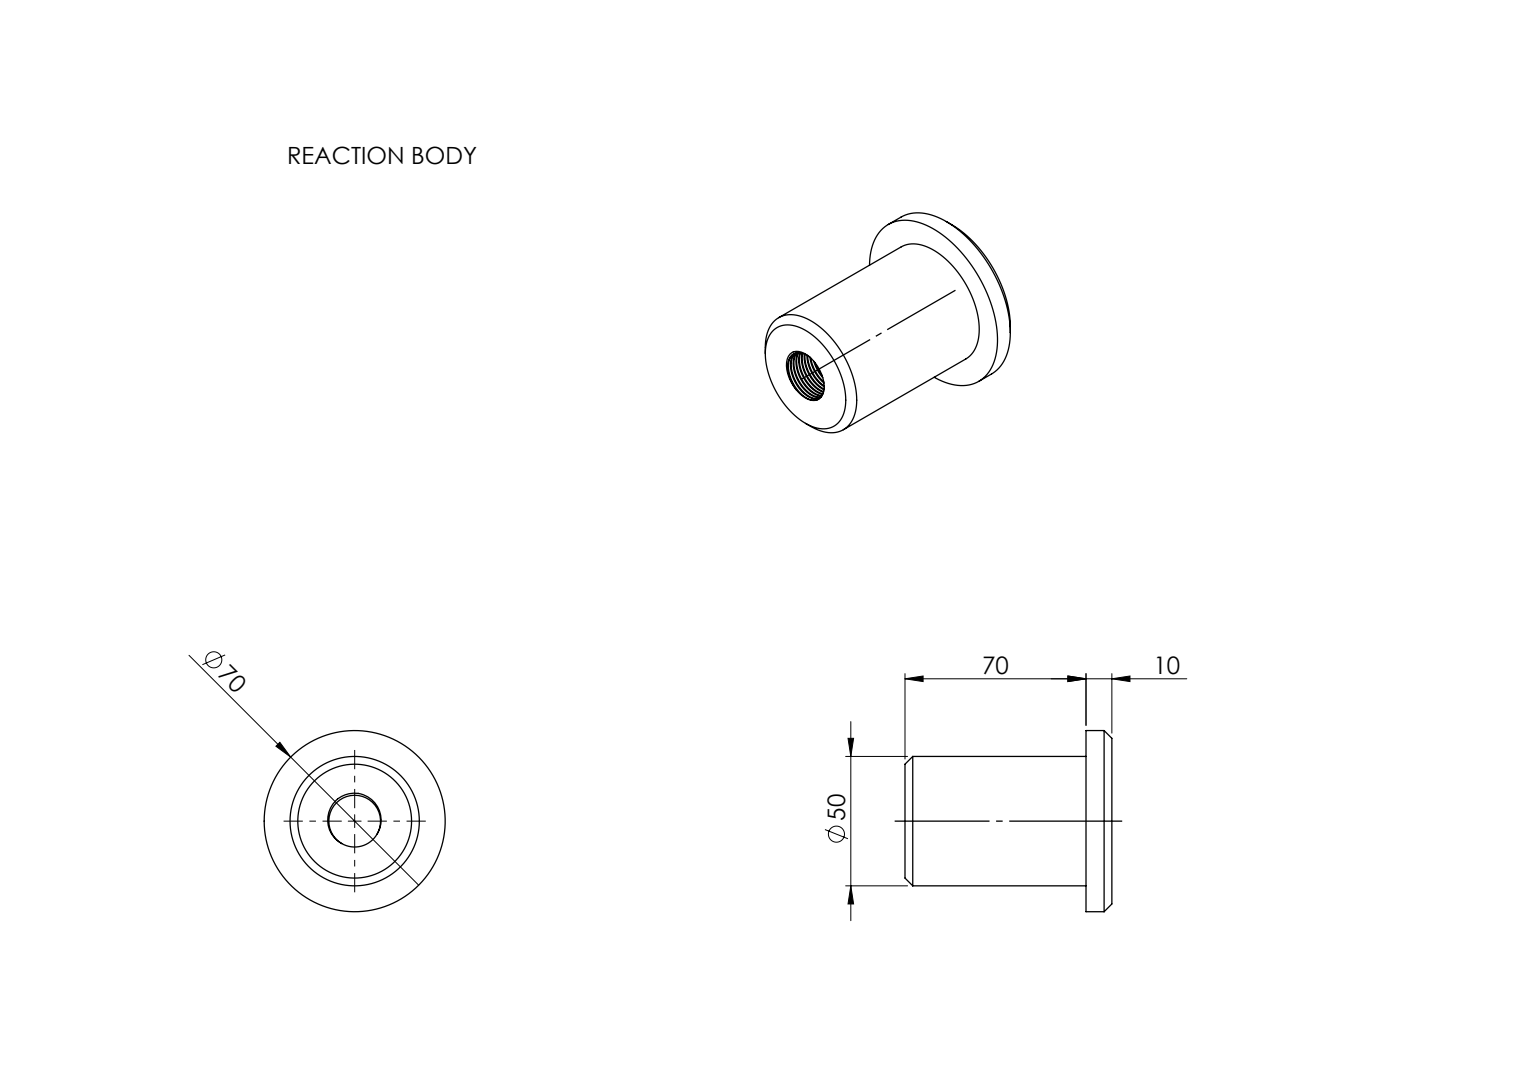
ISO-10303-21;
HEADER;
FILE_DESCRIPTION (('STEP AP203'),
    '1' );
FILE_NAME ('reaction body.step',
    '2026-09-28T05:57:06',
    ( '' ),
    ( '' ),
    'SwSTEP 2.0',
    'SolidWorks 2026',
    '' );
FILE_SCHEMA (( 'AUTOMOTIVE_DESIGN' ));
ENDSEC;

DATA;
#7=DIRECTION ( 'NONE',  ( -0.000000000000000000, -0.000000000000000000, -1.000000000000000000 ) ) ;
#8=CARTESIAN_POINT ( 'NONE',  ( -5.405949406249996869, 9.363379034771805109, -182.5312500020484094 ) ) ;
#10=DIRECTION ( 'NONE',  ( 0.000000000000000000, 0.000000000000000000, -1.000000000000000000 ) ) ;
#13=CARTESIAN_POINT ( 'NONE',  ( 10.81189881249999729, 0.000000000000000000, -100.3437500020483810 ) ) ;
#15=CARTESIAN_POINT ( 'NONE',  ( 10.81189881249999551, -6.242252689847874514, -106.6562500020483952 ) ) ;
#17=CARTESIAN_POINT ( 'NONE',  ( -10.81189881249999729, 6.242252689847871849, -113.2187500020483810 ) ) ;
#21=CARTESIAN_POINT ( 'NONE',  ( 5.000000000000000000, 8.660254037844385522, -142.7500000000000000 ) ) ;
#22=CARTESIAN_POINT ( 'NONE',  ( 4.999999999999992006, -8.660254037844389075, -2.249999999999974243 ) ) ;
#25=CARTESIAN_POINT ( 'NONE',  ( -9.999999999999998224, 5.773502691896259087, -178.7500000040967905 ) ) ;
#27=CARTESIAN_POINT ( 'NONE',  ( 10.81189881249999551, -6.242252689847874514, -29.96875000204834905 ) ) ;
#28=CARTESIAN_POINT ( 'NONE',  ( 5.000000000000000000, 8.660254037844385522, -117.2500000000000000 ) ) ;
#29=CARTESIAN_POINT ( 'NONE',  ( 5.405949406249992428, -9.363379034771808662, -141.0937500020483810 ) ) ;
#31=CARTESIAN_POINT ( 'NONE',  ( -2.293366432827344421E-15, -12.48450537969573659, -37.90625000204836681 ) ) ;
#32=( BOUNDED_CURVE ( )  B_SPLINE_CURVE ( 2, ( #493, #39950, #13606, #30683, #37364, #10382, #33502 ),
 .UNSPECIFIED., .F., .F. ) 
 B_SPLINE_CURVE_WITH_KNOTS ( ( 3, 2, 2, 3 ),
 ( 0.2462686567164180107, 0.2475124378109453960, 0.2487562189054727535, 0.2500000000000001110 ),
 .UNSPECIFIED. ) 
 CURVE ( )  GEOMETRIC_REPRESENTATION_ITEM ( )  RATIONAL_B_SPLINE_CURVE ( ( 0.9999999999999880096, 0.8660254037844506980, 1.000000000000000000, 0.8660254037844387076, 1.000000000000000000, 0.8660254037844267172, 1.000000000000011990 ) ) 
 REPRESENTATION_ITEM ( '' )  );
#34=CARTESIAN_POINT ( 'NONE',  ( 10.00000000000000000, 5.773502691896255534, -67.87500000000000000 ) ) ;
#35=CARTESIAN_POINT ( 'NONE',  ( 10.81189881249999729, 0.000000000000000000, -133.5312500020484094 ) ) ;
#37=ORIENTED_EDGE ( 'NONE', *, *, #14781, .T. ) ;
#38=CARTESIAN_POINT ( 'NONE',  ( -5.000000000000003553, -8.660254037844383745, -128.5000000000000000 ) ) ;
#39=CARTESIAN_POINT ( 'NONE',  ( 10.00000000000000000, 5.773502691896255534, -105.7500000040967905 ) ) ;
#41=CARTESIAN_POINT ( 'NONE',  ( -5.405949406250003975, -9.363379034771801557, -67.84375000204836681 ) ) ;
#47=CARTESIAN_POINT ( 'NONE',  ( 4.999999999999992006, -8.660254037844389075, -37.12500000409676915 ) ) ;
#55=EDGE_LOOP ( 'NONE', ( #10881, #42328, #28621, #40784 ) ) ;
#56=EDGE_CURVE ( 'NONE', #16041, #19819, #26737, .T. ) ;
#64=CARTESIAN_POINT ( 'NONE',  ( -2.293366432827344421E-15, -12.48450537969573659, -127.7187500020483668 ) ) ;
#65=CARTESIAN_POINT ( 'NONE',  ( -5.405949406249996869, 9.363379034771805109, -136.0312500020484094 ) ) ;
#67=CARTESIAN_POINT ( 'NONE',  ( -10.81189881249999729, -6.242252689847864744, -138.4687500020483810 ) ) ;
#68=CARTESIAN_POINT ( 'NONE',  ( 9.877642915644548438, -4.410630136379726451, -179.9999999999999716 ) ) ;
#69=( BOUNDED_CURVE ( )  B_SPLINE_CURVE ( 2, ( #4574, #21398, #14476, #34370, #4786, #36947, #20536 ),
 .UNSPECIFIED., .F., .F. ) 
 B_SPLINE_CURVE_WITH_KNOTS ( ( 3, 2, 2, 3 ),
 ( 0.1455223880597014963, 0.1467661691542288538, 0.1480099502487562391, 0.1492537313432835966 ),
 .UNSPECIFIED. ) 
 CURVE ( )  GEOMETRIC_REPRESENTATION_ITEM ( )  RATIONAL_B_SPLINE_CURVE ( ( 1.000000000000000000, 0.8660254037844387076, 1.000000000000000000, 0.8660254037844387076, 1.000000000000000000, 0.8660254037844357100, 1.000000000000003109 ) ) 
 REPRESENTATION_ITEM ( '' )  );
#70=CARTESIAN_POINT ( 'NONE',  ( 10.00000000000051159, -5.773502691895965988, -102.6249999999999858 ) ) ;
#71=CARTESIAN_POINT ( 'NONE',  ( 7.070501591499377789E-16, 11.54700538379251284, -165.1249999999999716 ) ) ;
#75=CARTESIAN_POINT ( 'NONE',  ( 10.81189881249999551, -6.242252689847874514, -53.96875000204837391 ) ) ;
#77=CARTESIAN_POINT ( 'NONE',  ( -2.293366432827344421E-15, -12.48450537969573659, -159.2187500020483810 ) ) ;
#81=CARTESIAN_POINT ( 'NONE',  ( 0.000000000000000000, 0.000000000000000000, -99.99999999999998579 ) ) ;
#83=CARTESIAN_POINT ( 'NONE',  ( 7.070501591499377789E-16, 11.54700538379251284, -90.12499999999997158 ) ) ;
#84=ORIENTED_EDGE ( 'NONE', *, *, #34120, .T. ) ;
#86=CARTESIAN_POINT ( 'NONE',  ( 5.405949406249992428, -9.363379034771808662, -112.7812500020483952 ) ) ;
#87=CARTESIAN_POINT ( 'NONE',  ( 9.999999999999998224, 0.000000000000000000, -129.8750000040967905 ) ) ;
#88=DIRECTION ( 'NONE',  ( -0.000000000000000000, -0.000000000000000000, -1.000000000000000000 ) ) ;
#92=CARTESIAN_POINT ( 'NONE',  ( -10.81189881249999729, 6.242252689847871849, -62.40625000204838813 ) ) ;
#99=DIRECTION ( 'NONE',  ( -0.000000000000000000, -0.000000000000000000, -1.000000000000000000 ) ) ;
#108=ORIENTED_EDGE ( 'NONE', *, *, #20529, .T. ) ;
#115=FACE_OUTER_BOUND ( 'NONE', #1522, .T. ) ;
#116=CARTESIAN_POINT ( 'NONE',  ( -9.999999999999998224, 1.224646799147353059E-15, -26.74999999999996803 ) ) ;
#120=CARTESIAN_POINT ( 'NONE',  ( -10.81189881249999907, -6.242252689847864744, -147.4687500020484094 ) ) ;
#121=CARTESIAN_POINT ( 'NONE',  ( -5.405949406249996869, 9.363379034771805109, -162.8437500020484094 ) ) ;
#124=CARTESIAN_POINT ( 'NONE',  ( -9.999999999999998224, 1.224646799147353059E-15, -188.7500000000000000 ) ) ;
#128=CARTESIAN_POINT ( 'NONE',  ( 10.81189881249999907, 6.242252689847868297, -184.2187500020483810 ) ) ;
#130=CARTESIAN_POINT ( 'NONE',  ( 5.405949406249992428, -9.363379034771808662, -51.28125000204835970 ) ) ;
#132=CARTESIAN_POINT ( 'NONE',  ( -9.999999999999998224, 1.224646799147353059E-15, -118.2500000000000000 ) ) ;
#135=CARTESIAN_POINT ( 'NONE',  ( -5.405949406249996869, 9.363379034771805109, -142.0312500020483810 ) ) ;
#136=CARTESIAN_POINT ( 'NONE',  ( -10.81189881249999729, 6.242252689847871849, -152.4062500020483810 ) ) ;
#141=CARTESIAN_POINT ( 'NONE',  ( -5.405949406249996869, 9.363379034771805109, -90.84375000204838102 ) ) ;
#142=ORIENTED_EDGE ( 'NONE', *, *, #37948, .T. ) ;
#144=CARTESIAN_POINT ( 'NONE',  ( -10.81189881249999729, 1.324075727343319199E-15, -186.5937500020483810 ) ) ;
#148=CARTESIAN_POINT ( 'NONE',  ( 10.81189881249999551, -6.242252689847874514, -81.15625000204839523 ) ) ;
#150=CARTESIAN_POINT ( 'NONE',  ( 5.000000000000000000, 8.660254037844385522, -57.62500000409676204 ) ) ;
#151=CARTESIAN_POINT ( 'NONE',  ( -10.81189881249999729, 6.242252689847871849, -17.21875000204836681 ) ) ;
#154=CARTESIAN_POINT ( 'NONE',  ( -10.81189881249999729, 6.242252689847871849, -11.40625000204836859 ) ) ;
#156=DIRECTION ( 'NONE',  ( -0.000000000000000000, -0.000000000000000000, -1.000000000000000000 ) ) ;
#158=CARTESIAN_POINT ( 'NONE',  ( 9.999999999999998224, 1.224646799147353059E-15, -99.99999999999998579 ) ) ;
#161=CARTESIAN_POINT ( 'NONE',  ( 0.000000000000000000, 0.000000000000000000, -99.99999999999998579 ) ) ;
#165=CARTESIAN_POINT ( 'NONE',  ( 10.81189881249999729, 6.242252689847867408, -101.7187500020483810 ) ) ;
#168=AXIS2_PLACEMENT_3D ( 'NONE', #1708, #40738, #1276 ) ;
#178=CARTESIAN_POINT ( 'NONE',  ( 5.405949406249999534, 9.363379034771803333, -149.7812500020483810 ) ) ;
#187=CARTESIAN_POINT ( 'NONE',  ( 5.405949406249999534, 9.363379034771803333, -74.59375000204838102 ) ) ;
#188=CARTESIAN_POINT ( 'NONE',  ( -10.81189881249999729, 1.324075727343319199E-15, -83.28125000204838102 ) ) ;
#190=CARTESIAN_POINT ( 'NONE',  ( -10.81189881249999729, -6.242252689847864744, -162.6562500020483810 ) ) ;
#191=CARTESIAN_POINT ( 'NONE',  ( -5.405949406249996869, 9.363379034771805109, -181.0312500020483810 ) ) ;
#192=CARTESIAN_POINT ( 'NONE',  ( -4.999999999999996447, 8.660254037844387298, -159.3750000040967905 ) ) ;
#194=CARTESIAN_POINT ( 'NONE',  ( -5.405949406250003975, -9.363379034771801557, -9.343750002048345493 ) ) ;
#196=CARTESIAN_POINT ( 'NONE',  ( -10.81189881249999729, 1.324075727343319199E-15, -113.0937500020483810 ) ) ;
#198=CARTESIAN_POINT ( 'NONE',  ( 10.81189881249999729, 0.000000000000000000, -13.53125000204835615 ) ) ;
#201=CARTESIAN_POINT ( 'NONE',  ( 5.405949406249999534, 9.363379034771803333, -112.2812500020483952 ) ) ;
#205=CARTESIAN_POINT ( 'NONE',  ( 9.999999999999996447, -5.773502691896262640, -83.50000000409676204 ) ) ;
#206=CARTESIAN_POINT ( 'NONE',  ( 9.999999999999742428, 5.773502691896404748, -134.2500000040967905 ) ) ;
#207=CARTESIAN_POINT ( 'NONE',  ( -10.81189881249999729, 1.324075727343319199E-15, -44.09375000204837391 ) ) ;
#208=ORIENTED_EDGE ( 'NONE', *, *, #27661, .F. ) ;
#212=CARTESIAN_POINT ( 'NONE',  ( 9.999999999999996447, -5.773502691896262640, -10.00000000409676026 ) ) ;
#215=CARTESIAN_POINT ( 'NONE',  ( 9.999999999999998224, 0.000000000000000000, -123.5000000000000000 ) ) ;
#218=ORIENTED_EDGE ( 'NONE', *, *, #5122, .T. ) ;
#223=VERTEX_POINT ( 'NONE', #23443 ) ;
#226=CARTESIAN_POINT ( 'NONE',  ( 10.81189881249999907, 6.242252689847868297, -182.9062500020484094 ) ) ;
#229=CARTESIAN_POINT ( 'NONE',  ( -5.405949406250003975, -9.363379034771801557, -102.3437500020483810 ) ) ;
#231=CARTESIAN_POINT ( 'NONE',  ( 10.81189881249999729, 0.000000000000000000, -105.0312500020483810 ) ) ;
#233=CARTESIAN_POINT ( 'NONE',  ( -5.405949406250003975, -9.363379034771801557, -115.8437500020483810 ) ) ;
#237=CARTESIAN_POINT ( 'NONE',  ( -9.999999999999998224, 1.224646799147353059E-15, -134.7499999999999716 ) ) ;
#238=CARTESIAN_POINT ( 'NONE',  ( -4.999999999999996447, 8.660254037844387298, -7.499999999999978684 ) ) ;
#241=CARTESIAN_POINT ( 'NONE',  ( -10.00000000000000000, -5.773502691896251982, -181.5000000040967905 ) ) ;
#243=CARTESIAN_POINT ( 'NONE',  ( 5.405949406249999534, 9.363379034771803333, -31.09375000204836326 ) ) ;
#245=CARTESIAN_POINT ( 'NONE',  ( 10.81189881249999907, 6.242252689847868297, -134.7187500020484094 ) ) ;
#247=CARTESIAN_POINT ( 'NONE',  ( 10.81189881249999729, 0.000000000000000000, -40.53125000204838102 ) ) ;
#249=CARTESIAN_POINT ( 'NONE',  ( 9.999999999999996447, -5.773502691896262640, -63.62499999999999289 ) ) ;
#250=CARTESIAN_POINT ( 'NONE',  ( 5.405949406249999534, 9.363379034771803333, -136.2812500020483810 ) ) ;
#253=ORIENTED_EDGE ( 'NONE', *, *, #28926, .T. ) ;
#254=CARTESIAN_POINT ( 'NONE',  ( -10.00000000000051337, 5.773502691895962435, -142.3750000000000000 ) ) ;
#255=CARTESIAN_POINT ( 'NONE',  ( -9.999999999999998224, 5.773502691896259087, -105.2500000040967763 ) ) ;
#256=CARTESIAN_POINT ( 'NONE',  ( -2.121150477449813534E-15, -11.54700538379251284, -146.3749999999999716 ) ) ;
#257=CARTESIAN_POINT ( 'NONE',  ( 10.81189881249999551, -6.242252689847874514, -67.46875000204838102 ) ) ;
#263=CARTESIAN_POINT ( 'NONE',  ( -10.00000000000000000, -5.773502691896251982, -39.00000000409676204 ) ) ;
#269=EDGE_CURVE ( 'NONE', #8961, #22977, #32528, .T. ) ;
#270=VERTEX_POINT ( 'NONE', #36591 ) ;
#274=CARTESIAN_POINT ( 'NONE',  ( 9.999999999999227285, 5.773502691896701400, -111.7500000040967478 ) ) ;
#279=CARTESIAN_POINT ( 'NONE',  ( -10.81189881249999729, 6.242252689847871849, -125.2187500020483810 ) ) ;
#280=CARTESIAN_POINT ( 'NONE',  ( 7.644554776091147741E-16, 12.48450537969573659, -128.6562500020483810 ) ) ;
#282=CARTESIAN_POINT ( 'NONE',  ( 10.81189881249999551, -6.242252689847874514, -139.4687500020483810 ) ) ;
#283=CARTESIAN_POINT ( 'NONE',  ( 10.64016988090102700, -2.046480638857292256, -180.0000000000000000 ) ) ;
#285=CARTESIAN_POINT ( 'NONE',  ( 7.070501591499377789E-16, 11.54700538379251284, -159.1250000000000000 ) ) ;
#286=CARTESIAN_POINT ( 'NONE',  ( -10.81189881249999729, 1.324075727343319199E-15, -0.7812500020483725827 ) ) ;
#289=CARTESIAN_POINT ( 'NONE',  ( -5.405949406249996869, 9.363379034771805109, -51.84375000204835260 ) ) ;
#291=CARTESIAN_POINT ( 'NONE',  ( 10.81189881249999551, -6.242252689847874514, -158.9687500020484094 ) ) ;
#296=CARTESIAN_POINT ( 'NONE',  ( -9.999999999999998224, 5.773502691896259087, -92.87500000000000000 ) ) ;
#297=ORIENTED_EDGE ( 'NONE', *, *, #13005, .T. ) ;
#298=CARTESIAN_POINT ( 'NONE',  ( -2.293366432827344421E-15, -12.48450537969573659, -112.9062500020483952 ) ) ;
#299=CARTESIAN_POINT ( 'NONE',  ( 10.00000000000000000, 5.773502691896255534, -128.2500000040967620 ) ) ;
#303=EDGE_CURVE ( 'NONE', #6776, #24567, #9100, .T. ) ;
#305=CARTESIAN_POINT ( 'NONE',  ( 5.405949406249999534, 9.363379034771803333, -50.78125000204835970 ) ) ;
#312=CARTESIAN_POINT ( 'NONE',  ( -4.999999999999996447, 8.660254037844387298, -130.8750000040967905 ) ) ;
#320=( BOUNDED_CURVE ( )  B_SPLINE_CURVE ( 2, ( #6511, #29389, #19660, #35453, #2432, #8903, #15567 ),
 .UNSPECIFIED., .F., .F. ) 
 B_SPLINE_CURVE_WITH_KNOTS ( ( 3, 2, 2, 3 ),
 ( 0.3955223880597015795, 0.3967661691542289648, 0.3980099502487563501, 0.3992537313432836799 ),
 .UNSPECIFIED. ) 
 CURVE ( )  GEOMETRIC_REPRESENTATION_ITEM ( )  RATIONAL_B_SPLINE_CURVE ( ( 0.9999999999999880096, 0.8660254037844506980, 1.000000000000000000, 0.8660254037844387076, 1.000000000000000000, 0.8660254037844267172, 1.000000000000011990 ) ) 
 REPRESENTATION_ITEM ( '' )  );
#327=CARTESIAN_POINT ( 'NONE',  ( -5.405949406249996869, 9.363379034771805109, -146.3437500020483810 ) ) ;
#328=CARTESIAN_POINT ( 'NONE',  ( 5.405949406249999534, 9.363379034771803333, -163.0937500020484094 ) ) ;
#330=( BOUNDED_CURVE ( )  B_SPLINE_CURVE ( 2, ( #4756, #1316, #14448, #8439, #17905, #11862, #34553 ),
 .UNSPECIFIED., .F., .F. ) 
 B_SPLINE_CURVE_WITH_KNOTS ( ( 3, 2, 2, 3 ),
 ( 0.1567164179104477695, 0.1579601990049751270, 0.1592039800995025123, 0.1604477611940298698 ),
 .UNSPECIFIED. ) 
 CURVE ( )  GEOMETRIC_REPRESENTATION_ITEM ( )  RATIONAL_B_SPLINE_CURVE ( ( 1.000000000000000000, 0.8660254037844387076, 1.000000000000000000, 0.8660254037844387076, 1.000000000000000000, 0.8660254037844357100, 1.000000000000003109 ) ) 
 REPRESENTATION_ITEM ( '' )  );
#331=FACE_OUTER_BOUND ( 'NONE', #10477, .T. ) ;
#332=CARTESIAN_POINT ( 'NONE',  ( -5.000000000000003553, -8.660254037844383745, -188.5000000000000000 ) ) ;
#335=CYLINDRICAL_SURFACE ( 'NONE', #35072, 9.999999999999998224 ) ;
#336=CARTESIAN_POINT ( 'NONE',  ( 7.644554776091147741E-16, 12.48450537969573659, -183.9687500020484094 ) ) ;
#339=CARTESIAN_POINT ( 'NONE',  ( 7.644554776091147741E-16, 12.48450537969573659, -50.65625000204837391 ) ) ;
#341=CARTESIAN_POINT ( 'NONE',  ( 5.000000000000000000, 8.660254037844385522, -112.7499999999999858 ) ) ;
#342=VERTEX_POINT ( 'NONE', #10257 ) ;
#344=CARTESIAN_POINT ( 'NONE',  ( 7.644554776091147741E-16, 12.48450537969573659, -137.6562500020484094 ) ) ;
#345=CARTESIAN_POINT ( 'NONE',  ( -10.81189881249999729, 1.324075727343319199E-15, -152.2812500020484094 ) ) ;
#347=CARTESIAN_POINT ( 'NONE',  ( -9.999999999999998224, 1.224646799147353059E-15, -125.7499999999999716 ) ) ;
#348=CARTESIAN_POINT ( 'NONE',  ( 10.81189881249999907, 6.242252689847868297, -82.21875000204836681 ) ) ;
#349=ORIENTED_EDGE ( 'NONE', *, *, #20808, .F. ) ;
#351=CARTESIAN_POINT ( 'NONE',  ( -2.293366432827344421E-15, -12.48450537969573659, -181.7187500020484094 ) ) ;
#357=CARTESIAN_POINT ( 'NONE',  ( -5.405949406250003975, -9.363379034771801557, -77.03125000204838102 ) ) ;
#360=CARTESIAN_POINT ( 'NONE',  ( -4.999999999999996447, 8.660254037844387298, -60.37500000409676204 ) ) ;
#361=CARTESIAN_POINT ( 'NONE',  ( 10.81189881249999907, 6.242252689847868297, -8.718750002048359704 ) ) ;
#364=CARTESIAN_POINT ( 'NONE',  ( -10.81189881249999729, 6.242252689847871849, -9.906250002048366810 ) ) ;
#366=CARTESIAN_POINT ( 'NONE',  ( 9.999999999999998224, 0.000000000000000000, -147.8750000040967905 ) ) ;
#369=CARTESIAN_POINT ( 'NONE',  ( -5.000000000000003553, -8.660254037844383745, -134.8750000040967905 ) ) ;
#374=CARTESIAN_POINT ( 'NONE',  ( -9.999999999999998224, 1.224646799147353059E-15, -160.6250000040967905 ) ) ;
#376=CARTESIAN_POINT ( 'NONE',  ( -5.405949406250003975, -9.363379034771801557, -100.8437500020483810 ) ) ;
#378=ORIENTED_EDGE ( 'NONE', *, *, #33115, .F. ) ;
#385=EDGE_CURVE ( 'NONE', #1917, #4764, #24732, .T. ) ;
#390=CARTESIAN_POINT ( 'NONE',  ( 10.81189881249999729, 0.000000000000000000, -145.5312500020483810 ) ) ;
#393=FACE_OUTER_BOUND ( 'NONE', #36030, .T. ) ;
#396=CARTESIAN_POINT ( 'NONE',  ( 10.81189881249999907, 6.242252689847868297, -73.21875000204836681 ) ) ;
#397=CARTESIAN_POINT ( 'NONE',  ( -10.81189881249999729, 1.324075727343319199E-15, -75.78125000204838102 ) ) ;
#399=DIRECTION ( 'NONE',  ( -1.000000000000000000, 0.000000000000000000, 0.000000000000000000 ) ) ;
#400=CARTESIAN_POINT ( 'NONE',  ( -10.81189881249999729, 1.324075727343319199E-15, -156.7812500020484094 ) ) ;
#401=CARTESIAN_POINT ( 'NONE',  ( -2.293366432827344421E-15, -12.48450537969573659, -168.4062500020483810 ) ) ;
#402=DIRECTION ( 'NONE',  ( -0.000000000000000000, -0.000000000000000000, -1.000000000000000000 ) ) ;
#403=CARTESIAN_POINT ( 'NONE',  ( -10.81189881249999729, 6.242252689847871849, -0.7187500020483517105 ) ) ;
#405=CARTESIAN_POINT ( 'NONE',  ( 10.81189881249999551, -6.242252689847874514, -107.9687500020483810 ) ) ;
#407=CARTESIAN_POINT ( 'NONE',  ( 10.81189881249999907, 6.242252689847868297, -13.40625000204837036 ) ) ;
#410=( BOUNDED_CURVE ( )  B_SPLINE_CURVE ( 2, ( #7723, #30182, #3850, #7503, #30606, #17408, #620 ),
 .UNSPECIFIED., .F., .F. ) 
 B_SPLINE_CURVE_WITH_KNOTS ( ( 3, 2, 2, 3 ),
 ( 0.1529850746268656692, 0.1542288557213930267, 0.1554726368159203842, 0.1567164179104477695 ),
 .UNSPECIFIED. ) 
 CURVE ( )  GEOMETRIC_REPRESENTATION_ITEM ( )  RATIONAL_B_SPLINE_CURVE ( ( 1.000000000000000000, 0.8660254037844387076, 1.000000000000000000, 0.8660254037844387076, 1.000000000000000000, 0.8660254037844387076, 1.000000000000000000 ) ) 
 REPRESENTATION_ITEM ( '' )  );
#412=CARTESIAN_POINT ( 'NONE',  ( 10.81189881249999729, 0.000000000000000000, -109.5312500020483810 ) ) ;
#415=ADVANCED_FACE ( 'NONE', ( #31205 ), #992, .F. ) ;
#416=CARTESIAN_POINT ( 'NONE',  ( -9.999999999999998224, 1.224646799147353059E-15, -87.12500000409677625 ) ) ;
#418=CARTESIAN_POINT ( 'NONE',  ( 10.81189881249999907, 6.242252689847868297, -41.71875000204835970 ) ) ;
#422=CARTESIAN_POINT ( 'NONE',  ( 9.999999999999998224, 0.000000000000000000, -140.0000000000000000 ) ) ;
#423=CARTESIAN_POINT ( 'NONE',  ( 4.999999999999992006, -8.660254037844389075, -13.12500000409674783 ) ) ;
#430=ORIENTED_EDGE ( 'NONE', *, *, #34123, .T. ) ;
#438=AXIS2_PLACEMENT_3D ( 'NONE', #20570, #30100, #539 ) ;
#441=CARTESIAN_POINT ( 'NONE',  ( -5.405949406250003975, -9.363379034771801557, -171.5312500020484094 ) ) ;
#442=CARTESIAN_POINT ( 'NONE',  ( -10.00000000000038547, 5.773502691896036154, -154.7500000040967905 ) ) ;
#444=CARTESIAN_POINT ( 'NONE',  ( 5.405949406249999534, 9.363379034771803333, -92.59375000204838102 ) ) ;
#446=CARTESIAN_POINT ( 'NONE',  ( 10.81189881249999907, 6.242252689847868297, -103.4062500020483952 ) ) ;
#448=CARTESIAN_POINT ( 'NONE',  ( -10.81189881249999729, 6.242252689847871849, -116.2187500020483810 ) ) ;
#450=( BOUNDED_CURVE ( )  B_SPLINE_CURVE ( 2, ( #33037, #22265, #38870, #35646, #2628, #12315, #3257 ),
 .UNSPECIFIED., .F., .F. ) 
 B_SPLINE_CURVE_WITH_KNOTS ( ( 3, 2, 2, 3 ),
 ( 0.2462686567164180107, 0.2475124378109453960, 0.2487562189054727535, 0.2500000000000001110 ),
 .UNSPECIFIED. ) 
 CURVE ( )  GEOMETRIC_REPRESENTATION_ITEM ( )  RATIONAL_B_SPLINE_CURVE ( ( 0.9999999999999880096, 0.8660254037844506980, 1.000000000000000000, 0.8660254037844387076, 1.000000000000000000, 0.8660254037844267172, 1.000000000000011990 ) ) 
 REPRESENTATION_ITEM ( '' )  );
#453=CARTESIAN_POINT ( 'NONE',  ( 5.000000000000000000, 8.660254037844385522, -7.749999999999978684 ) ) ;
#456=CARTESIAN_POINT ( 'NONE',  ( 10.00000000000000000, 5.773502691896255534, -180.7500000040968189 ) ) ;
#458=CARTESIAN_POINT ( 'NONE',  ( -5.405949406249996869, 9.363379034771805109, -30.84375000204836326 ) ) ;
#459=DIRECTION ( 'NONE',  ( -0.000000000000000000, -0.000000000000000000, -1.000000000000000000 ) ) ;
#460=CARTESIAN_POINT ( 'NONE',  ( 7.644554776091147741E-16, 12.48450537969573659, -140.4687500020483810 ) ) ;
#462=CARTESIAN_POINT ( 'NONE',  ( -5.405949406250003975, -9.363379034771801557, -38.03125000204838102 ) ) ;
#463=CARTESIAN_POINT ( 'NONE',  ( -5.000000000000003553, -8.660254037844383745, -148.0000000000000000 ) ) ;
#465=CARTESIAN_POINT ( 'NONE',  ( 5.000000000000000000, 8.660254037844385522, -57.24999999999996447 ) ) ;
#466=CARTESIAN_POINT ( 'NONE',  ( -10.81189881249999729, 6.242252689847871849, -128.4062500020484094 ) ) ;
#470=CARTESIAN_POINT ( 'NONE',  ( 7.070501591499377789E-16, 11.54700538379251284, -105.5000000040967763 ) ) ;
#472=CARTESIAN_POINT ( 'NONE',  ( 5.405949406249999534, 9.363379034771803333, -70.09375000204836681 ) ) ;
#478=CARTESIAN_POINT ( 'NONE',  ( -4.999999999999996447, 8.660254037844387298, -37.87500000409676915 ) ) ;
#490=CARTESIAN_POINT ( 'NONE',  ( 7.644554776091147741E-16, 12.48450537969573659, -196.1562500020484379 ) ) ;
#493=CARTESIAN_POINT ( 'NONE',  ( 9.999999999999998224, 0.000000000000000000, -150.5000000000000000 ) ) ;
#497=CARTESIAN_POINT ( 'NONE',  ( 5.405949406249999534, 9.363379034771803333, -127.0937500020483668 ) ) ;
#498=CARTESIAN_POINT ( 'NONE',  ( -10.00000000000000000, -5.773502691896251982, -193.5000000040967905 ) ) ;
#499=CARTESIAN_POINT ( 'NONE',  ( 5.405949406249992428, -9.363379034771808662, -135.2812500020483810 ) ) ;
#501=CARTESIAN_POINT ( 'NONE',  ( -10.81189881249999729, 6.242252689847871849, -135.7187500020483810 ) ) ;
#502=CARTESIAN_POINT ( 'NONE',  ( -2.121150477449813534E-15, -11.54700538379251284, -129.8750000000000000 ) ) ;
#504=CARTESIAN_POINT ( 'NONE',  ( 10.00000000000000000, 5.773502691896255534, -154.8750000000000000 ) ) ;
#508=CARTESIAN_POINT ( 'NONE',  ( -5.405949406249996869, 9.363379034771805109, -56.34375000204835970 ) ) ;
#509=CARTESIAN_POINT ( 'NONE',  ( -9.999999999999998224, 1.224646799147353059E-15, -142.2500000000000000 ) ) ;
#510=CARTESIAN_POINT ( 'NONE',  ( -10.81189881249999729, 6.242252689847871849, -165.7187500020483810 ) ) ;
#514=CARTESIAN_POINT ( 'NONE',  ( 5.000000000000000000, 8.660254037844385522, -87.24999999999998579 ) ) ;
#516=VERTEX_POINT ( 'NONE', #4861 ) ;
#517=CARTESIAN_POINT ( 'NONE',  ( 5.405949406249992428, -9.363379034771808662, -111.2812500020483810 ) ) ;
#518=CARTESIAN_POINT ( 'NONE',  ( 9.999999999999998224, 0.000000000000000000, -135.8750000040967905 ) ) ;
#519=CARTESIAN_POINT ( 'NONE',  ( -10.00000000000019185, -5.773502691896140071, -178.1249999999999432 ) ) ;
#522=CARTESIAN_POINT ( 'NONE',  ( 7.644554776091147741E-16, 12.48450537969573659, -49.15625000204837391 ) ) ;
#528=CARTESIAN_POINT ( 'NONE',  ( 7.070501591499376803E-16, 11.54700538379251284, -131.0000000040967905 ) ) ;
#530=VERTEX_POINT ( 'NONE', #27313 ) ;
#539=DIRECTION ( 'NONE',  ( -1.000000000000000000, 0.000000000000000000, 0.000000000000000000 ) ) ;
#542=CARTESIAN_POINT ( 'NONE',  ( -10.81189881249999907, -6.242252689847864744, -153.4687500020484094 ) ) ;
#543=CARTESIAN_POINT ( 'NONE',  ( 7.644554776091147741E-16, 12.48450537969573659, -164.4687500020483810 ) ) ;
#546=CARTESIAN_POINT ( 'NONE',  ( -4.999999999999996447, 8.660254037844387298, -183.0000000000000000 ) ) ;
#549=CARTESIAN_POINT ( 'NONE',  ( 9.999999999999998224, 0.000000000000000000, -168.8750000040967905 ) ) ;
#550=CARTESIAN_POINT ( 'NONE',  ( -10.81189881249999729, 6.242252689847871849, -188.2187500020483810 ) ) ;
#553=CARTESIAN_POINT ( 'NONE',  ( -10.81189881249999729, 6.242252689847871849, -51.90625000204837391 ) ) ;
#555=CARTESIAN_POINT ( 'NONE',  ( -2.121150477449813534E-15, -11.54700538379251284, -114.8749999999999716 ) ) ;
#556=ORIENTED_EDGE ( 'NONE', *, *, #24143, .F. ) ;
#557=CARTESIAN_POINT ( 'NONE',  ( 10.81189881249999551, -6.242252689847874514, -136.6562500020484094 ) ) ;
#558=CARTESIAN_POINT ( 'NONE',  ( -5.405949406250003975, -9.363379034771801557, -144.5312500020483810 ) ) ;
#560=CARTESIAN_POINT ( 'NONE',  ( -10.81189881249999729, 1.324075727343319199E-15, -80.09375000204838102 ) ) ;
#564=CARTESIAN_POINT ( 'NONE',  ( 5.405949406249992428, -9.363379034771808662, -181.5937500020483810 ) ) ;
#568=CARTESIAN_POINT ( 'NONE',  ( -5.405949406249996869, 9.363379034771805109, -77.53125000204838102 ) ) ;
#571=CARTESIAN_POINT ( 'NONE',  ( -9.999999999999998224, 5.773502691896259087, -49.75000000409676915 ) ) ;
#572=CARTESIAN_POINT ( 'NONE',  ( 10.81189881249999551, -6.242252689847874514, -8.968750002048359704 ) ) ;
#575=CARTESIAN_POINT ( 'NONE',  ( 10.81189881249999729, 0.000000000000000000, -4.531250002048375691 ) ) ;
#577=CARTESIAN_POINT ( 'NONE',  ( 7.320508151741852210, -7.320508031779506375, -100.0669873003032393 ) ) ;
#578=CARTESIAN_POINT ( 'NONE',  ( -9.999999999999227285, -5.773502691896698735, -103.5000000040967336 ) ) ;
#580=( BOUNDED_CURVE ( )  B_SPLINE_CURVE ( 2, ( #41162, #856, #11601, #23943, #21549, #20896, #11392 ),
 .UNSPECIFIED., .F., .F. ) 
 B_SPLINE_CURVE_WITH_KNOTS ( ( 3, 2, 2, 3 ),
 ( 0.4253731343283583266, 0.4266169154228856564, 0.4278606965174130417, 0.4291044776119404269 ),
 .UNSPECIFIED. ) 
 CURVE ( )  GEOMETRIC_REPRESENTATION_ITEM ( )  RATIONAL_B_SPLINE_CURVE ( ( 0.9999999999999880096, 0.8660254037844506980, 1.000000000000000000, 0.8660254037844387076, 1.000000000000000000, 0.8660254037844267172, 1.000000000000011990 ) ) 
 REPRESENTATION_ITEM ( '' )  );
#581=CARTESIAN_POINT ( 'NONE',  ( -9.999999999999998224, 1.224646799147353059E-15, -146.7500000000000000 ) ) ;
#583=ORIENTED_EDGE ( 'NONE', *, *, #23598, .F. ) ;
#585=CARTESIAN_POINT ( 'NONE',  ( 3.516324526667281347, 10.45435446766629894, -100.0500568239963002 ) ) ;
#595=CARTESIAN_POINT ( 'NONE',  ( 4.999999999999992006, -8.660254037844389075, -45.74999999999998579 ) ) ;
#601=CARTESIAN_POINT ( 'NONE',  ( 7.644554776091147741E-16, 12.48450537969573659, -149.6562500020484094 ) ) ;
#603=LINE ( 'NONE', #13718, #29480 ) ;
#608=CARTESIAN_POINT ( 'NONE',  ( -10.81189881249999729, 6.242252689847871849, -72.71875000204835260 ) ) ;
#609=CARTESIAN_POINT ( 'NONE',  ( -5.405949406249996869, 9.363379034771805109, -73.03125000204838102 ) ) ;
#611=CARTESIAN_POINT ( 'NONE',  ( 5.405949406249992428, -9.363379034771808662, -159.2812500020484094 ) ) ;
#612=CARTESIAN_POINT ( 'NONE',  ( 5.405949406249999534, 9.363379034771803333, -170.7812500020484094 ) ) ;
#614=DIRECTION ( 'NONE',  ( -0.000000000000000000, -0.000000000000000000, -1.000000000000000000 ) ) ;
#616=CARTESIAN_POINT ( 'NONE',  ( 10.81189881249999729, 0.000000000000000000, -107.8437500020483810 ) ) ;
#618=CARTESIAN_POINT ( 'NONE',  ( -10.81189881249999729, 1.324075727343319199E-15, -8.281250002048350822 ) ) ;
#620=CARTESIAN_POINT ( 'NONE',  ( 9.999999999999998224, 0.000000000000000000, -168.5000000000000000 ) ) ;
#621=CARTESIAN_POINT ( 'NONE',  ( 10.81189881249999729, 0.000000000000000000, -99.03125000204839523 ) ) ;
#623=CARTESIAN_POINT ( 'NONE',  ( 7.070501591499377789E-16, 11.54700538379251284, -75.50000000409677625 ) ) ;
#624=CARTESIAN_POINT ( 'NONE',  ( 9.999999999999998224, 0.000000000000000000, -146.3750000040967905 ) ) ;
#625=CARTESIAN_POINT ( 'NONE',  ( 10.81189881249999907, 6.242252689847868297, -32.71875000204835260 ) ) ;
#628=CARTESIAN_POINT ( 'NONE',  ( 5.405949406249999534, 9.363379034771803333, -31.28125000204837036 ) ) ;
#630=CARTESIAN_POINT ( 'NONE',  ( -9.999999999999998224, 1.224646799147353059E-15, -139.2499999999999716 ) ) ;
#633=CARTESIAN_POINT ( 'NONE',  ( -9.999999999999998224, 1.224646799147353059E-15, -13.62500000409674961 ) ) ;
#635=CARTESIAN_POINT ( 'NONE',  ( 7.070501591499376803E-16, 11.54700538379251284, -123.1249999999999858 ) ) ;
#637=ORIENTED_EDGE ( 'NONE', *, *, #8821, .T. ) ;
#642=SHAPE_DEFINITION_REPRESENTATION ( #7327, #6779 ) ;
#650=CARTESIAN_POINT ( 'NONE',  ( 7.644554776091147741E-16, 12.48450537969573659, -169.1562500020484094 ) ) ;
#651=EDGE_CURVE ( 'NONE', #26892, #19714, #35826, .T. ) ;
#655=CARTESIAN_POINT ( 'NONE',  ( 5.405949406249992428, -9.363379034771808662, -93.09375000204838102 ) ) ;
#656=CARTESIAN_POINT ( 'NONE',  ( -4.999999999999996447, 8.660254037844387298, -154.5000000000000000 ) ) ;
#657=CARTESIAN_POINT ( 'NONE',  ( -5.405949406250003975, -9.363379034771801557, -98.03125000204839523 ) ) ;
#659=CARTESIAN_POINT ( 'NONE',  ( 5.405949406249999534, 9.363379034771803333, -110.5937500020483810 ) ) ;
#662=CARTESIAN_POINT ( 'NONE',  ( 10.81189881249999729, 0.000000000000000000, -178.5312500020483810 ) ) ;
#663=CARTESIAN_POINT ( 'NONE',  ( 7.644554776091147741E-16, 12.48450537969573659, -196.1562500020484379 ) ) ;
#665=VECTOR ( 'NONE', #4017, 1000.000000000000000 ) ;
#667=CARTESIAN_POINT ( 'NONE',  ( 9.999999999999998224, 0.000000000000000000, -173.3750000040968189 ) ) ;
#669=CARTESIAN_POINT ( 'NONE',  ( -5.405949406249996869, 9.363379034771805109, -21.84375000204835615 ) ) ;
#671=CARTESIAN_POINT ( 'NONE',  ( -2.293366432827344421E-15, -12.48450537969573659, -126.2187500020483952 ) ) ;
#673=CARTESIAN_POINT ( 'NONE',  ( -10.81189881249999729, 6.242252689847871849, -29.40625000204835260 ) ) ;
#675=CARTESIAN_POINT ( 'NONE',  ( 7.070501591499377789E-16, 11.54700538379251284, -55.62499999999998579 ) ) ;
#676=CARTESIAN_POINT ( 'NONE',  ( -5.405949406250003975, -9.363379034771801557, -123.5312500020483952 ) ) ;
#681=CARTESIAN_POINT ( 'NONE',  ( 4.999999999999992006, -8.660254037844389075, -104.6250000040967763 ) ) ;
#682=CARTESIAN_POINT ( 'NONE',  ( 9.999999999999872102, 5.773502691896329253, -162.3750000000000000 ) ) ;
#683=CARTESIAN_POINT ( 'NONE',  ( -5.405949406250003975, -9.363379034771801557, -60.34375000204835970 ) ) ;
#687=CARTESIAN_POINT ( 'NONE',  ( 4.999999999999992006, -8.660254037844389075, -38.62500000409676915 ) ) ;
#691=EDGE_LOOP ( 'NONE', ( #4059, #17804, #37681, #25112 ) ) ;
#694=DIRECTION ( 'NONE',  ( -0.000000000000000000, -0.000000000000000000, -1.000000000000000000 ) ) ;
#698=CARTESIAN_POINT ( 'NONE',  ( 10.81189881249999729, 0.000000000000000000, -198.0312500020484094 ) ) ;
#704=CARTESIAN_POINT ( 'NONE',  ( 10.81189881249999551, -6.242252689847874514, -115.4687500020483810 ) ) ;
#705=CARTESIAN_POINT ( 'NONE',  ( 9.999999999999998224, 0.000000000000000000, -192.8750000040967905 ) ) ;
#706=CARTESIAN_POINT ( 'NONE',  ( -5.405949406249996869, 9.363379034771805109, -127.0312500020483952 ) ) ;
#708=CARTESIAN_POINT ( 'NONE',  ( 10.81189881249999729, 6.242252689847867408, -136.2187500020483810 ) ) ;
#709=CARTESIAN_POINT ( 'NONE',  ( 5.000000000000000000, 8.660254037844385522, -163.7500000000000000 ) ) ;
#711=CARTESIAN_POINT ( 'NONE',  ( -4.999999999999996447, 8.660254037844387298, -151.5000000000000000 ) ) ;
#712=CARTESIAN_POINT ( 'NONE',  ( -9.999999999999998224, 1.224646799147353059E-15, -19.24999999999996092 ) ) ;
#718=CARTESIAN_POINT ( 'NONE',  ( 10.81189881249999729, 0.000000000000000000, -44.84375000204837391 ) ) ;
#720=CARTESIAN_POINT ( 'NONE',  ( -10.81189881249999729, 1.324075727343319199E-15, -156.5937500020483810 ) ) ;
#724=CARTESIAN_POINT ( 'NONE',  ( 4.999999999999992006, -8.660254037844389075, -84.74999999999997158 ) ) ;
#727=CARTESIAN_POINT ( 'NONE',  ( 5.405949406249992428, -9.363379034771808662, -108.2812500020483810 ) ) ;
#728=CARTESIAN_POINT ( 'NONE',  ( 5.000000000000000000, 8.660254037844385522, -134.1250000040967620 ) ) ;
#729=CARTESIAN_POINT ( 'NONE',  ( -9.999999999999998224, 1.224646799147353059E-15, -115.6250000040967905 ) ) ;
#732=DIRECTION ( 'NONE',  ( -0.000000000000000000, -0.000000000000000000, -1.000000000000000000 ) ) ;
#733=CARTESIAN_POINT ( 'NONE',  ( -2.293366432827344421E-15, -12.48450537969573659, -49.90625000204838102 ) ) ;
#748=FACE_OUTER_BOUND ( 'NONE', #30201, .T. ) ;
#752=CARTESIAN_POINT ( 'NONE',  ( 7.644554776091147741E-16, 12.48450537969573659, -143.4687500020483810 ) ) ;
#753=CARTESIAN_POINT ( 'NONE',  ( 5.405949406249992428, -9.363379034771808662, -163.5937500020484094 ) ) ;
#755=DIRECTION ( 'NONE',  ( -0.000000000000000000, -0.000000000000000000, -1.000000000000000000 ) ) ;
#756=CARTESIAN_POINT ( 'NONE',  ( -5.000000000000003553, -8.660254037844383745, -182.5000000000000000 ) ) ;
#759=CARTESIAN_POINT ( 'NONE',  ( -10.81189881249999907, -6.242252689847864744, -175.9687500020483526 ) ) ;
#762=CARTESIAN_POINT ( 'NONE',  ( 10.81189881249999907, 6.242252689847868297, -52.40625000204838102 ) ) ;
#764=CARTESIAN_POINT ( 'NONE',  ( -5.000000000000003553, -8.660254037844383745, -104.4999999999999858 ) ) ;
#765=ORIENTED_EDGE ( 'NONE', *, *, #1965, .F. ) ;
#766=CARTESIAN_POINT ( 'NONE',  ( 5.405949406249992428, -9.363379034771808662, -138.2812500020483810 ) ) ;
#767=CARTESIAN_POINT ( 'NONE',  ( -10.81189881249999907, -6.242252689847864744, -150.6562500020484094 ) ) ;
#769=CARTESIAN_POINT ( 'NONE',  ( -10.81189881249999729, 6.242252689847871849, -84.71875000204836681 ) ) ;
#772=CARTESIAN_POINT ( 'NONE',  ( -5.405949406250003975, -9.363379034771801557, -181.8437500020483810 ) ) ;
#776=CARTESIAN_POINT ( 'NONE',  ( 7.644554776091147741E-16, 12.48450537969573659, -76.15625000204839523 ) ) ;
#779=CARTESIAN_POINT ( 'NONE',  ( 10.00000000000000000, 5.773502691896255534, -51.75000000409676204 ) ) ;
#780=CARTESIAN_POINT ( 'NONE',  ( -10.81189881249999729, 1.324075727343319199E-15, -8.093750002048343717 ) ) ;
#784=CARTESIAN_POINT ( 'NONE',  ( -10.81189881249999907, -6.242252689847864744, -6.656250002048364145 ) ) ;
#787=CARTESIAN_POINT ( 'NONE',  ( 9.999999999999998224, 0.000000000000000000, -102.8750000040967763 ) ) ;
#788=FACE_OUTER_BOUND ( 'NONE', #14986, .T. ) ;
#791=ORIENTED_EDGE ( 'NONE', *, *, #21137, .T. ) ;
#800=CARTESIAN_POINT ( 'NONE',  ( -9.999999999999742428, -5.773502691896402084, -122.6249999999999858 ) ) ;
#801=CARTESIAN_POINT ( 'NONE',  ( 7.070501591499377789E-16, 11.54700538379251284, -43.62499999999996447 ) ) ;
#808=LINE ( 'NONE', #1232, #21898 ) ;
#814=CARTESIAN_POINT ( 'NONE',  ( -2.293366432827344421E-15, -12.48450537969573659, -66.21875000204838102 ) ) ;
#815=CARTESIAN_POINT ( 'NONE',  ( -2.293366432827344421E-15, -12.48450537969573659, -78.40625000204838102 ) ) ;
#818=CARTESIAN_POINT ( 'NONE',  ( -10.81189881249999729, -6.242252689847864744, -158.1562500020484094 ) ) ;
#819=CARTESIAN_POINT ( 'NONE',  ( -10.81189881249999729, 6.242252689847871849, -170.4062500020484094 ) ) ;
#821=PLANE ( 'NONE',  #20595 ) ;
#823=CARTESIAN_POINT ( 'NONE',  ( -5.405949406249996869, 9.363379034771805109, -102.8437500020483810 ) ) ;
#824=DIRECTION ( 'NONE',  ( -0.000000000000000000, -0.000000000000000000, -1.000000000000000000 ) ) ;
#826=CARTESIAN_POINT ( 'NONE',  ( -5.405949406250003975, -9.363379034771801557, -3.531250002048374803 ) ) ;
#828=CARTESIAN_POINT ( 'NONE',  ( 10.81189881249999551, -6.242252689847874514, -100.6562500020483952 ) ) ;
#830=( BOUNDED_CURVE ( )  B_SPLINE_CURVE ( 2, ( #36833, #13512, #36415, #10287, #3833, #30164, #23686 ),
 .UNSPECIFIED., .F., .F. ) 
 B_SPLINE_CURVE_WITH_KNOTS ( ( 3, 2, 2, 3 ),
 ( 0.2910447761194031036, 0.2922885572139304333, 0.2935323383084578186, 0.2947761194029852039 ),
 .UNSPECIFIED. ) 
 CURVE ( )  GEOMETRIC_REPRESENTATION_ITEM ( )  RATIONAL_B_SPLINE_CURVE ( ( 0.9999999999999880096, 0.8660254037844506980, 1.000000000000000000, 0.8660254037844387076, 1.000000000000000000, 0.8660254037844267172, 1.000000000000011990 ) ) 
 REPRESENTATION_ITEM ( '' )  );
#831=CARTESIAN_POINT ( 'NONE',  ( -5.000000000000003553, -8.660254037844383745, -77.87500000409677625 ) ) ;
#832=CARTESIAN_POINT ( 'NONE',  ( 10.81189881249999907, 6.242252689847868297, -37.21875000204835260 ) ) ;
#835=CARTESIAN_POINT ( 'NONE',  ( 10.81189881249999907, 6.242252689847868297, -25.40625000204838102 ) ) ;
#839=CARTESIAN_POINT ( 'NONE',  ( 9.999999999999996447, -5.773502691896262640, -5.500000004096755823 ) ) ;
#841=AXIS2_PLACEMENT_3D ( 'NONE', #9008, #5137, #34714 ) ;
#849=ORIENTED_EDGE ( 'NONE', *, *, #18345, .F. ) ;
#855=ORIENTED_EDGE ( 'NONE', *, *, #34933, .F. ) ;
#856=CARTESIAN_POINT ( 'NONE',  ( 9.999999999999479527, 5.773502691896553074, -114.3749999999999716 ) ) ;
#858=CARTESIAN_POINT ( 'NONE',  ( -5.405949406250003975, -9.363379034771801557, -176.0312500020483810 ) ) ;
#861=CARTESIAN_POINT ( 'NONE',  ( 10.81189881249999907, 6.242252689847868297, -92.71875000204836681 ) ) ;
#863=CARTESIAN_POINT ( 'NONE',  ( 5.405949406249992428, -9.363379034771808662, -102.2812500020483952 ) ) ;
#865=CARTESIAN_POINT ( 'NONE',  ( 10.81189881249999551, -6.242252689847874514, -109.4687500020483952 ) ) ;
#869=CARTESIAN_POINT ( 'NONE',  ( 5.405949406249992428, -9.363379034771808662, -193.7812500020484094 ) ) ;
#872=CARTESIAN_POINT ( 'NONE',  ( -2.121150477449813534E-15, -11.54700538379251284, -173.7500000040968189 ) ) ;
#874=CARTESIAN_POINT ( 'NONE',  ( -5.405949406250003975, -9.363379034771801557, -19.84375000204835615 ) ) ;
#875=FACE_OUTER_BOUND ( 'NONE', #15728, .T. ) ;
#876=CARTESIAN_POINT ( 'NONE',  ( -10.81189881249999907, -6.242252689847864744, -133.9687500020483810 ) ) ;
#878=CARTESIAN_POINT ( 'NONE',  ( -10.81189881249999729, 1.324075727343319199E-15, -32.28125000204837391 ) ) ;
#879=CARTESIAN_POINT ( 'NONE',  ( -5.000000000000003553, -8.660254037844383745, -57.99999999999997158 ) ) ;
#880=CARTESIAN_POINT ( 'NONE',  ( -10.81189881249999907, -6.242252689847864744, -123.6562500020484094 ) ) ;
#882=ORIENTED_EDGE ( 'NONE', *, *, #22628, .F. ) ;
#884=CARTESIAN_POINT ( 'NONE',  ( 7.070501591499377789E-16, 11.54700538379251284, -104.0000000040967763 ) ) ;
#886=CARTESIAN_POINT ( 'NONE',  ( -2.293366432827344421E-15, -12.48450537969573659, -61.71875000204837391 ) ) ;
#887=ORIENTED_EDGE ( 'NONE', *, *, #16169, .T. ) ;
#892=CARTESIAN_POINT ( 'NONE',  ( 7.070501591499377789E-16, 11.54700538379251284, -30.50000000409674783 ) ) ;
#893=ADVANCED_FACE ( 'NONE', ( #38728 ), #31847, .F. ) ;
#895=CYLINDRICAL_SURFACE ( 'NONE', #29343, 9.999999999999998224 ) ;
#902=( BOUNDED_CURVE ( )  B_SPLINE_CURVE ( 2, ( #15846, #28631, #22560, #29046, #28420, #31441, #38756 ),
 .UNSPECIFIED., .F., .F. ) 
 B_SPLINE_CURVE_WITH_KNOTS ( ( 3, 2, 2, 3 ),
 ( 0.3619402985074628432, 0.3631840796019901729, 0.3644278606965175027, 0.3656716417910448325 ),
 .UNSPECIFIED. ) 
 CURVE ( )  GEOMETRIC_REPRESENTATION_ITEM ( )  RATIONAL_B_SPLINE_CURVE ( ( 0.9999999999999820144, 0.8660254037844566932, 1.000000000000000000, 0.8660254037844387076, 1.000000000000000000, 0.8660254037844327124, 1.000000000000005995 ) ) 
 REPRESENTATION_ITEM ( '' )  );
#906=CARTESIAN_POINT ( 'NONE',  ( 5.405949406249992428, -9.363379034771808662, -198.2812500020484094 ) ) ;
#912=CARTESIAN_POINT ( 'NONE',  ( 10.81189881249999551, -6.242252689847874514, -118.4687500020483810 ) ) ;
#913=CARTESIAN_POINT ( 'NONE',  ( 5.000000000000000000, 8.660254037844385522, -195.6250000040967905 ) ) ;
#914=CARTESIAN_POINT ( 'NONE',  ( 10.81189881249999907, 6.242252689847868297, -121.4062500020483810 ) ) ;
#916=CARTESIAN_POINT ( 'NONE',  ( 5.405949406249999534, 9.363379034771803333, -131.5937500020483810 ) ) ;
#919=CARTESIAN_POINT ( 'NONE',  ( 5.000000000000000000, 8.660254037844385522, -154.7500000000000000 ) ) ;
#920=CARTESIAN_POINT ( 'NONE',  ( 7.070501591499377789E-16, 11.54700538379251284, -19.62499999999997513 ) ) ;
#924=CARTESIAN_POINT ( 'NONE',  ( -10.81189881249999907, -6.242252689847864744, -43.96875000204835970 ) ) ;
#926=CARTESIAN_POINT ( 'NONE',  ( -10.81189881249999729, 6.242252689847871849, -153.7187500020483526 ) ) ;
#930=CARTESIAN_POINT ( 'NONE',  ( 6.220436543609608293, 8.439850853362262484, -179.9999999999998863 ) ) ;
#931=CARTESIAN_POINT ( 'NONE',  ( 4.999999999999992006, -8.660254037844389075, -86.24999999999998579 ) ) ;
#934=CARTESIAN_POINT ( 'NONE',  ( -10.81189881249999729, 6.242252689847871849, -110.4062500020483810 ) ) ;
#935=CARTESIAN_POINT ( 'NONE',  ( 10.00000000000000000, 5.773502691896255534, -125.2500000040967905 ) ) ;
#938=CARTESIAN_POINT ( 'NONE',  ( 9.999999999999998224, 0.000000000000000000, -129.8750000040967905 ) ) ;
#939=CARTESIAN_POINT ( 'NONE',  ( -2.293366432827344421E-15, -12.48450537969573659, -55.90625000204838102 ) ) ;
#944=ORIENTED_EDGE ( 'NONE', *, *, #33581, .T. ) ;
#946=ORIENTED_EDGE ( 'NONE', *, *, #37567, .T. ) ;
#956=FACE_OUTER_BOUND ( 'NONE', #6211, .T. ) ;
#961=CARTESIAN_POINT ( 'NONE',  ( -2.293366432827344421E-15, -12.48450537969573659, -142.7187500020484094 ) ) ;
#962=CARTESIAN_POINT ( 'NONE',  ( -10.81189881249999729, 1.324075727343319199E-15, -150.5937500020483810 ) ) ;
#965=CARTESIAN_POINT ( 'NONE',  ( -4.999999999999996447, 8.660254037844387298, -181.5000000000000000 ) ) ;
#969=CARTESIAN_POINT ( 'NONE',  ( 7.070501591499376803E-16, 11.54700538379251284, -168.5000000040967620 ) ) ;
#970=CARTESIAN_POINT ( 'NONE',  ( -10.81189881249999729, 1.324075727343319199E-15, -182.0937500020483810 ) ) ;
#973=CARTESIAN_POINT ( 'NONE',  ( 10.81189881249999729, 0.000000000000000000, -49.53125000204838813 ) ) ;
#975=CARTESIAN_POINT ( 'NONE',  ( -10.00000000000000000, -5.773502691896251982, -110.6249999999999858 ) ) ;
#977=CARTESIAN_POINT ( 'NONE',  ( -10.81189881249999729, 6.242252689847871849, -132.9062500020483810 ) ) ;
#978=CARTESIAN_POINT ( 'NONE',  ( 7.070501591499377789E-16, 11.54700538379251284, -146.0000000040967905 ) ) ;
#979=CARTESIAN_POINT ( 'NONE',  ( -10.81189881249999729, 6.242252689847871849, -147.9062500020483810 ) ) ;
#981=CARTESIAN_POINT ( 'NONE',  ( 5.405949406249992428, -9.363379034771808662, -85.59375000204836681 ) ) ;
#984=CARTESIAN_POINT ( 'NONE',  ( -10.81189881249999729, 6.242252689847871849, -180.7187500020483810 ) ) ;
#987=CARTESIAN_POINT ( 'NONE',  ( -5.000000000000003553, -8.660254037844383745, -158.5000000000000000 ) ) ;
#988=CARTESIAN_POINT ( 'NONE',  ( 7.644554776091147741E-16, 12.48450537969573659, -74.65625000204838102 ) ) ;
#990=CARTESIAN_POINT ( 'NONE',  ( 5.000000000000000000, 8.660254037844385522, -51.62500000409675494 ) ) ;
#991=CARTESIAN_POINT ( 'NONE',  ( -10.81189881249999729, 6.242252689847871849, -12.71875000204836326 ) ) ;
#992=CYLINDRICAL_SURFACE ( 'NONE', #29713, 9.999999999999998224 ) ;
#994=CARTESIAN_POINT ( 'NONE',  ( -10.81189881249999729, 1.324075727343319199E-15, -6.781250002048377468 ) ) ;
#998=CYLINDRICAL_SURFACE ( 'NONE', #23130, 24.99999999999999645 ) ;
#1002=VERTEX_POINT ( 'NONE', #35708 ) ;
#1003=( LENGTH_UNIT ( ) NAMED_UNIT ( * ) SI_UNIT ( .MILLI., .METRE. ) );
#1011=CARTESIAN_POINT ( 'NONE',  ( 9.999999999999996447, -5.773502691896262640, -42.62499999999997158 ) ) ;
#1013=CARTESIAN_POINT ( 'NONE',  ( 10.81189881249999551, -6.242252689847874514, -163.4687500020483810 ) ) ;
#1018=CARTESIAN_POINT ( 'NONE',  ( 9.999999999999998224, 0.000000000000000000, -200.0000000000000000 ) ) ;
#1023=CARTESIAN_POINT ( 'NONE',  ( -10.81189881249999907, -6.242252689847864744, -70.96875000204838102 ) ) ;
#1024=CARTESIAN_POINT ( 'NONE',  ( -10.81189881249999907, -6.242252689847864744, -80.15625000204839523 ) ) ;
#1026=CARTESIAN_POINT ( 'NONE',  ( -10.00000000000000000, -5.773502691896251982, -133.1250000000000000 ) ) ;
#1027=CARTESIAN_POINT ( 'NONE',  ( -5.405949406250003975, -9.363379034771801557, -156.5312500020484094 ) ) ;
#1028=CARTESIAN_POINT ( 'NONE',  ( -10.81189881249999907, -6.242252689847864744, -174.6562500020483810 ) ) ;
#1030=CARTESIAN_POINT ( 'NONE',  ( -5.405949406249996869, 9.363379034771805109, -105.8437500020483810 ) ) ;
#1031=CARTESIAN_POINT ( 'NONE',  ( 9.999999999999998224, 0.000000000000000000, -146.0000000000000000 ) ) ;
#1033=CARTESIAN_POINT ( 'NONE',  ( -2.293366432827344421E-15, -12.48450537969573659, -4.906250002048362369 ) ) ;
#1035=CARTESIAN_POINT ( 'NONE',  ( 10.81189881249999729, 0.000000000000000000, -100.5312500020483952 ) ) ;
#1037=CARTESIAN_POINT ( 'NONE',  ( 7.070501591499377789E-16, 11.54700538379251284, -72.50000000409676204 ) ) ;
#1039=CARTESIAN_POINT ( 'NONE',  ( 10.81189881249999907, 6.242252689847868297, -31.21875000204835260 ) ) ;
#1040=ORIENTED_EDGE ( 'NONE', *, *, #22283, .F. ) ;
#1042=CARTESIAN_POINT ( 'NONE',  ( -10.81189881249999729, 6.242252689847871849, -29.40625000204835260 ) ) ;
#1045=CARTESIAN_POINT ( 'NONE',  ( 5.000000000000000000, 8.660254037844385522, -0.6250000040967651493 ) ) ;
#1047=EDGE_CURVE ( 'NONE', #8327, #13549, #2902, .T. ) ;
#1049=DIRECTION ( 'NONE',  ( -1.000000000000000000, 0.000000000000000000, 0.000000000000000000 ) ) ;
#1051=ORIENTED_EDGE ( 'NONE', *, *, #12971, .T. ) ;
#1052=CARTESIAN_POINT ( 'NONE',  ( 0.000000000000000000, 0.000000000000000000, -180.0000000000000000 ) ) ;
#1063=CARTESIAN_POINT ( 'NONE',  ( -2.293366432827344421E-15, -12.48450537969573659, -169.9062500020483810 ) ) ;
#1067=CARTESIAN_POINT ( 'NONE',  ( -5.405949406249996869, 9.363379034771805109, -93.84375000204838102 ) ) ;
#1068=CARTESIAN_POINT ( 'NONE',  ( 9.999999999999998224, 0.000000000000000000, -106.9999999999999858 ) ) ;
#1069=CARTESIAN_POINT ( 'NONE',  ( -5.405949406249996869, 9.363379034771805109, -104.5312500020483810 ) ) ;
#1071=CARTESIAN_POINT ( 'NONE',  ( 10.81189881249999729, 6.242252689847867408, -107.7187500020483810 ) ) ;
#1074=CARTESIAN_POINT ( 'NONE',  ( 10.81189881249999551, -6.242252689847874514, -198.1562500020484379 ) ) ;
#1077=CARTESIAN_POINT ( 'NONE',  ( 5.000000000000000000, 8.660254037844385522, -176.1250000040968189 ) ) ;
#1079=CARTESIAN_POINT ( 'NONE',  ( 7.644554776091147741E-16, 12.48450537969573659, -18.96875000204837036 ) ) ;
#1080=DIRECTION ( 'NONE',  ( -0.000000000000000000, -0.000000000000000000, -1.000000000000000000 ) ) ;
#1081=CARTESIAN_POINT ( 'NONE',  ( -10.81189881249999729, 6.242252689847871849, -132.7187500020483810 ) ) ;
#1083=CARTESIAN_POINT ( 'NONE',  ( 10.81189881249999729, 0.000000000000000000, -31.53125000204837391 ) ) ;
#1086=CARTESIAN_POINT ( 'NONE',  ( -9.999999999999998224, 5.773502691896259087, -61.37499999999998579 ) ) ;
#1087=CARTESIAN_POINT ( 'NONE',  ( 7.644554776091147741E-16, 12.48450537969573659, -127.1562500020483952 ) ) ;
#1090=CARTESIAN_POINT ( 'NONE',  ( -9.999999999999998224, 0.000000000000000000, -99.99999999999998579 ) ) ;
#1091=CARTESIAN_POINT ( 'NONE',  ( 4.999999999999992006, -8.660254037844389075, -97.12500000409677625 ) ) ;
#1092=CARTESIAN_POINT ( 'NONE',  ( 10.00000000000051159, -5.773502691895965988, -151.0000000040967905 ) ) ;
#1093=CARTESIAN_POINT ( 'NONE',  ( 5.405949406249999534, 9.363379034771803333, -59.59375000204835970 ) ) ;
#1099=CARTESIAN_POINT ( 'NONE',  ( -10.00000000000000000, -5.773502691896251982, -31.50000000409674783 ) ) ;
#1104=CARTESIAN_POINT ( 'NONE',  ( -9.999999999999998224, 1.224646799147353059E-15, -129.1250000040967620 ) ) ;
#1108=DIRECTION ( 'NONE',  ( -0.000000000000000000, -0.000000000000000000, -1.000000000000000000 ) ) ;
#1111=CARTESIAN_POINT ( 'NONE',  ( 10.81189881249999551, -6.242252689847874514, -198.1562500020484379 ) ) ;
#1117=EDGE_CURVE ( 'NONE', #21693, #23210, #25367, .T. ) ;
#1119=CARTESIAN_POINT ( 'NONE',  ( -10.81189881249999907, -6.242252689847864744, -118.9687500020483810 ) ) ;
#1120=CARTESIAN_POINT ( 'NONE',  ( 10.00000000000000000, 5.773502691896255534, -195.7500000040968189 ) ) ;
#1122=CARTESIAN_POINT ( 'NONE',  ( 10.81189881249999729, 0.000000000000000000, -123.0312500020483952 ) ) ;
#1124=CARTESIAN_POINT ( 'NONE',  ( 10.81189881249999729, 0.000000000000000000, -127.3437500020483952 ) ) ;
#1127=CARTESIAN_POINT ( 'NONE',  ( -2.121150477449813534E-15, -11.54700538379251284, -158.3750000000000000 ) ) ;
#1128=CARTESIAN_POINT ( 'NONE',  ( -9.999999999999998224, 1.224646799147353059E-15, -17.74999999999996092 ) ) ;
#1131=CARTESIAN_POINT ( 'NONE',  ( 10.00000000000025402, -5.773502691896113426, -158.5000000040968473 ) ) ;
#1133=CARTESIAN_POINT ( 'NONE',  ( -5.405949406249996869, 9.363379034771805109, -42.84375000204837391 ) ) ;
#1135=CARTESIAN_POINT ( 'NONE',  ( -10.81189881249999729, 6.242252689847871849, -150.7187500020483810 ) ) ;
#1138=CARTESIAN_POINT ( 'NONE',  ( 7.564846744322244021, 7.391372818874605066, -180.0000000000000284 ) ) ;
#1139=CARTESIAN_POINT ( 'NONE',  ( -5.000000000000003553, -8.660254037844383745, -83.49999999999997158 ) ) ;
#1142=CARTESIAN_POINT ( 'NONE',  ( -2.293366432827344421E-15, -12.48450537969573659, -105.4062500020483810 ) ) ;
#1143=CARTESIAN_POINT ( 'NONE',  ( 9.999999999999996447, -5.773502691896262640, -121.0000000040967905 ) ) ;
#1144=CARTESIAN_POINT ( 'NONE',  ( -9.999999999999998224, 1.224646799147353059E-15, -154.6250000040967905 ) ) ;
#1148=CARTESIAN_POINT ( 'NONE',  ( -5.405949406250003975, -9.363379034771801557, -53.03125000204836681 ) ) ;
#1149=CARTESIAN_POINT ( 'NONE',  ( 4.999999999999992006, -8.660254037844389075, -135.7499999999999716 ) ) ;
#1152=CARTESIAN_POINT ( 'NONE',  ( -9.999999999999998224, 1.224646799147353059E-15, -178.6250000040968189 ) ) ;
#1154=EDGE_CURVE ( 'NONE', #530, #15993, #14272, .T. ) ;
#1162=CARTESIAN_POINT ( 'NONE',  ( -9.999999999999998224, 1.224646799147353059E-15, -129.1250000040967620 ) ) ;
#1171=CARTESIAN_POINT ( 'NONE',  ( -10.81189881249999729, 1.324075727343319199E-15, -144.5937500020483810 ) ) ;
#1172=CARTESIAN_POINT ( 'NONE',  ( -5.405949406249996869, 9.363379034771805109, -155.3437500020483810 ) ) ;
#1175=CARTESIAN_POINT ( 'NONE',  ( 10.00000000000025402, -5.773502691896113426, -139.0000000040967905 ) ) ;
#1176=CARTESIAN_POINT ( 'NONE',  ( -10.00000000000000000, -5.773502691896251982, -178.1250000000000284 ) ) ;
#1182=CARTESIAN_POINT ( 'NONE',  ( 10.81189881249999729, 0.000000000000000000, -181.3437500020483810 ) ) ;
#1186=CARTESIAN_POINT ( 'NONE',  ( 5.405949406249999534, 9.363379034771803333, -41.78125000204838102 ) ) ;
#1188=CARTESIAN_POINT ( 'NONE',  ( 7.070501591499377789E-16, 11.54700538379251284, -103.6249999999999858 ) ) ;
#1189=ORIENTED_EDGE ( 'NONE', *, *, #11626, .T. ) ;
#1190=CARTESIAN_POINT ( 'NONE',  ( 10.81189881249999551, -6.242252689847874514, -138.1562500020484094 ) ) ;
#1191=CARTESIAN_POINT ( 'NONE',  ( 9.999999999999998224, 0.000000000000000000, -150.8750000040967905 ) ) ;
#1192=CARTESIAN_POINT ( 'NONE',  ( -10.81189881249999729, 6.242252689847871849, -146.4062500020484094 ) ) ;
#1194=ORIENTED_EDGE ( 'NONE', *, *, #6940, .T. ) ;
#1196=CARTESIAN_POINT ( 'NONE',  ( 5.405949406249999534, 9.363379034771803333, -179.5937500020484094 ) ) ;
#1199=CARTESIAN_POINT ( 'NONE',  ( 10.81189881249999551, -6.242252689847874514, -73.65625000204836681 ) ) ;
#1201=EDGE_CURVE ( 'NONE', #41907, #40786, #11267, .T. ) ;
#1202=( BOUNDED_CURVE ( )  B_SPLINE_CURVE ( 2, ( #8969, #22135, #35309, #5739, #19512, #22982, #29456 ),
 .UNSPECIFIED., .F., .F. ) 
 B_SPLINE_CURVE_WITH_KNOTS ( ( 3, 2, 2, 3 ),
 ( 0.4291044776119404269, 0.4303482587064677567, 0.4315920398009951975, 0.4328358208955225273 ),
 .UNSPECIFIED. ) 
 CURVE ( )  GEOMETRIC_REPRESENTATION_ITEM ( )  RATIONAL_B_SPLINE_CURVE ( ( 0.9999999999999880096, 0.8660254037844506980, 1.000000000000000000, 0.8660254037844387076, 1.000000000000000000, 0.8660254037844207220, 1.000000000000017986 ) ) 
 REPRESENTATION_ITEM ( '' )  );
#1203=CARTESIAN_POINT ( 'NONE',  ( 7.070501591499377789E-16, 11.54700538379251284, -56.00000000409676915 ) ) ;
#1205=CARTESIAN_POINT ( 'NONE',  ( -5.405949406250003975, -9.363379034771801557, -13.84375000204834905 ) ) ;
#1207=CARTESIAN_POINT ( 'NONE',  ( -5.405949406250003975, -9.363379034771801557, -6.531250002048377468 ) ) ;
#1208=FACE_OUTER_BOUND ( 'NONE', #31158, .T. ) ;
#1209=CARTESIAN_POINT ( 'NONE',  ( -9.999999999999998224, 1.224646799147353059E-15, -148.2500000000000000 ) ) ;
#1225=CARTESIAN_POINT ( 'NONE',  ( -10.00000000000000000, -5.773502691896251982, -47.62499999999997158 ) ) ;
#1227=CARTESIAN_POINT ( 'NONE',  ( 7.644554776091147741E-16, 12.48450537969573659, -167.4687500020483810 ) ) ;
#1229=CARTESIAN_POINT ( 'NONE',  ( -5.000000000000003553, -8.660254037844383745, -99.99999999999998579 ) ) ;
#1232=CARTESIAN_POINT ( 'NONE',  ( -9.999999999999998224, 0.000000000000000000, -99.99999999999998579 ) ) ;
#1235=AXIS2_PLACEMENT_3D ( 'NONE', #20101, #3926, #25440 ) ;
#1239=CARTESIAN_POINT ( 'NONE',  ( -5.405949406249996869, 9.363379034771805109, -71.34375000204836681 ) ) ;
#1240=CARTESIAN_POINT ( 'NONE',  ( 7.644554776091147741E-16, 12.48450537969573659, -77.65625000204838102 ) ) ;
#1242=CARTESIAN_POINT ( 'NONE',  ( -10.00000000000000000, -5.773502691896251982, -128.6250000000000000 ) ) ;
#1243=CARTESIAN_POINT ( 'NONE',  ( 10.81189881249999551, -6.242252689847874514, -162.1562500020484094 ) ) ;
#1244=CARTESIAN_POINT ( 'NONE',  ( -5.405949406250003975, -9.363379034771801557, -174.5312500020484094 ) ) ;
#1246=FACE_BOUND ( 'NONE', #18987, .T. ) ;
#1248=CARTESIAN_POINT ( 'NONE',  ( 10.81189881249999907, 6.242252689847868297, -107.7187500020483810 ) ) ;
#1251=CARTESIAN_POINT ( 'NONE',  ( -5.405949406249996869, 9.363379034771805109, -4.031250002048375691 ) ) ;
#1254=CARTESIAN_POINT ( 'NONE',  ( 10.81189881249999551, -6.242252689847874514, -103.6562500020483668 ) ) ;
#1256=CARTESIAN_POINT ( 'NONE',  ( -10.00000000000000000, -5.773502691896251982, -79.50000000409679046 ) ) ;
#1257=CARTESIAN_POINT ( 'NONE',  ( 5.000000000000000000, 8.660254037844385522, -118.7500000000000000 ) ) ;
#1258=CARTESIAN_POINT ( 'NONE',  ( -5.405949406250003975, -9.363379034771801557, -30.34375000204836326 ) ) ;
#1261=CARTESIAN_POINT ( 'NONE',  ( -5.405949406250003975, -9.363379034771801557, -32.03125000204837391 ) ) ;
#1264=CARTESIAN_POINT ( 'NONE',  ( 9.999999999999998224, 0.000000000000000000, -0.8750000040967653714 ) ) ;
#1276=DIRECTION ( 'NONE',  ( -1.000000000000000000, 0.000000000000000000, 0.000000000000000000 ) ) ;
#1277=CARTESIAN_POINT ( 'NONE',  ( 3.018241686408907221, 10.32067256058293481, -99.99999999999997158 ) ) ;
#1279=CARTESIAN_POINT ( 'NONE',  ( 5.405949406249992428, -9.363379034771808662, -172.7812500020484094 ) ) ;
#1282=CARTESIAN_POINT ( 'NONE',  ( 5.405949406249999534, 9.363379034771803333, -91.09375000204838102 ) ) ;
#1285=CARTESIAN_POINT ( 'NONE',  ( 10.81189881249999551, -6.242252689847874514, -100.6562500020483952 ) ) ;
#1287=CARTESIAN_POINT ( 'NONE',  ( -10.81189881249999729, 6.242252689847871849, -104.2187500020483810 ) ) ;
#1290=CARTESIAN_POINT ( 'NONE',  ( -10.00000000000076916, 5.773502691895813221, -132.2500000040967620 ) ) ;
#1291=CARTESIAN_POINT ( 'NONE',  ( 5.405949406249999534, 9.363379034771803333, -199.2812500020484094 ) ) ;
#1293=CARTESIAN_POINT ( 'NONE',  ( 4.999999999999992006, -8.660254037844389075, -175.1250000040968189 ) ) ;
#1295=CARTESIAN_POINT ( 'NONE',  ( -5.405949406250003975, -9.363379034771801557, -22.84375000204835615 ) ) ;
#1296=CARTESIAN_POINT ( 'NONE',  ( 10.81189881249999907, 6.242252689847868297, -133.2187500020483810 ) ) ;
#1298=CARTESIAN_POINT ( 'NONE',  ( -5.405949406250003975, -9.363379034771801557, -29.03125000204837036 ) ) ;
#1301=CARTESIAN_POINT ( 'NONE',  ( 9.999999999999996447, -5.773502691896262640, -59.12499999999998579 ) ) ;
#1302=CARTESIAN_POINT ( 'NONE',  ( -2.293366432827344421E-15, -12.48450537969573659, -121.9062500020483952 ) ) ;
#1304=ORIENTED_EDGE ( 'NONE', *, *, #385, .T. ) ;
#1306=CARTESIAN_POINT ( 'NONE',  ( 7.070501591499377789E-16, 11.54700538379251284, -98.00000000409677625 ) ) ;
#1308=CARTESIAN_POINT ( 'NONE',  ( 7.644554776091147741E-16, 12.48450537969573659, -57.96875000204837391 ) ) ;
#1315=CARTESIAN_POINT ( 'NONE',  ( 10.00000000000000000, 5.773502691896255534, -24.75000000409677270 ) ) ;
#1316=CARTESIAN_POINT ( 'NONE',  ( 10.00000000000000000, 5.773502691896255534, -168.3750000000000000 ) ) ;
#1324=AXIS2_PLACEMENT_3D ( 'NONE', #15425, #28623, #25380 ) ;
#1325=CYLINDRICAL_SURFACE ( 'NONE', #23143, 9.999999999999998224 ) ;
#1328=CARTESIAN_POINT ( 'NONE',  ( 10.81189881249999907, 6.242252689847868297, -194.9062500020484379 ) ) ;
#1335=CARTESIAN_POINT ( 'NONE',  ( -10.81189881249999907, -6.242252689847864744, -114.4687500020483810 ) ) ;
#1336=CARTESIAN_POINT ( 'NONE',  ( 9.999999999999998224, 0.000000000000000000, -194.3750000040967905 ) ) ;
#1337=CARTESIAN_POINT ( 'NONE',  ( 5.405949406249999534, 9.363379034771803333, -127.2812500020483810 ) ) ;
#1339=CARTESIAN_POINT ( 'NONE',  ( -10.81189881249999729, -6.242252689847864744, -133.9687500020483810 ) ) ;
#1340=CARTESIAN_POINT ( 'NONE',  ( -5.000000000000003553, -8.660254037844383745, -166.3750000040967905 ) ) ;
#1343=CARTESIAN_POINT ( 'NONE',  ( -5.000000000000003553, -8.660254037844383745, -143.5000000000000000 ) ) ;
#1344=CARTESIAN_POINT ( 'NONE',  ( -2.121150477449813534E-15, -11.54700538379251284, -20.37499999999997513 ) ) ;
#1347=DIRECTION ( 'NONE',  ( -1.000000000000000000, 0.000000000000000000, 0.000000000000000000 ) ) ;
#1349=CARTESIAN_POINT ( 'NONE',  ( -5.405949406249996869, 9.363379034771805109, -48.84375000204838102 ) ) ;
#1350=CARTESIAN_POINT ( 'NONE',  ( 10.81189881249999907, 6.242252689847868297, -152.7187500020483810 ) ) ;
#1353=CARTESIAN_POINT ( 'NONE',  ( 3.970414520298676031, 9.602429920229235805, -180.0000000000001705 ) ) ;
#1354=CARTESIAN_POINT ( 'NONE',  ( 9.999999999999998224, 0.000000000000000000, -79.99999999999998579 ) ) ;
#1357=CARTESIAN_POINT ( 'NONE',  ( 10.81189881249999551, -6.242252689847874514, -105.1562500020483810 ) ) ;
#1358=CARTESIAN_POINT ( 'NONE',  ( 5.000000000000000000, 8.660254037844385522, -128.1250000040967620 ) ) ;
#1359=CARTESIAN_POINT ( 'NONE',  ( -2.121150477449813534E-15, -11.54700538379251284, -143.7500000040967905 ) ) ;
#1362=CARTESIAN_POINT ( 'NONE',  ( 10.81189881249999907, 6.242252689847868297, -47.90625000204837391 ) ) ;
#1369=EDGE_LOOP ( 'NONE', ( #15629, #29218, #26146, #12790 ) ) ;
#1372=AXIS2_PLACEMENT_3D ( 'NONE', #81, #29426, #10193 ) ;
#1373=ORIENTED_EDGE ( 'NONE', *, *, #7404, .F. ) ;
#1375=ORIENTED_EDGE ( 'NONE', *, *, #12974, .F. ) ;
#1380=CARTESIAN_POINT ( 'NONE',  ( 9.999999999999998224, 0.000000000000000000, -152.3750000040967905 ) ) ;
#1384=CARTESIAN_POINT ( 'NONE',  ( -2.293366432827344421E-15, -12.48450537969573659, -145.7187500020484094 ) ) ;
#1385=CARTESIAN_POINT ( 'NONE',  ( 10.81189881249999729, 0.000000000000000000, -150.0312500020483810 ) ) ;
#1386=CARTESIAN_POINT ( 'NONE',  ( -5.405949406250003975, -9.363379034771801557, -154.8437500020483810 ) ) ;
#1388=CARTESIAN_POINT ( 'NONE',  ( -2.121150477449813534E-15, -11.54700538379251284, -139.2500000040967905 ) ) ;
#1389=CARTESIAN_POINT ( 'NONE',  ( 4.999999999999992006, -8.660254037844389075, -179.2500000000000284 ) ) ;
#1395=CARTESIAN_POINT ( 'NONE',  ( 10.81189881249999551, -6.242252689847874514, -181.4687500020484094 ) ) ;
#1398=CYLINDRICAL_SURFACE ( 'NONE', #38576, 9.999999999999998224 ) ;
#1399=CARTESIAN_POINT ( 'NONE',  ( -10.81189881249999729, 6.242252689847871849, -41.40625000204836681 ) ) ;
#1401=CARTESIAN_POINT ( 'NONE',  ( -5.000000000000003553, -8.660254037844383745, -110.4999999999999858 ) ) ;
#1403=CARTESIAN_POINT ( 'NONE',  ( -10.81189881249999729, 6.242252689847871849, -129.9062500020483810 ) ) ;
#1404=CARTESIAN_POINT ( 'NONE',  ( 7.070501591499377789E-16, 11.54700538379251284, -152.0000000040967905 ) ) ;
#1405=CYLINDRICAL_SURFACE ( 'NONE', #22230, 9.999999999999998224 ) ;
#1409=CARTESIAN_POINT ( 'NONE',  ( 10.81189881249999729, 0.000000000000000000, -173.8437500020484094 ) ) ;
#1412=( BOUNDED_CURVE ( )  B_SPLINE_CURVE ( 2, ( #12336, #12550, #41693, #35248, #28560, #34822, #34607 ),
 .UNSPECIFIED., .F., .F. ) 
 B_SPLINE_CURVE_WITH_KNOTS ( ( 3, 2, 2, 3 ),
 ( 0.1231343283582089221, 0.1243781094527362935, 0.1256218905472636649, 0.1268656716417910224 ),
 .UNSPECIFIED. ) 
 CURVE ( )  GEOMETRIC_REPRESENTATION_ITEM ( )  RATIONAL_B_SPLINE_CURVE ( ( 1.000000000000002887, 0.8660254037844355990, 1.000000000000000000, 0.8660254037844387076, 1.000000000000000000, 0.8660254037844417052, 0.9999999999999970024 ) ) 
 REPRESENTATION_ITEM ( '' )  );
#1414=CARTESIAN_POINT ( 'NONE',  ( 7.644554776091147741E-16, 12.48450537969573659, -67.15625000204838102 ) ) ;
#1416=CARTESIAN_POINT ( 'NONE',  ( -10.00000000000000000, -5.773502691896251982, -49.50000000409676915 ) ) ;
#1417=CARTESIAN_POINT ( 'NONE',  ( -5.405949406249996869, 9.363379034771805109, -5.343750002048369474 ) ) ;
#1420=LINE ( 'NONE', #14554, #21342 ) ;
#1423=CARTESIAN_POINT ( 'NONE',  ( 0.000000000000000000, 0.000000000000000000, -99.99999999999998579 ) ) ;
#1427=EDGE_LOOP ( 'NONE', ( #33363, #21517, #24368, #7565 ) ) ;
#1437=CARTESIAN_POINT ( 'NONE',  ( -9.999999999999998224, 5.773502691896259087, -44.87499999999997868 ) ) ;
#1439=CARTESIAN_POINT ( 'NONE',  ( 5.405949406249999534, 9.363379034771803333, -166.0937500020484094 ) ) ;
#1440=CARTESIAN_POINT ( 'NONE',  ( 10.81189881249999729, 0.000000000000000000, -176.8437500020483810 ) ) ;
#1442=CARTESIAN_POINT ( 'NONE',  ( 9.999999999999998224, 1.224646799147353059E-15, -99.99999999999998579 ) ) ;
#1447=DIRECTION ( 'NONE',  ( -0.000000000000000000, -0.000000000000000000, -1.000000000000000000 ) ) ;
#1450=CARTESIAN_POINT ( 'NONE',  ( 10.81189881249999551, -6.242252689847874514, -59.96875000204837391 ) ) ;
#1451=CARTESIAN_POINT ( 'NONE',  ( -10.81189881249999729, 6.242252689847871849, -69.90625000204839523 ) ) ;
#1453=CARTESIAN_POINT ( 'NONE',  ( -9.999999999999998224, 1.224646799147353059E-15, -130.2499999999999716 ) ) ;
#1455=CARTESIAN_POINT ( 'NONE',  ( 7.644554776091147741E-16, 12.48450537969573659, -146.6562500020484094 ) ) ;
#1456=CARTESIAN_POINT ( 'NONE',  ( 10.81189881249999907, 6.242252689847868297, -166.4062500020483810 ) ) ;
#1460=CARTESIAN_POINT ( 'NONE',  ( 10.81189881249999907, 6.242252689847868297, -100.2187500020483810 ) ) ;
#1461=CARTESIAN_POINT ( 'NONE',  ( 0.000000000000000000, 0.000000000000000000, -99.99999999999998579 ) ) ;
#1463=CARTESIAN_POINT ( 'NONE',  ( 5.405949406249999534, 9.363379034771803333, -193.0937500020484094 ) ) ;
#1465=CARTESIAN_POINT ( 'NONE',  ( 5.339643252401987006, -9.254418622957800267, -180.0000000000000000 ) ) ;
#1466=CARTESIAN_POINT ( 'NONE',  ( -10.81189881249999729, 6.242252689847871849, -98.40625000204838102 ) ) ;
#1469=CARTESIAN_POINT ( 'NONE',  ( 9.999999999999996447, -5.773502691896262640, -79.00000000409677625 ) ) ;
#1471=CARTESIAN_POINT ( 'NONE',  ( -2.293366432827344421E-15, -12.48450537969573659, -37.71875000204835970 ) ) ;
#1474=CARTESIAN_POINT ( 'NONE',  ( -5.405949406249996869, 9.363379034771805109, -25.03125000204836681 ) ) ;
#1477=CARTESIAN_POINT ( 'NONE',  ( -10.00000000000000000, -5.773502691896251982, -4.500000004096754047 ) ) ;
#1482=ORIENTED_EDGE ( 'NONE', *, *, #30429, .T. ) ;
#1484=ORIENTED_EDGE ( 'NONE', *, *, #33061, .T. ) ;
#1495=CARTESIAN_POINT ( 'NONE',  ( 10.81189881249999551, -6.242252689847874514, -165.1562500020483526 ) ) ;
#1499=CARTESIAN_POINT ( 'NONE',  ( 5.405949406249999534, 9.363379034771803333, -89.59375000204838102 ) ) ;
#1501=CARTESIAN_POINT ( 'NONE',  ( 10.81189881249999907, 6.242252689847868297, -193.2187500020484094 ) ) ;
#1502=CARTESIAN_POINT ( 'NONE',  ( -2.293366432827344421E-15, -12.48450537969573659, -88.90625000204838102 ) ) ;
#1504=CARTESIAN_POINT ( 'NONE',  ( 10.81189881249999729, 0.000000000000000000, -109.3437500020483810 ) ) ;
#1506=CARTESIAN_POINT ( 'NONE',  ( 10.00000000000051159, -5.773502691895965988, -150.6250000000000000 ) ) ;
#1507=CARTESIAN_POINT ( 'NONE',  ( 10.81189881249999551, -6.242252689847874514, -171.1562500020484094 ) ) ;
#1508=CARTESIAN_POINT ( 'NONE',  ( -5.405949406249996869, 9.363379034771805109, -197.5312500020484094 ) ) ;
#1510=CARTESIAN_POINT ( 'NONE',  ( 5.000000000000000000, 8.660254037844385522, -171.6250000040968189 ) ) ;
#1512=CARTESIAN_POINT ( 'NONE',  ( -10.81189881249999907, -6.242252689847864744, -19.96875000204837036 ) ) ;
#1514=CARTESIAN_POINT ( 'NONE',  ( 10.81189881249999729, 0.000000000000000000, -118.3437500020483810 ) ) ;
#1516=CARTESIAN_POINT ( 'NONE',  ( 5.405949406249999534, 9.363379034771803333, -25.28125000204836681 ) ) ;
#1519=CARTESIAN_POINT ( 'NONE',  ( 10.00000000000000000, 5.773502691896255534, -54.37499999999997868 ) ) ;
#1520=CARTESIAN_POINT ( 'NONE',  ( -10.81189881249999729, 6.242252689847871849, -120.9062500020483952 ) ) ;
#1522=EDGE_LOOP ( 'NONE', ( #14719, #38827, #7628, #15946 ) ) ;
#1523=VECTOR ( 'NONE', #7678, 1000.000000000000000 ) ;
#1524=CARTESIAN_POINT ( 'NONE',  ( 9.999999999999996447, -5.773502691896262640, -100.0000000040967763 ) ) ;
#1527=CARTESIAN_POINT ( 'NONE',  ( -5.405949406250003975, -9.363379034771801557, -54.34375000204835970 ) ) ;
#1528=ORIENTED_EDGE ( 'NONE', *, *, #29121, .F. ) ;
#1533=CARTESIAN_POINT ( 'NONE',  ( -10.00000000000000000, -5.773502691896251982, -27.00000000409677625 ) ) ;
#1537=( BOUNDED_CURVE ( )  B_SPLINE_CURVE ( 2, ( #23012, #29486, #22163, #26039, #22797, #29273, #36166 ),
 .UNSPECIFIED., .F., .F. ) 
 B_SPLINE_CURVE_WITH_KNOTS ( ( 3, 2, 2, 3 ),
 ( 0.1455223880597014963, 0.1467661691542288538, 0.1480099502487562391, 0.1492537313432835966 ),
 .UNSPECIFIED. ) 
 CURVE ( )  GEOMETRIC_REPRESENTATION_ITEM ( )  RATIONAL_B_SPLINE_CURVE ( ( 1.000000000000000000, 0.8660254037844387076, 1.000000000000000000, 0.8660254037844387076, 1.000000000000000000, 0.8660254037844357100, 1.000000000000003109 ) ) 
 REPRESENTATION_ITEM ( '' )  );
#1543=CARTESIAN_POINT ( 'NONE',  ( 0.000000000000000000, 0.000000000000000000, -99.99999999999998579 ) ) ;
#1547=CARTESIAN_POINT ( 'NONE',  ( -10.81189881249999729, 6.242252689847871849, -186.9062500020484094 ) ) ;
#1553=CARTESIAN_POINT ( 'NONE',  ( -10.81189881249999729, 1.324075727343319199E-15, -116.0937500020483810 ) ) ;
#1555=CARTESIAN_POINT ( 'NONE',  ( -10.81189881249999729, 1.324075727343319199E-15, -128.2812500020483810 ) ) ;
#1557=CARTESIAN_POINT ( 'NONE',  ( -2.293366432827344421E-15, -12.48450537969573659, -130.7187500020483810 ) ) ;
#1558=EDGE_CURVE ( 'NONE', #3006, #10534, #18160, .T. ) ;
#1560=CARTESIAN_POINT ( 'NONE',  ( 9.999999999999742428, 5.773502691896404748, -157.8750000000000000 ) ) ;
#1561=CARTESIAN_POINT ( 'NONE',  ( -2.121150477449813534E-15, -11.54700538379251284, -149.3750000000000000 ) ) ;
#1562=CARTESIAN_POINT ( 'NONE',  ( -5.000000000000003553, -8.660254037844383745, -21.99999999999996447 ) ) ;
#1566=CARTESIAN_POINT ( 'NONE',  ( -9.999999999999998224, 1.224646799147353059E-15, -165.1250000040967905 ) ) ;
#1568=CARTESIAN_POINT ( 'NONE',  ( -10.81189881249999729, 1.324075727343319199E-15, -42.59375000204837391 ) ) ;
#1569=DIRECTION ( 'NONE',  ( -1.000000000000000000, 0.000000000000000000, 0.000000000000000000 ) ) ;
#1570=CARTESIAN_POINT ( 'NONE',  ( -10.81189881249999729, 1.324075727343319199E-15, -152.0937500020483810 ) ) ;
#1574=CARTESIAN_POINT ( 'NONE',  ( -5.000000000000003553, -8.660254037844383745, -78.99999999999998579 ) ) ;
#1576=ORIENTED_EDGE ( 'NONE', *, *, #8183, .T. ) ;
#1577=CARTESIAN_POINT ( 'NONE',  ( 5.405949406249999534, 9.363379034771803333, -100.2812500020483952 ) ) ;
#1578=CARTESIAN_POINT ( 'NONE',  ( -9.999999999999998224, 5.773502691896259087, -120.2500000040967763 ) ) ;
#1582=CARTESIAN_POINT ( 'NONE',  ( 5.405949406249999534, 9.363379034771803333, -43.28125000204838102 ) ) ;
#1591=VERTEX_POINT ( 'NONE', #28126 ) ;
#1601=CARTESIAN_POINT ( 'NONE',  ( 10.81189881249999907, 6.242252689847868297, -143.7187500020483810 ) ) ;
#1602=CARTESIAN_POINT ( 'NONE',  ( 10.81189881249999551, -6.242252689847874514, -148.6562500020484094 ) ) ;
#1603=CARTESIAN_POINT ( 'NONE',  ( 10.81189881249999729, 0.000000000000000000, -157.3437500020483810 ) ) ;
#1605=CARTESIAN_POINT ( 'NONE',  ( 0.000000000000000000, 0.000000000000000000, -99.99999999999998579 ) ) ;
#1606=CARTESIAN_POINT ( 'NONE',  ( -9.999999999999998224, 5.773502691896259087, -172.3750000000000000 ) ) ;
#1612=CARTESIAN_POINT ( 'NONE',  ( 10.81189881249999729, 0.000000000000000000, -176.8437500020483810 ) ) ;
#1616=CARTESIAN_POINT ( 'NONE',  ( 10.81189881249999551, -6.242252689847874514, -45.15625000204836681 ) ) ;
#1618=CARTESIAN_POINT ( 'NONE',  ( -4.999999999999996447, 8.660254037844387298, -95.99999999999998579 ) ) ;
#1619=ORIENTED_EDGE ( 'NONE', *, *, #27249, .F. ) ;
#1620=CARTESIAN_POINT ( 'NONE',  ( -10.81189881249999729, 6.242252689847871849, -126.9062500020483810 ) ) ;
#1621=CARTESIAN_POINT ( 'NONE',  ( -4.999999999999996447, 8.660254037844387298, -145.8750000040967905 ) ) ;
#1624=ORIENTED_EDGE ( 'NONE', *, *, #4298, .F. ) ;
#1625=CARTESIAN_POINT ( 'NONE',  ( 10.81189881249999729, 0.000000000000000000, -170.8437500020484094 ) ) ;
#1629=CARTESIAN_POINT ( 'NONE',  ( 10.81189881249999907, 6.242252689847868297, -68.90625000204839523 ) ) ;
#1631=CARTESIAN_POINT ( 'NONE',  ( 7.070501591499377789E-16, 11.54700538379251284, -47.00000000409676915 ) ) ;
#1632=CARTESIAN_POINT ( 'NONE',  ( 10.81189881249999729, 0.000000000000000000, -1.343750002048366143 ) ) ;
#1643=DIRECTION ( 'NONE',  ( -1.000000000000000000, 0.000000000000000000, 0.000000000000000000 ) ) ;
#1644=VERTEX_POINT ( 'NONE', #2013 ) ;
#1652=CARTESIAN_POINT ( 'NONE',  ( 9.999999999999998224, 0.000000000000000000, -39.49999999999997868 ) ) ;
#1654=CARTESIAN_POINT ( 'NONE',  ( -2.293366432827344421E-15, -12.48450537969573659, -166.7187500020484094 ) ) ;
#1655=CARTESIAN_POINT ( 'NONE',  ( -10.81189881249999729, 1.324075727343319199E-15, -179.0937500020484094 ) ) ;
#1657=CARTESIAN_POINT ( 'NONE',  ( 10.00000000000000000, 5.773502691896255534, -192.3750000000000000 ) ) ;
#1664=( BOUNDED_CURVE ( )  B_SPLINE_CURVE ( 2, ( #16887, #3328, #42587, #528, #312, #3755, #13012 ),
 .UNSPECIFIED., .F., .F. ) 
 B_SPLINE_CURVE_WITH_KNOTS ( ( 3, 2, 2, 3 ),
 ( 0.3358208955223880854, 0.3370646766169154707, 0.3383084577114429670, 0.3395522388059703522 ),
 .UNSPECIFIED. ) 
 CURVE ( )  GEOMETRIC_REPRESENTATION_ITEM ( )  RATIONAL_B_SPLINE_CURVE ( ( 1.000000000000000000, 0.8660254037844387076, 1.000000000000000000, 0.8660254037844387076, 1.000000000000000000, 0.8660254037844148378, 1.000000000000023981 ) ) 
 REPRESENTATION_ITEM ( '' )  );
#1665=CARTESIAN_POINT ( 'NONE',  ( 7.644554776091147741E-16, 12.48450537969573659, -62.46875000204838102 ) ) ;
#1666=ADVANCED_FACE ( 'NONE', ( #3485 ), #9741, .F. ) ;
#1667=CARTESIAN_POINT ( 'NONE',  ( -2.293366432827344421E-15, -12.48450537969573659, -69.40625000204838102 ) ) ;
#1669=CARTESIAN_POINT ( 'NONE',  ( 4.999999999999992006, -8.660254037844389075, -129.7499999999999716 ) ) ;
#1671=CARTESIAN_POINT ( 'NONE',  ( 10.81189881249999551, -6.242252689847874514, -153.1562500020484094 ) ) ;
#1672=CARTESIAN_POINT ( 'NONE',  ( 10.81189881249999551, -6.242252689847874514, -160.6562500020484379 ) ) ;
#1675=CARTESIAN_POINT ( 'NONE',  ( 10.81189881249999907, 6.242252689847868297, -97.21875000204836681 ) ) ;
#1678=CARTESIAN_POINT ( 'NONE',  ( -10.81189881249999729, 1.324075727343319199E-15, -195.5937500020484094 ) ) ;
#1680=CARTESIAN_POINT ( 'NONE',  ( -7.482077728350252421, -6.785286198130088486, -179.9999999999999432 ) ) ;
#1681=CARTESIAN_POINT ( 'NONE',  ( 10.81189881249999551, -6.242252689847874514, -90.15625000204836681 ) ) ;
#1683=CARTESIAN_POINT ( 'NONE',  ( 10.00000000000000000, 5.773502691896255534, -69.75000000409679046 ) ) ;
#1685=CARTESIAN_POINT ( 'NONE',  ( 10.81189881249999551, -6.242252689847874514, -28.46875000204837391 ) ) ;
#1686=ORIENTED_EDGE ( 'NONE', *, *, #38833, .F. ) ;
#1688=CARTESIAN_POINT ( 'NONE',  ( 5.405949406249999534, 9.363379034771803333, -17.78125000204835970 ) ) ;
#1692=CARTESIAN_POINT ( 'NONE',  ( 7.070501591499377789E-16, 11.54700538379251284, -2.000000004096752715 ) ) ;
#1695=EDGE_CURVE ( 'NONE', #38211, #15832, #13172, .T. ) ;
#1699=ORIENTED_EDGE ( 'NONE', *, *, #30651, .T. ) ;
#1708=CARTESIAN_POINT ( 'NONE',  ( 0.000000000000000000, 0.000000000000000000, -99.99999999999998579 ) ) ;
#1709=CARTESIAN_POINT ( 'NONE',  ( -9.999999999999998224, 1.224646799147353059E-15, -109.2499999999999858 ) ) ;
#1712=CARTESIAN_POINT ( 'NONE',  ( -10.81189881249999729, 1.324075727343319199E-15, -167.2812500020484094 ) ) ;
#1715=CARTESIAN_POINT ( 'NONE',  ( 10.81189881249999907, 6.242252689847868297, -89.71875000204836681 ) ) ;
#1717=CARTESIAN_POINT ( 'NONE',  ( -5.405949406250003975, -9.363379034771801557, -192.3437500020484094 ) ) ;
#1718=CARTESIAN_POINT ( 'NONE',  ( -5.405949406249996869, 9.363379034771805109, -95.53125000204838102 ) ) ;
#1721=EDGE_CURVE ( 'NONE', #40615, #41419, #39953, .T. ) ;
#1722=( BOUNDED_CURVE ( )  B_SPLINE_CURVE ( 2, ( #19865, #682, #36283, #39510, #9732, #13586, #39931 ),
 .UNSPECIFIED., .F., .F. ) 
 B_SPLINE_CURVE_WITH_KNOTS ( ( 3, 2, 2, 3 ),
 ( 0.1865671641791045166, 0.1878109452736318741, 0.1890547263681592594, 0.1902985074626866169 ),
 .UNSPECIFIED. ) 
 CURVE ( )  GEOMETRIC_REPRESENTATION_ITEM ( )  RATIONAL_B_SPLINE_CURVE ( ( 0.9999999999999970024, 0.8660254037844417052, 1.000000000000000000, 0.8660254037844387076, 1.000000000000000000, 0.8660254037844327124, 1.000000000000005995 ) ) 
 REPRESENTATION_ITEM ( '' )  );
#1724=CARTESIAN_POINT ( 'NONE',  ( -5.405949406249996869, 9.363379034771805109, -175.0312500020484094 ) ) ;
#1725=CARTESIAN_POINT ( 'NONE',  ( 10.81189881249999551, -6.242252689847874514, -192.1562500020484094 ) ) ;
#1727=EDGE_CURVE ( 'NONE', #30416, #22548, #14877, .T. ) ;
#1728=CARTESIAN_POINT ( 'NONE',  ( 5.000000000000000000, 8.660254037844385522, -162.6250000040967905 ) ) ;
#1730=CARTESIAN_POINT ( 'NONE',  ( -2.293366432827344421E-15, -12.48450537969573659, -13.71875000204836326 ) ) ;
#1732=CARTESIAN_POINT ( 'NONE',  ( -10.81189881249999729, 1.324075727343319199E-15, -122.0937500020483952 ) ) ;
#1734=CARTESIAN_POINT ( 'NONE',  ( 7.644554776091147741E-16, 12.48450537969573659, -19.15625000204837391 ) ) ;
#1737=CARTESIAN_POINT ( 'NONE',  ( 9.999999999999996447, -5.773502691896262640, -50.12499999999997868 ) ) ;
#1738=CARTESIAN_POINT ( 'NONE',  ( 7.644554776091147741E-16, 12.48450537969573659, -118.1562500020483952 ) ) ;
#1741=CARTESIAN_POINT ( 'NONE',  ( 9.999999999999996447, -5.773502691896262640, -92.50000000409677625 ) ) ;
#1744=CARTESIAN_POINT ( 'NONE',  ( -2.293366432827344421E-15, -12.48450537969573659, -46.71875000204835970 ) ) ;
#1745=ORIENTED_EDGE ( 'NONE', *, *, #21741, .F. ) ;
#1750=CARTESIAN_POINT ( 'NONE',  ( 5.000000000000000000, 8.660254037844385522, -30.62500000409676559 ) ) ;
#1751=EDGE_CURVE ( 'NONE', #16776, #39083, #12547, .T. ) ;
#1756=VERTEX_POINT ( 'NONE', #38891 ) ;
#1764=CARTESIAN_POINT ( 'NONE',  ( 10.81189881249999907, 6.242252689847868297, -188.9062500020484379 ) ) ;
#1769=CARTESIAN_POINT ( 'NONE',  ( 5.405949406249999534, 9.363379034771803333, -107.5937500020483810 ) ) ;
#1770=CARTESIAN_POINT ( 'NONE',  ( -5.405949406250003975, -9.363379034771801557, -117.5312500020483952 ) ) ;
#1772=CARTESIAN_POINT ( 'NONE',  ( 10.81189881249999551, -6.242252689847874514, -130.4687500020483810 ) ) ;
#1775=CARTESIAN_POINT ( 'NONE',  ( 4.999999999999992006, -8.660254037844389075, -146.2500000000000000 ) ) ;
#1776=CARTESIAN_POINT ( 'NONE',  ( 9.999999999999998224, 0.000000000000000000, -13.99999999999995737 ) ) ;
#1779=CARTESIAN_POINT ( 'NONE',  ( 5.000000000000000000, 8.660254037844385522, -191.1250000040967905 ) ) ;
#1781=CARTESIAN_POINT ( 'NONE',  ( 10.81189881249999551, -6.242252689847874514, -35.96875000204835260 ) ) ;
#1782=DIRECTION ( 'NONE',  ( -1.000000000000000000, 0.000000000000000000, 0.000000000000000000 ) ) ;
#1783=CARTESIAN_POINT ( 'NONE',  ( 5.405949406249992428, -9.363379034771808662, -144.0937500020483810 ) ) ;
#1785=CARTESIAN_POINT ( 'NONE',  ( 4.999999999999992006, -8.660254037844389075, -101.6250000040967905 ) ) ;
#1787=CARTESIAN_POINT ( 'NONE',  ( -2.121150477449813534E-15, -11.54700538379251284, -77.37499999999997158 ) ) ;
#1789=VERTEX_POINT ( 'NONE', #19450 ) ;
#1790=CARTESIAN_POINT ( 'NONE',  ( -6.652853726956785785, 8.522716305231336165, -100.0000000000000142 ) ) ;
#1791=CARTESIAN_POINT ( 'NONE',  ( 7.070501591499377789E-16, 11.54700538379251284, -126.5000000040967905 ) ) ;
#1793=CARTESIAN_POINT ( 'NONE',  ( -10.81189881249999729, 1.324075727343319199E-15, -78.59375000204838102 ) ) ;
#1797=( BOUNDED_CURVE ( )  B_SPLINE_CURVE ( 2, ( #37492, #33630, #3642, #16769, #11574, #41355, #27788 ),
 .UNSPECIFIED., .F., .F. ) 
 B_SPLINE_CURVE_WITH_KNOTS ( ( 3, 2, 2, 3 ),
 ( 0.3246268656716419510, 0.3258706467661692807, 0.3271144278606965550, 0.3283582089552238847 ),
 .UNSPECIFIED. ) 
 CURVE ( )  GEOMETRIC_REPRESENTATION_ITEM ( )  RATIONAL_B_SPLINE_CURVE ( ( 0.9999999999999820144, 0.8660254037844566932, 1.000000000000000000, 0.8660254037844387076, 1.000000000000000000, 0.8660254037844387076, 1.000000000000000000 ) ) 
 REPRESENTATION_ITEM ( '' )  );
#1799=CARTESIAN_POINT ( 'NONE',  ( -10.81189881249999729, 6.242252689847871849, -42.90625000204836681 ) ) ;
#1800=CARTESIAN_POINT ( 'NONE',  ( 9.999999999999994671, -5.773502691896262640, -137.1250000000000000 ) ) ;
#1803=CARTESIAN_POINT ( 'NONE',  ( 10.00000000000000000, 5.773502691896255534, -165.7500000040967905 ) ) ;
#1804=FACE_OUTER_BOUND ( 'NONE', #27162, .T. ) ;
#1807=ORIENTED_EDGE ( 'NONE', *, *, #32387, .F. ) ;
#1809=AXIS2_PLACEMENT_3D ( 'NONE', #26701, #34039, #16752 ) ;
#1818=CARTESIAN_POINT ( 'NONE',  ( 10.81189881249999729, 0.000000000000000000, -131.8437500020484094 ) ) ;
#1819=CARTESIAN_POINT ( 'NONE',  ( 7.644554776091147741E-16, 12.48450537969573659, -137.6562500020483810 ) ) ;
#1820=CARTESIAN_POINT ( 'NONE',  ( -10.81189881249999729, 6.242252689847871849, -152.2187500020483810 ) ) ;
#1823=CARTESIAN_POINT ( 'NONE',  ( -5.000000000000003553, -8.660254037844383745, -173.5000000000000284 ) ) ;
#1826=CARTESIAN_POINT ( 'NONE',  ( -7.870332919771452218, 7.330147429241407053, -99.99999999999998579 ) ) ;
#1827=CARTESIAN_POINT ( 'NONE',  ( -5.405949406249996869, 9.363379034771805109, -168.8437500020484094 ) ) ;
#1831=CARTESIAN_POINT ( 'NONE',  ( 5.405949406249999534, 9.363379034771803333, -46.28125000204838813 ) ) ;
#1833=CARTESIAN_POINT ( 'NONE',  ( 4.999999999999992006, -8.660254037844389075, -101.2499999999999858 ) ) ;
#1837=CARTESIAN_POINT ( 'NONE',  ( 5.405949406249999534, 9.363379034771803333, -125.7812500020483668 ) ) ;
#1838=CARTESIAN_POINT ( 'NONE',  ( 10.00000000000000000, 5.773502691896255534, -149.2500000040968189 ) ) ;
#1839=CARTESIAN_POINT ( 'NONE',  ( -2.121150477449813534E-15, -11.54700538379251284, -167.3750000000000000 ) ) ;
#1842=CARTESIAN_POINT ( 'NONE',  ( 5.405949406249992428, -9.363379034771808662, -175.5937500020484094 ) ) ;
#1844=CARTESIAN_POINT ( 'NONE',  ( -10.00000000000000000, -5.773502691896252870, -166.1249999999999716 ) ) ;
#1846=CARTESIAN_POINT ( 'NONE',  ( -10.81189881249999729, 1.324075727343319199E-15, -69.78125000204838102 ) ) ;
#1848=CARTESIAN_POINT ( 'NONE',  ( 9.999999999999998224, 0.000000000000000000, -44.37500000409677625 ) ) ;
#1849=CARTESIAN_POINT ( 'NONE',  ( 10.81189881249999907, 6.242252689847868297, -5.718750002048356151 ) ) ;
#1850=CARTESIAN_POINT ( 'NONE',  ( -10.00000000000051337, 5.773502691895962435, -147.2500000040967905 ) ) ;
#1860=ORIENTED_EDGE ( 'NONE', *, *, #9956, .F. ) ;
#1862=CARTESIAN_POINT ( 'NONE',  ( 0.000000000000000000, 0.000000000000000000, -99.99999999999998579 ) ) ;
#1864=ORIENTED_EDGE ( 'NONE', *, *, #33908, .F. ) ;
#1866=DIRECTION ( 'NONE',  ( -1.000000000000000000, 0.000000000000000000, 0.000000000000000000 ) ) ;
#1870=CARTESIAN_POINT ( 'NONE',  ( 5.000000000000000000, 8.660254037844385522, -112.7499999999999858 ) ) ;
#1871=CARTESIAN_POINT ( 'NONE',  ( -10.00000000000000000, -5.773502691896251982, -37.12499999999995737 ) ) ;
#1874=CARTESIAN_POINT ( 'NONE',  ( -10.81189881249999729, 1.324075727343319199E-15, -167.0937500020484094 ) ) ;
#1875=DIRECTION ( 'NONE',  ( -0.000000000000000000, -0.000000000000000000, -1.000000000000000000 ) ) ;
#1877=CARTESIAN_POINT ( 'NONE',  ( -9.999999999999998224, 1.224646799147353059E-15, -197.7500000000000000 ) ) ;
#1882=CARTESIAN_POINT ( 'NONE',  ( -2.293366432827344421E-15, -12.48450537969573659, -66.40625000204838102 ) ) ;
#1884=CARTESIAN_POINT ( 'NONE',  ( 7.070501591499377789E-16, 11.54700538379251284, -120.1249999999999858 ) ) ;
#1885=CARTESIAN_POINT ( 'NONE',  ( -2.293366432827344421E-15, -12.48450537969573659, -147.4062500020483810 ) ) ;
#1886=CARTESIAN_POINT ( 'NONE',  ( 5.405949406249999534, 9.363379034771803333, -164.7812500020484094 ) ) ;
#1888=CARTESIAN_POINT ( 'NONE',  ( 9.999999999999872102, 5.773502691896329253, -159.7500000040967905 ) ) ;
#1889=CARTESIAN_POINT ( 'NONE',  ( 7.644554776091147741E-16, 12.48450537969573659, -95.46875000204839523 ) ) ;
#1890=ORIENTED_EDGE ( 'NONE', *, *, #2901, .T. ) ;
#1892=CARTESIAN_POINT ( 'NONE',  ( -10.81189881249999907, -6.242252689847864744, -196.9687500020484379 ) ) ;
#1894=DIRECTION ( 'NONE',  ( -0.000000000000000000, -0.000000000000000000, -1.000000000000000000 ) ) ;
#1895=CARTESIAN_POINT ( 'NONE',  ( -10.81189881249999729, 1.324075727343319199E-15, -89.28125000204838102 ) ) ;
#1897=CARTESIAN_POINT ( 'NONE',  ( -4.999999999999996447, 8.660254037844387298, -64.87500000409676204 ) ) ;
#1898=CYLINDRICAL_SURFACE ( 'NONE', #24332, 9.999999999999998224 ) ;
#1899=CARTESIAN_POINT ( 'NONE',  ( -2.293366432827344421E-15, -12.48450537969573659, -24.21875000204837036 ) ) ;
#1902=CARTESIAN_POINT ( 'NONE',  ( -10.81189881249999729, 6.242252689847871849, -23.40625000204837747 ) ) ;
#1913=LINE ( 'NONE', #7523, #37956 ) ;
#1914=EDGE_CURVE ( 'NONE', #40028, #30244, #7708, .T. ) ;
#1915=ORIENTED_EDGE ( 'NONE', *, *, #23824, .T. ) ;
#1917=VERTEX_POINT ( 'NONE', #17050 ) ;
#1926=CARTESIAN_POINT ( 'NONE',  ( 7.644554776091147741E-16, 12.48450537969573659, -163.1562500020484094 ) ) ;
#1927=CARTESIAN_POINT ( 'NONE',  ( 9.999999999999998224, 0.000000000000000000, -171.8750000040968189 ) ) ;
#1929=CARTESIAN_POINT ( 'NONE',  ( -10.81189881249999907, -6.242252689847864744, -84.46875000204836681 ) ) ;
#1930=CARTESIAN_POINT ( 'NONE',  ( 9.999999999999998224, 0.000000000000000000, -101.3750000040967905 ) ) ;
#1931=CARTESIAN_POINT ( 'NONE',  ( 7.644554776091147741E-16, 12.48450537969573659, -197.4687500020484094 ) ) ;
#1932=CARTESIAN_POINT ( 'NONE',  ( -10.81189881249999729, 1.324075727343319199E-15, -92.28125000204838102 ) ) ;
#1936=CARTESIAN_POINT ( 'NONE',  ( 5.405949406249992428, -9.363379034771808662, -175.7812500020484094 ) ) ;
#1937=CARTESIAN_POINT ( 'NONE',  ( 5.405949406249992428, -9.363379034771808662, -189.2812500020484094 ) ) ;
#1939=CARTESIAN_POINT ( 'NONE',  ( 4.999999999999992006, -8.660254037844389075, -166.1250000040967905 ) ) ;
#1941=CARTESIAN_POINT ( 'NONE',  ( 10.81189881249999907, 6.242252689847868297, -16.21875000204836326 ) ) ;
#1943=CARTESIAN_POINT ( 'NONE',  ( 10.81189881249999551, -6.242252689847874514, -119.9687500020483952 ) ) ;
#1945=CARTESIAN_POINT ( 'NONE',  ( -10.81189881249999729, 6.242252689847871849, -20.40625000204837391 ) ) ;
#1948=CARTESIAN_POINT ( 'NONE',  ( 9.999999999999998224, 0.000000000000000000, -51.49999999999996447 ) ) ;
#1949=CARTESIAN_POINT ( 'NONE',  ( 10.81189881249999729, 0.000000000000000000, -118.5312500020483952 ) ) ;
#1952=CARTESIAN_POINT ( 'NONE',  ( 10.00000000000000000, 5.773502691896255534, -89.25000000409677625 ) ) ;
#1955=CARTESIAN_POINT ( 'NONE',  ( -10.81189881249999907, -6.242252689847864744, -51.46875000204837391 ) ) ;
#1960=VECTOR ( 'NONE', #12558, 1000.000000000000000 ) ;
#1961=CARTESIAN_POINT ( 'NONE',  ( -9.999999999999998224, 1.224646799147353059E-15, -22.62500000409675849 ) ) ;
#1965=EDGE_CURVE ( 'NONE', #41954, #2320, #10794, .T. ) ;
#1966=CARTESIAN_POINT ( 'NONE',  ( -9.999999999999998224, 0.000000000000000000, -99.99999999999998579 ) ) ;
#1973=EDGE_LOOP ( 'NONE', ( #218, #36575, #20996, #11706 ) ) ;
#1979=( BOUNDED_CURVE ( )  B_SPLINE_CURVE ( 2, ( #2008, #18167, #34595, #1359, #27898, #37606, #31361 ),
 .UNSPECIFIED., .F., .F. ) 
 B_SPLINE_CURVE_WITH_KNOTS ( ( 3, 2, 2, 3 ),
 ( 0.2723880597014926574, 0.2736318407960199872, 0.2748756218905473725, 0.2761194029850747578 ),
 .UNSPECIFIED. ) 
 CURVE ( )  GEOMETRIC_REPRESENTATION_ITEM ( )  RATIONAL_B_SPLINE_CURVE ( ( 0.9999999999999880096, 0.8660254037844506980, 1.000000000000000000, 0.8660254037844387076, 1.000000000000000000, 0.8660254037844267172, 1.000000000000011990 ) ) 
 REPRESENTATION_ITEM ( '' )  );
#1980=CARTESIAN_POINT ( 'NONE',  ( -10.81189881249999907, -6.242252689847864744, -186.6562500020484094 ) ) ;
#1984=CARTESIAN_POINT ( 'NONE',  ( 7.644554776091147741E-16, 12.48450537969573659, -111.9687500020483952 ) ) ;
#1986=CARTESIAN_POINT ( 'NONE',  ( -5.405949406250003975, -9.363379034771801557, -120.5312500020483952 ) ) ;
#1988=CARTESIAN_POINT ( 'NONE',  ( -10.81189881249999729, 6.242252689847871849, -122.2187500020483810 ) ) ;
#1991=CARTESIAN_POINT ( 'NONE',  ( 9.999999999999998224, 0.000000000000000000, -149.0000000000000000 ) ) ;
#1992=CARTESIAN_POINT ( 'NONE',  ( 10.00000000000000000, 5.773502691896255534, -9.374999999999966249 ) ) ;
#1996=CARTESIAN_POINT ( 'NONE',  ( 4.999999999999992006, -8.660254037844389075, -190.1250000040967905 ) ) ;
#1998=CARTESIAN_POINT ( 'NONE',  ( -10.81189881249999729, 1.324075727343319199E-15, -39.59375000204837391 ) ) ;
#1999=CARTESIAN_POINT ( 'NONE',  ( 5.405949406249999534, 9.363379034771803333, -146.5937500020483810 ) ) ;
#2001=FACE_OUTER_BOUND ( 'NONE', #8783, .T. ) ;
#2002=CARTESIAN_POINT ( 'NONE',  ( -2.121150477449813534E-15, -11.54700538379251284, -74.37499999999995737 ) ) ;
#2003=CARTESIAN_POINT ( 'NONE',  ( -10.81189881249999729, 6.242252689847871849, -138.9062500020484094 ) ) ;
#2006=CARTESIAN_POINT ( 'NONE',  ( -5.405949406249996869, 9.363379034771805109, -103.0312500020483952 ) ) ;
#2007=CARTESIAN_POINT ( 'NONE',  ( 4.999999999999992006, -8.660254037844389075, -113.6250000040967763 ) ) ;
#2008=CARTESIAN_POINT ( 'NONE',  ( -9.999999999999998224, 1.224646799147353059E-15, -144.1250000040967905 ) ) ;
#2009=CARTESIAN_POINT ( 'NONE',  ( -2.293366432827344421E-15, -12.48450537969573659, -70.71875000204838102 ) ) ;
#2012=CARTESIAN_POINT ( 'NONE',  ( 10.81189881249999551, -6.242252689847874514, -46.65625000204836681 ) ) ;
#2013=CARTESIAN_POINT ( 'NONE',  ( 9.999999999999998224, 0.000000000000000000, -149.0000000000000000 ) ) ;
#2017=AXIS2_PLACEMENT_3D ( 'NONE', #6538, #22950, #36317 ) ;
#2023=CARTESIAN_POINT ( 'NONE',  ( -5.000000000000003553, -8.660254037844383745, -176.8750000040967905 ) ) ;
#2031=CARTESIAN_POINT ( 'NONE',  ( -5.405949406249996869, 9.363379034771805109, -137.3437500020484094 ) ) ;
#2032=CARTESIAN_POINT ( 'NONE',  ( 7.644554776091147741E-16, 12.48450537969573659, -142.1562500020483810 ) ) ;
#2033=CARTESIAN_POINT ( 'NONE',  ( -10.81189881249999729, -6.242252689847864744, -144.4687500020484094 ) ) ;
#2036=CARTESIAN_POINT ( 'NONE',  ( 9.999999999999998224, 0.000000000000000000, -174.5000000000000284 ) ) ;
#2041=CARTESIAN_POINT ( 'NONE',  ( 10.81189881249999551, -6.242252689847874514, -166.4687500020484094 ) ) ;
#2044=( BOUNDED_CURVE ( )  B_SPLINE_CURVE ( 2, ( #32659, #3088, #16428, #16216, #29627, #70, #13194 ),
 .UNSPECIFIED., .F., .F. ) 
 B_SPLINE_CURVE_WITH_KNOTS ( ( 3, 2, 2, 3 ),
 ( 0.4813432835820896649, 0.4825870646766170502, 0.4838308457711443800, 0.4850746268656717652 ),
 .UNSPECIFIED. ) 
 CURVE ( )  GEOMETRIC_REPRESENTATION_ITEM ( )  RATIONAL_B_SPLINE_CURVE ( ( 0.9999999999999880096, 0.8660254037844506980, 1.000000000000000000, 0.8660254037844387076, 1.000000000000000000, 0.8660254037844267172, 1.000000000000011990 ) ) 
 REPRESENTATION_ITEM ( '' )  );
#2046=CARTESIAN_POINT ( 'NONE',  ( -10.81189881249999729, 1.324075727343319199E-15, -45.78125000204838813 ) ) ;
#2048=CARTESIAN_POINT ( 'NONE',  ( 10.00000000000000000, 5.773502691896255534, -97.87499999999998579 ) ) ;
#2050=CARTESIAN_POINT ( 'NONE',  ( -5.405949406249996869, 9.363379034771805109, -124.0312500020483952 ) ) ;
#2051=CARTESIAN_POINT ( 'NONE',  ( -2.121150477449813534E-15, -11.54700538379251284, -136.2500000040967620 ) ) ;
#2056=CARTESIAN_POINT ( 'NONE',  ( 10.81189881249999551, -6.242252689847874514, -175.4687500020484094 ) ) ;
#2059=DIRECTION ( 'NONE',  ( 1.000000000000000000, 0.000000000000000000, 0.000000000000000000 ) ) ;
#2060=CARTESIAN_POINT ( 'NONE',  ( -10.81189881249999729, 6.242252689847871849, -66.90625000204839523 ) ) ;
#2061=CARTESIAN_POINT ( 'NONE',  ( -2.121150477449813534E-15, -11.54700538379251284, -43.25000000409676204 ) ) ;
#2063=CARTESIAN_POINT ( 'NONE',  ( -5.405949406250003975, -9.363379034771801557, -3.343750002048367698 ) ) ;
#2084=CARTESIAN_POINT ( 'NONE',  ( -2.121150477449813534E-15, -11.54700538379251284, -35.37499999999996447 ) ) ;
#2087=CARTESIAN_POINT ( 'NONE',  ( 10.81189881249999907, 6.242252689847868297, -157.2187500020483810 ) ) ;
#2089=CARTESIAN_POINT ( 'NONE',  ( -10.81189881249999729, 1.324075727343319199E-15, -174.5937500020484094 ) ) ;
#2092=CARTESIAN_POINT ( 'NONE',  ( 9.999999999999996447, -5.773502691896262640, -194.1250000000000284 ) ) ;
#2094=DIRECTION ( 'NONE',  ( -0.000000000000000000, -0.000000000000000000, -1.000000000000000000 ) ) ;
#2097=CARTESIAN_POINT ( 'NONE',  ( 10.81189881249999551, -6.242252689847874514, -67.65625000204838102 ) ) ;
#2099=CARTESIAN_POINT ( 'NONE',  ( -2.121150477449813534E-15, -11.54700538379251284, -125.3749999999999858 ) ) ;
#2100=EDGE_CURVE ( 'NONE', #5246, #9953, #41342, .T. ) ;
#2102=CARTESIAN_POINT ( 'NONE',  ( 7.644554776091147741E-16, 12.48450537969573659, -152.6562500020484094 ) ) ;
#2103=CARTESIAN_POINT ( 'NONE',  ( -5.405949406250003975, -9.363379034771801557, -161.0312500020484094 ) ) ;
#2106=CARTESIAN_POINT ( 'NONE',  ( -5.405949406249996869, 9.363379034771805109, -96.84375000204838102 ) ) ;
#2107=EDGE_LOOP ( 'NONE', ( #19879, #6050, #26566, #8377 ) ) ;
#2109=CARTESIAN_POINT ( 'NONE',  ( -2.293366432827344421E-15, -12.48450537969573659, -193.7187500020484094 ) ) ;
#2111=CARTESIAN_POINT ( 'NONE',  ( -4.534034563800342532, -9.223041764796271025, -180.0000000000000000 ) ) ;
#2113=CARTESIAN_POINT ( 'NONE',  ( -5.405949406250003975, -9.363379034771801557, -92.03125000204838102 ) ) ;
#2115=CARTESIAN_POINT ( 'NONE',  ( -5.000000000000003553, -8.660254037844383745, -64.37500000409676204 ) ) ;
#2117=CARTESIAN_POINT ( 'NONE',  ( 10.81189881249999729, 0.000000000000000000, -26.84375000204835970 ) ) ;
#2120=CARTESIAN_POINT ( 'NONE',  ( -10.81189881249999729, 6.242252689847871849, -17.40625000204837391 ) ) ;
#2122=CARTESIAN_POINT ( 'NONE',  ( 5.000000000000000000, 8.660254037844385522, -160.7500000000000000 ) ) ;
#2130=CARTESIAN_POINT ( 'NONE',  ( 9.999999999999998224, 0.000000000000000000, -179.3750000040967905 ) ) ;
#2136=CARTESIAN_POINT ( 'NONE',  ( -9.999999999999998224, 1.224646799147353059E-15, -173.7500000000000284 ) ) ;
#2138=CARTESIAN_POINT ( 'NONE',  ( -10.00000000000051337, 5.773502691895962435, -124.3749999999999858 ) ) ;
#2139=CARTESIAN_POINT ( 'NONE',  ( -2.293366432827344421E-15, -12.48450537969573659, -166.9062500020483810 ) ) ;
#2144=CARTESIAN_POINT ( 'NONE',  ( -10.81189881249999729, 6.242252689847871849, -84.71875000204836681 ) ) ;
#2145=CARTESIAN_POINT ( 'NONE',  ( -10.81189881249999729, 1.324075727343319199E-15, -195.5937500020484094 ) ) ;
#2146=CARTESIAN_POINT ( 'NONE',  ( 10.81189881249999907, 6.242252689847868297, -89.90625000204839523 ) ) ;
#2150=CARTESIAN_POINT ( 'NONE',  ( 7.644554776091147741E-16, 12.48450537969573659, -176.6562500020484094 ) ) ;
#2151=CARTESIAN_POINT ( 'NONE',  ( 10.81189881249999907, 6.242252689847868297, -191.9062500020484094 ) ) ;
#2153=CARTESIAN_POINT ( 'NONE',  ( 9.999999999999996447, -5.773502691896262640, -166.0000000040967905 ) ) ;
#2155=CARTESIAN_POINT ( 'NONE',  ( -5.405949406250003975, -9.363379034771801557, -12.34375000204834905 ) ) ;
#2157=CARTESIAN_POINT ( 'NONE',  ( -10.81189881249999729, 6.242252689847871849, -125.2187500020483810 ) ) ;
#2160=CARTESIAN_POINT ( 'NONE',  ( 10.81189881249999729, 0.000000000000000000, -21.03125000204836326 ) ) ;
#2162=CARTESIAN_POINT ( 'NONE',  ( 4.999999999999992006, -8.660254037844389075, -136.1250000040967620 ) ) ;
#2163=CARTESIAN_POINT ( 'NONE',  ( -2.121150477449813534E-15, -11.54700538379251284, -50.37499999999997158 ) ) ;
#2164=CARTESIAN_POINT ( 'NONE',  ( 10.81189881249999907, 6.242252689847868297, -119.9062500020483810 ) ) ;
#2167=CARTESIAN_POINT ( 'NONE',  ( -9.999999999999998224, 1.224646799147353059E-15, -91.62500000409677625 ) ) ;
#2170=CARTESIAN_POINT ( 'NONE',  ( -10.81189881249999907, -6.242252689847864744, -48.46875000204837391 ) ) ;
#2175=CARTESIAN_POINT ( 'NONE',  ( -5.000000000000003553, -8.660254037844383745, -17.87500000409675138 ) ) ;
#2192=CARTESIAN_POINT ( 'NONE',  ( -10.81189881249999729, 6.242252689847871849, -191.4062500020484094 ) ) ;
#2195=CARTESIAN_POINT ( 'NONE',  ( 5.405949406249999534, 9.363379034771803333, -110.5937500020483810 ) ) ;
#2197=CARTESIAN_POINT ( 'NONE',  ( 10.81189881249999907, 6.242252689847868297, -115.4062500020484094 ) ) ;
#2199=CARTESIAN_POINT ( 'NONE',  ( 10.81189881249999729, 6.242252689847867408, -122.7187500020483952 ) ) ;
#2202=CARTESIAN_POINT ( 'NONE',  ( -10.00000000000025580, 5.773502691896109873, -157.3750000000000000 ) ) ;
#2203=CARTESIAN_POINT ( 'NONE',  ( -10.00000000000000000, -5.773502691896251982, -149.6250000000000284 ) ) ;
#2204=CARTESIAN_POINT ( 'NONE',  ( 9.999999999999996447, -5.773502691896262640, -15.62499999999997158 ) ) ;
#2208=CARTESIAN_POINT ( 'NONE',  ( 10.00000000000000000, 5.773502691896255534, -189.7500000040968189 ) ) ;
#2210=CARTESIAN_POINT ( 'NONE',  ( -10.81189881249999729, 6.242252689847871849, -38.21875000204835970 ) ) ;
#2212=CARTESIAN_POINT ( 'NONE',  ( 5.405949406249992428, -9.363379034771808662, -142.5937500020483810 ) ) ;
#2213=ADVANCED_FACE ( 'NONE', ( #14820 ), #895, .F. ) ;
#2217=CARTESIAN_POINT ( 'NONE',  ( -2.121150477449813534E-15, -11.54700538379251284, -78.87500000000000000 ) ) ;
#2218=CARTESIAN_POINT ( 'NONE',  ( 5.405949406249999534, 9.363379034771803333, -137.7812500020483810 ) ) ;
#2220=( BOUNDED_CURVE ( )  B_SPLINE_CURVE ( 2, ( #18721, #19353, #32333, #29086, #28880, #5567, #2130 ),
 .UNSPECIFIED., .F., .F. ) 
 B_SPLINE_CURVE_WITH_KNOTS ( ( 3, 2, 2, 3 ),
 ( 0.09390547265583264192, 0.09452736318407961580, 0.09577114427860701495, 0.09701492537313441411 ),
 .UNSPECIFIED. ) 
 CURVE ( )  GEOMETRIC_REPRESENTATION_ITEM ( )  RATIONAL_B_SPLINE_CURVE ( ( 0.9330127018922194093, 0.9330127039406161948, 1.000000000000000000, 0.8660254037844387076, 1.000000000000000000, 0.8660254037844297148, 1.000000000000008882 ) ) 
 REPRESENTATION_ITEM ( '' )  );
#2224=CARTESIAN_POINT ( 'NONE',  ( -2.121150477449813534E-15, -11.54700538379251284, -119.7500000040967905 ) ) ;
#2226=CARTESIAN_POINT ( 'NONE',  ( 10.81189881249999551, -6.242252689847874514, -71.96875000204836681 ) ) ;
#2229=CARTESIAN_POINT ( 'NONE',  ( -4.999999999999996447, 8.660254037844387298, -130.5000000000000000 ) ) ;
#2231=CARTESIAN_POINT ( 'NONE',  ( 5.405949406249992428, -9.363379034771808662, -40.78125000204838102 ) ) ;
#2236=CARTESIAN_POINT ( 'NONE',  ( -10.00000000000025580, 5.773502691896109873, -152.8750000000000000 ) ) ;
#2241=( BOUNDED_CURVE ( )  B_SPLINE_CURVE ( 2, ( #25776, #29433, #19275, #12163, #38929, #35497, #12371 ),
 .UNSPECIFIED., .F., .F. ) 
 B_SPLINE_CURVE_WITH_KNOTS ( ( 3, 2, 2, 3 ),
 ( 0.2014925373134328901, 0.2027363184079602476, 0.2039800995024875774, 0.2052238805970149627 ),
 .UNSPECIFIED. ) 
 CURVE ( )  GEOMETRIC_REPRESENTATION_ITEM ( )  RATIONAL_B_SPLINE_CURVE ( ( 0.9999999999999940048, 0.8660254037844447028, 1.000000000000000000, 0.8660254037844387076, 1.000000000000000000, 0.8660254037844357100, 1.000000000000002887 ) ) 
 REPRESENTATION_ITEM ( '' )  );
#2244=ORIENTED_EDGE ( 'NONE', *, *, #20142, .F. ) ;
#2246=CARTESIAN_POINT ( 'NONE',  ( 5.000000000000000000, 8.660254037844385522, -135.6250000040967620 ) ) ;
#2255=CARTESIAN_POINT ( 'NONE',  ( 7.644554776091147741E-16, 12.48450537969573659, -131.4687500020483810 ) ) ;
#2256=CARTESIAN_POINT ( 'NONE',  ( -2.293366432827344421E-15, -12.48450537969573659, -142.9062500020483810 ) ) ;
#2257=CARTESIAN_POINT ( 'NONE',  ( 10.81189881249999551, -6.242252689847874514, -142.4687500020483810 ) ) ;
#2260=CARTESIAN_POINT ( 'NONE',  ( -9.999999999999998224, 5.773502691896259087, -170.8750000000000000 ) ) ;
#2265=CARTESIAN_POINT ( 'NONE',  ( 5.405949406249992428, -9.363379034771808662, -168.0937500020484094 ) ) ;
#2269=CARTESIAN_POINT ( 'NONE',  ( -10.81189881249999729, 1.324075727343319199E-15, -33.78125000204837391 ) ) ;
#2271=CARTESIAN_POINT ( 'NONE',  ( 9.999999999999996447, -5.773502691896262640, -101.1250000000000000 ) ) ;
#2274=CARTESIAN_POINT ( 'NONE',  ( 10.81189881249999729, 0.000000000000000000, -118.5312500020483952 ) ) ;
#2275=CARTESIAN_POINT ( 'NONE',  ( 10.00000000000000000, 5.773502691896255534, -143.2500000040967905 ) ) ;
#2281=CARTESIAN_POINT ( 'NONE',  ( 5.405949406249999534, 9.363379034771803333, -67.28125000204838102 ) ) ;
#2286=EDGE_LOOP ( 'NONE', ( #18485, #33810 ) ) ;
#2288=CARTESIAN_POINT ( 'NONE',  ( 7.070501591499376803E-16, 11.54700538379251284, -173.0000000040967905 ) ) ;
#2300=CARTESIAN_POINT ( 'NONE',  ( 9.999999999999996447, -5.773502691896262640, -39.62499999999995737 ) ) ;
#2304=CARTESIAN_POINT ( 'NONE',  ( -10.81189881249999729, 1.324075727343319199E-15, -161.0937500020484094 ) ) ;
#2305=CARTESIAN_POINT ( 'NONE',  ( -2.293366432827344421E-15, -12.48450537969573659, -166.7187500020483810 ) ) ;
#2308=CARTESIAN_POINT ( 'NONE',  ( 10.00000000000000000, 5.773502691896255534, -193.8750000000000284 ) ) ;
#2312=CARTESIAN_POINT ( 'NONE',  ( 10.81189881249999551, -6.242252689847874514, -70.65625000204839523 ) ) ;
#2314=CARTESIAN_POINT ( 'NONE',  ( 9.999999999999996447, -5.773502691896262640, -122.1250000000000000 ) ) ;
#2315=ORIENTED_EDGE ( 'NONE', *, *, #39416, .F. ) ;
#2316=CARTESIAN_POINT ( 'NONE',  ( 10.81189881249999729, 6.242252689847867408, -148.4062500020484094 ) ) ;
#2317=CARTESIAN_POINT ( 'NONE',  ( -5.405949406250003975, -9.363379034771801557, -165.5312500020484094 ) ) ;
#2318=CARTESIAN_POINT ( 'NONE',  ( 4.999999999999992006, -8.660254037844389075, -179.2500000000000284 ) ) ;
#2319=CARTESIAN_POINT ( 'NONE',  ( 10.81189881249999729, 0.000000000000000000, -94.34375000204838102 ) ) ;
#2320=VERTEX_POINT ( 'NONE', #19347 ) ;
#2322=CARTESIAN_POINT ( 'NONE',  ( -10.81189881249999729, 6.242252689847871849, -198.7187500020484379 ) ) ;
#2324=CARTESIAN_POINT ( 'NONE',  ( -7.747353181636939645, -6.452982553152641465, -179.9999999999999432 ) ) ;
#2326=CARTESIAN_POINT ( 'NONE',  ( 5.405949406249999534, 9.363379034771803333, -92.78125000204838102 ) ) ;
#2328=CARTESIAN_POINT ( 'NONE',  ( -2.121150477449813534E-15, -11.54700538379251284, -64.25000000409677625 ) ) ;
#2330=CARTESIAN_POINT ( 'NONE',  ( -10.81189881249999729, 6.242252689847871849, -27.71875000204837391 ) ) ;
#2331=CARTESIAN_POINT ( 'NONE',  ( 9.999999999999998224, 0.000000000000000000, -100.9999999999999858 ) ) ;
#2334=CARTESIAN_POINT ( 'NONE',  ( 7.644554776091147741E-16, 12.48450537969573659, -23.65625000204838102 ) ) ;
#2340=ORIENTED_EDGE ( 'NONE', *, *, #1727, .T. ) ;
#2341=CARTESIAN_POINT ( 'NONE',  ( -9.999999999999996447, 5.773502691896259975, -169.7500000040967905 ) ) ;
#2349=CARTESIAN_POINT ( 'NONE',  ( -9.999999999999998224, 0.000000000000000000, -99.99999999999998579 ) ) ;
#2350=CARTESIAN_POINT ( 'NONE',  ( 9.462123412026320679, -3.482913390811684717, -100.0000000000000426 ) ) ;
#2351=CARTESIAN_POINT ( 'NONE',  ( 7.070501591499376803E-16, 11.54700538379251284, -124.6249999999999858 ) ) ;
#2352=CARTESIAN_POINT ( 'NONE',  ( -10.81189881249999907, -6.242252689847864744, -161.1562500020484094 ) ) ;
#2357=CARTESIAN_POINT ( 'NONE',  ( 10.81189881249999729, 0.000000000000000000, -88.34375000204838102 ) ) ;
#2358=CARTESIAN_POINT ( 'NONE',  ( 7.644554776091147741E-16, 12.48450537969573659, -92.65625000204839523 ) ) ;
#2362=CARTESIAN_POINT ( 'NONE',  ( 5.405949406249999534, 9.363379034771803333, -172.2812500020484094 ) ) ;
#2363=CARTESIAN_POINT ( 'NONE',  ( 5.405949406249992428, -9.363379034771808662, -192.2812500020484094 ) ) ;
#2365=CARTESIAN_POINT ( 'NONE',  ( -9.999999999999998224, 5.773502691896259087, -163.7500000040967905 ) ) ;
#2367=CARTESIAN_POINT ( 'NONE',  ( 10.81189881249999907, 6.242252689847868297, -17.71875000204836681 ) ) ;
#2369=CARTESIAN_POINT ( 'NONE',  ( 5.405949406249992428, -9.363379034771808662, -121.5937500020483952 ) ) ;
#2371=CARTESIAN_POINT ( 'NONE',  ( -10.81189881249999907, -6.242252689847864744, -23.15625000204837747 ) ) ;
#2374=CARTESIAN_POINT ( 'NONE',  ( 5.405949406249992428, -9.363379034771808662, -115.7812500020483952 ) ) ;
#2378=CARTESIAN_POINT ( 'NONE',  ( -4.999999999999996447, 8.660254037844387298, -94.87500000409677625 ) ) ;
#2381=CARTESIAN_POINT ( 'NONE',  ( -5.405949406249996869, 9.363379034771805109, -50.34375000204835260 ) ) ;
#2386=CARTESIAN_POINT ( 'NONE',  ( -5.000000000000003553, -8.660254037844383745, -16.37500000409675138 ) ) ;
#2387=CARTESIAN_POINT ( 'NONE',  ( 10.00000000000051159, -5.773502691895965988, -119.5000000040967905 ) ) ;
#2389=ORIENTED_EDGE ( 'NONE', *, *, #4119, .T. ) ;
#2390=CARTESIAN_POINT ( 'NONE',  ( -8.660253955908514101, -5.000000141917089636, -180.0000000000000284 ) ) ;
#2400=CARTESIAN_POINT ( 'NONE',  ( -2.293366432827344421E-15, -12.48450537969573659, -186.4062500020484094 ) ) ;
#2402=FACE_OUTER_BOUND ( 'NONE', #32173, .T. ) ;
#2404=CARTESIAN_POINT ( 'NONE',  ( 10.81189881249999729, 0.000000000000000000, -109.3437500020483810 ) ) ;
#2406=CARTESIAN_POINT ( 'NONE',  ( 5.405949406249992428, -9.363379034771808662, -114.2812500020483952 ) ) ;
#2408=CARTESIAN_POINT ( 'NONE',  ( 5.405949406249999534, 9.363379034771803333, -124.0937500020483952 ) ) ;
#2411=CARTESIAN_POINT ( 'NONE',  ( 4.999999999999992006, -8.660254037844389075, -138.7499999999999716 ) ) ;
#2412=CARTESIAN_POINT ( 'NONE',  ( -9.999999999999998224, 5.773502691896259087, -13.37499999999996980 ) ) ;
#2415=CARTESIAN_POINT ( 'NONE',  ( 4.999999999999992006, -8.660254037844389075, -191.6250000040967905 ) ) ;
#2417=CARTESIAN_POINT ( 'NONE',  ( 5.405949406249999534, 9.363379034771803333, -35.59375000204836681 ) ) ;
#2419=CARTESIAN_POINT ( 'NONE',  ( 10.81189881249999729, 0.000000000000000000, -149.8437500020483810 ) ) ;
#2421=CARTESIAN_POINT ( 'NONE',  ( 10.00000000000000000, 5.773502691896255534, -136.8750000000000000 ) ) ;
#2422=CARTESIAN_POINT ( 'NONE',  ( 4.999999999999992006, -8.660254037844389075, -77.24999999999998579 ) ) ;
#2423=CARTESIAN_POINT ( 'NONE',  ( 5.405949406249992428, -9.363379034771808662, -141.2812500020483810 ) ) ;
#2427=CARTESIAN_POINT ( 'NONE',  ( -5.000000000000003553, -8.660254037844383745, -116.8750000040967905 ) ) ;
#2428=CARTESIAN_POINT ( 'NONE',  ( 10.81189881249999907, 6.242252689847868297, -71.71875000204836681 ) ) ;
#2432=CARTESIAN_POINT ( 'NONE',  ( -4.999999999999996447, 8.660254037844387298, -118.8750000040967905 ) ) ;
#2433=CARTESIAN_POINT ( 'NONE',  ( -10.81189881249999729, 1.324075727343319199E-15, -35.28125000204837391 ) ) ;
#2445=CARTESIAN_POINT ( 'NONE',  ( 4.999999999999992006, -8.660254037844389075, -176.6250000040968189 ) ) ;
#2451=CARTESIAN_POINT ( 'NONE',  ( -2.121150477449813534E-15, -11.54700538379251284, -176.3750000000000000 ) ) ;
#2452=CARTESIAN_POINT ( 'NONE',  ( -2.293366432827344421E-15, -12.48450537969573659, -132.2187500020483810 ) ) ;
#2454=CARTESIAN_POINT ( 'NONE',  ( -10.81189881249999729, 6.242252689847871849, -141.9062500020484094 ) ) ;
#2457=CARTESIAN_POINT ( 'NONE',  ( 10.81189881249999729, 0.000000000000000000, -145.3437500020483810 ) ) ;
#2459=DIRECTION ( 'NONE',  ( -0.000000000000000000, -0.000000000000000000, -1.000000000000000000 ) ) ;
#2460=CARTESIAN_POINT ( 'NONE',  ( -9.999999999999998224, 5.773502691896259087, -169.3750000000000000 ) ) ;
#2464=CARTESIAN_POINT ( 'NONE',  ( -2.293366432827344421E-15, -12.48450537969573659, -63.21875000204838102 ) ) ;
#2465=CARTESIAN_POINT ( 'NONE',  ( 10.00000000000051159, -5.773502691895965988, -149.1249999999999716 ) ) ;
#2466=CARTESIAN_POINT ( 'NONE',  ( 5.405949406249999534, 9.363379034771803333, -170.5937500020484094 ) ) ;
#2469=VECTOR ( 'NONE', #30727, 1000.000000000000000 ) ;
#2471=CARTESIAN_POINT ( 'NONE',  ( 5.405949406249992428, -9.363379034771808662, -33.28125000204837391 ) ) ;
#2473=CARTESIAN_POINT ( 'NONE',  ( 10.00000000000000000, 5.773502691896255534, -102.3749999999999858 ) ) ;
#2475=CARTESIAN_POINT ( 'NONE',  ( 10.81189881249999729, 6.242252689847867408, -118.4062500020483810 ) ) ;
#2476=CARTESIAN_POINT ( 'NONE',  ( -4.999999999999996447, 8.660254037844387298, -141.3750000040967905 ) ) ;
#2477=CARTESIAN_POINT ( 'NONE',  ( 9.999999999999998224, 0.000000000000000000, -125.0000000000000000 ) ) ;
#2482=CARTESIAN_POINT ( 'NONE',  ( -5.405949406250003975, -9.363379034771801557, -59.03125000204836681 ) ) ;
#2489=AXIS2_PLACEMENT_3D ( 'NONE', #21699, #28618, #1866 ) ;
#2497=VERTEX_POINT ( 'NONE', #39412 ) ;
#2500=EDGE_CURVE ( 'NONE', #342, #5087, #34448, .T. ) ;
#2508=CARTESIAN_POINT ( 'NONE',  ( 10.00000000000000000, 5.773502691896255534, -33.37499999999996447 ) ) ;
#2511=CARTESIAN_POINT ( 'NONE',  ( -10.81189881249999907, -6.242252689847864744, -156.4687500020484379 ) ) ;
#2512=CARTESIAN_POINT ( 'NONE',  ( -2.293366432827344421E-15, -12.48450537969573659, -169.7187500020483810 ) ) ;
#2515=CARTESIAN_POINT ( 'NONE',  ( 9.999999999999998224, 0.000000000000000000, -192.5000000000000000 ) ) ;
#2520=CARTESIAN_POINT ( 'NONE',  ( -10.81189881249999907, -6.242252689847864744, -59.15625000204838102 ) ) ;
#2522=CARTESIAN_POINT ( 'NONE',  ( -4.999999999999996447, 8.660254037844387298, -120.0000000000000000 ) ) ;
#2523=ADVANCED_FACE ( 'NONE', ( #29927 ), #10474, .F. ) ;
#2525=CARTESIAN_POINT ( 'NONE',  ( -5.405949406250003975, -9.363379034771801557, -138.5312500020484094 ) ) ;
#2526=CARTESIAN_POINT ( 'NONE',  ( -10.81189881249999729, 6.242252689847871849, -158.4062500020483810 ) ) ;
#2529=CARTESIAN_POINT ( 'NONE',  ( 10.81189881249999907, 6.242252689847868297, -92.71875000204836681 ) ) ;
#2532=CARTESIAN_POINT ( 'NONE',  ( -10.81189881249999729, 1.324075727343319199E-15, -185.0937500020483810 ) ) ;
#2534=CARTESIAN_POINT ( 'NONE',  ( -4.999999999999996447, 8.660254037844387298, -165.0000000000000000 ) ) ;
#2535=CARTESIAN_POINT ( 'NONE',  ( -5.000000000000003553, -8.660254037844383745, -145.0000000000000000 ) ) ;
#2536=CARTESIAN_POINT ( 'NONE',  ( 5.405949406249999534, 9.363379034771803333, -95.78125000204838102 ) ) ;
#2538=CARTESIAN_POINT ( 'NONE',  ( 7.070501591499377789E-16, 11.54700538379251284, -71.00000000409676204 ) ) ;
#2540=CARTESIAN_POINT ( 'NONE',  ( 10.81189881249999551, -6.242252689847874514, -22.46875000204837036 ) ) ;
#2541=ORIENTED_EDGE ( 'NONE', *, *, #35673, .F. ) ;
#2543=CARTESIAN_POINT ( 'NONE',  ( -10.81189881249999907, -6.242252689847864744, -20.15625000204837747 ) ) ;
#2561=LINE ( 'NONE', #31489, #24582 ) ;
#2563=CARTESIAN_POINT ( 'NONE',  ( -10.81189881249999729, 1.324075727343319199E-15, -159.7812500020484094 ) ) ;
#2569=CARTESIAN_POINT ( 'NONE',  ( -10.81189881249999729, 6.242252689847871849, -81.71875000204838102 ) ) ;
#2570=CARTESIAN_POINT ( 'NONE',  ( 10.81189881249999729, 0.000000000000000000, -88.53125000204838102 ) ) ;
#2572=DIRECTION ( 'NONE',  ( -0.000000000000000000, -0.000000000000000000, -1.000000000000000000 ) ) ;
#2573=CARTESIAN_POINT ( 'NONE',  ( 10.81189881249999729, 6.242252689847867408, -166.4062500020483810 ) ) ;
#2574=CARTESIAN_POINT ( 'NONE',  ( 10.81189881249999551, -6.242252689847874514, -183.1562500020484094 ) ) ;
#2576=CARTESIAN_POINT ( 'NONE',  ( -5.000000000000003553, -8.660254037844383745, -163.3750000040967905 ) ) ;
#2578=CARTESIAN_POINT ( 'NONE',  ( 7.644554776091147741E-16, 12.48450537969573659, -14.46875000204836503 ) ) ;
#2580=CARTESIAN_POINT ( 'NONE',  ( -10.81189881249999729, 6.242252689847871849, -116.2187500020483810 ) ) ;
#2582=CARTESIAN_POINT ( 'NONE',  ( -10.81189881249999729, 1.324075727343319199E-15, -20.28125000204836326 ) ) ;
#2585=CARTESIAN_POINT ( 'NONE',  ( -10.81189881249999729, 6.242252689847871849, -114.9062500020483952 ) ) ;
#2588=CARTESIAN_POINT ( 'NONE',  ( -10.00000000000000000, -5.773502691896251982, -93.00000000409679046 ) ) ;
#2591=CARTESIAN_POINT ( 'NONE',  ( 5.405949406249999534, 9.363379034771803333, -50.59375000204835260 ) ) ;
#2596=CARTESIAN_POINT ( 'NONE',  ( 7.070501591499377789E-16, 11.54700538379251284, -23.00000000409677270 ) ) ;
#2597=( BOUNDED_CURVE ( )  B_SPLINE_CURVE ( 2, ( #8920, #5042, #18405, #15791, #21648, #25543, #28354 ),
 .UNSPECIFIED., .F., .F. ) 
 B_SPLINE_CURVE_WITH_KNOTS ( ( 3, 2, 2, 3 ),
 ( 0.3395522388059703522, 0.3407960199004976820, 0.3420398009950250118, 0.3432835820895522860 ),
 .UNSPECIFIED. ) 
 CURVE ( )  GEOMETRIC_REPRESENTATION_ITEM ( )  RATIONAL_B_SPLINE_CURVE ( ( 0.9999999999999761302, 0.8660254037844625774, 1.000000000000000000, 0.8660254037844387076, 1.000000000000000000, 0.8660254037844327124, 1.000000000000005995 ) ) 
 REPRESENTATION_ITEM ( '' )  );
#2610=CARTESIAN_POINT ( 'NONE',  ( 7.644554776091147741E-16, 12.48450537969573659, -179.6562500020484094 ) ) ;
#2614=CARTESIAN_POINT ( 'NONE',  ( -5.405949406249996869, 9.363379034771805109, -105.8437500020483810 ) ) ;
#2616=CARTESIAN_POINT ( 'NONE',  ( 7.644554776091147741E-16, 12.48450537969573659, -118.1562500020483952 ) ) ;
#2618=CARTESIAN_POINT ( 'NONE',  ( -10.81189881249999729, -6.242252689847864744, -118.9687500020483810 ) ) ;
#2621=CARTESIAN_POINT ( 'NONE',  ( -10.00000000000000000, -5.773502691896251982, -142.1250000000000000 ) ) ;
#2622=CARTESIAN_POINT ( 'NONE',  ( -2.121150477449813534E-15, -11.54700538379251284, -11.37499999999996803 ) ) ;
#2625=CARTESIAN_POINT ( 'NONE',  ( -4.999999999999996447, 8.660254037844387298, -189.3750000040967905 ) ) ;
#2627=CARTESIAN_POINT ( 'NONE',  ( -10.81189881249999729, 6.242252689847871849, -36.71875000204835260 ) ) ;
#2628=CARTESIAN_POINT ( 'NONE',  ( -4.999999999999996447, 8.660254037844387298, -148.8750000040967905 ) ) ;
#2629=CARTESIAN_POINT ( 'NONE',  ( 5.405949406249992428, -9.363379034771808662, -147.0937500020483810 ) ) ;
#2632=EDGE_CURVE ( 'NONE', #24776, #23457, #28398, .T. ) ;
#2633=DIRECTION ( 'NONE',  ( -1.000000000000000000, 0.000000000000000000, 0.000000000000000000 ) ) ;
#2634=CARTESIAN_POINT ( 'NONE',  ( 9.999999999999996447, -5.773502691896262640, -69.62499999999998579 ) ) ;
#2635=CARTESIAN_POINT ( 'NONE',  ( 10.81189881249999907, 6.242252689847868297, -142.4062500020484094 ) ) ;
#2638=CARTESIAN_POINT ( 'NONE',  ( -2.121150477449813534E-15, -11.54700538379251284, -118.2500000040968047 ) ) ;
#2640=CARTESIAN_POINT ( 'NONE',  ( 7.644554776091147741E-16, 12.48450537969573659, -75.96875000204838102 ) ) ;
#2644=CARTESIAN_POINT ( 'NONE',  ( -5.000000000000003553, -8.660254037844383745, -157.3750000040967905 ) ) ;
#2645=CARTESIAN_POINT ( 'NONE',  ( -10.81189881249999729, 1.324075727343319199E-15, -33.78125000204837391 ) ) ;
#2649=DIRECTION ( 'NONE',  ( -1.000000000000000000, 0.000000000000000000, 0.000000000000000000 ) ) ;
#2661=CARTESIAN_POINT ( 'NONE',  ( 10.81189881249999907, 6.242252689847868297, -131.7187500020483810 ) ) ;
#2662=CARTESIAN_POINT ( 'NONE',  ( 5.405949406249992428, -9.363379034771808662, -139.7812500020483810 ) ) ;
#2664=CARTESIAN_POINT ( 'NONE',  ( -5.405949406250003975, -9.363379034771801557, -144.3437500020483810 ) ) ;
#2667=CARTESIAN_POINT ( 'NONE',  ( -10.00000000000000000, -5.773502691896251982, -163.1250000000000284 ) ) ;
#2669=CARTESIAN_POINT ( 'NONE',  ( 1.351487262974977233, 10.72709830801206543, -100.0000000000000000 ) ) ;
#2671=CARTESIAN_POINT ( 'NONE',  ( -10.81189881249999907, -6.242252689847864744, -61.96875000204838102 ) ) ;
#2672=LINE ( 'NONE', #5911, #13671 ) ;
#2673=CARTESIAN_POINT ( 'NONE',  ( 5.405949406249999534, 9.363379034771803333, -173.5937500020484094 ) ) ;
#2678=CARTESIAN_POINT ( 'NONE',  ( 4.999999999999992006, -8.660254037844389075, -89.24999999999998579 ) ) ;
#2680=CARTESIAN_POINT ( 'NONE',  ( 5.405949406249992428, -9.363379034771808662, -115.7812500020483952 ) ) ;
#2681=CARTESIAN_POINT ( 'NONE',  ( -9.999999999999998224, 1.224646799147353059E-15, -141.1250000040967905 ) ) ;
#2685=ADVANCED_FACE ( 'NONE', ( #788 ), #13066, .F. ) ;
#2686=AXIS2_PLACEMENT_3D ( 'NONE', #37107, #1080, #7551 ) ;
#2688=CARTESIAN_POINT ( 'NONE',  ( 10.81189881249999551, -6.242252689847874514, -61.65625000204838813 ) ) ;
#2691=CARTESIAN_POINT ( 'NONE',  ( -9.999999999999872102, -5.773502691896326589, -163.1250000000000000 ) ) ;
#2695=CARTESIAN_POINT ( 'NONE',  ( 0.000000000000000000, 0.000000000000000000, -99.99999999999998579 ) ) ;
#2697=ORIENTED_EDGE ( 'NONE', *, *, #31089, .T. ) ;
#2707=FACE_OUTER_BOUND ( 'NONE', #8962, .T. ) ;
#2708=CARTESIAN_POINT ( 'NONE',  ( 9.999999999999998224, 0.000000000000000000, -31.99999999999997158 ) ) ;
#2711=CARTESIAN_POINT ( 'NONE',  ( -10.81189881249999907, -6.242252689847864744, -157.9687500020484379 ) ) ;
#2712=CARTESIAN_POINT ( 'NONE',  ( 10.81189881249999729, 6.242252689847867408, -170.7187500020483810 ) ) ;
#2714=DIRECTION ( 'NONE',  ( -0.000000000000000000, -0.000000000000000000, -1.000000000000000000 ) ) ;
#2715=CARTESIAN_POINT ( 'NONE',  ( -10.00000000000000000, -5.773502691896251982, -187.1250000000000284 ) ) ;
#2716=AXIS2_PLACEMENT_3D ( 'NONE', #32719, #9196, #2730 ) ;
#2722=CARTESIAN_POINT ( 'NONE',  ( 10.81189881249999729, 0.000000000000000000, -60.03125000204836681 ) ) ;
#2724=CARTESIAN_POINT ( 'NONE',  ( -9.999999999999998224, 5.773502691896259087, -125.8749999999999858 ) ) ;
#2725=ORIENTED_EDGE ( 'NONE', *, *, #651, .F. ) ;
#2727=CARTESIAN_POINT ( 'NONE',  ( -10.81189881249999729, 1.324075727343319199E-15, -140.2812500020483810 ) ) ;
#2728=CARTESIAN_POINT ( 'NONE',  ( 7.644554776091147741E-16, 12.48450537969573659, -160.1562500020484094 ) ) ;
#2730=DIRECTION ( 'NONE',  ( -1.000000000000000000, 0.000000000000000000, 0.000000000000000000 ) ) ;
#2731=CARTESIAN_POINT ( 'NONE',  ( -2.293366432827344421E-15, -12.48450537969573659, -91.71875000204838102 ) ) ;
#2733=ORIENTED_EDGE ( 'NONE', *, *, #18814, .T. ) ;
#2735=CARTESIAN_POINT ( 'NONE',  ( -5.405949406250003975, -9.363379034771801557, -186.3437500020483810 ) ) ;
#2738=EDGE_CURVE ( 'NONE', #11060, #7201, #24090, .T. ) ;
#2739=LINE ( 'NONE', #35760, #13424 ) ;
#2741=CARTESIAN_POINT ( 'NONE',  ( 5.405949406249999534, 9.363379034771803333, -88.28125000204838102 ) ) ;
#2744=CARTESIAN_POINT ( 'NONE',  ( -5.000000000000003553, -8.660254037844383745, -59.87500000409676204 ) ) ;
#2745=CARTESIAN_POINT ( 'NONE',  ( 5.405949406249999534, 9.363379034771803333, -14.59375000204835082 ) ) ;
#2746=ORIENTED_EDGE ( 'NONE', *, *, #1154, .F. ) ;
#2748=CARTESIAN_POINT ( 'NONE',  ( -10.81189881249999907, -6.242252689847864744, -15.65625000204837214 ) ) ;
#2758=ORIENTED_EDGE ( 'NONE', *, *, #29095, .T. ) ;
#2768=CARTESIAN_POINT ( 'NONE',  ( 9.999999999999998224, 0.000000000000000000, -126.8750000040967905 ) ) ;
#2769=CARTESIAN_POINT ( 'NONE',  ( -9.999999999999998224, 1.224646799147353059E-15, -128.7499999999999716 ) ) ;
#2770=CARTESIAN_POINT ( 'NONE',  ( -5.405949406249996869, 9.363379034771805109, -160.0312500020484094 ) ) ;
#2777=CARTESIAN_POINT ( 'NONE',  ( 10.81189881249999907, 6.242252689847868297, -79.21875000204838102 ) ) ;
#2778=CARTESIAN_POINT ( 'NONE',  ( 5.405949406249992428, -9.363379034771808662, -81.28125000204839523 ) ) ;
#2781=CARTESIAN_POINT ( 'NONE',  ( 5.405949406249992428, -9.363379034771808662, -169.7812500020484094 ) ) ;
#2782=CARTESIAN_POINT ( 'NONE',  ( 5.405949406249999534, 9.363379034771803333, -178.2812500020484094 ) ) ;
#2783=CARTESIAN_POINT ( 'NONE',  ( 4.999999999999992006, -8.660254037844389075, -152.6250000040967905 ) ) ;
#2785=CARTESIAN_POINT ( 'NONE',  ( 7.644554776091147741E-16, 12.48450537969573659, -2.468750002048353043 ) ) ;
#2787=CARTESIAN_POINT ( 'NONE',  ( -10.81189881249999729, 6.242252689847871849, -110.2187500020483810 ) ) ;
#2789=CARTESIAN_POINT ( 'NONE',  ( -10.81189881249999729, 6.242252689847871849, -15.90625000204837036 ) ) ;
#2792=CARTESIAN_POINT ( 'NONE',  ( 10.81189881249999907, 6.242252689847868297, -107.9062500020483668 ) ) ;
#2795=CARTESIAN_POINT ( 'NONE',  ( -4.999999999999996447, 8.660254037844387298, -82.87500000409676204 ) ) ;
#2796=CARTESIAN_POINT ( 'NONE',  ( -5.000000000000003553, -8.660254037844383745, -101.5000000000000000 ) ) ;
#2797=CARTESIAN_POINT ( 'NONE',  ( 5.405949406249992428, -9.363379034771808662, -40.59375000204837391 ) ) ;
#2798=ORIENTED_EDGE ( 'NONE', *, *, #29945, .T. ) ;
#2803=CARTESIAN_POINT ( 'NONE',  ( 4.999999999999992006, -8.660254037844389075, -17.62500000409675138 ) ) ;
#2813=ORIENTED_EDGE ( 'NONE', *, *, #21859, .F. ) ;
#2817=CARTESIAN_POINT ( 'NONE',  ( 10.81189881249999907, 6.242252689847868297, -184.4062500020484094 ) ) ;
#2819=DIRECTION ( 'NONE',  ( -1.000000000000000000, 0.000000000000000000, 0.000000000000000000 ) ) ;
#2821=CARTESIAN_POINT ( 'NONE',  ( 5.405949406249992428, -9.363379034771808662, -103.5937500020483668 ) ) ;
#2822=CARTESIAN_POINT ( 'NONE',  ( 9.999999999999998224, 0.000000000000000000, -113.3750000040967763 ) ) ;
#2823=CARTESIAN_POINT ( 'NONE',  ( 7.644554776091147741E-16, 12.48450537969573659, -106.1562500020483952 ) ) ;
#2825=CARTESIAN_POINT ( 'NONE',  ( -5.405949406250003975, -9.363379034771801557, -118.8437500020483810 ) ) ;
#2828=CARTESIAN_POINT ( 'NONE',  ( -4.999999999999996447, 8.660254037844387298, -138.0000000000000000 ) ) ;
#2829=CARTESIAN_POINT ( 'NONE',  ( -2.121150477449813534E-15, -11.54700538379251284, -5.374999999999963585 ) ) ;
#2832=CARTESIAN_POINT ( 'NONE',  ( -9.999999999999998224, 1.224646799147353059E-15, -177.1250000040968189 ) ) ;
#2834=CARTESIAN_POINT ( 'NONE',  ( -2.293366432827344421E-15, -12.48450537969573659, -31.71875000204834905 ) ) ;
#2836=CARTESIAN_POINT ( 'NONE',  ( -5.405949406250003975, -9.363379034771801557, -135.3437500020484094 ) ) ;
#2839=CARTESIAN_POINT ( 'NONE',  ( -2.121150477449813534E-15, -11.54700538379251284, -66.87499999999998579 ) ) ;
#2840=CARTESIAN_POINT ( 'NONE',  ( -2.293366432827344421E-15, -12.48450537969573659, -142.9062500020483810 ) ) ;
#2843=( BOUNDED_CURVE ( )  B_SPLINE_CURVE ( 2, ( #38433, #11881, #28306, #35211, #25499, #5641, #21820 ),
 .UNSPECIFIED., .F., .F. ) 
 B_SPLINE_CURVE_WITH_KNOTS ( ( 3, 2, 2, 3 ),
 ( 0.2425373134328359381, 0.2437810945273632957, 0.2450248756218906532, 0.2462686567164180107 ),
 .UNSPECIFIED. ) 
 CURVE ( )  GEOMETRIC_REPRESENTATION_ITEM ( )  RATIONAL_B_SPLINE_CURVE ( ( 0.9999999999999880096, 0.8660254037844506980, 1.000000000000000000, 0.8660254037844387076, 1.000000000000000000, 0.8660254037844267172, 1.000000000000011990 ) ) 
 REPRESENTATION_ITEM ( '' )  );
#2845=CARTESIAN_POINT ( 'NONE',  ( 4.999999999999992006, -8.660254037844389075, -115.1250000040967905 ) ) ;
#2846=CARTESIAN_POINT ( 'NONE',  ( 7.070501591499376803E-16, 11.54700538379251284, -169.6250000000000000 ) ) ;
#2847=CARTESIAN_POINT ( 'NONE',  ( 7.644554776091147741E-16, 12.48450537969573659, -62.46875000204838102 ) ) ;
#2853=CARTESIAN_POINT ( 'NONE',  ( -10.00000000000000000, -5.773502691896251982, -42.00000000409675494 ) ) ;
#2854=CARTESIAN_POINT ( 'NONE',  ( -10.81189881249999907, -6.242252689847864744, -33.65625000204835970 ) ) ;
#2856=CARTESIAN_POINT ( 'NONE',  ( 5.000000000000000000, 8.660254037844385522, -166.7500000000000000 ) ) ;
#2861=ORIENTED_EDGE ( 'NONE', *, *, #19230, .F. ) ;
#2866=CARTESIAN_POINT ( 'NONE',  ( 9.999999999999998224, 0.000000000000000000, -135.8750000040967905 ) ) ;
#2870=LINE ( 'NONE', #26168, #1960 ) ;
#2874=CARTESIAN_POINT ( 'NONE',  ( 10.81189881249999551, -6.242252689847874514, -127.4687500020483810 ) ) ;
#2875=CARTESIAN_POINT ( 'NONE',  ( 5.405949406249992428, -9.363379034771808662, -130.7812500020483810 ) ) ;
#2877=CARTESIAN_POINT ( 'NONE',  ( 10.81189881249999729, 0.000000000000000000, -148.3437500020483810 ) ) ;
#2878=CARTESIAN_POINT ( 'NONE',  ( 10.75125155253628684, -1.347400678069339497, -179.9999999999999716 ) ) ;
#2880=CARTESIAN_POINT ( 'NONE',  ( -9.999999999999998224, 5.773502691896259087, -163.3750000000000000 ) ) ;
#2884=CARTESIAN_POINT ( 'NONE',  ( 10.81189881249999551, -6.242252689847874514, -61.46875000204837391 ) ) ;
#2885=CARTESIAN_POINT ( 'NONE',  ( 9.999999999999998224, 0.000000000000000000, -174.5000000000000284 ) ) ;
#2886=CARTESIAN_POINT ( 'NONE',  ( 10.81189881249999907, 6.242252689847868297, -161.7187500020483810 ) ) ;
#2889=DIRECTION ( 'NONE',  ( -0.000000000000000000, -0.000000000000000000, -1.000000000000000000 ) ) ;
#2891=CARTESIAN_POINT ( 'NONE',  ( 5.000000000000000000, 8.660254037844385522, -88.74999999999998579 ) ) ;
#2893=CARTESIAN_POINT ( 'NONE',  ( -10.81189881249999729, 6.242252689847871849, -119.4062500020483952 ) ) ;
#2894=CARTESIAN_POINT ( 'NONE',  ( -4.999999999999996447, 8.660254037844387298, -139.8750000040968189 ) ) ;
#2899=CARTESIAN_POINT ( 'NONE',  ( 10.81189881249999907, 6.242252689847868297, -58.40625000204838102 ) ) ;
#2901=EDGE_CURVE ( 'NONE', #34857, #5520, #8109, .T. ) ;
#2902=LINE ( 'NONE', #29227, #32461 ) ;
#2907=ORIENTED_EDGE ( 'NONE', *, *, #27941, .F. ) ;
#2908=CARTESIAN_POINT ( 'NONE',  ( -9.999999999999996447, 5.773502691896259975, -172.7500000040967905 ) ) ;
#2912=DIRECTION ( 'NONE',  ( -0.000000000000000000, -0.000000000000000000, -1.000000000000000000 ) ) ;
#2914=( BOUNDED_CURVE ( )  B_SPLINE_CURVE ( 2, ( #26707, #10293, #24063, #34210, #7652, #20803, #33991 ),
 .UNSPECIFIED., .F., .F. ) 
 B_SPLINE_CURVE_WITH_KNOTS ( ( 3, 2, 2, 3 ),
 ( 0.4179104477611941260, 0.4191542288557215112, 0.4203980099502488965, 0.4216417910447762818 ),
 .UNSPECIFIED. ) 
 CURVE ( )  GEOMETRIC_REPRESENTATION_ITEM ( )  RATIONAL_B_SPLINE_CURVE ( ( 0.9999999999999880096, 0.8660254037844506980, 1.000000000000000000, 0.8660254037844387076, 1.000000000000000000, 0.8660254037844207220, 1.000000000000017986 ) ) 
 REPRESENTATION_ITEM ( '' )  );
#2915=ORIENTED_EDGE ( 'NONE', *, *, #25715, .T. ) ;
#2920=LINE ( 'NONE', #39161, #36379 ) ;
#2921=ADVANCED_FACE ( 'NONE', ( #5084 ), #998, .T. ) ;
#2922=CARTESIAN_POINT ( 'NONE',  ( 9.999999999999998224, 0.000000000000000000, -27.49999999999996803 ) ) ;
#2925=CARTESIAN_POINT ( 'NONE',  ( 10.81189881249999551, -6.242252689847874514, -157.4687500020484094 ) ) ;
#2926=VECTOR ( 'NONE', #25853, 1000.000000000000000 ) ;
#2927=CARTESIAN_POINT ( 'NONE',  ( 5.405949406249992428, -9.363379034771808662, -174.0937500020484094 ) ) ;
#2930=CARTESIAN_POINT ( 'NONE',  ( 9.999999999999996447, -5.773502691896262640, -191.1250000000000000 ) ) ;
#2935=CARTESIAN_POINT ( 'NONE',  ( -5.405949406249996869, 9.363379034771805109, -195.8437500020484094 ) ) ;
#2937=CARTESIAN_POINT ( 'NONE',  ( 10.81189881249999907, 6.242252689847868297, -61.40625000204838102 ) ) ;
#2939=CARTESIAN_POINT ( 'NONE',  ( -9.999999999999998224, 5.773502691896259087, -113.8750000000000000 ) ) ;
#2940=EDGE_LOOP ( 'NONE', ( #37354, #29611, #22134, #12697 ) ) ;
#2941=CARTESIAN_POINT ( 'NONE',  ( 10.81189881249999729, 6.242252689847867408, -145.4062500020484094 ) ) ;
#2942=CARTESIAN_POINT ( 'NONE',  ( -5.405949406250003975, -9.363379034771801557, -153.5312500020484094 ) ) ;
#2946=CARTESIAN_POINT ( 'NONE',  ( -5.405949406249996869, 9.363379034771805109, -87.84375000204836681 ) ) ;
#2949=CARTESIAN_POINT ( 'NONE',  ( 10.81189881249999907, 6.242252689847868297, -191.7187500020484094 ) ) ;
#2953=CARTESIAN_POINT ( 'NONE',  ( 10.81189881249999907, 6.242252689847868297, -82.40625000204836681 ) ) ;
#2955=CARTESIAN_POINT ( 'NONE',  ( -9.999999999999998224, 1.224646799147353059E-15, -60.12500000409676204 ) ) ;
#2956=CARTESIAN_POINT ( 'NONE',  ( -5.405949406250003975, -9.363379034771801557, -15.34375000204835082 ) ) ;
#2957=CARTESIAN_POINT ( 'NONE',  ( 9.999999999999998224, 1.224646799147353059E-15, -99.99999999999998579 ) ) ;
#2959=CARTESIAN_POINT ( 'NONE',  ( -5.405949406250003975, -9.363379034771801557, -11.03125000204835438 ) ) ;
#2976=LINE ( 'NONE', #28247, #25674 ) ;
#2981=DIRECTION ( 'NONE',  ( 0.000000000000000000, 0.000000000000000000, 1.000000000000000000 ) ) ;
#2982=CARTESIAN_POINT ( 'NONE',  ( 10.81189881249999551, -6.242252689847874514, -154.6562500020484379 ) ) ;
#2988=CARTESIAN_POINT ( 'NONE',  ( -2.293366432827344421E-15, -12.48450537969573659, -76.71875000204838102 ) ) ;
#2989=CARTESIAN_POINT ( 'NONE',  ( 5.405949406249992428, -9.363379034771808662, -82.78125000204838102 ) ) ;
#2992=CARTESIAN_POINT ( 'NONE',  ( 10.81189881249999729, 6.242252689847867408, -167.9062500020484094 ) ) ;
#2993=CARTESIAN_POINT ( 'NONE',  ( -10.81189881249999907, -6.242252689847864744, -180.6562500020484094 ) ) ;
#2994=CARTESIAN_POINT ( 'NONE',  ( -10.00000000000000000, -5.773502691896251982, -156.0000000040967905 ) ) ;
#2996=CARTESIAN_POINT ( 'NONE',  ( 10.81189881249999551, -6.242252689847874514, -7.468750002048357928 ) ) ;
#2997=CARTESIAN_POINT ( 'NONE',  ( 9.999999999999998224, 0.000000000000000000, -162.8750000040967905 ) ) ;
#2998=CARTESIAN_POINT ( 'NONE',  ( -5.405949406249996869, 9.363379034771805109, -117.8437500020483810 ) ) ;
#3000=CARTESIAN_POINT ( 'NONE',  ( -5.405949406250003975, -9.363379034771801557, -14.03125000204835615 ) ) ;
#3004=CARTESIAN_POINT ( 'NONE',  ( 5.405949406249992428, -9.363379034771808662, -105.2812500020483810 ) ) ;
#3006=VERTEX_POINT ( 'NONE', #38304 ) ;
#3007=CARTESIAN_POINT ( 'NONE',  ( 5.000000000000000000, 8.660254037844385522, -83.12500000409676204 ) ) ;
#3009=CARTESIAN_POINT ( 'NONE',  ( -2.293366432827344421E-15, -12.48450537969573659, -39.21875000204835970 ) ) ;
#3014=CARTESIAN_POINT ( 'NONE',  ( 4.999999999999992006, -8.660254037844389075, -14.62500000409674961 ) ) ;
#3015=CARTESIAN_POINT ( 'NONE',  ( -2.121150477449813534E-15, -11.54700538379251284, -119.7500000040967905 ) ) ;
#3018=CARTESIAN_POINT ( 'NONE',  ( -9.999999999999998224, 1.224646799147353059E-15, -152.7500000000000000 ) ) ;
#3024=ORIENTED_EDGE ( 'NONE', *, *, #1117, .T. ) ;
#3028=CARTESIAN_POINT ( 'NONE',  ( 5.405949406249999534, 9.363379034771803333, -182.7812500020484094 ) ) ;
#3030=CARTESIAN_POINT ( 'NONE',  ( 5.000000000000000000, 8.660254037844385522, -155.1250000040967905 ) ) ;
#3031=EDGE_CURVE ( 'NONE', #15525, #23116, #8537, .T. ) ;
#3033=CARTESIAN_POINT ( 'NONE',  ( -5.405949406250003975, -9.363379034771801557, -103.8437500020483810 ) ) ;
#3035=CARTESIAN_POINT ( 'NONE',  ( 10.81189881249999729, 0.000000000000000000, -111.0312500020483810 ) ) ;
#3037=CARTESIAN_POINT ( 'NONE',  ( 10.81189881249999551, -6.242252689847874514, -113.9687500020483668 ) ) ;
#3040=CARTESIAN_POINT ( 'NONE',  ( 9.999999999999998224, 0.000000000000000000, -137.0000000000000000 ) ) ;
#3041=CARTESIAN_POINT ( 'NONE',  ( -5.000000000000003553, -8.660254037844383745, -5.499999999999976907 ) ) ;
#3044=CARTESIAN_POINT ( 'NONE',  ( 10.00000000000000000, 5.773502691896255534, -182.2500000040968189 ) ) ;
#3046=CARTESIAN_POINT ( 'NONE',  ( -10.81189881249999729, 6.242252689847871849, -29.21875000204834905 ) ) ;
#3047=CARTESIAN_POINT ( 'NONE',  ( -4.999999999999996447, 8.660254037844387298, -117.0000000000000000 ) ) ;
#3048=CARTESIAN_POINT ( 'NONE',  ( -10.81189881249999729, 6.242252689847871849, -135.7187500020483810 ) ) ;
#3051=DIRECTION ( 'NONE',  ( -1.000000000000000000, 0.000000000000000000, 0.000000000000000000 ) ) ;
#3052=CARTESIAN_POINT ( 'NONE',  ( 5.000000000000000000, 8.660254037844385522, -64.74999999999997158 ) ) ;
#3053=CARTESIAN_POINT ( 'NONE',  ( -5.405949406250003975, -9.363379034771801557, -132.5312500020484094 ) ) ;
#3058=CARTESIAN_POINT ( 'NONE',  ( -4.999999999999996447, 8.660254037844387298, -111.3750000040967763 ) ) ;
#3060=CARTESIAN_POINT ( 'NONE',  ( -5.405949406249996869, 9.363379034771805109, -69.84375000204836681 ) ) ;
#3066=CARTESIAN_POINT ( 'NONE',  ( 10.00000000000000000, 5.773502691896255534, -38.25000000409675494 ) ) ;
#3067=CARTESIAN_POINT ( 'NONE',  ( -10.81189881249999729, 1.324075727343319199E-15, -39.78125000204838102 ) ) ;
#3071=CARTESIAN_POINT ( 'NONE',  ( -10.00000000000051337, 5.773502691895962435, -150.2500000040967620 ) ) ;
#3073=ORIENTED_EDGE ( 'NONE', *, *, #2738, .T. ) ;
#3078=CARTESIAN_POINT ( 'NONE',  ( 5.000000000000000000, 8.660254037844385522, -111.6250000040967763 ) ) ;
#3082=CARTESIAN_POINT ( 'NONE',  ( 10.81189881249999729, 0.000000000000000000, -122.8437500020483952 ) ) ;
#3083=CARTESIAN_POINT ( 'NONE',  ( 7.644554776091147741E-16, 12.48450537969573659, -131.6562500020483810 ) ) ;
#3085=CARTESIAN_POINT ( 'NONE',  ( -10.81189881249999729, 1.324075727343319199E-15, -138.5937500020483810 ) ) ;
#3086=CARTESIAN_POINT ( 'NONE',  ( 10.80649504056860088, 0.7923051018166373805, -180.0000000000000000 ) ) ;
#3088=CARTESIAN_POINT ( 'NONE',  ( -9.999999999999479527, -5.773502691896549521, -103.1249999999999858 ) ) ;
#3089=CARTESIAN_POINT ( 'NONE',  ( 9.999999999999998224, 0.000000000000000000, -164.0000000000000000 ) ) ;
#3094=CARTESIAN_POINT ( 'NONE',  ( -10.81189881249999907, -6.242252689847864744, -49.96875000204837391 ) ) ;
#3095=CARTESIAN_POINT ( 'NONE',  ( 5.405949406249992428, -9.363379034771808662, -163.5937500020484094 ) ) ;
#3100=CARTESIAN_POINT ( 'NONE',  ( -4.999999999999996447, 8.660254037844387298, -88.49999999999998579 ) ) ;
#3101=ORIENTED_EDGE ( 'NONE', *, *, #33115, .T. ) ;
#3102=( BOUNDED_CURVE ( )  B_SPLINE_CURVE ( 2, ( #15926, #42054, #2796, #29127, #41416, #38829, #28500 ),
 .UNSPECIFIED., .F., .F. ) 
 B_SPLINE_CURVE_WITH_KNOTS ( ( 3, 2, 2, 3 ),
 ( 0.4888059701492538101, 0.4900497512437811398, 0.4912935323383085806, 0.4925373134328359104 ),
 .UNSPECIFIED. ) 
 CURVE ( )  GEOMETRIC_REPRESENTATION_ITEM ( )  RATIONAL_B_SPLINE_CURVE ( ( 0.9999999999999940048, 0.8660254037844447028, 1.000000000000000000, 0.8660254037844387076, 1.000000000000000000, 0.8660254037844267172, 1.000000000000011990 ) ) 
 REPRESENTATION_ITEM ( '' )  );
#3103=CARTESIAN_POINT ( 'NONE',  ( -10.81189881249999729, 6.242252689847871849, -122.4062500020483952 ) ) ;
#3104=CARTESIAN_POINT ( 'NONE',  ( 4.999999999999992006, -8.660254037844389075, -136.1250000040967620 ) ) ;
#3108=CARTESIAN_POINT ( 'NONE',  ( 7.644554776091147741E-16, 12.48450537969573659, -62.65625000204838813 ) ) ;
#3114=CARTESIAN_POINT ( 'NONE',  ( 5.000000000000000000, 8.660254037844385522, -167.1250000040967905 ) ) ;
#3115=CARTESIAN_POINT ( 'NONE',  ( 5.000000000000000000, 8.660254037844385522, -174.2500000000000284 ) ) ;
#3119=ORIENTED_EDGE ( 'NONE', *, *, #33868, .T. ) ;
#3124=VECTOR ( 'NONE', #15169, 1000.000000000000000 ) ;
#3129=CARTESIAN_POINT ( 'NONE',  ( -9.999999999999998224, 1.224646799147353059E-15, -28.24999999999996803 ) ) ;
#3132=CARTESIAN_POINT ( 'NONE',  ( -10.81189881249999729, 6.242252689847871849, -152.2187500020483526 ) ) ;
#3133=CARTESIAN_POINT ( 'NONE',  ( -5.405949406250003975, -9.363379034771801557, -169.8437500020484094 ) ) ;
#3134=EDGE_CURVE ( 'NONE', #21806, #30027, #4937, .T. ) ;
#3135=CARTESIAN_POINT ( 'NONE',  ( -4.999999999999996447, 8.660254037844387298, -123.3750000040967905 ) ) ;
#3138=CARTESIAN_POINT ( 'NONE',  ( -10.00000000000000000, -5.773502691896251982, -188.6250000000000284 ) ) ;
#3143=CARTESIAN_POINT ( 'NONE',  ( -10.81189881249999907, -6.242252689847864744, -189.4687500020484094 ) ) ;
#3145=CARTESIAN_POINT ( 'NONE',  ( 10.81189881249999551, -6.242252689847874514, -60.15625000204838813 ) ) ;
#3147=CARTESIAN_POINT ( 'NONE',  ( -5.000000000000003553, -8.660254037844383745, -114.9999999999999858 ) ) ;
#3148=ORIENTED_EDGE ( 'NONE', *, *, #19813, .T. ) ;
#3149=CARTESIAN_POINT ( 'NONE',  ( 5.405949406249992428, -9.363379034771808662, -139.7812500020483810 ) ) ;
#3150=CARTESIAN_POINT ( 'NONE',  ( -5.405949406249996869, 9.363379034771805109, -157.0312500020484094 ) ) ;
#3152=CARTESIAN_POINT ( 'NONE',  ( -4.999999999999996447, 8.660254037844387298, -104.9999999999999858 ) ) ;
#3153=CARTESIAN_POINT ( 'NONE',  ( -10.81189881249999729, 1.324075727343319199E-15, -87.59375000204836681 ) ) ;
#3156=CARTESIAN_POINT ( 'NONE',  ( -10.81189881249999729, 1.324075727343319199E-15, -191.0937500020484094 ) ) ;
#3161=CARTESIAN_POINT ( 'NONE',  ( 10.81189881249999907, 6.242252689847868297, -86.90625000204836681 ) ) ;
#3165=CARTESIAN_POINT ( 'NONE',  ( 10.00000000000000000, 5.773502691896255534, -60.75000000409676915 ) ) ;
#3166=CARTESIAN_POINT ( 'NONE',  ( 10.81189881249999729, 0.000000000000000000, -17.84375000204835260 ) ) ;
#3167=CARTESIAN_POINT ( 'NONE',  ( -5.000000000000003553, -8.660254037844383745, -137.8750000040967905 ) ) ;
#3169=CARTESIAN_POINT ( 'NONE',  ( 7.644554776091147741E-16, 12.48450537969573659, -16.15625000204837391 ) ) ;
#3172=VECTOR ( 'NONE', #40705, 1000.000000000000000 ) ;
#3173=( BOUNDED_CURVE ( )  B_SPLINE_CURVE ( 2, ( #22582, #13055, #26249, #12424, #9202, #6400, #41995 ),
 .UNSPECIFIED., .F., .F. ) 
 B_SPLINE_CURVE_WITH_KNOTS ( ( 3, 2, 2, 3 ),
 ( 0.4067164179104478250, 0.4079601990049751548, 0.4092039800995025400, 0.4104477611940299253 ),
 .UNSPECIFIED. ) 
 CURVE ( )  GEOMETRIC_REPRESENTATION_ITEM ( )  RATIONAL_B_SPLINE_CURVE ( ( 0.9999999999999940048, 0.8660254037844447028, 1.000000000000000000, 0.8660254037844387076, 1.000000000000000000, 0.8660254037844327124, 1.000000000000005995 ) ) 
 REPRESENTATION_ITEM ( '' )  );
#3181=CARTESIAN_POINT ( 'NONE',  ( 5.405949406249999534, 9.363379034771803333, -101.5937500020483810 ) ) ;
#3183=ORIENTED_EDGE ( 'NONE', *, *, #13019, .F. ) ;
#3189=VECTOR ( 'NONE', #15892, 1000.000000000000000 ) ;
#3191=DIRECTION ( 'NONE',  ( 1.000000000000000000, 0.000000000000000000, 0.000000000000000000 ) ) ;
#3192=CARTESIAN_POINT ( 'NONE',  ( -5.405949406249996869, 9.363379034771805109, -154.0312500020484094 ) ) ;
#3198=CARTESIAN_POINT ( 'NONE',  ( -2.293366432827344421E-15, -12.48450537969573659, -78.21875000204838102 ) ) ;
#3199=CARTESIAN_POINT ( 'NONE',  ( -5.405949406250003975, -9.363379034771801557, -81.53125000204839523 ) ) ;
#3202=CARTESIAN_POINT ( 'NONE',  ( -5.405949406249996869, 9.363379034771805109, -164.5312500020484094 ) ) ;
#3203=CARTESIAN_POINT ( 'NONE',  ( 7.644554776091147741E-16, 12.48450537969573659, -176.6562500020484094 ) ) ;
#3204=CARTESIAN_POINT ( 'NONE',  ( -5.000000000000003553, -8.660254037844383745, -154.3750000040967905 ) ) ;
#3205=FACE_OUTER_BOUND ( 'NONE', #36082, .T. ) ;
#3206=CARTESIAN_POINT ( 'NONE',  ( -10.81189881249999729, 6.242252689847871849, -8.218750002048357928 ) ) ;
#3208=CARTESIAN_POINT ( 'NONE',  ( 10.81189881249999551, -6.242252689847874514, -116.9687500020483952 ) ) ;
#3210=CARTESIAN_POINT ( 'NONE',  ( -10.81189881249999907, -6.242252689847864744, -11.15625000204836859 ) ) ;
#3213=CARTESIAN_POINT ( 'NONE',  ( 10.81189881249999729, 0.000000000000000000, -108.0312500020483810 ) ) ;
#3217=CARTESIAN_POINT ( 'NONE',  ( 4.999999999999992006, -8.660254037844389075, -80.62500000409677625 ) ) ;
#3218=CARTESIAN_POINT ( 'NONE',  ( -9.999999999999998224, 1.224646799147353059E-15, -141.1250000040967905 ) ) ;
#3219=CARTESIAN_POINT ( 'NONE',  ( 10.81189881249999551, -6.242252689847874514, -43.46875000204836681 ) ) ;
#3224=CARTESIAN_POINT ( 'NONE',  ( -2.121150477449813534E-15, -11.54700538379251284, -11.75000000409676026 ) ) ;
#3225=EDGE_CURVE ( 'NONE', #33328, #28517, #33114, .T. ) ;
#3229=LINE ( 'NONE', #23288, #20688 ) ;
#3236=CYLINDRICAL_SURFACE ( 'NONE', #36275, 9.999999999999998224 ) ;
#3238=CARTESIAN_POINT ( 'NONE',  ( -10.81189881249999907, -6.242252689847864744, -179.1562500020484094 ) ) ;
#3240=FACE_OUTER_BOUND ( 'NONE', #25788, .T. ) ;
#3242=CARTESIAN_POINT ( 'NONE',  ( -10.81189881249999907, -6.242252689847864744, -100.9687500020483810 ) ) ;
#3244=CARTESIAN_POINT ( 'NONE',  ( 10.81189881249999551, -6.242252689847874514, -109.6562500020483810 ) ) ;
#3246=CARTESIAN_POINT ( 'NONE',  ( 7.644554776091147741E-16, 12.48450537969573659, -114.9687500020483668 ) ) ;
#3249=CARTESIAN_POINT ( 'NONE',  ( 4.999999999999992006, -8.660254037844389075, -141.7500000000000000 ) ) ;
#3250=CARTESIAN_POINT ( 'NONE',  ( -5.000000000000003553, -8.660254037844383745, -2.499999999999974243 ) ) ;
#3254=CARTESIAN_POINT ( 'NONE',  ( 4.999999999999992006, -8.660254037844389075, -184.1250000040967905 ) ) ;
#3256=CARTESIAN_POINT ( 'NONE',  ( 10.81189881249999729, 0.000000000000000000, -29.84375000204836326 ) ) ;
#3257=CARTESIAN_POINT ( 'NONE',  ( -9.999999999999998224, 1.224646799147353059E-15, -148.6250000040967905 ) ) ;
#3258=CARTESIAN_POINT ( 'NONE',  ( -10.81189881249999729, 6.242252689847871849, -140.2187500020483810 ) ) ;
#3260=CARTESIAN_POINT ( 'NONE',  ( 5.405949406249999534, 9.363379034771803333, -35.78125000204837391 ) ) ;
#3262=CARTESIAN_POINT ( 'NONE',  ( 7.070501591499377789E-16, 11.54700538379251284, -66.12500000000000000 ) ) ;
#3263=CARTESIAN_POINT ( 'NONE',  ( 5.405949406249992428, -9.363379034771808662, -132.2812500020483810 ) ) ;
#3267=CARTESIAN_POINT ( 'NONE',  ( 7.070501591499377789E-16, 11.54700538379251284, -107.0000000040967763 ) ) ;
#3268=CARTESIAN_POINT ( 'NONE',  ( 5.405949406249992428, -9.363379034771808662, -69.09375000204836681 ) ) ;
#3272=EDGE_CURVE ( 'NONE', #25139, #4764, #1664, .T. ) ;
#3274=CARTESIAN_POINT ( 'NONE',  ( -5.000000000000003553, -8.660254037844383745, -131.8750000040967905 ) ) ;
#3275=CARTESIAN_POINT ( 'NONE',  ( 4.999999999999992006, -8.660254037844389075, -32.62500000409676915 ) ) ;
#3276=EDGE_CURVE ( 'NONE', #516, #6299, #13646, .T. ) ;
#3277=CARTESIAN_POINT ( 'NONE',  ( -9.999999999999998224, 0.000000000000000000, -99.99999999999998579 ) ) ;
#3282=CARTESIAN_POINT ( 'NONE',  ( 9.999999999999998224, 0.000000000000000000, -122.3750000040967905 ) ) ;
#3294=( BOUNDED_CURVE ( )  B_SPLINE_CURVE ( 2, ( #33749, #14064, #27258, #40397, #10844, #37176, #20776 ),
 .UNSPECIFIED., .F., .F. ) 
 B_SPLINE_CURVE_WITH_KNOTS ( ( 3, 2, 2, 3 ),
 ( 0.1716417910447761430, 0.1728855721393035005, 0.1741293532338308858, 0.1753731343283582433 ),
 .UNSPECIFIED. ) 
 CURVE ( )  GEOMETRIC_REPRESENTATION_ITEM ( )  RATIONAL_B_SPLINE_CURVE ( ( 0.9999999999999970024, 0.8660254037844417052, 1.000000000000000000, 0.8660254037844387076, 1.000000000000000000, 0.8660254037844357100, 1.000000000000003109 ) ) 
 REPRESENTATION_ITEM ( '' )  );
#3296=CARTESIAN_POINT ( 'NONE',  ( 10.81189881249999907, 6.242252689847868297, -125.7187500020483810 ) ) ;
#3297=CARTESIAN_POINT ( 'NONE',  ( -10.81189881249999729, 1.324075727343319199E-15, -129.7812500020483810 ) ) ;
#3299=CARTESIAN_POINT ( 'NONE',  ( -5.405949406249996869, 9.363379034771805109, -135.8437500020484094 ) ) ;
#3301=CARTESIAN_POINT ( 'NONE',  ( 5.000000000000000000, 8.660254037844385522, -166.7500000000000000 ) ) ;
#3305=CARTESIAN_POINT ( 'NONE',  ( -10.81189881249999729, 1.324075727343319199E-15, -57.59375000204835970 ) ) ;
#3307=CARTESIAN_POINT ( 'NONE',  ( -5.405949406250003975, -9.363379034771801557, -163.8437500020484094 ) ) ;
#3312=CARTESIAN_POINT ( 'NONE',  ( 9.999999999999998224, 0.000000000000000000, -87.49999999999998579 ) ) ;
#3314=CARTESIAN_POINT ( 'NONE',  ( -5.405949406250003975, -9.363379034771801557, -107.0312500020483810 ) ) ;
#3315=CARTESIAN_POINT ( 'NONE',  ( -9.999999999999998224, 5.773502691896259087, -133.7500000040967905 ) ) ;
#3319=CARTESIAN_POINT ( 'NONE',  ( -10.81189881249999729, 1.324075727343319199E-15, -57.78125000204836681 ) ) ;
#3323=VECTOR ( 'NONE', #37906, 1000.000000000000000 ) ;
#3328=CARTESIAN_POINT ( 'NONE',  ( 10.00000000000000000, 5.773502691896255534, -131.2500000040967905 ) ) ;
#3334=ORIENTED_EDGE ( 'NONE', *, *, #11748, .T. ) ;
#3341=CARTESIAN_POINT ( 'NONE',  ( -2.121150477449813534E-15, -11.54700538379251284, -29.37499999999995381 ) ) ;
#3344=CARTESIAN_POINT ( 'NONE',  ( -5.405949406249996869, 9.363379034771805109, -152.3437500020483810 ) ) ;
#3345=CARTESIAN_POINT ( 'NONE',  ( -10.81189881249999729, -6.242252689847864744, -162.4687500020483526 ) ) ;
#3348=CARTESIAN_POINT ( 'NONE',  ( 5.000000000000000000, 8.660254037844385522, -189.2500000000000000 ) ) ;
#3353=CARTESIAN_POINT ( 'NONE',  ( -5.405949406249996869, 9.363379034771805109, -185.3437500020483810 ) ) ;
#3356=CARTESIAN_POINT ( 'NONE',  ( -10.81189881249999729, 6.242252689847871849, -59.40625000204838813 ) ) ;
#3358=CARTESIAN_POINT ( 'NONE',  ( 9.999999999999998224, 0.000000000000000000, -115.9999999999999858 ) ) ;
#3360=CARTESIAN_POINT ( 'NONE',  ( 5.405949406249999534, 9.363379034771803333, -140.7812500020483810 ) ) ;
#3361=CARTESIAN_POINT ( 'NONE',  ( -10.81189881249999729, 1.324075727343319199E-15, -156.7812500020484094 ) ) ;
#3363=CARTESIAN_POINT ( 'NONE',  ( 0.000000000000000000, 0.000000000000000000, -99.99999999999998579 ) ) ;
#3364=CARTESIAN_POINT ( 'NONE',  ( -5.405949406250003975, -9.363379034771801557, -93.34375000204838102 ) ) ;
#3367=CARTESIAN_POINT ( 'NONE',  ( -10.81189881249999907, -6.242252689847864744, -190.9687500020484379 ) ) ;
#3370=CARTESIAN_POINT ( 'NONE',  ( -5.405949406250003975, -9.363379034771801557, -86.03125000204838102 ) ) ;
#3372=CARTESIAN_POINT ( 'NONE',  ( 4.999999999999992006, -8.660254037844389075, -59.62500000409676204 ) ) ;
#3373=CARTESIAN_POINT ( 'NONE',  ( -10.81189881249999729, 6.242252689847871849, -15.71875000204836503 ) ) ;
#3376=CARTESIAN_POINT ( 'NONE',  ( 10.81189881249999551, -6.242252689847874514, -15.15625000204837036 ) ) ;
#3379=CARTESIAN_POINT ( 'NONE',  ( 9.999999999999998224, 0.000000000000000000, -156.5000000000000000 ) ) ;
#3380=CARTESIAN_POINT ( 'NONE',  ( 9.999999999999998224, 0.000000000000000000, -134.3750000040967905 ) ) ;
#3400=CARTESIAN_POINT ( 'NONE',  ( 5.405949406249999534, 9.363379034771803333, -157.2812500020484094 ) ) ;
#3402=CARTESIAN_POINT ( 'NONE',  ( -9.999999999999998224, 1.224646799147353059E-15, -121.2500000000000000 ) ) ;
#3406=CARTESIAN_POINT ( 'NONE',  ( 10.81189881249999729, 0.000000000000000000, -74.84375000204838102 ) ) ;
#3407=CARTESIAN_POINT ( 'NONE',  ( 5.405949406249992428, -9.363379034771808662, -87.28125000204838102 ) ) ;
#3410=CARTESIAN_POINT ( 'NONE',  ( -5.405949406249996869, 9.363379034771805109, -163.0312500020484094 ) ) ;
#3411=CARTESIAN_POINT ( 'NONE',  ( -10.81189881249999729, 6.242252689847871849, -183.9062500020484094 ) ) ;
#3412=CARTESIAN_POINT ( 'NONE',  ( 7.070501591499377789E-16, 11.54700538379251284, -158.0000000040968189 ) ) ;
#3413=DIRECTION ( 'NONE',  ( -0.000000000000000000, -0.000000000000000000, -1.000000000000000000 ) ) ;
#3414=CARTESIAN_POINT ( 'NONE',  ( 5.405949406249992428, -9.363379034771808662, -7.593750002048343717 ) ) ;
#3415=DIRECTION ( 'NONE',  ( -0.000000000000000000, -0.000000000000000000, -1.000000000000000000 ) ) ;
#3416=CARTESIAN_POINT ( 'NONE',  ( -2.293366432827344421E-15, -12.48450537969573659, -114.2187500020483668 ) ) ;
#3418=CARTESIAN_POINT ( 'NONE',  ( 10.81189881249999551, -6.242252689847874514, -12.15625000204836859 ) ) ;
#3421=CARTESIAN_POINT ( 'NONE',  ( 7.644554776091147741E-16, 12.48450537969573659, -109.1562500020483810 ) ) ;
#3424=CARTESIAN_POINT ( 'NONE',  ( -5.000000000000003553, -8.660254037844383745, -85.37500000409677625 ) ) ;
#3425=CARTESIAN_POINT ( 'NONE',  ( -5.000000000000003553, -8.660254037844383745, -140.8750000040967905 ) ) ;
#3426=CARTESIAN_POINT ( 'NONE',  ( -5.405949406250003975, -9.363379034771801557, -39.34375000204837391 ) ) ;
#3432=CARTESIAN_POINT ( 'NONE',  ( 4.999999999999992006, -8.660254037844389075, -8.625000004096744277 ) ) ;
#3433=AXIS2_PLACEMENT_3D ( 'NONE', #8938, #6125, #25770 ) ;
#3446=CARTESIAN_POINT ( 'NONE',  ( 10.81189881249999551, -6.242252689847874514, -181.6562500020484379 ) ) ;
#3447=CARTESIAN_POINT ( 'NONE',  ( 9.999999999999998224, 0.000000000000000000, -146.3750000040967905 ) ) ;
#3450=CARTESIAN_POINT ( 'NONE',  ( 5.405949406249999534, 9.363379034771803333, -100.0937500020483810 ) ) ;
#3452=CARTESIAN_POINT ( 'NONE',  ( 7.644554776091147741E-16, 12.48450537969573659, -107.6562500020483810 ) ) ;
#3454=CARTESIAN_POINT ( 'NONE',  ( 5.405949406249999534, 9.363379034771803333, -112.0937500020483810 ) ) ;
#3456=( BOUNDED_CURVE ( )  B_SPLINE_CURVE ( 2, ( #26183, #26393, #32245, #6121, #39544, #36104, #2885 ),
 .UNSPECIFIED., .F., .F. ) 
 B_SPLINE_CURVE_WITH_KNOTS ( ( 3, 2, 2, 3 ),
 ( 0.1231343283582089221, 0.1243781094527362935, 0.1256218905472636649, 0.1268656716417910224 ),
 .UNSPECIFIED. ) 
 CURVE ( )  GEOMETRIC_REPRESENTATION_ITEM ( )  RATIONAL_B_SPLINE_CURVE ( ( 1.000000000000002887, 0.8660254037844355990, 1.000000000000000000, 0.8660254037844387076, 1.000000000000000000, 0.8660254037844417052, 0.9999999999999970024 ) ) 
 REPRESENTATION_ITEM ( '' )  );
#3458=CARTESIAN_POINT ( 'NONE',  ( -1.119103713019287571, 10.75960476264953769, -99.99999999999997158 ) ) ;
#3459=CARTESIAN_POINT ( 'NONE',  ( 4.999999999999992006, -8.660254037844389075, -131.2499999999999716 ) ) ;
#3460=CARTESIAN_POINT ( 'NONE',  ( 5.000000000000000000, 8.660254037844385522, -1.749999999999973799 ) ) ;
#3463=CARTESIAN_POINT ( 'NONE',  ( -10.00000000000000000, -5.773502691896251982, -183.0000000040967905 ) ) ;
#3465=CARTESIAN_POINT ( 'NONE',  ( 10.81189881249999907, 6.242252689847868297, -31.21875000204835260 ) ) ;
#3467=CARTESIAN_POINT ( 'NONE',  ( -5.405949406250003975, -9.363379034771801557, -138.3437500020484094 ) ) ;
#3469=CARTESIAN_POINT ( 'NONE',  ( 10.81189881249999729, 0.000000000000000000, -33.03125000204837391 ) ) ;
#3471=CARTESIAN_POINT ( 'NONE',  ( 4.999999999999992006, -8.660254037844389075, -68.24999999999997158 ) ) ;
#3472=CARTESIAN_POINT ( 'NONE',  ( 5.405949406249992428, -9.363379034771808662, -130.7812500020483810 ) ) ;
#3475=CARTESIAN_POINT ( 'NONE',  ( -9.999999999999227285, -5.773502691896698735, -128.6249999999999716 ) ) ;
#3476=CARTESIAN_POINT ( 'NONE',  ( 9.999999999999996447, -5.773502691896262640, -109.0000000040967763 ) ) ;
#3478=CARTESIAN_POINT ( 'NONE',  ( -2.293366432827344421E-15, -12.48450537969573659, -69.21875000204839523 ) ) ;
#3479=EDGE_LOOP ( 'NONE', ( #37947, #38840, #19933, #6103 ) ) ;
#3484=CARTESIAN_POINT ( 'NONE',  ( 9.999999999999998224, 0.000000000000000000, -38.37500000409676915 ) ) ;
#3485=FACE_OUTER_BOUND ( 'NONE', #38048, .T. ) ;
#3489=VERTEX_POINT ( 'NONE', #39776 ) ;
#3495=DIRECTION ( 'NONE',  ( -0.000000000000000000, -0.000000000000000000, -1.000000000000000000 ) ) ;
#3501=CARTESIAN_POINT ( 'NONE',  ( -5.405949406249996869, 9.363379034771805109, -125.3437500020483952 ) ) ;
#3502=CARTESIAN_POINT ( 'NONE',  ( -10.81189881249999907, -6.242252689847864744, -134.1562500020483810 ) ) ;
#3504=CARTESIAN_POINT ( 'NONE',  ( -5.405949406249996869, 9.363379034771805109, -137.3437500020484094 ) ) ;
#3505=EDGE_CURVE ( 'NONE', #20876, #17374, #37182, .T. ) ;
#3506=FACE_OUTER_BOUND ( 'NONE', #9648, .T. ) ;
#3508=CARTESIAN_POINT ( 'NONE',  ( -9.999999999999998224, 5.773502691896259087, -160.3749999999999716 ) ) ;
#3513=CARTESIAN_POINT ( 'NONE',  ( 10.81189881249999551, -6.242252689847874514, -55.46875000204837391 ) ) ;
#3515=CARTESIAN_POINT ( 'NONE',  ( 5.405949406249992428, -9.363379034771808662, -165.0937500020484094 ) ) ;
#3521=CARTESIAN_POINT ( 'NONE',  ( 9.999999999999996447, -5.773502691896262640, -90.62499999999998579 ) ) ;
#3523=CARTESIAN_POINT ( 'NONE',  ( -5.405949406250003975, -9.363379034771801557, -111.5312500020483810 ) ) ;
#3524=CARTESIAN_POINT ( 'NONE',  ( -5.000000000000003553, -8.660254037844383745, -133.3750000040967905 ) ) ;
#3530=CARTESIAN_POINT ( 'NONE',  ( 10.81189881249999551, -6.242252689847874514, -52.65625000204837391 ) ) ;
#3533=EDGE_CURVE ( 'NONE', #28805, #3574, #7624, .T. ) ;
#3554=CARTESIAN_POINT ( 'NONE',  ( -9.999999999999998224, 5.773502691896259087, -29.87499999999995737 ) ) ;
#3557=CARTESIAN_POINT ( 'NONE',  ( 5.405949406249999534, 9.363379034771803333, -146.5937500020483810 ) ) ;
#3558=CARTESIAN_POINT ( 'NONE',  ( -2.293366432827344421E-15, -12.48450537969573659, -160.7187500020483810 ) ) ;
#3560=CARTESIAN_POINT ( 'NONE',  ( -9.999999999999998224, 0.000000000000000000, -99.99999999999998579 ) ) ;
#3562=CARTESIAN_POINT ( 'NONE',  ( -4.999999999999996447, 8.660254037844387298, -184.5000000000000000 ) ) ;
#3564=CARTESIAN_POINT ( 'NONE',  ( 9.999999999999998224, 0.000000000000000000, -167.3750000040967905 ) ) ;
#3566=FACE_OUTER_BOUND ( 'NONE', #31635, .T. ) ;
#3567=CARTESIAN_POINT ( 'NONE',  ( -10.81189881249999729, 6.242252689847871849, -189.7187500020484379 ) ) ;
#3570=CARTESIAN_POINT ( 'NONE',  ( -5.405949406250003975, -9.363379034771801557, -54.53125000204836681 ) ) ;
#3572=CARTESIAN_POINT ( 'NONE',  ( 4.999999999999992006, -8.660254037844389075, -113.2499999999999858 ) ) ;
#3574=VERTEX_POINT ( 'NONE', #31157 ) ;
#3575=CARTESIAN_POINT ( 'NONE',  ( 10.81189881249999551, -6.242252689847874514, -135.1562500020483810 ) ) ;
#3576=CARTESIAN_POINT ( 'NONE',  ( 5.405949406249992428, -9.363379034771808662, -147.2812500020483810 ) ) ;
#3580=CARTESIAN_POINT ( 'NONE',  ( 5.405949406249999534, 9.363379034771803333, -85.09375000204836681 ) ) ;
#3583=CARTESIAN_POINT ( 'NONE',  ( -2.293366432827344421E-15, -12.48450537969573659, -180.2187500020484094 ) ) ;
#3585=CARTESIAN_POINT ( 'NONE',  ( 9.999999999999994671, -5.773502691896262640, -171.6250000000000000 ) ) ;
#3587=CARTESIAN_POINT ( 'NONE',  ( 7.644554776091147741E-16, 12.48450537969573659, -80.65625000204839523 ) ) ;
#3589=( BOUNDED_CURVE ( )  B_SPLINE_CURVE ( 2, ( #41800, #42435, #12442, #35568, #35355, #42223, #21753 ),
 .UNSPECIFIED., .F., .F. ) 
 B_SPLINE_CURVE_WITH_KNOTS ( ( 3, 2, 2, 3 ),
 ( 0.4104477611940299253, 0.4116915422885572551, 0.4129353233830846959, 0.4141791044776120256 ),
 .UNSPECIFIED. ) 
 CURVE ( )  GEOMETRIC_REPRESENTATION_ITEM ( )  RATIONAL_B_SPLINE_CURVE ( ( 0.9999999999999940048, 0.8660254037844447028, 1.000000000000000000, 0.8660254037844387076, 1.000000000000000000, 0.8660254037844267172, 1.000000000000011990 ) ) 
 REPRESENTATION_ITEM ( '' )  );
#3591=CARTESIAN_POINT ( 'NONE',  ( -5.000000000000003553, -8.660254037844383745, -56.87500000409676204 ) ) ;
#3592=CARTESIAN_POINT ( 'NONE',  ( -2.293366432827344421E-15, -12.48450537969573659, -7.718750002048357040 ) ) ;
#3593=CARTESIAN_POINT ( 'NONE',  ( -2.121150477449813534E-15, -11.54700538379251284, -137.7500000040967905 ) ) ;
#3596=CARTESIAN_POINT ( 'NONE',  ( 10.81189881249999551, -6.242252689847874514, -13.65625000204837036 ) ) ;
#3600=CARTESIAN_POINT ( 'NONE',  ( -4.999999999999996447, 8.660254037844387298, -177.3750000040967905 ) ) ;
#3601=( BOUNDED_CURVE ( )  B_SPLINE_CURVE ( 2, ( #35125, #20928, #2535, #15454, #21945, #12217, #25409 ),
 .UNSPECIFIED., .F., .F. ) 
 B_SPLINE_CURVE_WITH_KNOTS ( ( 3, 2, 2, 3 ),
 ( 0.2723880597014926574, 0.2736318407960199872, 0.2748756218905473725, 0.2761194029850747578 ),
 .UNSPECIFIED. ) 
 CURVE ( )  GEOMETRIC_REPRESENTATION_ITEM ( )  RATIONAL_B_SPLINE_CURVE ( ( 0.9999999999999880096, 0.8660254037844506980, 1.000000000000000000, 0.8660254037844387076, 1.000000000000000000, 0.8660254037844267172, 1.000000000000011990 ) ) 
 REPRESENTATION_ITEM ( '' )  );
#3620=CARTESIAN_POINT ( 'NONE',  ( 5.405949406249992428, -9.363379034771808662, -148.7812500020483810 ) ) ;
#3625=LINE ( 'NONE', #13933, #25268 ) ;
#3628=CARTESIAN_POINT ( 'NONE',  ( -10.81189881249999729, 1.324075727343319199E-15, -68.09375000204836681 ) ) ;
#3629=CARTESIAN_POINT ( 'NONE',  ( -5.405949406250003975, -9.363379034771801557, -75.53125000204838102 ) ) ;
#3631=CYLINDRICAL_SURFACE ( 'NONE', #11668, 9.999999999999998224 ) ;
#3632=CARTESIAN_POINT ( 'NONE',  ( -10.81189881249999729, 6.242252689847871849, -161.4062500020483810 ) ) ;
#3633=CARTESIAN_POINT ( 'NONE',  ( -5.405949406250003975, -9.363379034771801557, -168.5312500020484094 ) ) ;
#3635=CARTESIAN_POINT ( 'NONE',  ( 0.000000000000000000, 0.000000000000000000, -99.99999999999998579 ) ) ;
#3636=CARTESIAN_POINT ( 'NONE',  ( 5.405949406249999534, 9.363379034771803333, -2.593750002048367254 ) ) ;
#3637=LINE ( 'NONE', #20229, #24071 ) ;
#3638=CARTESIAN_POINT ( 'NONE',  ( -5.405949406250003975, -9.363379034771801557, -105.3437500020483810 ) ) ;
#3640=CARTESIAN_POINT ( 'NONE',  ( -10.81189881249999729, 6.242252689847871849, -9.906250002048366810 ) ) ;
#3642=CARTESIAN_POINT ( 'NONE',  ( -5.000000000000003553, -8.660254037844383745, -133.3750000040967905 ) ) ;
#3643=CARTESIAN_POINT ( 'NONE',  ( 10.81189881249999551, -6.242252689847874514, -106.6562500020483952 ) ) ;
#3646=CARTESIAN_POINT ( 'NONE',  ( -2.121150477449813534E-15, -11.54700538379251284, -85.25000000409676204 ) ) ;
#3647=CARTESIAN_POINT ( 'NONE',  ( -9.999999999999479527, -5.773502691896549521, -141.0000000040967620 ) ) ;
#3648=CARTESIAN_POINT ( 'NONE',  ( 5.405949406249999534, 9.363379034771803333, -43.09375000204837391 ) ) ;
#3649=ORIENTED_EDGE ( 'NONE', *, *, #30246, .F. ) ;
#3653=CARTESIAN_POINT ( 'NONE',  ( -9.999999999999998224, 5.773502691896259087, -10.75000000409676026 ) ) ;
#3654=EDGE_CURVE ( 'NONE', #9895, #13418, #3294, .T. ) ;
#3658=ORIENTED_EDGE ( 'NONE', *, *, #13010, .T. ) ;
#3664=ORIENTED_EDGE ( 'NONE', *, *, #20347, .T. ) ;
#3666=CARTESIAN_POINT ( 'NONE',  ( 5.000000000000000000, 8.660254037844385522, -128.1250000040967620 ) ) ;
#3667=CARTESIAN_POINT ( 'NONE',  ( 5.405949406249999534, 9.363379034771803333, -173.7812500020484094 ) ) ;
#3671=CARTESIAN_POINT ( 'NONE',  ( 10.81189881249999551, -6.242252689847874514, -104.9687500020483810 ) ) ;
#3673=CARTESIAN_POINT ( 'NONE',  ( 5.405949406249999534, 9.363379034771803333, -104.7812500020483810 ) ) ;
#3675=CARTESIAN_POINT ( 'NONE',  ( -10.81189881249999729, -6.242252689847864744, -114.4687500020483810 ) ) ;
#3680=CARTESIAN_POINT ( 'NONE',  ( -2.121150477449813534E-15, -11.54700538379251284, -2.374999999999960920 ) ) ;
#3683=CARTESIAN_POINT ( 'NONE',  ( 10.00000000000000000, 5.773502691896255534, -183.7500000040968189 ) ) ;
#3685=CARTESIAN_POINT ( 'NONE',  ( 5.405949406249992428, -9.363379034771808662, -27.09375000204835970 ) ) ;
#3687=CARTESIAN_POINT ( 'NONE',  ( -10.81189881249999907, -6.242252689847864744, -141.4687500020484094 ) ) ;
#3689=CARTESIAN_POINT ( 'NONE',  ( 7.644554776091147741E-16, 12.48450537969573659, -37.15625000204836681 ) ) ;
#3690=CARTESIAN_POINT ( 'NONE',  ( 9.999999999999227285, 5.773502691896701400, -111.3749999999999432 ) ) ;
#3691=CARTESIAN_POINT ( 'NONE',  ( -10.00000000000000000, -5.773502691896251982, -58.12499999999997868 ) ) ;
#3692=CARTESIAN_POINT ( 'NONE',  ( 7.644554776091147741E-16, 12.48450537969573659, -128.6562500020483810 ) ) ;
#3695=CARTESIAN_POINT ( 'NONE',  ( 4.999999999999992006, -8.660254037844389075, -131.2499999999999716 ) ) ;
#3696=CARTESIAN_POINT ( 'NONE',  ( 5.000000000000000000, 8.660254037844385522, -105.6250000040967763 ) ) ;
#3698=CARTESIAN_POINT ( 'NONE',  ( 10.81189881249999551, -6.242252689847874514, -65.96875000204838102 ) ) ;
#3699=ORIENTED_EDGE ( 'NONE', *, *, #17219, .F. ) ;
#3704=CARTESIAN_POINT ( 'NONE',  ( -9.999999999999998224, 1.224646799147353059E-15, -33.12500000409676915 ) ) ;
#3705=DIRECTION ( 'NONE',  ( -1.000000000000000000, 0.000000000000000000, 0.000000000000000000 ) ) ;
#3712=CARTESIAN_POINT ( 'NONE',  ( 7.070501591499376803E-16, 11.54700538379251284, -126.5000000040967763 ) ) ;
#3716=CARTESIAN_POINT ( 'NONE',  ( -5.405949406249996869, 9.363379034771805109, -196.0312500020484094 ) ) ;
#3718=CARTESIAN_POINT ( 'NONE',  ( -10.00000000000051337, 5.773502691895962435, -144.2500000040967905 ) ) ;
#3722=CARTESIAN_POINT ( 'NONE',  ( 10.81189881249999907, 6.242252689847868297, -124.2187500020483952 ) ) ;
#3723=CARTESIAN_POINT ( 'NONE',  ( -10.81189881249999729, 6.242252689847871849, -131.4062500020484094 ) ) ;
#3725=CARTESIAN_POINT ( 'NONE',  ( 7.644554776091147741E-16, 12.48450537969573659, -135.9687500020483810 ) ) ;
#3728=CARTESIAN_POINT ( 'NONE',  ( -4.999999999999996447, 8.660254037844387298, -153.0000000000000000 ) ) ;
#3733=CARTESIAN_POINT ( 'NONE',  ( -2.293366432827344421E-15, -12.48450537969573659, -57.21875000204836681 ) ) ;
#3735=CARTESIAN_POINT ( 'NONE',  ( -5.405949406250003975, -9.363379034771801557, -162.3437500020484094 ) ) ;
#3739=CARTESIAN_POINT ( 'NONE',  ( 4.999999999999992006, -8.660254037844389075, -83.24999999999997158 ) ) ;
#3740=EDGE_LOOP ( 'NONE', ( #29551, #84, #2315, #31538 ) ) ;
#3741=CARTESIAN_POINT ( 'NONE',  ( -5.405949406250003975, -9.363379034771801557, -108.5312500020483810 ) ) ;
#3742=CARTESIAN_POINT ( 'NONE',  ( -9.999999999999998224, 5.773502691896259087, -135.2500000040967905 ) ) ;
#3747=CARTESIAN_POINT ( 'NONE',  ( 10.81189881249999729, 0.000000000000000000, -52.53125000204835970 ) ) ;
#3752=EDGE_CURVE ( 'NONE', #37078, #21806, #1412, .T. ) ;
#3755=CARTESIAN_POINT ( 'NONE',  ( -10.00000000000102496, 5.773502691895664007, -130.7500000040967620 ) ) ;
#3764=DIRECTION ( 'NONE',  ( -1.000000000000000000, 0.000000000000000000, 0.000000000000000000 ) ) ;
#3768=CARTESIAN_POINT ( 'NONE',  ( -10.81189881249999729, 1.324075727343319199E-15, -146.0937500020483810 ) ) ;
#3769=CARTESIAN_POINT ( 'NONE',  ( 7.644554776091147741E-16, 12.48450537969573659, -162.9687500020483810 ) ) ;
#3772=CARTESIAN_POINT ( 'NONE',  ( 9.999999999999996447, -5.773502691896262640, -182.1250000000000000 ) ) ;
#3776=CARTESIAN_POINT ( 'NONE',  ( 10.81189881249999907, 6.242252689847868297, -188.7187500020484094 ) ) ;
#3780=CARTESIAN_POINT ( 'NONE',  ( 10.81189881249999907, 6.242252689847868297, -53.90625000204838102 ) ) ;
#3782=CARTESIAN_POINT ( 'NONE',  ( 9.999999999999996447, -5.773502691896262640, -119.1249999999999858 ) ) ;
#3785=CARTESIAN_POINT ( 'NONE',  ( -2.293366432827344421E-15, -12.48450537969573659, -132.4062500020483810 ) ) ;
#3786=CARTESIAN_POINT ( 'NONE',  ( -10.81189881249999729, 6.242252689847871849, -144.9062500020484094 ) ) ;
#3788=CARTESIAN_POINT ( 'NONE',  ( 4.999999999999992006, -8.660254037844389075, -125.2500000000000000 ) ) ;
#3789=CARTESIAN_POINT ( 'NONE',  ( -5.405949406249996869, 9.363379034771805109, -80.34375000204838102 ) ) ;
#3790=VERTEX_POINT ( 'NONE', #25322 ) ;
#3792=CARTESIAN_POINT ( 'NONE',  ( 10.81189881249999729, 0.000000000000000000, -176.8437500020483810 ) ) ;
#3795=CARTESIAN_POINT ( 'NONE',  ( -9.999999999999998224, 1.224646799147353059E-15, -135.1250000040967620 ) ) ;
#3796=CARTESIAN_POINT ( 'NONE',  ( -10.81189881249999907, -6.242252689847864744, -74.15625000204835260 ) ) ;
#3798=CARTESIAN_POINT ( 'NONE',  ( 4.999999999999992006, -8.660254037844389075, -55.12500000409675494 ) ) ;
#3799=CARTESIAN_POINT ( 'NONE',  ( 10.81189881249999907, 6.242252689847868297, -11.71875000204836148 ) ) ;
#3801=CARTESIAN_POINT ( 'NONE',  ( 10.81189881249999729, 0.000000000000000000, -6.031250002048377468 ) ) ;
#3810=ADVANCED_FACE ( 'NONE', ( #1804 ), #25535, .F. ) ;
#3813=CARTESIAN_POINT ( 'NONE',  ( -9.999999999999742428, -5.773502691896402084, -160.5000000040968189 ) ) ;
#3814=CARTESIAN_POINT ( 'NONE',  ( -10.81189881249999729, 1.324075727343319199E-15, -102.5937500020483810 ) ) ;
#3821=CARTESIAN_POINT ( 'NONE',  ( -9.999999999999998224, 0.000000000000000000, -99.99999999999998579 ) ) ;
#3822=CARTESIAN_POINT ( 'NONE',  ( -9.999999999999998224, 5.773502691896259087, -43.37499999999997158 ) ) ;
#3826=EDGE_CURVE ( 'NONE', #8327, #39928, #26234, .T. ) ;
#3828=CARTESIAN_POINT ( 'NONE',  ( 0.000000000000000000, 0.000000000000000000, -180.0000000000000000 ) ) ;
#3829=CARTESIAN_POINT ( 'NONE',  ( 10.81189881249999551, -6.242252689847874514, -145.6562500020484094 ) ) ;
#3833=CARTESIAN_POINT ( 'NONE',  ( -4.999999999999996447, 8.660254037844387298, -141.0000000000000000 ) ) ;
#3836=CARTESIAN_POINT ( 'NONE',  ( -5.405949406249996869, 9.363379034771805109, -72.84375000204838102 ) ) ;
#3838=CARTESIAN_POINT ( 'NONE',  ( -5.405949406250003975, -9.363379034771801557, -74.03125000204838102 ) ) ;
#3841=CARTESIAN_POINT ( 'NONE',  ( -5.405949406249996869, 9.363379034771805109, -157.0312500020484094 ) ) ;
#3842=CARTESIAN_POINT ( 'NONE',  ( 5.405949406249999534, 9.363379034771803333, -172.2812500020484094 ) ) ;
#3845=CARTESIAN_POINT ( 'NONE',  ( 10.81189881249999729, 0.000000000000000000, -109.3437500020483810 ) ) ;
#3847=CARTESIAN_POINT ( 'NONE',  ( 7.644554776091147741E-16, 12.48450537969573659, -4.156250002048361480 ) ) ;
#3850=CARTESIAN_POINT ( 'NONE',  ( -5.000000000000003553, -8.660254037844383745, -169.0000000000000000 ) ) ;
#3851=CARTESIAN_POINT ( 'NONE',  ( -10.81189881249999907, -6.242252689847864744, -96.65625000204839523 ) ) ;
#3854=CARTESIAN_POINT ( 'NONE',  ( -4.999999999999996447, 8.660254037844387298, -78.37500000409677625 ) ) ;
#3855=CARTESIAN_POINT ( 'NONE',  ( 9.999999999999998224, 0.000000000000000000, -140.3750000040967905 ) ) ;
#3856=CARTESIAN_POINT ( 'NONE',  ( -5.405949406250003975, -9.363379034771801557, -34.84375000204836681 ) ) ;
#3859=CARTESIAN_POINT ( 'NONE',  ( 10.81189881249999729, 0.000000000000000000, -34.53125000204837391 ) ) ;
#3861=DIRECTION ( 'NONE',  ( -0.000000000000000000, -0.000000000000000000, -1.000000000000000000 ) ) ;
#3862=CARTESIAN_POINT ( 'NONE',  ( 4.999999999999992006, -8.660254037844389075, -10.12500000409674605 ) ) ;
#3865=APPLICATION_CONTEXT ( 'configuration controlled 3d designs of mechanical parts and assemblies' ) ;
#3870=ORIENTED_EDGE ( 'NONE', *, *, #21602, .F. ) ;
#3876=ORIENTED_EDGE ( 'NONE', *, *, #22021, .T. ) ;
#3880=CARTESIAN_POINT ( 'NONE',  ( -2.293366432827344421E-15, -12.48450537969573659, -172.9062500020484379 ) ) ;
#3881=DIRECTION ( 'NONE',  ( -1.000000000000000000, 0.000000000000000000, 0.000000000000000000 ) ) ;
#3883=CARTESIAN_POINT ( 'NONE',  ( 10.81189881249999729, 0.000000000000000000, -89.84375000204838102 ) ) ;
#3884=CARTESIAN_POINT ( 'NONE',  ( 10.81189881249999907, 6.242252689847868297, -101.9062500020484094 ) ) ;
#3886=CARTESIAN_POINT ( 'NONE',  ( 10.81189881249999729, 0.000000000000000000, -110.8437500020483810 ) ) ;
#3890=CARTESIAN_POINT ( 'NONE',  ( -5.405949406250003975, -9.363379034771801557, -195.5312500020484094 ) ) ;
#3893=CARTESIAN_POINT ( 'NONE',  ( 7.070501591499377789E-16, 11.54700538379251284, -170.0000000040967905 ) ) ;
#3895=CARTESIAN_POINT ( 'NONE',  ( 5.405949406249992428, -9.363379034771808662, -24.09375000204835970 ) ) ;
#3896=DIRECTION ( 'NONE',  ( -1.000000000000000000, 0.000000000000000000, 0.000000000000000000 ) ) ;
#3897=CARTESIAN_POINT ( 'NONE',  ( -10.81189881249999907, -6.242252689847864744, -126.4687500020483810 ) ) ;
#3899=CARTESIAN_POINT ( 'NONE',  ( 10.81189881249999729, 0.000000000000000000, -27.03125000204836681 ) ) ;
#3902=CARTESIAN_POINT ( 'NONE',  ( -2.121150477449813534E-15, -11.54700538379251284, -62.37499999999998579 ) ) ;
#3903=CARTESIAN_POINT ( 'NONE',  ( 10.81189881249999551, -6.242252689847874514, -127.6562500020483952 ) ) ;
#3905=ORIENTED_EDGE ( 'NONE', *, *, #24377, .T. ) ;
#3906=CARTESIAN_POINT ( 'NONE',  ( 10.00000000000025402, -5.773502691896113426, -131.1250000000000000 ) ) ;
#3907=CARTESIAN_POINT ( 'NONE',  ( -5.000000000000003553, -8.660254037844383745, -104.8750000040967763 ) ) ;
#3909=CARTESIAN_POINT ( 'NONE',  ( 10.81189881249999907, 6.242252689847868297, -58.21875000204838102 ) ) ;
#3913=DIRECTION ( 'NONE',  ( -1.000000000000000000, 0.000000000000000000, 0.000000000000000000 ) ) ;
#3914=CARTESIAN_POINT ( 'NONE',  ( 10.00000000000000000, 5.773502691896255534, -39.75000000409675494 ) ) ;
#3924=CARTESIAN_POINT ( 'NONE',  ( 5.405949406249999534, 9.363379034771803333, -194.7812500020484094 ) ) ;
#3926=DIRECTION ( 'NONE',  ( 0.000000000000000000, 0.000000000000000000, -1.000000000000000000 ) ) ;
#3930=CARTESIAN_POINT ( 'NONE',  ( -5.405949406249996869, 9.363379034771805109, -116.3437500020483810 ) ) ;
#3931=CARTESIAN_POINT ( 'NONE',  ( 4.999999999999992006, -8.660254037844389075, -193.1250000040967905 ) ) ;
#3932=CARTESIAN_POINT ( 'NONE',  ( -10.81189881249999907, -6.242252689847864744, -125.1562500020483810 ) ) ;
#3934=CARTESIAN_POINT ( 'NONE',  ( 5.405949406249992428, -9.363379034771808662, -138.0937500020483810 ) ) ;
#3937=CARTESIAN_POINT ( 'NONE',  ( 5.000000000000000000, 8.660254037844385522, -151.7500000000000000 ) ) ;
#3938=CARTESIAN_POINT ( 'NONE',  ( 5.000000000000000000, 8.660254037844385522, -24.24999999999996447 ) ) ;
#3942=CARTESIAN_POINT ( 'NONE',  ( 5.405949406249999534, 9.363379034771803333, -50.59375000204835260 ) ) ;
#3944=CARTESIAN_POINT ( 'NONE',  ( 10.81189881249999551, -6.242252689847874514, -152.9687500020484094 ) ) ;
#3948=CARTESIAN_POINT ( 'NONE',  ( -10.00000000000000000, -5.773502691896251982, -85.12499999999997158 ) ) ;
#3951=CARTESIAN_POINT ( 'NONE',  ( -2.293366432827344421E-15, -12.48450537969573659, -109.9062500020483810 ) ) ;
#3952=CARTESIAN_POINT ( 'NONE',  ( 9.999999999999996447, -5.773502691896262640, -133.0000000040967905 ) ) ;
#3956=CARTESIAN_POINT ( 'NONE',  ( -5.405949406249996869, 9.363379034771805109, -52.03125000204835970 ) ) ;
#3963=( BOUNDED_CURVE ( )  B_SPLINE_CURVE ( 2, ( #11981, #5308, #1870, #14996, #28195, #41328, #24967 ),
 .UNSPECIFIED., .F., .F. ) 
 B_SPLINE_CURVE_WITH_KNOTS ( ( 3, 2, 2, 3 ),
 ( 0.4328358208955225273, 0.4340796019900499125, 0.4353233830845772978, 0.4365671641791046276 ),
 .UNSPECIFIED. ) 
 CURVE ( )  GEOMETRIC_REPRESENTATION_ITEM ( )  RATIONAL_B_SPLINE_CURVE ( ( 0.9999999999999820144, 0.8660254037844566932, 1.000000000000000000, 0.8660254037844387076, 1.000000000000000000, 0.8660254037844207220, 1.000000000000017986 ) ) 
 REPRESENTATION_ITEM ( '' )  );
#3977=CARTESIAN_POINT ( 'NONE',  ( 5.405949406249992428, -9.363379034771808662, -144.0937500020483810 ) ) ;
#3978=CARTESIAN_POINT ( 'NONE',  ( -5.405949406249996869, 9.363379034771805109, -159.8437500020484094 ) ) ;
#3980=CARTESIAN_POINT ( 'NONE',  ( 10.00000000000000000, 5.773502691896255534, -178.8750000000000000 ) ) ;
#3983=FACE_OUTER_BOUND ( 'NONE', #8521, .T. ) ;
#3985=CARTESIAN_POINT ( 'NONE',  ( -10.81189881249999729, 6.242252689847871849, -185.2187500020483810 ) ) ;
#3988=CARTESIAN_POINT ( 'NONE',  ( -5.405949406249996869, 9.363379034771805109, -49.03125000204838813 ) ) ;
#3990=CARTESIAN_POINT ( 'NONE',  ( -4.999999999999996447, 8.660254037844387298, -106.4999999999999858 ) ) ;
#3992=CARTESIAN_POINT ( 'NONE',  ( 10.81189881249999729, 0.000000000000000000, -130.5312500020484094 ) ) ;
#3993=CARTESIAN_POINT ( 'NONE',  ( -10.81189881249999907, -6.242252689847864744, -149.1562500020483810 ) ) ;
#3995=CARTESIAN_POINT ( 'NONE',  ( 7.644554776091147741E-16, 12.48450537969573659, -78.96875000204839523 ) ) ;
#3997=ORIENTED_EDGE ( 'NONE', *, *, #41197, .F. ) ;
#3999=CARTESIAN_POINT ( 'NONE',  ( 5.405949406249992428, -9.363379034771808662, -180.0937500020484094 ) ) ;
#4001=VECTOR ( 'NONE', #14838, 1000.000000000000000 ) ;
#4003=CARTESIAN_POINT ( 'NONE',  ( -10.81189881249999729, 6.242252689847871849, -78.90625000204838102 ) ) ;
#4005=CARTESIAN_POINT ( 'NONE',  ( -9.999999999999998224, 1.224646799147353059E-15, -49.62500000409675494 ) ) ;
#4006=CARTESIAN_POINT ( 'NONE',  ( -5.405949406249996869, 9.363379034771805109, -12.84375000204834905 ) ) ;
#4007=CARTESIAN_POINT ( 'NONE',  ( 0.000000000000000000, 0.000000000000000000, -99.99999999999998579 ) ) ;
#4009=CARTESIAN_POINT ( 'NONE',  ( -2.293366432827344421E-15, -12.48450537969573659, -6.406250002048363257 ) ) ;
#4011=CARTESIAN_POINT ( 'NONE',  ( 8.660254119780192994, -4.999999858083012505, -99.99999999999998579 ) ) ;
#4017=DIRECTION ( 'NONE',  ( -0.000000000000000000, -0.000000000000000000, -1.000000000000000000 ) ) ;
#4025=CARTESIAN_POINT ( 'NONE',  ( -2.121150477449813534E-15, -11.54700538379251284, -47.37499999999997868 ) ) ;
#4034=CARTESIAN_POINT ( 'NONE',  ( -10.00000000000025580, 5.773502691896109873, -160.7500000040967620 ) ) ;
#4038=CARTESIAN_POINT ( 'NONE',  ( -10.81189881249999729, 6.242252689847871849, -71.21875000204839523 ) ) ;
#4040=CARTESIAN_POINT ( 'NONE',  ( -10.81189881249999729, 1.324075727343319199E-15, -72.78125000204838102 ) ) ;
#4043=CARTESIAN_POINT ( 'NONE',  ( 7.644554776091147741E-16, 12.48450537969573659, -155.6562500020483810 ) ) ;
#4044=CARTESIAN_POINT ( 'NONE',  ( -2.293366432827344421E-15, -12.48450537969573659, -175.9062500020483810 ) ) ;
#4045=CARTESIAN_POINT ( 'NONE',  ( 5.405949406249992428, -9.363379034771808662, -0.09375000204836503315 ) ) ;
#4046=CARTESIAN_POINT ( 'NONE',  ( 0.000000000000000000, 0.000000000000000000, -99.99999999999998579 ) ) ;
#4047=CARTESIAN_POINT ( 'NONE',  ( 5.405949406249992428, -9.363379034771808662, -109.5937500020483810 ) ) ;
#4048=CARTESIAN_POINT ( 'NONE',  ( 9.999999999999612754, 5.773502691896477579, -156.3750000000000000 ) ) ;
#4050=CARTESIAN_POINT ( 'NONE',  ( 10.81189881249999907, 6.242252689847868297, -2.906250002048360592 ) ) ;
#4054=CARTESIAN_POINT ( 'NONE',  ( 10.81189881249999551, -6.242252689847874514, -102.1562500020483952 ) ) ;
#4056=CARTESIAN_POINT ( 'NONE',  ( 7.070501591499377789E-16, 11.54700538379251284, -80.00000000409679046 ) ) ;
#4058=CARTESIAN_POINT ( 'NONE',  ( -5.405949406249996869, 9.363379034771805109, -35.34375000204836681 ) ) ;
#4059=ORIENTED_EDGE ( 'NONE', *, *, #26989, .T. ) ;
#4061=CARTESIAN_POINT ( 'NONE',  ( 5.405949406249992428, -9.363379034771808662, -30.28125000204837036 ) ) ;
#4064=EDGE_CURVE ( 'NONE', #35407, #13549, #40830, .T. ) ;
#4065=CARTESIAN_POINT ( 'NONE',  ( -9.999999999999998224, 5.773502691896259087, -1.750000004096752271 ) ) ;
#4067=ADVANCED_FACE ( 'NONE', ( #29607 ), #6936, .F. ) ;
#4076=AXIS2_PLACEMENT_3D ( 'NONE', #21825, #35005, #15335 ) ;
#4085=( BOUNDED_CURVE ( )  B_SPLINE_CURVE ( 2, ( #10896, #20829, #24089, #17796, #40880, #21258, #4864 ),
 .UNSPECIFIED., .F., .F. ) 
 B_SPLINE_CURVE_WITH_KNOTS ( ( 3, 2, 2, 3 ),
 ( 0.2985074626865671932, 0.2997512437810946340, 0.3009950248756220192, 0.3022388059701494045 ),
 .UNSPECIFIED. ) 
 CURVE ( )  GEOMETRIC_REPRESENTATION_ITEM ( )  RATIONAL_B_SPLINE_CURVE ( ( 0.9999999999999940048, 0.8660254037844447028, 1.000000000000000000, 0.8660254037844387076, 1.000000000000000000, 0.8660254037844207220, 1.000000000000017986 ) ) 
 REPRESENTATION_ITEM ( '' )  );
#4086=CARTESIAN_POINT ( 'NONE',  ( 7.644554776091147741E-16, 12.48450537969573659, -175.1562500020484094 ) ) ;
#4089=CARTESIAN_POINT ( 'NONE',  ( 10.81189881249999729, 0.000000000000000000, -94.34375000204838102 ) ) ;
#4090=CARTESIAN_POINT ( 'NONE',  ( 10.81189881249999551, -6.242252689847874514, -102.1562500020483952 ) ) ;
#4092=CARTESIAN_POINT ( 'NONE',  ( -5.405949406249996869, 9.363379034771805109, -108.8437500020483810 ) ) ;
#4094=CARTESIAN_POINT ( 'NONE',  ( -5.000000000000003553, -8.660254037844383745, -104.8750000040967763 ) ) ;
#4096=CARTESIAN_POINT ( 'NONE',  ( 10.81189881249999551, -6.242252689847874514, -193.6562500020484379 ) ) ;
#4100=CARTESIAN_POINT ( 'NONE',  ( 4.999999999999992006, -8.660254037844389075, -173.6250000040968189 ) ) ;
#4102=CARTESIAN_POINT ( 'NONE',  ( -10.81189881249999729, 1.324075727343319199E-15, -23.09375000204835615 ) ) ;
#4103=LINE ( 'NONE', #26558, #25431 ) ;
#4104=CARTESIAN_POINT ( 'NONE',  ( 5.405949406249992428, -9.363379034771808662, -130.5937500020483810 ) ) ;
#4106=CARTESIAN_POINT ( 'NONE',  ( -2.293366432827344421E-15, -12.48450537969573659, -28.90625000204835615 ) ) ;
#4108=CARTESIAN_POINT ( 'NONE',  ( 9.999999999999998224, 0.000000000000000000, -57.49999999999996447 ) ) ;
#4109=CARTESIAN_POINT ( 'NONE',  ( 5.405949406249992428, -9.363379034771808662, -127.7812500020483810 ) ) ;
#4112=VECTOR ( 'NONE', #39758, 1000.000000000000000 ) ;
#4114=CARTESIAN_POINT ( 'NONE',  ( -10.00000000000000000, -5.773502691896251982, -102.0000000040967905 ) ) ;
#4116=CARTESIAN_POINT ( 'NONE',  ( 10.81189881249999907, 6.242252689847868297, -61.21875000204836681 ) ) ;
#4117=ORIENTED_EDGE ( 'NONE', *, *, #17760, .F. ) ;
#4119=EDGE_CURVE ( 'NONE', #36081, #32882, #42477, .T. ) ;
#4122=CARTESIAN_POINT ( 'NONE',  ( 9.999999999999998224, 0.000000000000000000, -26.37500000409676204 ) ) ;
#4124=DIRECTION ( 'NONE',  ( -1.000000000000000000, 0.000000000000000000, 0.000000000000000000 ) ) ;
#4126=VECTOR ( 'NONE', #34449, 1000.000000000000000 ) ;
#4131=CARTESIAN_POINT ( 'NONE',  ( 10.81189881249999907, 6.242252689847868297, -197.9062500020484379 ) ) ;
#4137=CARTESIAN_POINT ( 'NONE',  ( 10.81189881249999907, 6.242252689847868297, -118.2187500020483810 ) ) ;
#4138=CARTESIAN_POINT ( 'NONE',  ( 5.000000000000000000, 8.660254037844385522, -192.6250000040967905 ) ) ;
#4139=CARTESIAN_POINT ( 'NONE',  ( 10.81189881249999729, 0.000000000000000000, -121.5312500020483952 ) ) ;
#4141=CARTESIAN_POINT ( 'NONE',  ( 5.405949406249999534, 9.363379034771803333, -133.0937500020483810 ) ) ;
#4142=CARTESIAN_POINT ( 'NONE',  ( -9.999999999999998224, 1.224646799147353059E-15, -166.6250000040967905 ) ) ;
#4144=CARTESIAN_POINT ( 'NONE',  ( 5.000000000000000000, 8.660254037844385522, -153.2500000000000000 ) ) ;
#4145=CARTESIAN_POINT ( 'NONE',  ( 10.00000000000000000, 5.773502691896255534, -21.37499999999997868 ) ) ;
#4150=CARTESIAN_POINT ( 'NONE',  ( -2.293366432827344421E-15, -12.48450537969573659, -46.71875000204835970 ) ) ;
#4151=CARTESIAN_POINT ( 'NONE',  ( -9.999999999999479527, -5.773502691896549521, -142.1249999999999716 ) ) ;
#4152=CARTESIAN_POINT ( 'NONE',  ( -5.405949406249996869, 9.363379034771805109, -153.8437500020483810 ) ) ;
#4155=CARTESIAN_POINT ( 'NONE',  ( 7.070501591499377789E-16, 11.54700538379251284, -84.12499999999997158 ) ) ;
#4158=CARTESIAN_POINT ( 'NONE',  ( 10.81189881249999729, 0.000000000000000000, -114.0312500020483952 ) ) ;
#4159=CARTESIAN_POINT ( 'NONE',  ( -9.999999999999998224, 1.224646799147353059E-15, -127.6250000040967620 ) ) ;
#4160=CARTESIAN_POINT ( 'NONE',  ( -5.000000000000003553, -8.660254037844383745, -111.9999999999999858 ) ) ;
#4164=CARTESIAN_POINT ( 'NONE',  ( -5.405949406249996869, 9.363379034771805109, -53.53125000204836681 ) ) ;
#4168=CARTESIAN_POINT ( 'NONE',  ( -10.00000000000051337, 5.773502691895962435, -109.3749999999999858 ) ) ;
#4170=( BOUNDED_CURVE ( )  B_SPLINE_CURVE ( 2, ( #24476, #28942, #22035, #15951, #11493, #42287, #22452 ),
 .UNSPECIFIED., .F., .F. ) 
 B_SPLINE_CURVE_WITH_KNOTS ( ( 3, 2, 2, 3 ),
 ( 0.3320895522388061516, 0.3333333333333334259, 0.3345771144278607556, 0.3358208955223880854 ),
 .UNSPECIFIED. ) 
 CURVE ( )  GEOMETRIC_REPRESENTATION_ITEM ( )  RATIONAL_B_SPLINE_CURVE ( ( 0.9999999999999820144, 0.8660254037844566932, 1.000000000000000000, 0.8660254037844387076, 1.000000000000000000, 0.8660254037844387076, 1.000000000000000000 ) ) 
 REPRESENTATION_ITEM ( '' )  );
#4177=ORIENTED_EDGE ( 'NONE', *, *, #34029, .T. ) ;
#4183=VECTOR ( 'NONE', #17096, 1000.000000000000000 ) ;
#4186=CARTESIAN_POINT ( 'NONE',  ( 10.81189881249999729, 0.000000000000000000, -137.8437500020484094 ) ) ;
#4187=CARTESIAN_POINT ( 'NONE',  ( 7.644554776091147741E-16, 12.48450537969573659, -158.4687500020483810 ) ) ;
#4190=CARTESIAN_POINT ( 'NONE',  ( 5.000000000000000000, 8.660254037844385522, -181.7500000000000000 ) ) ;
#4192=CARTESIAN_POINT ( 'NONE',  ( 7.070501591499376803E-16, 11.54700538379251284, -151.6250000000000000 ) ) ;
#4195=CARTESIAN_POINT ( 'NONE',  ( -5.405949406250003975, -9.363379034771801557, -177.3437500020483810 ) ) ;
#4198=CARTESIAN_POINT ( 'NONE',  ( 5.405949406249992428, -9.363379034771808662, -52.78125000204836681 ) ) ;
#4200=CARTESIAN_POINT ( 'NONE',  ( 7.070501591499377789E-16, 11.54700538379251284, -106.6249999999999716 ) ) ;
#4202=VERTEX_POINT ( 'NONE', #27001 ) ;
#4203=CARTESIAN_POINT ( 'NONE',  ( -2.293366432827344421E-15, -12.48450537969573659, -138.4062500020484094 ) ) ;
#4204=CARTESIAN_POINT ( 'NONE',  ( 9.999999999999996447, -5.773502691896262640, -158.5000000040968189 ) ) ;
#4205=CARTESIAN_POINT ( 'NONE',  ( -2.293366432827344421E-15, -12.48450537969573659, -148.9062500020483810 ) ) ;
#4207=CARTESIAN_POINT ( 'NONE',  ( -10.81189881249999729, 1.324075727343319199E-15, -84.59375000204836681 ) ) ;
#4210=CARTESIAN_POINT ( 'NONE',  ( -10.81189881249999907, -6.242252689847864744, -180.4687500020484094 ) ) ;
#4213=CARTESIAN_POINT ( 'NONE',  ( 0.000000000000000000, 0.000000000000000000, -99.99999999999998579 ) ) ;
#4214=CARTESIAN_POINT ( 'NONE',  ( -10.81189881249999907, -6.242252689847864744, -75.65625000204839523 ) ) ;
#4216=AXIS2_PLACEMENT_3D ( 'NONE', #4380, #24029, #26828 ) ;
#4218=CARTESIAN_POINT ( 'NONE',  ( -5.000000000000003553, -8.660254037844383745, -50.87500000409675494 ) ) ;
#4219=CARTESIAN_POINT ( 'NONE',  ( -10.81189881249999729, 1.324075727343319199E-15, -12.59375000204834905 ) ) ;
#4223=CARTESIAN_POINT ( 'NONE',  ( -5.405949406250003975, -9.363379034771801557, -3.531250002048374803 ) ) ;
#4226=CARTESIAN_POINT ( 'NONE',  ( -5.000000000000003553, -8.660254037844383745, -103.3750000040967763 ) ) ;
#4230=ORIENTED_EDGE ( 'NONE', *, *, #28859, .T. ) ;
#4239=CARTESIAN_POINT ( 'NONE',  ( 5.000000000000000000, 8.660254037844385522, -43.74999999999998579 ) ) ;
#4241=CARTESIAN_POINT ( 'NONE',  ( 10.81189881249999729, 0.000000000000000000, -167.8437500020484094 ) ) ;
#4244=CARTESIAN_POINT ( 'NONE',  ( -9.999999999999998224, 1.224646799147353059E-15, -128.7499999999999716 ) ) ;
#4250=CARTESIAN_POINT ( 'NONE',  ( 7.070501591499376803E-16, 11.54700538379251284, -161.0000000040968189 ) ) ;
#4253=CARTESIAN_POINT ( 'NONE',  ( 5.405949406249992428, -9.363379034771808662, -67.59375000204836681 ) ) ;
#4254=CARTESIAN_POINT ( 'NONE',  ( -5.405949406249996869, 9.363379034771805109, -79.03125000204838102 ) ) ;
#4256=CARTESIAN_POINT ( 'NONE',  ( 10.00000000000000000, 5.773502691896255534, -132.3750000000000000 ) ) ;
#4257=CARTESIAN_POINT ( 'NONE',  ( 10.81189881249999551, -6.242252689847874514, -160.6562500020484094 ) ) ;
#4258=CARTESIAN_POINT ( 'NONE',  ( 5.405949406249999534, 9.363379034771803333, -175.2812500020484094 ) ) ;
#4259=AXIS2_PLACEMENT_3D ( 'NONE', #39266, #22879, #32805 ) ;
#4260=CARTESIAN_POINT ( 'NONE',  ( -10.81189881249999907, -6.242252689847864744, -0.4687500020483514329 ) ) ;
#4261=DIRECTION ( 'NONE',  ( -1.000000000000000000, 0.000000000000000000, 0.000000000000000000 ) ) ;
#4262=CARTESIAN_POINT ( 'NONE',  ( 10.81189881249999551, -6.242252689847874514, -106.4687500020483810 ) ) ;
#4263=CARTESIAN_POINT ( 'NONE',  ( 7.070501591499376803E-16, 11.54700538379251284, -156.1250000000000000 ) ) ;
#4265=CARTESIAN_POINT ( 'NONE',  ( -2.293366432827344421E-15, -12.48450537969573659, -6.406250002048363257 ) ) ;
#4268=CARTESIAN_POINT ( 'NONE',  ( 10.81189881249999907, 6.242252689847868297, -98.90625000204839523 ) ) ;
#4270=CARTESIAN_POINT ( 'NONE',  ( 5.000000000000000000, 8.660254037844385522, -77.12500000409677625 ) ) ;
#4272=CARTESIAN_POINT ( 'NONE',  ( -2.293366432827344421E-15, -12.48450537969573659, -31.71875000204834905 ) ) ;
#4275=CARTESIAN_POINT ( 'NONE',  ( -10.81189881249999729, 6.242252689847871849, -24.90625000204838102 ) ) ;
#4278=CARTESIAN_POINT ( 'NONE',  ( -10.00000000000000000, -5.773502691896251982, -1.500000004096752271 ) ) ;
#4281=EDGE_CURVE ( 'NONE', #42437, #28218, #36922, .T. ) ;
#4282=CARTESIAN_POINT ( 'NONE',  ( -9.999999999999742428, -5.773502691896402084, -156.0000000040968473 ) ) ;
#4284=ORIENTED_EDGE ( 'NONE', *, *, #33039, .F. ) ;
#4285=FACE_OUTER_BOUND ( 'NONE', #37764, .T. ) ;
#4297=CARTESIAN_POINT ( 'NONE',  ( -10.81189881249999729, 1.324075727343319199E-15, -170.2812500020484094 ) ) ;
#4298=EDGE_CURVE ( 'NONE', #25488, #13677, #23467, .T. ) ;
#4300=CARTESIAN_POINT ( 'NONE',  ( 5.405949406249992428, -9.363379034771808662, -94.59375000204838102 ) ) ;
#4301=CARTESIAN_POINT ( 'NONE',  ( 9.999999999999479527, 5.773502691896553074, -113.2500000040967620 ) ) ;
#4302=CARTESIAN_POINT ( 'NONE',  ( 10.81189881249999907, 6.242252689847868297, -100.4062500020483952 ) ) ;
#4304=CARTESIAN_POINT ( 'NONE',  ( -10.81189881249999729, 6.242252689847871849, -110.2187500020483810 ) ) ;
#4308=CARTESIAN_POINT ( 'NONE',  ( 10.81189881249999729, 0.000000000000000000, -199.5312500020484094 ) ) ;
#4311=CARTESIAN_POINT ( 'NONE',  ( 7.070501591499377789E-16, 11.54700538379251284, -176.0000000040968189 ) ) ;
#4313=CARTESIAN_POINT ( 'NONE',  ( 10.81189881249999907, 6.242252689847868297, -19.21875000204836681 ) ) ;
#4315=CARTESIAN_POINT ( 'NONE',  ( -5.405949406250003975, -9.363379034771801557, -133.8437500020484094 ) ) ;
#4317=CARTESIAN_POINT ( 'NONE',  ( 5.405949406249992428, -9.363379034771808662, -27.28125000204836681 ) ) ;
#4320=CARTESIAN_POINT ( 'NONE',  ( 9.999999999999998224, 0.000000000000000000, -158.3750000040967905 ) ) ;
#4321=CARTESIAN_POINT ( 'NONE',  ( -9.999999999999998224, 5.773502691896259087, -62.87499999999998579 ) ) ;
#4322=CARTESIAN_POINT ( 'NONE',  ( -5.405949406250003975, -9.363379034771801557, -120.5312500020483952 ) ) ;
#4326=CARTESIAN_POINT ( 'NONE',  ( -2.121150477449813534E-15, -11.54700538379251284, -103.2500000040967763 ) ) ;
#4328=CARTESIAN_POINT ( 'NONE',  ( 10.81189881249999729, 0.000000000000000000, -59.84375000204835970 ) ) ;
#4329=VERTEX_POINT ( 'NONE', #37127 ) ;
#4333=CARTESIAN_POINT ( 'NONE',  ( 4.999999999999992006, -8.660254037844389075, -26.62500000409676204 ) ) ;
#4335=ADVANCED_FACE ( 'NONE', ( #4336 ), #17908, .F. ) ;
#4336=FACE_OUTER_BOUND ( 'NONE', #32090, .T. ) ;
#4340=EDGE_CURVE ( 'NONE', #30728, #18233, #34772, .T. ) ;
#4347=CARTESIAN_POINT ( 'NONE',  ( -2.293366432827344421E-15, -12.48450537969573659, -193.9062500020484094 ) ) ;
#4353=CARTESIAN_POINT ( 'NONE',  ( 10.81189881249999551, -6.242252689847874514, -116.9687500020483952 ) ) ;
#4354=CARTESIAN_POINT ( 'NONE',  ( 5.405949406249992428, -9.363379034771808662, -0.09375000204836503315 ) ) ;
#4355=CARTESIAN_POINT ( 'NONE',  ( 5.405949406249992428, -9.363379034771808662, -127.7812500020483810 ) ) ;
#4357=CARTESIAN_POINT ( 'NONE',  ( 10.81189881249999729, 6.242252689847867408, -130.2187500020483810 ) ) ;
#4361=CARTESIAN_POINT ( 'NONE',  ( -2.121150477449813534E-15, -11.54700538379251284, -152.3750000000000000 ) ) ;
#4362=CARTESIAN_POINT ( 'NONE',  ( -9.999999999999998224, 5.773502691896259087, -17.87499999999997513 ) ) ;
#4367=CARTESIAN_POINT ( 'NONE',  ( -10.81189881249999729, 1.324075727343319199E-15, -47.09375000204838102 ) ) ;
#4368=CARTESIAN_POINT ( 'NONE',  ( -9.999999999999998224, 1.224646799147353059E-15, -171.1250000040968189 ) ) ;
#4369=CARTESIAN_POINT ( 'NONE',  ( -2.293366432827344421E-15, -12.48450537969573659, -154.7187500020483810 ) ) ;
#4373=CARTESIAN_POINT ( 'NONE',  ( 10.00000000000000000, 5.773502691896255534, -81.37499999999998579 ) ) ;
#4375=EDGE_LOOP ( 'NONE', ( #6883, #24316, #26270, #14560 ) ) ;
#4377=CARTESIAN_POINT ( 'NONE',  ( 9.999999999999996447, -5.773502691896262640, -122.5000000040967905 ) ) ;
#4380=CARTESIAN_POINT ( 'NONE',  ( 0.000000000000000000, 0.000000000000000000, -99.99999999999998579 ) ) ;
#4381=CARTESIAN_POINT ( 'NONE',  ( -10.81189881249999907, -6.242252689847864744, -54.65625000204838102 ) ) ;
#4382=CARTESIAN_POINT ( 'NONE',  ( -9.999999999999998224, 1.224646799147353059E-15, -136.2499999999999716 ) ) ;
#4385=CARTESIAN_POINT ( 'NONE',  ( -9.999999999999996447, 5.773502691896259975, -165.2500000040967905 ) ) ;
#4394=EDGE_CURVE ( 'NONE', #16041, #33493, #11865, .T. ) ;
#4395=CARTESIAN_POINT ( 'NONE',  ( 0.000000000000000000, 0.000000000000000000, -99.99999999999998579 ) ) ;
#4400=CARTESIAN_POINT ( 'NONE',  ( 5.405949406249992428, -9.363379034771808662, -138.0937500020483810 ) ) ;
#4401=CARTESIAN_POINT ( 'NONE',  ( 10.81189881249999551, -6.242252689847874514, -157.4687500020484379 ) ) ;
#4403=CARTESIAN_POINT ( 'NONE',  ( 4.999999999999992006, -8.660254037844389075, -139.1250000040967905 ) ) ;
#4404=CARTESIAN_POINT ( 'NONE',  ( -10.00000000000000000, -5.773502691896251982, -179.6250000000000284 ) ) ;
#4406=CARTESIAN_POINT ( 'NONE',  ( -2.520757610592990083, 10.51993215483609490, -99.99999999999995737 ) ) ;
#4409=CARTESIAN_POINT ( 'NONE',  ( 10.81189881249999551, -6.242252689847874514, -175.4687500020484094 ) ) ;
#4413=CARTESIAN_POINT ( 'NONE',  ( -2.293366432827344421E-15, -12.48450537969573659, -54.40625000204838102 ) ) ;
#4415=CARTESIAN_POINT ( 'NONE',  ( -9.999999999999998224, 5.773502691896259087, -109.3750000000000000 ) ) ;
#4417=CARTESIAN_POINT ( 'NONE',  ( 10.81189881249999729, 6.242252689847867408, -134.9062500020483810 ) ) ;
#4418=CARTESIAN_POINT ( 'NONE',  ( -4.999999999999996447, 8.660254037844387298, -150.3750000040967905 ) ) ;
#4419=CARTESIAN_POINT ( 'NONE',  ( 5.405949406249992428, -9.363379034771808662, -148.7812500020483810 ) ) ;
#4423=CARTESIAN_POINT ( 'NONE',  ( -10.81189881249999729, 1.324075727343319199E-15, -179.0937500020484094 ) ) ;
#4426=( BOUNDED_CURVE ( )  B_SPLINE_CURVE ( 2, ( #11234, #41003, #4771, #6006, #9026, #18946, #2769 ),
 .UNSPECIFIED., .F., .F. ) 
 B_SPLINE_CURVE_WITH_KNOTS ( ( 3, 2, 2, 3 ),
 ( 0.3507462686567164867, 0.3519900497512438720, 0.3532338308457712572, 0.3544776119402986980 ),
 .UNSPECIFIED. ) 
 CURVE ( )  GEOMETRIC_REPRESENTATION_ITEM ( )  RATIONAL_B_SPLINE_CURVE ( ( 0.9999999999999940048, 0.8660254037844447028, 1.000000000000000000, 0.8660254037844387076, 1.000000000000000000, 0.8660254037844207220, 1.000000000000017986 ) ) 
 REPRESENTATION_ITEM ( '' )  );
#4428=CARTESIAN_POINT ( 'NONE',  ( 5.405949406249992428, -9.363379034771808662, -78.28125000204838102 ) ) ;
#4430=CARTESIAN_POINT ( 'NONE',  ( -9.999999999999998224, 1.224646799147353059E-15, -55.62500000409676204 ) ) ;
#4431=CARTESIAN_POINT ( 'NONE',  ( 5.405949406249999534, 9.363379034771803333, -10.09375000204834549 ) ) ;
#4434=CARTESIAN_POINT ( 'NONE',  ( 5.405949406249999534, 9.363379034771803333, -5.781250002048377468 ) ) ;
#4441=EDGE_LOOP ( 'NONE', ( #28605, #21906, #40386, #26571 ) ) ;
#4442=CARTESIAN_POINT ( 'NONE',  ( 0.000000000000000000, 0.000000000000000000, -99.99999999999998579 ) ) ;
#4444=EDGE_LOOP ( 'NONE', ( #4635, #2340, #108, #23454 ) ) ;
#4450=CARTESIAN_POINT ( 'NONE',  ( 10.00000000000000000, 5.773502691896255534, -45.37499999999997158 ) ) ;
#4452=CARTESIAN_POINT ( 'NONE',  ( 7.644554776091147741E-16, 12.48450537969573659, -162.9687500020483810 ) ) ;
#4462=EDGE_CURVE ( 'NONE', #7311, #33113, #34555, .T. ) ;
#4463=CARTESIAN_POINT ( 'NONE',  ( -10.81189881249999907, -6.242252689847864744, -72.46875000204835260 ) ) ;
#4464=CARTESIAN_POINT ( 'NONE',  ( 10.81189881249999729, 0.000000000000000000, -76.53125000204838102 ) ) ;
#4466=CARTESIAN_POINT ( 'NONE',  ( 7.070501591499377789E-16, 11.54700538379251284, -135.1250000000000000 ) ) ;
#4468=CARTESIAN_POINT ( 'NONE',  ( 10.81189881249999551, -6.242252689847874514, -159.1562500020484094 ) ) ;
#4469=CARTESIAN_POINT ( 'NONE',  ( 5.405949406249992428, -9.363379034771808662, -174.2812500020484094 ) ) ;
#4471=DIRECTION ( 'NONE',  ( 0.000000000000000000, 0.000000000000000000, -1.000000000000000000 ) ) ;
#4472=CARTESIAN_POINT ( 'NONE',  ( -5.405949406250003975, -9.363379034771801557, -108.3437500020483810 ) ) ;
#4473=CARTESIAN_POINT ( 'NONE',  ( -9.999999999999998224, 1.224646799147353059E-15, -130.6250000040967620 ) ) ;
#4475=CARTESIAN_POINT ( 'NONE',  ( 7.644554776091147741E-16, 12.48450537969573659, -1.156250002048359038 ) ) ;
#4478=CARTESIAN_POINT ( 'NONE',  ( 7.644554776091147741E-16, 12.48450537969573659, -98.65625000204838102 ) ) ;
#4481=CARTESIAN_POINT ( 'NONE',  ( -5.000000000000003553, -8.660254037844383745, -73.37500000409677625 ) ) ;
#4483=CARTESIAN_POINT ( 'NONE',  ( -10.81189881249999907, -6.242252689847864744, -37.96875000204835970 ) ) ;
#4484=EDGE_LOOP ( 'NONE', ( #27084, #12915, #33120, #2907 ) ) ;
#4486=CARTESIAN_POINT ( 'NONE',  ( 10.81189881249999907, 6.242252689847868297, -26.90625000204838813 ) ) ;
#4489=CARTESIAN_POINT ( 'NONE',  ( -5.000000000000003553, -8.660254037844383745, -1.375000004096765815 ) ) ;
#4504=CARTESIAN_POINT ( 'NONE',  ( 10.81189881249999551, -6.242252689847874514, -172.6562500020484379 ) ) ;
#4505=CARTESIAN_POINT ( 'NONE',  ( 9.999999999999998224, 1.224646799147353059E-15, -99.99999999999998579 ) ) ;
#4507=CARTESIAN_POINT ( 'NONE',  ( 7.644554776091147741E-16, 12.48450537969573659, -92.46875000204838102 ) ) ;
#4509=CARTESIAN_POINT ( 'NONE',  ( 7.070501591499376803E-16, 11.54700538379251284, -154.6250000000000284 ) ) ;
#4510=CARTESIAN_POINT ( 'NONE',  ( -10.81189881249999729, 6.242252689847871849, -96.90625000204838102 ) ) ;
#4512=CARTESIAN_POINT ( 'NONE',  ( -5.405949406250003975, -9.363379034771801557, -106.8437500020483810 ) ) ;
#4515=CARTESIAN_POINT ( 'NONE',  ( 10.81189881249999551, -6.242252689847874514, -195.1562500020484379 ) ) ;
#4518=CARTESIAN_POINT ( 'NONE',  ( 9.999999999999998224, 0.000000000000000000, -170.3750000040968189 ) ) ;
#4520=CARTESIAN_POINT ( 'NONE',  ( -5.405949406249996869, 9.363379034771805109, -20.34375000204835615 ) ) ;
#4522=CARTESIAN_POINT ( 'NONE',  ( 5.405949406249992428, -9.363379034771808662, -127.5937500020483668 ) ) ;
#4525=CARTESIAN_POINT ( 'NONE',  ( 5.405949406249999534, 9.363379034771803333, -31.28125000204837036 ) ) ;
#4528=CARTESIAN_POINT ( 'NONE',  ( 10.00000000000000000, 5.773502691896255534, -58.87499999999997868 ) ) ;
#4529=CARTESIAN_POINT ( 'NONE',  ( -5.405949406250003975, -9.363379034771801557, -128.0312500020484094 ) ) ;
#4532=CARTESIAN_POINT ( 'NONE',  ( 10.00000000000025402, -5.773502691896113426, -117.6250000000000142 ) ) ;
#4533=CARTESIAN_POINT ( 'NONE',  ( 9.999999999999996447, -5.773502691896262640, -101.5000000040967905 ) ) ;
#4534=CYLINDRICAL_SURFACE ( 'NONE', #8465, 9.999999999999998224 ) ;
#4536=CARTESIAN_POINT ( 'NONE',  ( -10.81189881249999729, 1.324075727343319199E-15, -59.09375000204835970 ) ) ;
#4537=ORIENTED_EDGE ( 'NONE', *, *, #19813, .F. ) ;
#4542=CARTESIAN_POINT ( 'NONE',  ( -9.999999999999998224, 1.224646799147353059E-15, -30.12500000409676204 ) ) ;
#4548=AXIS2_PLACEMENT_3D ( 'NONE', #17327, #40410, #39788 ) ;
#4557=CARTESIAN_POINT ( 'NONE',  ( -5.405949406249996869, 9.363379034771805109, -199.0312500020484094 ) ) ;
#4563=CARTESIAN_POINT ( 'NONE',  ( 5.405949406249992428, -9.363379034771808662, -115.5937500020483810 ) ) ;
#4564=CARTESIAN_POINT ( 'NONE',  ( -9.999999999999998224, 1.224646799147353059E-15, -195.1250000040967905 ) ) ;
#4565=CARTESIAN_POINT ( 'NONE',  ( 10.81189881249999907, 6.242252689847868297, -127.4062500020483810 ) ) ;
#4567=CARTESIAN_POINT ( 'NONE',  ( -5.405949406249996869, 9.363379034771805109, -134.3437500020484094 ) ) ;
#4570=CARTESIAN_POINT ( 'NONE',  ( 9.999999999999998224, 0.000000000000000000, -158.0000000000000000 ) ) ;
#4571=CARTESIAN_POINT ( 'NONE',  ( 5.000000000000000000, 8.660254037844385522, -16.74999999999996092 ) ) ;
#4574=CARTESIAN_POINT ( 'NONE',  ( -9.999999999999998224, 1.224646799147353059E-15, -170.7500000000000000 ) ) ;
#4576=CARTESIAN_POINT ( 'NONE',  ( -2.293366432827344421E-15, -12.48450537969573659, -49.71875000204836681 ) ) ;
#4578=EDGE_CURVE ( 'NONE', #28777, #34758, #42226, .T. ) ;
#4579=CARTESIAN_POINT ( 'NONE',  ( -5.405949406249996869, 9.363379034771805109, -155.3437500020483810 ) ) ;
#4583=CARTESIAN_POINT ( 'NONE',  ( 1.498518790203807738, 10.17864512702100832, -179.9999999999998863 ) ) ;
#4584=CARTESIAN_POINT ( 'NONE',  ( 9.999999999999996447, -5.773502691896262640, -80.12500000000000000 ) ) ;
#4586=ADVANCED_FACE ( 'NONE', ( #24347 ), #10722, .F. ) ;
#4588=CARTESIAN_POINT ( 'NONE',  ( 7.644554776091147741E-16, 12.48450537969573659, -104.6562500020483810 ) ) ;
#4589=CARTESIAN_POINT ( 'NONE',  ( 10.00000000000000000, 5.773502691896255534, -123.7500000040967905 ) ) ;
#4593=CARTESIAN_POINT ( 'NONE',  ( -10.81189881249999729, 6.242252689847871849, -47.40625000204836681 ) ) ;
#4599=VERTEX_POINT ( 'NONE', #1031 ) ;
#4603=EDGE_CURVE ( 'NONE', #27698, #42437, #8601, .T. ) ;
#4604=ORIENTED_EDGE ( 'NONE', *, *, #19687, .F. ) ;
#4614=CARTESIAN_POINT ( 'NONE',  ( 10.81189881249999907, 6.242252689847868297, -140.7187500020483810 ) ) ;
#4615=CARTESIAN_POINT ( 'NONE',  ( 10.81189881249999729, 0.000000000000000000, -148.5312500020483810 ) ) ;
#4616=CARTESIAN_POINT ( 'NONE',  ( 5.405949406249999534, 9.363379034771803333, -151.0937500020483810 ) ) ;
#4618=CARTESIAN_POINT ( 'NONE',  ( -2.121150477449813534E-15, -11.54700538379251284, -182.3750000000000000 ) ) ;
#4622=CARTESIAN_POINT ( 'NONE',  ( 9.999999999999872102, 5.773502691896329253, -168.7500000040967905 ) ) ;
#4623=CARTESIAN_POINT ( 'NONE',  ( 10.81189881249999729, 0.000000000000000000, -175.3437500020483810 ) ) ;
#4627=CARTESIAN_POINT ( 'NONE',  ( -10.81189881249999729, 1.324075727343319199E-15, -44.28125000204838102 ) ) ;
#4629=CARTESIAN_POINT ( 'NONE',  ( 9.999999999999996447, -5.773502691896262640, -107.1249999999999858 ) ) ;
#4631=CARTESIAN_POINT ( 'NONE',  ( -2.293366432827344421E-15, -12.48450537969573659, -127.9062500020483952 ) ) ;
#4632=CARTESIAN_POINT ( 'NONE',  ( 5.000000000000000000, 8.660254037844385522, -144.6250000040967905 ) ) ;
#4633=FACE_OUTER_BOUND ( 'NONE', #42222, .T. ) ;
#4635=ORIENTED_EDGE ( 'NONE', *, *, #18426, .F. ) ;
#4637=CARTESIAN_POINT ( 'NONE',  ( -5.405949406250003975, -9.363379034771801557, -169.8437500020484094 ) ) ;
#4641=CARTESIAN_POINT ( 'NONE',  ( 5.405949406249992428, -9.363379034771808662, -64.78125000204838102 ) ) ;
#4643=CARTESIAN_POINT ( 'NONE',  ( 9.999999999999998224, 0.000000000000000000, -50.37500000409675494 ) ) ;
#4644=CARTESIAN_POINT ( 'NONE',  ( 10.81189881249999907, 6.242252689847868297, -2.718750002048353043 ) ) ;
#4648=DIRECTION ( 'NONE',  ( -1.000000000000000000, 0.000000000000000000, 0.000000000000000000 ) ) ;
#4649=CARTESIAN_POINT ( 'NONE',  ( 4.999999999999992006, -8.660254037844389075, -103.1250000040967763 ) ) ;
#4662=CARTESIAN_POINT ( 'NONE',  ( -9.999999999999998224, 5.773502691896259087, -46.37499999999996447 ) ) ;
#4664=CARTESIAN_POINT ( 'NONE',  ( 10.81189881249999551, -6.242252689847874514, -164.9687500020484094 ) ) ;
#4665=CARTESIAN_POINT ( 'NONE',  ( 8.614196012144985204, -6.533971456632194474, -179.9999999999999716 ) ) ;
#4669=CARTESIAN_POINT ( 'NONE',  ( -9.999999999999998224, 1.224646799147353059E-15, -175.2500000000000284 ) ) ;
#4677=CARTESIAN_POINT ( 'NONE',  ( -10.81189881249999907, -6.242252689847864744, -63.46875000204838102 ) ) ;
#4678=CARTESIAN_POINT ( 'NONE',  ( 10.81189881249999729, 0.000000000000000000, -67.53125000204838102 ) ) ;
#4680=CARTESIAN_POINT ( 'NONE',  ( -4.999999999999996447, 8.660254037844387298, -130.5000000000000000 ) ) ;
#4681=CARTESIAN_POINT ( 'NONE',  ( 10.81189881249999729, 0.000000000000000000, -147.0312500020483810 ) ) ;
#4682=CARTESIAN_POINT ( 'NONE',  ( -10.81189881249999907, -6.242252689847864744, -161.1562500020484094 ) ) ;
#4683=DIRECTION ( 'NONE',  ( -1.000000000000000000, 0.000000000000000000, 0.000000000000000000 ) ) ;
#4685=CARTESIAN_POINT ( 'NONE',  ( 10.81189881249999729, 0.000000000000000000, -101.8437500020483810 ) ) ;
#4687=CARTESIAN_POINT ( 'NONE',  ( 5.405949406249992428, -9.363379034771808662, -7.781250002048350822 ) ) ;
#4689=CARTESIAN_POINT ( 'NONE',  ( 8.614196012144985204, -6.533971456632194474, -180.0000000000000000 ) ) ;
#4690=CARTESIAN_POINT ( 'NONE',  ( -10.81189881249999907, -6.242252689847864744, -99.65625000204839523 ) ) ;
#4692=CARTESIAN_POINT ( 'NONE',  ( 9.999999999999998224, 0.000000000000000000, -75.87500000409677625 ) ) ;
#4693=CARTESIAN_POINT ( 'NONE',  ( 9.999999999999479527, 5.773502691896553074, -118.8749999999999858 ) ) ;
#4694=CARTESIAN_POINT ( 'NONE',  ( -5.405949406249996869, 9.363379034771805109, -36.84375000204836681 ) ) ;
#4697=CARTESIAN_POINT ( 'NONE',  ( -10.81189881249999729, 1.324075727343319199E-15, -27.78125000204837036 ) ) ;
#4699=CARTESIAN_POINT ( 'NONE',  ( -4.999999999999996447, 8.660254037844387298, -7.875000004096744277 ) ) ;
#4706=AXIS2_PLACEMENT_3D ( 'NONE', #9135, #12566, #5260 ) ;
#4708=ORIENTED_EDGE ( 'NONE', *, *, #42274, .F. ) ;
#4717=CARTESIAN_POINT ( 'NONE',  ( 5.405949406249999534, 9.363379034771803333, -167.7812500020484094 ) ) ;
#4720=CARTESIAN_POINT ( 'NONE',  ( 7.644554776091147741E-16, 12.48450537969573659, -89.46875000204838102 ) ) ;
#4722=CARTESIAN_POINT ( 'NONE',  ( -10.81189881249999729, 6.242252689847871849, -197.2187500020484379 ) ) ;
#4723=CARTESIAN_POINT ( 'NONE',  ( -10.81189881249999729, 1.324075727343319199E-15, -104.2812500020483810 ) ) ;
#4725=CARTESIAN_POINT ( 'NONE',  ( -10.81189881249999729, -6.242252689847864744, -103.9687500020483810 ) ) ;
#4727=( BOUNDED_CURVE ( )  B_SPLINE_CURVE ( 2, ( #9062, #42480, #9266, #3015, #35822, #2387, #19399 ),
 .UNSPECIFIED., .F., .F. ) 
 B_SPLINE_CURVE_WITH_KNOTS ( ( 3, 2, 2, 3 ),
 ( 0.3917910447761194792, 0.3930348258706468090, 0.3942786069651742498, 0.3955223880597015795 ),
 .UNSPECIFIED. ) 
 CURVE ( )  GEOMETRIC_REPRESENTATION_ITEM ( )  RATIONAL_B_SPLINE_CURVE ( ( 0.9999999999999940048, 0.8660254037844447028, 1.000000000000000000, 0.8660254037844387076, 1.000000000000000000, 0.8660254037844267172, 1.000000000000011990 ) ) 
 REPRESENTATION_ITEM ( '' )  );
#4729=CARTESIAN_POINT ( 'NONE',  ( -9.999999999999998224, 1.224646799147353059E-15, -124.6250000040967763 ) ) ;
#4730=CARTESIAN_POINT ( 'NONE',  ( -10.81189881249999729, 6.242252689847871849, -194.4062500020484094 ) ) ;
#4733=CARTESIAN_POINT ( 'NONE',  ( 10.00000000000000000, 5.773502691896255534, -170.2500000040967905 ) ) ;
#4735=CARTESIAN_POINT ( 'NONE',  ( -2.293366432827344421E-15, -12.48450537969573659, -25.71875000204837391 ) ) ;
#4737=CARTESIAN_POINT ( 'NONE',  ( 10.81189881249999729, 0.000000000000000000, -128.8437500020484094 ) ) ;
#4739=CARTESIAN_POINT ( 'NONE',  ( 5.405949406249992428, -9.363379034771808662, -25.78125000204836681 ) ) ;
#4742=CARTESIAN_POINT ( 'NONE',  ( -9.999999999999998224, 1.224646799147353059E-15, -52.24999999999996447 ) ) ;
#4743=CARTESIAN_POINT ( 'NONE',  ( -10.81189881249999729, 1.324075727343319199E-15, -122.2812500020483952 ) ) ;
#4746=CARTESIAN_POINT ( 'NONE',  ( -10.00000000000000000, -5.773502691896251982, -100.5000000040967905 ) ) ;
#4747=CARTESIAN_POINT ( 'NONE',  ( -5.000000000000003553, -8.660254037844383745, -113.4999999999999858 ) ) ;
#4749=CARTESIAN_POINT ( 'NONE',  ( -10.81189881249999729, 6.242252689847871849, -54.71875000204837391 ) ) ;
#4755=CARTESIAN_POINT ( 'NONE',  ( -4.999999999999996447, 8.660254037844387298, -28.87500000409676204 ) ) ;
#4756=CARTESIAN_POINT ( 'NONE',  ( 9.999999999999998224, 0.000000000000000000, -168.5000000000000000 ) ) ;
#4764=VERTEX_POINT ( 'NONE', #4473 ) ;
#4765=DIRECTION ( 'NONE',  ( -0.000000000000000000, -0.000000000000000000, -1.000000000000000000 ) ) ;
#4766=CARTESIAN_POINT ( 'NONE',  ( 9.999999999999998224, 0.000000000000000000, -174.8750000040967905 ) ) ;
#4768=CARTESIAN_POINT ( 'NONE',  ( -5.405949406250003975, -9.363379034771801557, -188.0312500020484094 ) ) ;
#4771=CARTESIAN_POINT ( 'NONE',  ( 5.000000000000000000, 8.660254037844385522, -129.2499999999999716 ) ) ;
#4775=CARTESIAN_POINT ( 'NONE',  ( -2.293366432827344421E-15, -12.48450537969573659, -121.7187500020483952 ) ) ;
#4776=CARTESIAN_POINT ( 'NONE',  ( 7.644554776091147741E-16, 12.48450537969573659, 0.5312499979516493998 ) ) ;
#4777=CARTESIAN_POINT ( 'NONE',  ( 5.405949406249992428, -9.363379034771808662, -126.2812500020483668 ) ) ;
#4779=CARTESIAN_POINT ( 'NONE',  ( -5.405949406250003975, -9.363379034771801557, -130.8437500020484094 ) ) ;
#4782=CARTESIAN_POINT ( 'NONE',  ( -4.999999999999996447, 8.660254037844387298, -150.0000000000000000 ) ) ;
#4783=CARTESIAN_POINT ( 'NONE',  ( -4.999999999999996447, 8.660254037844387298, -20.99999999999996447 ) ) ;
#4786=CARTESIAN_POINT ( 'NONE',  ( 4.999999999999992006, -8.660254037844389075, -170.2500000000000000 ) ) ;
#4788=CARTESIAN_POINT ( 'NONE',  ( 5.405949406249992428, -9.363379034771808662, -43.59375000204837391 ) ) ;
#4789=DIRECTION ( 'NONE',  ( -0.000000000000000000, -0.000000000000000000, -1.000000000000000000 ) ) ;
#4790=CARTESIAN_POINT ( 'NONE',  ( 10.81189881249999729, 0.000000000000000000, -154.3437500020483810 ) ) ;
#4794=CARTESIAN_POINT ( 'NONE',  ( 7.070501591499377789E-16, 11.54700538379251284, -76.62499999999997158 ) ) ;
#4796=EDGE_LOOP ( 'NONE', ( #13179, #1194, #23884, #1624 ) ) ;
#4797=CARTESIAN_POINT ( 'NONE',  ( 10.81189881249999729, 0.000000000000000000, -102.0312500020483952 ) ) ;
#4798=CARTESIAN_POINT ( 'NONE',  ( 7.070501591499377789E-16, 11.54700538379251284, -122.0000000040967905 ) ) ;
#4799=CARTESIAN_POINT ( 'NONE',  ( 4.999999999999992006, -8.660254037844389075, -154.1250000040967905 ) ) ;
#4803=CARTESIAN_POINT ( 'NONE',  ( 7.644554776091147741E-16, 12.48450537969573659, -44.65625000204836681 ) ) ;
#4808=CARTESIAN_POINT ( 'NONE',  ( -4.999999999999996447, 8.660254037844387298, -109.4999999999999858 ) ) ;
#4812=EDGE_CURVE ( 'NONE', #31374, #5830, #27784, .T. ) ;
#4826=CARTESIAN_POINT ( 'NONE',  ( 10.81189881249999729, 0.000000000000000000, -145.3437500020483810 ) ) ;
#4827=CARTESIAN_POINT ( 'NONE',  ( -5.405949406249996869, 9.363379034771805109, -145.0312500020483810 ) ) ;
#4828=CARTESIAN_POINT ( 'NONE',  ( 10.81189881249999729, 0.000000000000000000, -154.3437500020483810 ) ) ;
#4831=CARTESIAN_POINT ( 'NONE',  ( -9.999999999999998224, 5.773502691896259087, -175.3750000000000000 ) ) ;
#4835=CARTESIAN_POINT ( 'NONE',  ( -8.865618880899917897, 5.969117493042149114, -99.99999999999998579 ) ) ;
#4836=CARTESIAN_POINT ( 'NONE',  ( -5.405949406249996869, 9.363379034771805109, -176.3437500020483810 ) ) ;
#4841=CARTESIAN_POINT ( 'NONE',  ( -10.81189881249999729, 1.324075727343319199E-15, -41.28125000204838102 ) ) ;
#4843=CARTESIAN_POINT ( 'NONE',  ( 9.999999999999998224, 0.000000000000000000, -105.4999999999999858 ) ) ;
#4846=CARTESIAN_POINT ( 'NONE',  ( -10.81189881249999729, 6.242252689847871849, -128.4062500020483810 ) ) ;
#4847=CARTESIAN_POINT ( 'NONE',  ( -9.999999999999998224, 5.773502691896259087, -145.7500000040967905 ) ) ;
#4848=CARTESIAN_POINT ( 'NONE',  ( 4.999999999999992006, -8.660254037844389075, -167.2500000000000000 ) ) ;
#4849=EDGE_CURVE ( 'NONE', #33599, #11060, #30655, .T. ) ;
#4852=CARTESIAN_POINT ( 'NONE',  ( 10.81189881249999907, 6.242252689847868297, -172.2187500020483810 ) ) ;
#4855=CARTESIAN_POINT ( 'NONE',  ( -9.999999999999998224, 1.224646799147353059E-15, -109.6250000040967763 ) ) ;
#4857=CARTESIAN_POINT ( 'NONE',  ( 7.644554776091147741E-16, 12.48450537969573659, -71.65625000204836681 ) ) ;
#4859=CARTESIAN_POINT ( 'NONE',  ( -2.121150477449813534E-15, -11.54700538379251284, -44.75000000409676204 ) ) ;
#4860=CARTESIAN_POINT ( 'NONE',  ( -2.293366432827344421E-15, -12.48450537969573659, -4.718750002048355263 ) ) ;
#4861=CARTESIAN_POINT ( 'NONE',  ( 31.99999999999997158, 0.000000000000000000, -180.0000000000000000 ) ) ;
#4864=CARTESIAN_POINT ( 'NONE',  ( -9.999999999999998224, 1.224646799147353059E-15, -138.1250000040967620 ) ) ;
#4874=ORIENTED_EDGE ( 'NONE', *, *, #35749, .T. ) ;
#4883=CARTESIAN_POINT ( 'NONE',  ( -9.999999999999998224, 1.224646799147353059E-15, -34.24999999999997158 ) ) ;
#4885=CARTESIAN_POINT ( 'NONE',  ( -5.405949406249996869, 9.363379034771805109, -168.8437500020484094 ) ) ;
#4886=CARTESIAN_POINT ( 'NONE',  ( 5.405949406249999534, 9.363379034771803333, -176.5937500020484094 ) ) ;
#4888=CARTESIAN_POINT ( 'NONE',  ( -2.121150477449813534E-15, -11.54700538379251284, -167.7500000040968189 ) ) ;
#4889=CARTESIAN_POINT ( 'NONE',  ( -10.00000000000076916, 5.773502691895813221, -103.7500000040967763 ) ) ;
#4895=CARTESIAN_POINT ( 'NONE',  ( 5.405949406249992428, -9.363379034771808662, -61.59375000204836681 ) ) ;
#4896=CARTESIAN_POINT ( 'NONE',  ( -5.405949406250003975, -9.363379034771801557, -69.53125000204838102 ) ) ;
#4898=CARTESIAN_POINT ( 'NONE',  ( -5.000000000000003553, -8.660254037844383745, -128.5000000000000000 ) ) ;
#4900=CARTESIAN_POINT ( 'NONE',  ( 7.644554776091147741E-16, 12.48450537969573659, -154.1562500020484094 ) ) ;
#4901=CARTESIAN_POINT ( 'NONE',  ( 5.405949406249999534, 9.363379034771803333, -161.7812500020484094 ) ) ;
#4903=CARTESIAN_POINT ( 'NONE',  ( -9.999999999999998224, 1.224646799147353059E-15, -157.6250000040967905 ) ) ;
#4904=CARTESIAN_POINT ( 'NONE',  ( 5.000000000000000000, 8.660254037844385522, -159.6250000040967905 ) ) ;
#4905=CARTESIAN_POINT ( 'NONE',  ( 10.81189881249999551, -6.242252689847874514, -98.96875000204838102 ) ) ;
#4908=CARTESIAN_POINT ( 'NONE',  ( -5.405949406249996869, 9.363379034771805109, -195.8437500020484094 ) ) ;
#4910=CARTESIAN_POINT ( 'NONE',  ( 2.933915056720935777, -10.14638297711852388, -180.0000000000000284 ) ) ;
#4911=CARTESIAN_POINT ( 'NONE',  ( 10.81189881249999907, 6.242252689847868297, -92.90625000204839523 ) ) ;
#4913=CARTESIAN_POINT ( 'NONE',  ( -9.999999999999998224, 1.224646799147353059E-15, -72.12500000409677625 ) ) ;
#4914=CARTESIAN_POINT ( 'NONE',  ( 7.070501591499376803E-16, 11.54700538379251284, -118.6250000000000142 ) ) ;
#4915=CARTESIAN_POINT ( 'NONE',  ( -2.293366432827344421E-15, -12.48450537969573659, -27.21875000204837747 ) ) ;
#4918=CARTESIAN_POINT ( 'NONE',  ( 7.644554776091147741E-16, 12.48450537969573659, -28.15625000204838102 ) ) ;
#4921=CARTESIAN_POINT ( 'NONE',  ( -9.999999999999998224, 1.224646799147353059E-15, -4.625000004096769146 ) ) ;
#4928=DIRECTION ( 'NONE',  ( 0.000000000000000000, 0.000000000000000000, 1.000000000000000000 ) ) ;
#4935=DIRECTION ( 'NONE',  ( -0.000000000000000000, -0.000000000000000000, -1.000000000000000000 ) ) ;
#4937=( BOUNDED_CURVE ( )  B_SPLINE_CURVE ( 2, ( #32059, #25579, #31854, #2288, #18448, #2908, #28607 ),
 .UNSPECIFIED., .F., .F. ) 
 B_SPLINE_CURVE_WITH_KNOTS ( ( 3, 2, 2, 3 ),
 ( 0.1268656716417910224, 0.1281094527363183799, 0.1293532338308457652, 0.1305970149253731227 ),
 .UNSPECIFIED. ) 
 CURVE ( )  GEOMETRIC_REPRESENTATION_ITEM ( )  RATIONAL_B_SPLINE_CURVE ( ( 1.000000000000003109, 0.8660254037844358210, 1.000000000000000000, 0.8660254037844387076, 1.000000000000000000, 0.8660254037844387076, 1.000000000000000000 ) ) 
 REPRESENTATION_ITEM ( '' )  );
#4938=LINE ( 'NONE', #39949, #28819 ) ;
#4939=CARTESIAN_POINT ( 'NONE',  ( 10.81189881249999551, -6.242252689847874514, -168.1562500020484094 ) ) ;
#4941=LINE ( 'NONE', #4505, #26734 ) ;
#4942=ADVANCED_FACE ( 'NONE', ( #27271 ), #13443, .F. ) ;
#4944=CARTESIAN_POINT ( 'NONE',  ( 10.81189881249999907, 6.242252689847868297, -88.21875000204838102 ) ) ;
#4945=CARTESIAN_POINT ( 'NONE',  ( 9.999999999999998224, 0.000000000000000000, -102.5000000000000000 ) ) ;
#4946=CARTESIAN_POINT ( 'NONE',  ( -10.81189881249999729, 1.324075727343319199E-15, -192.5937500020484094 ) ) ;
#4947=CARTESIAN_POINT ( 'NONE',  ( 5.405949406249992428, -9.363379034771808662, -93.28125000204838102 ) ) ;
#4951=CARTESIAN_POINT ( 'NONE',  ( 10.81189881249999551, -6.242252689847874514, -175.6562500020484094 ) ) ;
#4952=CARTESIAN_POINT ( 'NONE',  ( 7.644554776091147741E-16, 12.48450537969573659, -187.1562500020484094 ) ) ;
#4954=CARTESIAN_POINT ( 'NONE',  ( -9.999999999999998224, 1.224646799147353059E-15, -165.1250000040967905 ) ) ;
#4956=CARTESIAN_POINT ( 'NONE',  ( 7.644554776091147741E-16, 12.48450537969573659, -9.968750002048359704 ) ) ;
#4958=CARTESIAN_POINT ( 'NONE',  ( -10.81189881249999729, 6.242252689847871849, -122.2187500020483810 ) ) ;
#4960=CARTESIAN_POINT ( 'NONE',  ( 7.644554776091147741E-16, 12.48450537969573659, -20.65625000204837747 ) ) ;
#4962=CARTESIAN_POINT ( 'NONE',  ( 10.00000000000000000, 5.773502691896255534, -52.87499999999997868 ) ) ;
#4963=CARTESIAN_POINT ( 'NONE',  ( 5.405949406249999534, 9.363379034771803333, -116.7812500020483952 ) ) ;
#4967=AXIS2_PLACEMENT_3D ( 'NONE', #8535, #35295, #34656 ) ;
#4968=CARTESIAN_POINT ( 'NONE',  ( 9.999999999999996447, -5.773502691896262640, -97.00000000409677625 ) ) ;
#4971=CARTESIAN_POINT ( 'NONE',  ( -10.81189881249999907, -6.242252689847864744, -46.96875000204835970 ) ) ;
#4977=CARTESIAN_POINT ( 'NONE',  ( -9.999999999999998224, 5.773502691896259087, -28.75000000409674783 ) ) ;
#4983=DIRECTION ( 'NONE',  ( -0.000000000000000000, -0.000000000000000000, -1.000000000000000000 ) ) ;
#4990=DIRECTION ( 'NONE',  ( -1.000000000000000000, 0.000000000000000000, 0.000000000000000000 ) ) ;
#4994=ADVANCED_FACE ( 'NONE', ( #748 ), #20154, .T. ) ;
#4996=CARTESIAN_POINT ( 'NONE',  ( 5.405949406249992428, -9.363379034771808662, -187.7812500020484094 ) ) ;
#5001=CARTESIAN_POINT ( 'NONE',  ( 5.405949406249999534, 9.363379034771803333, -109.0937500020483810 ) ) ;
#5003=CARTESIAN_POINT ( 'NONE',  ( 10.81189881249999907, 6.242252689847868297, -116.9062500020483952 ) ) ;
#5005=CARTESIAN_POINT ( 'NONE',  ( 10.81189881249999729, 6.242252689847867408, -127.2187500020483810 ) ) ;
#5008=CARTESIAN_POINT ( 'NONE',  ( -10.00000000000000000, -5.773502691896251982, -151.1250000000000284 ) ) ;
#5009=CARTESIAN_POINT ( 'NONE',  ( -4.999999999999996447, 8.660254037844387298, -16.49999999999995737 ) ) ;
#5015=CARTESIAN_POINT ( 'NONE',  ( -2.293366432827344421E-15, -12.48450537969573659, -45.21875000204835970 ) ) ;
#5017=CARTESIAN_POINT ( 'NONE',  ( 7.644554776091147741E-16, 12.48450537969573659, -149.4687500020484094 ) ) ;
#5021=CARTESIAN_POINT ( 'NONE',  ( -9.999999999999998224, 5.773502691896259087, -77.87499999999998579 ) ) ;
#5023=VERTEX_POINT ( 'NONE', #6056 ) ;
#5025=CARTESIAN_POINT ( 'NONE',  ( -2.121150477449813534E-15, -11.54700538379251284, -121.2500000040967905 ) ) ;
#5026=CARTESIAN_POINT ( 'NONE',  ( -5.000000000000003553, -8.660254037844383745, -154.3750000040967905 ) ) ;
#5027=CARTESIAN_POINT ( 'NONE',  ( 7.644554776091147741E-16, 12.48450537969573659, -84.96875000204835260 ) ) ;
#5030=CARTESIAN_POINT ( 'NONE',  ( -9.999999999999998224, 1.224646799147353059E-15, -131.7499999999999716 ) ) ;
#5031=CARTESIAN_POINT ( 'NONE',  ( 5.405949406249999534, 9.363379034771803333, -47.78125000204838813 ) ) ;
#5042=CARTESIAN_POINT ( 'NONE',  ( -9.999999999998969713, -5.773502691896847949, -130.5000000040967905 ) ) ;
#5046=CARTESIAN_POINT ( 'NONE',  ( -5.405949406249996869, 9.363379034771805109, -129.8437500020484094 ) ) ;
#5047=CARTESIAN_POINT ( 'NONE',  ( 10.81189881249999907, 6.242252689847868297, -139.4062500020484094 ) ) ;
#5048=CARTESIAN_POINT ( 'NONE',  ( -5.405949406250003975, -9.363379034771801557, -153.3437500020483810 ) ) ;
#5051=CARTESIAN_POINT ( 'NONE',  ( -9.999999999999998224, 1.224646799147353059E-15, -170.7500000000000000 ) ) ;
#5054=CARTESIAN_POINT ( 'NONE',  ( -9.564224651208778738, -3.791567223145488885, -99.99999999999998579 ) ) ;
#5055=CARTESIAN_POINT ( 'NONE',  ( 7.644554776091147741E-16, 12.48450537969573659, -179.4687500020483810 ) ) ;
#5060=CARTESIAN_POINT ( 'NONE',  ( -10.81189881249999729, 6.242252689847871849, -47.40625000204836681 ) ) ;
#5062=CARTESIAN_POINT ( 'NONE',  ( -5.000000000000003553, -8.660254037844383745, -95.49999999999998579 ) ) ;
#5063=ORIENTED_EDGE ( 'NONE', *, *, #21137, .F. ) ;
#5064=CARTESIAN_POINT ( 'NONE',  ( -5.405949406249996869, 9.363379034771805109, -128.5312500020484094 ) ) ;
#5065=CARTESIAN_POINT ( 'NONE',  ( 9.999999999999998224, 0.000000000000000000, -149.3750000040967905 ) ) ;
#5066=DIRECTION ( 'NONE',  ( -0.000000000000000000, -0.000000000000000000, -1.000000000000000000 ) ) ;
#5069=CARTESIAN_POINT ( 'NONE',  ( -5.405949406249996869, 9.363379034771805109, -171.8437500020484094 ) ) ;
#5071=ADVANCED_FACE ( 'NONE', ( #2402 ), #5637, .F. ) ;
#5075=CARTESIAN_POINT ( 'NONE',  ( 10.81189881249999551, -6.242252689847874514, -70.65625000204839523 ) ) ;
#5076=CARTESIAN_POINT ( 'NONE',  ( -4.999999999999996447, 8.660254037844387298, -40.87500000409677625 ) ) ;
#5077=CARTESIAN_POINT ( 'NONE',  ( -10.81189881249999729, 1.324075727343319199E-15, -5.093750002048369474 ) ) ;
#5081=CARTESIAN_POINT ( 'NONE',  ( 9.999999999999479527, 5.773502691896553074, -148.8749999999999432 ) ) ;
#5082=ORIENTED_EDGE ( 'NONE', *, *, #6833, .F. ) ;
#5083=CARTESIAN_POINT ( 'NONE',  ( -9.999999999999998224, 1.224646799147353059E-15, -115.2499999999999858 ) ) ;
#5084=FACE_OUTER_BOUND ( 'NONE', #35114, .T. ) ;
#5087=VERTEX_POINT ( 'NONE', #41049 ) ;
#5091=ORIENTED_EDGE ( 'NONE', *, *, #14781, .F. ) ;
#5096=VERTEX_POINT ( 'NONE', #5843 ) ;
#5098=CARTESIAN_POINT ( 'NONE',  ( -9.999999999999998224, 5.773502691896259087, -40.37499999999997158 ) ) ;
#5101=CARTESIAN_POINT ( 'NONE',  ( -5.405949406249996869, 9.363379034771805109, -164.3437500020484094 ) ) ;
#5103=CARTESIAN_POINT ( 'NONE',  ( -5.405949406249996869, 9.363379034771805109, -177.8437500020483810 ) ) ;
#5104=CARTESIAN_POINT ( 'NONE',  ( -4.999999999999996447, 8.660254037844387298, -192.0000000000000000 ) ) ;
#5109=CARTESIAN_POINT ( 'NONE',  ( 5.405949406249999534, 9.363379034771803333, -65.59375000204836681 ) ) ;
#5110=CARTESIAN_POINT ( 'NONE',  ( 5.405949406249992428, -9.363379034771808662, -70.78125000204838102 ) ) ;
#5112=CARTESIAN_POINT ( 'NONE',  ( -2.121150477449813534E-15, -11.54700538379251284, -126.8749999999999858 ) ) ;
#5113=CARTESIAN_POINT ( 'NONE',  ( 5.405949406249999534, 9.363379034771803333, -148.2812500020483810 ) ) ;
#5114=CARTESIAN_POINT ( 'NONE',  ( 10.81189881249999729, 0.000000000000000000, -160.5312500020484094 ) ) ;
#5115=FACE_OUTER_BOUND ( 'NONE', #23717, .T. ) ;
#5117=CARTESIAN_POINT ( 'NONE',  ( -10.81189881249999729, 6.242252689847871849, -96.71875000204838102 ) ) ;
#5118=ORIENTED_EDGE ( 'NONE', *, *, #17487, .T. ) ;
#5120=CARTESIAN_POINT ( 'NONE',  ( 10.81189881249999551, -6.242252689847874514, -197.9687500020484094 ) ) ;
#5122=EDGE_CURVE ( 'NONE', #24722, #41312, #4170, .T. ) ;
#5124=CARTESIAN_POINT ( 'NONE',  ( -10.81189881249999907, -6.242252689847864744, -93.65625000204840944 ) ) ;
#5126=EDGE_CURVE ( 'NONE', #6299, #18722, #28688, .T. ) ;
#5127=CARTESIAN_POINT ( 'NONE',  ( 5.000000000000000000, 8.660254037844385522, -65.12500000409676204 ) ) ;
#5129=CARTESIAN_POINT ( 'NONE',  ( 5.405949406249999534, 9.363379034771803333, -25.09375000204835970 ) ) ;
#5130=ORIENTED_EDGE ( 'NONE', *, *, #6833, .T. ) ;
#5133=CARTESIAN_POINT ( 'NONE',  ( -10.81189881249999729, 1.324075727343319199E-15, -23.28125000204836326 ) ) ;
#5137=DIRECTION ( 'NONE',  ( 0.000000000000000000, 0.000000000000000000, -1.000000000000000000 ) ) ;
#5146=ORIENTED_EDGE ( 'NONE', *, *, #5790, .T. ) ;
#5147=VERTEX_POINT ( 'NONE', #35630 ) ;
#5152=CARTESIAN_POINT ( 'NONE',  ( 1.776448412236305119, 10.65631784354585498, -99.99999999999995737 ) ) ;
#5153=CARTESIAN_POINT ( 'NONE',  ( 7.070501591499376803E-16, 11.54700538379251284, -156.5000000040968189 ) ) ;
#5154=CARTESIAN_POINT ( 'NONE',  ( 5.405949406249992428, -9.363379034771808662, -166.7812500020484094 ) ) ;
#5155=DIRECTION ( 'NONE',  ( 0.000000000000000000, 0.000000000000000000, 1.000000000000000000 ) ) ;
#5157=CARTESIAN_POINT ( 'NONE',  ( -10.81189881249999907, -6.242252689847864744, -88.96875000204836681 ) ) ;
#5159=CARTESIAN_POINT ( 'NONE',  ( 7.644554776091147741E-16, 12.48450537969573659, -192.9687500020483810 ) ) ;
#5160=CARTESIAN_POINT ( 'NONE',  ( -5.405949406249996869, 9.363379034771805109, -94.03125000204838102 ) ) ;
#5164=CARTESIAN_POINT ( 'NONE',  ( -10.81189881249999729, -6.242252689847864744, -176.1562500020484094 ) ) ;
#5165=CARTESIAN_POINT ( 'NONE',  ( 10.81189881249999907, 6.242252689847868297, -187.4062500020484379 ) ) ;
#5167=CARTESIAN_POINT ( 'NONE',  ( 9.999999999999996447, -5.773502691896262640, -167.5000000040968189 ) ) ;
#5168=CARTESIAN_POINT ( 'NONE',  ( 7.644554776091147741E-16, 12.48450537969573659, -15.96875000204836503 ) ) ;
#5170=CARTESIAN_POINT ( 'NONE',  ( -5.405949406250003975, -9.363379034771801557, -120.3437500020483952 ) ) ;
#5172=CARTESIAN_POINT ( 'NONE',  ( 10.81189881249999729, 0.000000000000000000, -18.03125000204835970 ) ) ;
#5174=CARTESIAN_POINT ( 'NONE',  ( 9.999999999999994671, -5.773502691896262640, -136.0000000040967905 ) ) ;
#5175=CARTESIAN_POINT ( 'NONE',  ( -5.000000000000003553, -8.660254037844383745, -53.49999999999996447 ) ) ;
#5176=CARTESIAN_POINT ( 'NONE',  ( 10.81189881249999907, 6.242252689847868297, -118.4062500020484094 ) ) ;
#5180=CARTESIAN_POINT ( 'NONE',  ( 9.999999999999998224, 0.000000000000000000, -89.37500000409677625 ) ) ;
#5183=CARTESIAN_POINT ( 'NONE',  ( 5.405949406249992428, -9.363379034771808662, -52.59375000204835260 ) ) ;
#5189=CARTESIAN_POINT ( 'NONE',  ( 9.999999999999996447, -5.773502691896262640, -19.00000000409676915 ) ) ;
#5199=DIRECTION ( 'NONE',  ( -1.000000000000000000, 0.000000000000000000, 0.000000000000000000 ) ) ;
#5203=CARTESIAN_POINT ( 'NONE',  ( 10.81189881249999907, 6.242252689847868297, -187.4062500020484379 ) ) ;
#5207=CARTESIAN_POINT ( 'NONE',  ( -10.81189881249999729, 6.242252689847871849, -110.2187500020483810 ) ) ;
#5209=CARTESIAN_POINT ( 'NONE',  ( 5.405949406249992428, -9.363379034771808662, -120.2812500020483952 ) ) ;
#5211=CARTESIAN_POINT ( 'NONE',  ( 5.405949406249992428, -9.363379034771808662, -124.5937500020483952 ) ) ;
#5214=CARTESIAN_POINT ( 'NONE',  ( 9.999999999999998224, 0.000000000000000000, -144.5000000000000000 ) ) ;
#5215=CARTESIAN_POINT ( 'NONE',  ( 9.999999999999998224, 0.000000000000000000, -10.99999999999995381 ) ) ;
#5218=CARTESIAN_POINT ( 'NONE',  ( -9.999999999999998224, 1.224646799147353059E-15, -192.1250000040967905 ) ) ;
#5220=CARTESIAN_POINT ( 'NONE',  ( -5.405949406249996869, 9.363379034771805109, -33.84375000204836681 ) ) ;
#5221=CARTESIAN_POINT ( 'NONE',  ( 9.999999999999998224, 0.000000000000000000, -162.8750000040967905 ) ) ;
#5222=CARTESIAN_POINT ( 'NONE',  ( 5.405949406249999534, 9.363379034771803333, -143.5937500020483810 ) ) ;
#5224=CARTESIAN_POINT ( 'NONE',  ( 9.999999999999479527, 5.773502691896553074, -145.8750000000000000 ) ) ;
#5225=CIRCLE ( 'NONE', #15554, 24.99999999999999645 ) ;
#5226=CARTESIAN_POINT ( 'NONE',  ( 9.999999999999996447, -5.773502691896262640, -77.12499999999998579 ) ) ;
#5227=CARTESIAN_POINT ( 'NONE',  ( -10.81189881249999907, -6.242252689847864744, -140.1562500020484094 ) ) ;
#5232=CARTESIAN_POINT ( 'NONE',  ( 7.644554776091147741E-16, 12.48450537969573659, -101.6562500020483952 ) ) ;
#5233=CARTESIAN_POINT ( 'NONE',  ( 5.000000000000000000, 8.660254037844385522, -116.1250000040967905 ) ) ;
#5234=CARTESIAN_POINT ( 'NONE',  ( -9.999999999999479527, -5.773502691896549521, -140.6250000000000000 ) ) ;
#5235=CARTESIAN_POINT ( 'NONE',  ( -10.81189881249999729, 6.242252689847871849, -77.21875000204838102 ) ) ;
#5238=CARTESIAN_POINT ( 'NONE',  ( -10.81189881249999729, 6.242252689847871849, -45.90625000204836681 ) ) ;
#5239=( BOUNDED_CURVE ( )  B_SPLINE_CURVE ( 2, ( #38706, #36468, #38275, #9140, #8932, #30006, #20057 ),
 .UNSPECIFIED., .F., .F. ) 
 B_SPLINE_CURVE_WITH_KNOTS ( ( 3, 2, 2, 3 ),
 ( 0.4216417910447762818, 0.4228855721393036671, 0.4241293532338309413, 0.4253731343283583266 ),
 .UNSPECIFIED. ) 
 CURVE ( )  GEOMETRIC_REPRESENTATION_ITEM ( )  RATIONAL_B_SPLINE_CURVE ( ( 0.9999999999999820144, 0.8660254037844566932, 1.000000000000000000, 0.8660254037844387076, 1.000000000000000000, 0.8660254037844267172, 1.000000000000011990 ) ) 
 REPRESENTATION_ITEM ( '' )  );
#5240=CARTESIAN_POINT ( 'NONE',  ( 4.999999999999992006, -8.660254037844389075, -137.2499999999999716 ) ) ;
#5246=VERTEX_POINT ( 'NONE', #1380 ) ;
#5248=AXIS2_PLACEMENT_3D ( 'NONE', #22088, #14578, #27766 ) ;
#5250=CARTESIAN_POINT ( 'NONE',  ( -4.999999999999996447, 8.660254037844387298, -135.3750000040967905 ) ) ;
#5257=CARTESIAN_POINT ( 'NONE',  ( 10.81189881249999551, -6.242252689847874514, -136.4687500020483810 ) ) ;
#5258=CARTESIAN_POINT ( 'NONE',  ( -10.81189881249999729, 1.324075727343319199E-15, -138.7812500020483810 ) ) ;
#5259=CARTESIAN_POINT ( 'NONE',  ( 10.81189881249999729, 6.242252689847867408, -151.2187500020484094 ) ) ;
#5260=DIRECTION ( 'NONE',  ( -1.000000000000000000, 0.000000000000000000, 0.000000000000000000 ) ) ;
#5262=CARTESIAN_POINT ( 'NONE',  ( -9.999999999999998224, 1.224646799147353059E-15, -172.2500000000000000 ) ) ;
#5266=CARTESIAN_POINT ( 'NONE',  ( -10.00648583918756884, -2.605931783459911610, -100.0000000000000000 ) ) ;
#5267=CARTESIAN_POINT ( 'NONE',  ( 5.405949406249992428, -9.363379034771808662, -171.0937500020484094 ) ) ;
#5271=CARTESIAN_POINT ( 'NONE',  ( -10.81189881249999907, -6.242252689847864744, -45.65625000204837391 ) ) ;
#5273=CARTESIAN_POINT ( 'NONE',  ( 9.999999999999998224, 0.000000000000000000, -96.49999999999998579 ) ) ;
#5275=CARTESIAN_POINT ( 'NONE',  ( 10.81189881249999729, 0.000000000000000000, -123.0312500020483952 ) ) ;
#5276=CARTESIAN_POINT ( 'NONE',  ( 4.999999999999992006, -8.660254037844389075, -146.6250000040967905 ) ) ;
#5280=CARTESIAN_POINT ( 'NONE',  ( 10.81189881249999729, 0.000000000000000000, -175.3437500020483810 ) ) ;
#5284=CARTESIAN_POINT ( 'NONE',  ( 10.81189881249999729, 0.000000000000000000, -66.03125000204838102 ) ) ;
#5286=CARTESIAN_POINT ( 'NONE',  ( -2.121150477449813534E-15, -11.54700538379251284, -41.75000000409676204 ) ) ;
#5287=CARTESIAN_POINT ( 'NONE',  ( -5.405949406249996869, 9.363379034771805109, -0.8437500020483656993 ) ) ;
#5307=ORIENTED_EDGE ( 'NONE', *, *, #24919, .T. ) ;
#5308=CARTESIAN_POINT ( 'NONE',  ( 9.999999999999227285, 5.773502691896701400, -112.8749999999999716 ) ) ;
#5310=CARTESIAN_POINT ( 'NONE',  ( 7.070501591499377789E-16, 11.54700538379251284, -40.62499999999997158 ) ) ;
#5313=( BOUNDED_CURVE ( )  B_SPLINE_CURVE ( 2, ( #6166, #16264, #9810, #39168, #12825, #29891, #13450 ),
 .UNSPECIFIED., .F., .F. ) 
 B_SPLINE_CURVE_WITH_KNOTS ( ( 3, 2, 2, 3 ),
 ( 0.1828358208955224162, 0.1840796019900497738, 0.1853233830845771313, 0.1865671641791045166 ),
 .UNSPECIFIED. ) 
 CURVE ( )  GEOMETRIC_REPRESENTATION_ITEM ( )  RATIONAL_B_SPLINE_CURVE ( ( 0.9999999999999970024, 0.8660254037844417052, 1.000000000000000000, 0.8660254037844387076, 1.000000000000000000, 0.8660254037844357100, 1.000000000000002887 ) ) 
 REPRESENTATION_ITEM ( '' )  );
#5314=CARTESIAN_POINT ( 'NONE',  ( -5.405949406249996869, 9.363379034771805109, -153.8437500020483810 ) ) ;
#5315=CARTESIAN_POINT ( 'NONE',  ( 10.81189881249999729, 0.000000000000000000, -175.3437500020483810 ) ) ;
#5317=CARTESIAN_POINT ( 'NONE',  ( 7.070501591499377789E-16, 11.54700538379251284, -193.6250000000000000 ) ) ;
#5322=CARTESIAN_POINT ( 'NONE',  ( -10.81189881249999907, -6.242252689847864744, -66.65625000204839523 ) ) ;
#5324=CARTESIAN_POINT ( 'NONE',  ( -9.999999999999998224, 1.224646799147353059E-15, -127.2499999999999716 ) ) ;
#5325=CARTESIAN_POINT ( 'NONE',  ( -5.405949406250003975, -9.363379034771801557, -150.5312500020483810 ) ) ;
#5326=CARTESIAN_POINT ( 'NONE',  ( 7.644554776091147741E-16, 12.48450537969573659, -167.6562500020483810 ) ) ;
#5329=CARTESIAN_POINT ( 'NONE',  ( 10.81189881249999729, 0.000000000000000000, -98.84375000204838102 ) ) ;
#5332=CARTESIAN_POINT ( 'NONE',  ( -10.81189881249999729, 6.242252689847871849, -194.2187500020483810 ) ) ;
#5336=CARTESIAN_POINT ( 'NONE',  ( -5.405949406250003975, -9.363379034771801557, -95.03125000204838102 ) ) ;
#5338=CARTESIAN_POINT ( 'NONE',  ( 10.00000000000000000, 5.773502691896255534, -68.25000000409679046 ) ) ;
#5340=CARTESIAN_POINT ( 'NONE',  ( 10.81189881249999907, 6.242252689847868297, -25.21875000204837747 ) ) ;
#5343=CARTESIAN_POINT ( 'NONE',  ( -5.405949406249996869, 9.363379034771805109, -17.53125000204835970 ) ) ;
#5345=CARTESIAN_POINT ( 'NONE',  ( 9.999999999999872102, 5.773502691896329253, -160.8750000000000000 ) ) ;
#5364=EDGE_CURVE ( 'NONE', #19714, #4329, #35323, .T. ) ;
#5365=ADVANCED_FACE ( 'NONE', ( #3240 ), #39481, .T. ) ;
#5367=CARTESIAN_POINT ( 'NONE',  ( -10.81189881249999907, -6.242252689847864744, -162.6562500020483810 ) ) ;
#5372=CARTESIAN_POINT ( 'NONE',  ( -5.405949406249996869, 9.363379034771805109, -83.34375000204836681 ) ) ;
#5374=CARTESIAN_POINT ( 'NONE',  ( 5.405949406249999534, 9.363379034771803333, -197.5937500020484094 ) ) ;
#5375=CARTESIAN_POINT ( 'NONE',  ( -5.405949406250003975, -9.363379034771801557, -96.53125000204839523 ) ) ;
#5379=CARTESIAN_POINT ( 'NONE',  ( -10.81189881249999729, -6.242252689847864744, -173.1562500020484379 ) ) ;
#5380=CARTESIAN_POINT ( 'NONE',  ( -5.405949406250003975, -9.363379034771801557, -188.0312500020484094 ) ) ;
#5382=CARTESIAN_POINT ( 'NONE',  ( -9.999999999999998224, 1.224646799147353059E-15, -160.6250000040967905 ) ) ;
#5384=CARTESIAN_POINT ( 'NONE',  ( 10.81189881249999729, 0.000000000000000000, -14.84375000204835082 ) ) ;
#5385=CYLINDRICAL_SURFACE ( 'NONE', #35777, 9.999999999999998224 ) ;
#5386=CARTESIAN_POINT ( 'NONE',  ( 5.405949406249999534, 9.363379034771803333, -119.5937500020483810 ) ) ;
#5388=CARTESIAN_POINT ( 'NONE',  ( 10.81189881249999907, 6.242252689847868297, -20.90625000204837747 ) ) ;
#5390=EDGE_CURVE ( 'NONE', #1002, #36790, #8006, .T. ) ;
#5391=CARTESIAN_POINT ( 'NONE',  ( 9.999999999999998224, 0.000000000000000000, -135.8750000040967905 ) ) ;
#5392=CARTESIAN_POINT ( 'NONE',  ( -9.999999999999998224, 5.773502691896259087, -50.87499999999997868 ) ) ;
#5393=CARTESIAN_POINT ( 'NONE',  ( -10.81189881249999729, 6.242252689847871849, -119.4062500020483952 ) ) ;
#5396=CARTESIAN_POINT ( 'NONE',  ( -2.121150477449813534E-15, -11.54700538379251284, -92.75000000409677625 ) ) ;
#5397=DIRECTION ( 'NONE',  ( -1.000000000000000000, 0.000000000000000000, 0.000000000000000000 ) ) ;
#5399=CARTESIAN_POINT ( 'NONE',  ( -5.405949406250003975, -9.363379034771801557, -52.84375000204835970 ) ) ;
#5400=ORIENTED_EDGE ( 'NONE', *, *, #8956, .T. ) ;
#5408=CARTESIAN_POINT ( 'NONE',  ( -4.999999999999996447, 8.660254037844387298, -21.37500000409675494 ) ) ;
#5424=CARTESIAN_POINT ( 'NONE',  ( 5.405949406249999534, 9.363379034771803333, -187.2812500020484094 ) ) ;
#5427=AXIS2_PLACEMENT_3D ( 'NONE', #35737, #42184, #6165 ) ;
#5428=CARTESIAN_POINT ( 'NONE',  ( -5.405949406249996869, 9.363379034771805109, -113.3437500020483810 ) ) ;
#5430=CARTESIAN_POINT ( 'NONE',  ( -5.405949406250003975, -9.363379034771801557, -119.0312500020483952 ) ) ;
#5432=CARTESIAN_POINT ( 'NONE',  ( 5.405949406249999534, 9.363379034771803333, -121.0937500020483952 ) ) ;
#5435=CARTESIAN_POINT ( 'NONE',  ( 5.000000000000000000, 8.660254037844385522, -144.2500000000000000 ) ) ;
#5436=CARTESIAN_POINT ( 'NONE',  ( 10.00000000000000000, 5.773502691896255534, -13.87499999999997158 ) ) ;
#5437=EDGE_CURVE ( 'NONE', #20460, #25374, #33681, .T. ) ;
#5440=CARTESIAN_POINT ( 'NONE',  ( 7.070501591499377789E-16, 11.54700538379251284, -189.5000000040968189 ) ) ;
#5442=CARTESIAN_POINT ( 'NONE',  ( -2.293366432827344421E-15, -12.48450537969573659, -39.21875000204835970 ) ) ;
#5444=CARTESIAN_POINT ( 'NONE',  ( 10.81189881249999551, -6.242252689847874514, -145.4687500020483810 ) ) ;
#5447=CARTESIAN_POINT ( 'NONE',  ( -10.00000000000000000, -5.773502691896251982, -77.62499999999998579 ) ) ;
#5448=CARTESIAN_POINT ( 'NONE',  ( 5.405949406249999534, 9.363379034771803333, -143.7812500020483810 ) ) ;
#5450=ORIENTED_EDGE ( 'NONE', *, *, #35980, .F. ) ;
#5452=CARTESIAN_POINT ( 'NONE',  ( -9.999999999999998224, 1.224646799147353059E-15, -117.1250000040967905 ) ) ;
#5454=CARTESIAN_POINT ( 'NONE',  ( 5.405949406249999534, 9.363379034771803333, -73.09375000204838102 ) ) ;
#5458=CARTESIAN_POINT ( 'NONE',  ( -2.293366432827344421E-15, -12.48450537969573659, -40.90625000204836681 ) ) ;
#5469=AXIS2_PLACEMENT_3D ( 'NONE', #1605, #7863, #21011 ) ;
#5474=CARTESIAN_POINT ( 'NONE',  ( -5.405949406250003975, -9.363379034771801557, -135.3437500020484094 ) ) ;
#5475=CARTESIAN_POINT ( 'NONE',  ( -5.405949406250003975, -9.363379034771801557, -140.0312500020484094 ) ) ;
#5476=( BOUNDED_CURVE ( )  B_SPLINE_CURVE ( 2, ( #9646, #27110, #29935, #26685, #13073, #23030, #20409 ),
 .UNSPECIFIED., .F., .F. ) 
 B_SPLINE_CURVE_WITH_KNOTS ( ( 3, 2, 2, 3 ),
 ( 0.2276119402985075368, 0.2288557213930349221, 0.2300995024875622796, 0.2313432835820896372 ),
 .UNSPECIFIED. ) 
 CURVE ( )  GEOMETRIC_REPRESENTATION_ITEM ( )  RATIONAL_B_SPLINE_CURVE ( ( 0.9999999999999910072, 0.8660254037844477004, 1.000000000000000000, 0.8660254037844387076, 1.000000000000000000, 0.8660254037844297148, 1.000000000000008882 ) ) 
 REPRESENTATION_ITEM ( '' )  );
#5477=CARTESIAN_POINT ( 'NONE',  ( -2.293366432827344421E-15, -12.48450537969573659, -142.7187500020483810 ) ) ;
#5479=CARTESIAN_POINT ( 'NONE',  ( 7.070501591499377789E-16, 11.54700538379251284, -172.6249999999999716 ) ) ;
#5484=CARTESIAN_POINT ( 'NONE',  ( -7.290834969540838983, 7.951501520053491312, -99.99999999999995737 ) ) ;
#5485=CARTESIAN_POINT ( 'NONE',  ( 7.644554776091147741E-16, 12.48450537969573659, -173.4687500020483810 ) ) ;
#5489=CARTESIAN_POINT ( 'NONE',  ( -10.81189881249999907, -6.242252689847864744, -42.65625000204836681 ) ) ;
#5491=CARTESIAN_POINT ( 'NONE',  ( -9.999999999999998224, 1.224646799147353059E-15, -98.74999999999998579 ) ) ;
#5493=CARTESIAN_POINT ( 'NONE',  ( -10.81189881249999729, -6.242252689847864744, -126.6562500020483810 ) ) ;
#5494=CARTESIAN_POINT ( 'NONE',  ( -2.121150477449813534E-15, -11.54700538379251284, -143.7500000040968189 ) ) ;
#5500=CARTESIAN_POINT ( 'NONE',  ( 10.81189881249999551, -6.242252689847874514, -69.15625000204839523 ) ) ;
#5502=CARTESIAN_POINT ( 'NONE',  ( 0.000000000000000000, 0.000000000000000000, -99.99999999999998579 ) ) ;
#5511=ORIENTED_EDGE ( 'NONE', *, *, #19077, .T. ) ;
#5512=CARTESIAN_POINT ( 'NONE',  ( 4.999999999999992006, -8.660254037844389075, -178.1250000040968189 ) ) ;
#5514=ORIENTED_EDGE ( 'NONE', *, *, #29945, .F. ) ;
#5520=VERTEX_POINT ( 'NONE', #20899 ) ;
#5521=CYLINDRICAL_SURFACE ( 'NONE', #27505, 9.999999999999998224 ) ;
#5522=CARTESIAN_POINT ( 'NONE',  ( -2.121150477449813534E-15, -11.54700538379251284, -33.87499999999995737 ) ) ;
#5525=CARTESIAN_POINT ( 'NONE',  ( 10.81189881249999907, 6.242252689847868297, -161.7187500020483810 ) ) ;
#5526=CARTESIAN_POINT ( 'NONE',  ( 5.405949406249999534, 9.363379034771803333, -172.0937500020484094 ) ) ;
#5530=CARTESIAN_POINT ( 'NONE',  ( 5.000000000000000000, 8.660254037844385522, -198.2500000000000000 ) ) ;
#5535=CARTESIAN_POINT ( 'NONE',  ( -5.405949406249996869, 9.363379034771805109, -70.03125000204838102 ) ) ;
#5537=CARTESIAN_POINT ( 'NONE',  ( 4.999999999999992006, -8.660254037844389075, -122.2500000000000000 ) ) ;
#5538=EDGE_LOOP ( 'NONE', ( #37836, #18432, #17220, #37888 ) ) ;
#5539=CARTESIAN_POINT ( 'NONE',  ( 10.81189881249999729, 0.000000000000000000, -148.5312500020483810 ) ) ;
#5540=CARTESIAN_POINT ( 'NONE',  ( -10.81189881249999729, 1.324075727343319199E-15, -161.2812500020484094 ) ) ;
#5542=CYLINDRICAL_SURFACE ( 'NONE', #2716, 9.999999999999998224 ) ;
#5543=CARTESIAN_POINT ( 'NONE',  ( -10.81189881249999907, -6.242252689847864744, -94.96875000204838102 ) ) ;
#5546=CARTESIAN_POINT ( 'NONE',  ( 5.405949406249999534, 9.363379034771803333, -197.5937500020484094 ) ) ;
#5548=CARTESIAN_POINT ( 'NONE',  ( -0.03154043146628307537, -10.44038505333712052, -179.9999999999999716 ) ) ;
#5550=CARTESIAN_POINT ( 'NONE',  ( 5.405949406249992428, -9.363379034771808662, -88.78125000204838102 ) ) ;
#5552=CARTESIAN_POINT ( 'NONE',  ( 7.070501591499377789E-16, 11.54700538379251284, -66.50000000409677625 ) ) ;
#5553=DIRECTION ( 'NONE',  ( -1.000000000000000000, 0.000000000000000000, 0.000000000000000000 ) ) ;
#5554=CARTESIAN_POINT ( 'NONE',  ( -5.405949406249996869, 9.363379034771805109, -27.84375000204836326 ) ) ;
#5558=CARTESIAN_POINT ( 'NONE',  ( 10.81189881249999551, -6.242252689847874514, -16.65625000204837391 ) ) ;
#5559=EDGE_CURVE ( 'NONE', #31328, #35190, #4941, .T. ) ;
#5567=CARTESIAN_POINT ( 'NONE',  ( 10.00000000000038014, -5.773502691896040595, -179.5000000040967620 ) ) ;
#5570=VERTEX_POINT ( 'NONE', #27819 ) ;
#5576=CARTESIAN_POINT ( 'NONE',  ( -2.121150477449813534E-15, -11.54700538379251284, -127.2500000040967763 ) ) ;
#5578=CARTESIAN_POINT ( 'NONE',  ( -10.81189881249999907, -6.242252689847864744, -164.1562500020484094 ) ) ;
#5580=CARTESIAN_POINT ( 'NONE',  ( 9.999999999999866773, -5.773502691896336358, -172.0000000040967620 ) ) ;
#5584=CARTESIAN_POINT ( 'NONE',  ( 5.405949406249992428, -9.363379034771808662, -82.59375000204836681 ) ) ;
#5585=CARTESIAN_POINT ( 'NONE',  ( 10.81189881249999907, 6.242252689847868297, -191.7187500020484094 ) ) ;
#5586=CARTESIAN_POINT ( 'NONE',  ( 7.644554776091147741E-16, 12.48450537969573659, -95.65625000204838102 ) ) ;
#5590=CARTESIAN_POINT ( 'NONE',  ( -10.81189881249999729, -6.242252689847864744, -171.6562500020484094 ) ) ;
#5591=CARTESIAN_POINT ( 'NONE',  ( 5.405949406249999534, 9.363379034771803333, -191.7812500020484094 ) ) ;
#5593=CARTESIAN_POINT ( 'NONE',  ( -9.999999999999998224, 1.224646799147353059E-15, -163.6250000040967905 ) ) ;
#5595=CARTESIAN_POINT ( 'NONE',  ( 7.644554776091147741E-16, 12.48450537969573659, -17.46875000204836681 ) ) ;
#5597=CARTESIAN_POINT ( 'NONE',  ( 5.405949406249999534, 9.363379034771803333, -122.5937500020483952 ) ) ;
#5599=CARTESIAN_POINT ( 'NONE',  ( -5.405949406250003975, -9.363379034771801557, -23.03125000204836326 ) ) ;
#5601=CARTESIAN_POINT ( 'NONE',  ( -9.999999999999998224, 1.224646799147353059E-15, -157.6250000040967905 ) ) ;
#5602=CARTESIAN_POINT ( 'NONE',  ( -10.81189881249999729, 6.242252689847871849, -113.4062500020483810 ) ) ;
#5604=ORIENTED_EDGE ( 'NONE', *, *, #20666, .F. ) ;
#5605=CARTESIAN_POINT ( 'NONE',  ( -10.00000000000000000, -5.773502691896251982, -88.50000000409679046 ) ) ;
#5608=CARTESIAN_POINT ( 'NONE',  ( -2.293366432827344421E-15, -12.48450537969573659, -51.21875000204836681 ) ) ;
#5614=CARTESIAN_POINT ( 'NONE',  ( 4.999999999999992006, -8.660254037844389075, -22.12500000409675494 ) ) ;
#5621=ORIENTED_EDGE ( 'NONE', *, *, #35493, .T. ) ;
#5622=CARTESIAN_POINT ( 'NONE',  ( 7.070501591499376803E-16, 11.54700538379251284, -143.0000000040967905 ) ) ;
#5632=CARTESIAN_POINT ( 'NONE',  ( 9.999999999999998224, 0.000000000000000000, -176.0000000000000000 ) ) ;
#5635=CARTESIAN_POINT ( 'NONE',  ( -10.81189881249999729, 6.242252689847871849, -189.9062500020484379 ) ) ;
#5637=CYLINDRICAL_SURFACE ( 'NONE', #17619, 9.999999999999998224 ) ;
#5640=CARTESIAN_POINT ( 'NONE',  ( -10.81189881249999729, 6.242252689847871849, -113.2187500020483952 ) ) ;
#5641=CARTESIAN_POINT ( 'NONE',  ( 10.00000000000051159, -5.773502691895965988, -149.5000000040967905 ) ) ;
#5642=CARTESIAN_POINT ( 'NONE',  ( -5.405949406249996869, 9.363379034771805109, -116.5312500020483952 ) ) ;
#5644=CARTESIAN_POINT ( 'NONE',  ( -5.405949406250003975, -9.363379034771801557, -121.8437500020483952 ) ) ;
#5648=CARTESIAN_POINT ( 'NONE',  ( -2.121150477449813534E-15, -11.54700538379251284, -150.8750000000000284 ) ) ;
#5649=CARTESIAN_POINT ( 'NONE',  ( -5.000000000000003553, -8.660254037844383745, -15.99999999999995914 ) ) ;
#5653=CARTESIAN_POINT ( 'NONE',  ( 9.999999999999998224, 0.000000000000000000, -188.3750000040967905 ) ) ;
#5655=CARTESIAN_POINT ( 'NONE',  ( 5.405949406249999534, 9.363379034771803333, -37.09375000204836681 ) ) ;
#5657=CARTESIAN_POINT ( 'NONE',  ( 10.81189881249999907, 6.242252689847868297, -145.2187500020484094 ) ) ;
#5659=CARTESIAN_POINT ( 'NONE',  ( 9.999999999999998224, 0.000000000000000000, -101.3750000040967905 ) ) ;
#5660=CARTESIAN_POINT ( 'NONE',  ( 5.000000000000000000, 8.660254037844385522, -75.24999999999998579 ) ) ;
#5661=CARTESIAN_POINT ( 'NONE',  ( 10.81189881249999551, -6.242252689847874514, -142.6562500020484094 ) ) ;
#5665=CARTESIAN_POINT ( 'NONE',  ( -9.999999999999998224, 5.773502691896259087, -112.7500000040967763 ) ) ;
#5666=CARTESIAN_POINT ( 'NONE',  ( 7.644554776091147741E-16, 12.48450537969573659, -77.46875000204838102 ) ) ;
#5673=CARTESIAN_POINT ( 'NONE',  ( 5.405949406249999534, 9.363379034771803333, -34.28125000204837391 ) ) ;
#5683=VECTOR ( 'NONE', #19780, 1000.000000000000000 ) ;
#5684=ORIENTED_EDGE ( 'NONE', *, *, #41197, .T. ) ;
#5686=EDGE_CURVE ( 'NONE', #25155, #24776, #15277, .T. ) ;
#5691=DIRECTION ( 'NONE',  ( -0.000000000000000000, -0.000000000000000000, -1.000000000000000000 ) ) ;
#5695=CARTESIAN_POINT ( 'NONE',  ( 10.81189881249999907, 6.242252689847868297, -134.7187500020484094 ) ) ;
#5696=CARTESIAN_POINT ( 'NONE',  ( -5.405949406249996869, 9.363379034771805109, -140.5312500020484094 ) ) ;
#5697=CARTESIAN_POINT ( 'NONE',  ( 5.000000000000000000, 8.660254037844385522, -104.1250000040967763 ) ) ;
#5698=CARTESIAN_POINT ( 'NONE',  ( -5.405949406249996869, 9.363379034771805109, -146.3437500020483810 ) ) ;
#5699=CARTESIAN_POINT ( 'NONE',  ( 9.999999999999479527, 5.773502691896553074, -127.8749999999999858 ) ) ;
#5701=CARTESIAN_POINT ( 'NONE',  ( -5.000000000000003553, -8.660254037844383745, -169.0000000000000000 ) ) ;
#5706=CARTESIAN_POINT ( 'NONE',  ( 5.405949406249992428, -9.363379034771808662, -172.5937500020484094 ) ) ;
#5710=CARTESIAN_POINT ( 'NONE',  ( -10.81189881249999729, 6.242252689847871849, -33.90625000204835970 ) ) ;
#5712=CARTESIAN_POINT ( 'NONE',  ( -9.999999999999998224, 5.773502691896259087, -97.37500000000000000 ) ) ;
#5714=CARTESIAN_POINT ( 'NONE',  ( 10.81189881249999729, 6.242252689847867408, -121.4062500020483810 ) ) ;
#5715=CARTESIAN_POINT ( 'NONE',  ( 10.00000000000000000, 5.773502691896255534, -138.7500000040967905 ) ) ;
#5720=CARTESIAN_POINT ( 'NONE',  ( -10.81189881249999729, 6.242252689847871849, -56.40625000204838813 ) ) ;
#5731=CARTESIAN_POINT ( 'NONE',  ( -9.999999999999998224, 1.224646799147353059E-15, -178.6250000040968189 ) ) ;
#5739=CARTESIAN_POINT ( 'NONE',  ( -2.121150477449813534E-15, -11.54700538379251284, -112.2500000040967763 ) ) ;
#5740=CARTESIAN_POINT ( 'NONE',  ( 7.070501591499377789E-16, 11.54700538379251284, -37.62499999999996447 ) ) ;
#5743=CARTESIAN_POINT ( 'NONE',  ( -5.405949406249996869, 9.363379034771805109, -156.8437500020483810 ) ) ;
#5744=CARTESIAN_POINT ( 'NONE',  ( 5.405949406249999534, 9.363379034771803333, -173.5937500020484094 ) ) ;
#5746=CARTESIAN_POINT ( 'NONE',  ( -10.00000000000102496, 5.773502691895664007, -131.8749999999999432 ) ) ;
#5747=CARTESIAN_POINT ( 'NONE',  ( -5.000000000000003553, -8.660254037844383745, -193.0000000000000000 ) ) ;
#5752=CARTESIAN_POINT ( 'NONE',  ( 10.81189881249999551, -6.242252689847874514, -61.65625000204838813 ) ) ;
#5754=CARTESIAN_POINT ( 'NONE',  ( 7.070501591499377789E-16, 11.54700538379251284, -124.6249999999999858 ) ) ;
#5756=CARTESIAN_POINT ( 'NONE',  ( 7.644554776091147741E-16, 12.48450537969573659, -142.1562500020484094 ) ) ;
#5757=CARTESIAN_POINT ( 'NONE',  ( -10.81189881249999729, 6.242252689847871849, -155.4062500020483810 ) ) ;
#5759=CARTESIAN_POINT ( 'NONE',  ( -10.00000000000076916, 5.773502691895813221, -104.8749999999999716 ) ) ;
#5760=CARTESIAN_POINT ( 'NONE',  ( 10.81189881249999551, -6.242252689847874514, -86.96875000204838102 ) ) ;
#5763=CARTESIAN_POINT ( 'NONE',  ( 10.81189881249999907, 6.242252689847868297, -196.2187500020484094 ) ) ;
#5767=CARTESIAN_POINT ( 'NONE',  ( 10.81189881249999729, 0.000000000000000000, -88.53125000204838102 ) ) ;
#5769=CARTESIAN_POINT ( 'NONE',  ( -2.121150477449813534E-15, -11.54700538379251284, -65.75000000409679046 ) ) ;
#5771=CARTESIAN_POINT ( 'NONE',  ( 5.405949406249992428, -9.363379034771808662, -27.09375000204835970 ) ) ;
#5774=CARTESIAN_POINT ( 'NONE',  ( -5.405949406249996869, 9.363379034771805109, -23.53125000204836681 ) ) ;
#5785=ORIENTED_EDGE ( 'NONE', *, *, #16511, .F. ) ;
#5790=EDGE_CURVE ( 'NONE', #18722, #6299, #8813, .T. ) ;
#5794=CARTESIAN_POINT ( 'NONE',  ( -5.405949406250003975, -9.363379034771801557, -156.5312500020484094 ) ) ;
#5799=CARTESIAN_POINT ( 'NONE',  ( 10.81189881249999551, -6.242252689847874514, -76.46875000204838102 ) ) ;
#5800=CARTESIAN_POINT ( 'NONE',  ( 10.81189881249999907, 6.242252689847868297, -88.40625000204839523 ) ) ;
#5802=LINE ( 'NONE', #19376, #19926 ) ;
#5803=CARTESIAN_POINT ( 'NONE',  ( -2.293366432827344421E-15, -12.48450537969573659, -171.4062500020484379 ) ) ;
#5804=CARTESIAN_POINT ( 'NONE',  ( -5.405949406250003975, -9.363379034771801557, -185.0312500020484094 ) ) ;
#5806=CARTESIAN_POINT ( 'NONE',  ( -5.000000000000003553, -8.660254037844383745, -166.3750000040967905 ) ) ;
#5808=CARTESIAN_POINT ( 'NONE',  ( 10.81189881249999551, -6.242252689847874514, -14.96875000204836503 ) ) ;
#5809=CARTESIAN_POINT ( 'NONE',  ( 9.999999999999998224, 0.000000000000000000, -156.5000000000000000 ) ) ;
#5810=CARTESIAN_POINT ( 'NONE',  ( -5.405949406249996869, 9.363379034771805109, -125.3437500020483952 ) ) ;
#5812=CARTESIAN_POINT ( 'NONE',  ( 10.81189881249999729, 0.000000000000000000, -22.53125000204836326 ) ) ;
#5815=CARTESIAN_POINT ( 'NONE',  ( 5.405949406249992428, -9.363379034771808662, -114.2812500020483952 ) ) ;
#5818=CARTESIAN_POINT ( 'NONE',  ( 10.00000000000000000, 5.773502691896255534, -95.25000000409679046 ) ) ;
#5821=CARTESIAN_POINT ( 'NONE',  ( 10.81189881249999729, 0.000000000000000000, -52.34375000204835260 ) ) ;
#5827=CARTESIAN_POINT ( 'NONE',  ( -9.999999999999998224, 1.224646799147353059E-15, -21.12500000409675494 ) ) ;
#5830=VERTEX_POINT ( 'NONE', #24812 ) ;
#5839=CARTESIAN_POINT ( 'NONE',  ( -9.999999999999998224, 1.224646799147353059E-15, -166.6250000040967905 ) ) ;
#5841=CARTESIAN_POINT ( 'NONE',  ( -10.81189881249999729, 1.324075727343319199E-15, -179.2812500020484094 ) ) ;
#5843=CARTESIAN_POINT ( 'NONE',  ( 9.999999999999998224, 0.000000000000000000, -131.0000000000000000 ) ) ;
#5847=CARTESIAN_POINT ( 'NONE',  ( 10.81189881249999551, -6.242252689847874514, -106.4687500020483810 ) ) ;
#5849=CARTESIAN_POINT ( 'NONE',  ( -5.405949406249996869, 9.363379034771805109, -113.5312500020483952 ) ) ;
#5851=CARTESIAN_POINT ( 'NONE',  ( 10.81189881249999551, -6.242252689847874514, -119.9687500020483952 ) ) ;
#5853=VECTOR ( 'NONE', #27951, 1000.000000000000000 ) ;
#5854=CARTESIAN_POINT ( 'NONE',  ( -9.999999999999998224, 1.224646799147353059E-15, -157.2500000000000000 ) ) ;
#5855=CARTESIAN_POINT ( 'NONE',  ( 10.00000000000000000, 5.773502691896255534, -136.8750000000000000 ) ) ;
#5856=CARTESIAN_POINT ( 'NONE',  ( -5.000000000000003553, -8.660254037844383745, -14.49999999999995737 ) ) ;
#5859=CARTESIAN_POINT ( 'NONE',  ( -5.000000000000003553, -8.660254037844383745, -185.8750000040967905 ) ) ;
#5861=CARTESIAN_POINT ( 'NONE',  ( -10.81189881249999729, 6.242252689847871849, -41.21875000204835970 ) ) ;
#5863=CARTESIAN_POINT ( 'NONE',  ( 5.405949406249999534, 9.363379034771803333, -149.5937500020483810 ) ) ;
#5865=CARTESIAN_POINT ( 'NONE',  ( 7.070501591499376803E-16, 11.54700538379251284, -136.6250000000000000 ) ) ;
#5866=CARTESIAN_POINT ( 'NONE',  ( 10.00000000000000000, 5.773502691896255534, -64.87499999999998579 ) ) ;
#5867=CARTESIAN_POINT ( 'NONE',  ( -10.81189881249999729, 6.242252689847871849, -143.4062500020484094 ) ) ;
#5872=CARTESIAN_POINT ( 'NONE',  ( 9.999999999999998224, 0.000000000000000000, -119.3750000040967905 ) ) ;
#5873=CARTESIAN_POINT ( 'NONE',  ( -4.999999999999996447, 8.660254037844387298, -169.5000000000000000 ) ) ;
#5874=CARTESIAN_POINT ( 'NONE',  ( 10.81189881249999551, -6.242252689847874514, -76.46875000204838102 ) ) ;
#5879=CARTESIAN_POINT ( 'NONE',  ( -10.81189881249999729, 6.242252689847871849, -35.40625000204835970 ) ) ;
#5884=CARTESIAN_POINT ( 'NONE',  ( 9.999999999999998224, 0.000000000000000000, -164.3750000040967905 ) ) ;
#5893=EDGE_CURVE ( 'NONE', #30027, #3790, #15744, .T. ) ;
#5898=CARTESIAN_POINT ( 'NONE',  ( 5.405949406249999534, 9.363379034771803333, -134.5937500020483810 ) ) ;
#5899=VECTOR ( 'NONE', #17979, 1000.000000000000000 ) ;
#5900=CARTESIAN_POINT ( 'NONE',  ( 5.405949406249999534, 9.363379034771803333, -137.7812500020483810 ) ) ;
#5902=CARTESIAN_POINT ( 'NONE',  ( -10.81189881249999729, -6.242252689847864744, -148.9687500020484094 ) ) ;
#5903=ADVANCED_FACE ( 'NONE', ( #15897 ), #6009, .F. ) ;
#5906=CARTESIAN_POINT ( 'NONE',  ( -9.999999999999998224, 1.224646799147353059E-15, -164.7500000000000000 ) ) ;
#5908=DIRECTION ( 'NONE',  ( -0.000000000000000000, -0.000000000000000000, -1.000000000000000000 ) ) ;
#5910=CARTESIAN_POINT ( 'NONE',  ( -2.293366432827344421E-15, -12.48450537969573659, -58.71875000204837391 ) ) ;
#5911=CARTESIAN_POINT ( 'NONE',  ( 9.999999999999998224, 1.224646799147353059E-15, -99.99999999999998579 ) ) ;
#5912=CARTESIAN_POINT ( 'NONE',  ( 7.644554776091147741E-16, 12.48450537969573659, -168.9687500020483810 ) ) ;
#5919=CARTESIAN_POINT ( 'NONE',  ( 5.000000000000000000, 8.660254037844385522, -96.24999999999998579 ) ) ;
#5921=CARTESIAN_POINT ( 'NONE',  ( -10.81189881249999729, -6.242252689847864744, -122.1562500020483810 ) ) ;
#5922=CARTESIAN_POINT ( 'NONE',  ( 4.999999999999992006, -8.660254037844389075, -142.1250000040967905 ) ) ;
#5927=CARTESIAN_POINT ( 'NONE',  ( 5.405949406249992428, -9.363379034771808662, -63.28125000204837391 ) ) ;
#5952=CARTESIAN_POINT ( 'NONE',  ( 7.070501591499377789E-16, 11.54700538379251284, -27.12499999999998224 ) ) ;
#5955=CARTESIAN_POINT ( 'NONE',  ( -10.81189881249999729, 6.242252689847871849, -161.2187500020483526 ) ) ;
#5956=CARTESIAN_POINT ( 'NONE',  ( 5.405949406249992428, -9.363379034771808662, -169.5937500020484094 ) ) ;
#5959=CARTESIAN_POINT ( 'NONE',  ( 9.999999999999998224, 0.000000000000000000, -191.0000000000000000 ) ) ;
#5963=CIRCLE ( 'NONE', #5248, 22.00000000000000711 ) ;
#5964=CARTESIAN_POINT ( 'NONE',  ( 7.644554776091147741E-16, 12.48450537969573659, -58.15625000204838102 ) ) ;
#5966=CARTESIAN_POINT ( 'NONE',  ( 4.999999999999992006, -8.660254037844389075, -123.7500000000000000 ) ) ;
#5968=CARTESIAN_POINT ( 'NONE',  ( -2.293366432827344421E-15, -12.48450537969573659, -145.9062500020484094 ) ) ;
#5969=CARTESIAN_POINT ( 'NONE',  ( -2.293366432827344421E-15, -12.48450537969573659, -159.4062500020483810 ) ) ;
#5973=CARTESIAN_POINT ( 'NONE',  ( 7.644554776091147741E-16, 12.48450537969573659, -90.96875000204838102 ) ) ;
#5976=CARTESIAN_POINT ( 'NONE',  ( 5.405949406249999534, 9.363379034771803333, -188.5937500020483810 ) ) ;
#5980=CARTESIAN_POINT ( 'NONE',  ( 10.81189881249999729, 0.000000000000000000, -85.53125000204838102 ) ) ;
#5982=CARTESIAN_POINT ( 'NONE',  ( -10.00000000000000000, -5.773502691896251982, -60.00000000409677625 ) ) ;
#5983=CARTESIAN_POINT ( 'NONE',  ( 10.81189881249999551, -6.242252689847874514, -14.96875000204836503 ) ) ;
#5986=CARTESIAN_POINT ( 'NONE',  ( 5.405949406249999534, 9.363379034771803333, -8.781250002048352599 ) ) ;
#5988=CARTESIAN_POINT ( 'NONE',  ( -4.999999999999996447, 8.660254037844387298, -136.8750000040967905 ) ) ;
#6005=CARTESIAN_POINT ( 'NONE',  ( -9.999999999999227285, -5.773502691896698735, -127.5000000040967763 ) ) ;
#6006=CARTESIAN_POINT ( 'NONE',  ( 7.070501591499376803E-16, 11.54700538379251284, -129.1250000000000000 ) ) ;
#6007=CARTESIAN_POINT ( 'NONE',  ( 10.81189881249999907, 6.242252689847868297, -157.4062500020483810 ) ) ;
#6009=CYLINDRICAL_SURFACE ( 'NONE', #18442, 9.999999999999998224 ) ;
#6013=CARTESIAN_POINT ( 'NONE',  ( 10.81189881249999907, 6.242252689847868297, -76.21875000204836681 ) ) ;
#6014=CARTESIAN_POINT ( 'NONE',  ( 10.81189881249999551, -6.242252689847874514, -87.15625000204838102 ) ) ;
#6017=CARTESIAN_POINT ( 'NONE',  ( 5.405949406249992428, -9.363379034771808662, -168.2812500020484094 ) ) ;
#6018=CARTESIAN_POINT ( 'NONE',  ( 10.81189881249999551, -6.242252689847874514, -178.6562500020484094 ) ) ;
#6020=CARTESIAN_POINT ( 'NONE',  ( -9.999999999999998224, 1.224646799147353059E-15, -154.6250000040967905 ) ) ;
#6022=CARTESIAN_POINT ( 'NONE',  ( -10.81189881249999729, 6.242252689847871849, -6.718750002048357040 ) ) ;
#6024=CARTESIAN_POINT ( 'NONE',  ( 10.81189881249999907, 6.242252689847868297, -110.7187500020483810 ) ) ;
#6026=CARTESIAN_POINT ( 'NONE',  ( 5.405949406249992428, -9.363379034771808662, -10.78125000204835438 ) ) ;
#6029=CARTESIAN_POINT ( 'NONE',  ( 10.81189881249999551, -6.242252689847874514, -108.1562500020483810 ) ) ;
#6032=CARTESIAN_POINT ( 'NONE',  ( -9.999999999999998224, 5.773502691896259087, -93.25000000409677625 ) ) ;
#6034=CARTESIAN_POINT ( 'NONE',  ( 7.644554776091147741E-16, 12.48450537969573659, -42.96875000204835970 ) ) ;
#6035=ORIENTED_EDGE ( 'NONE', *, *, #34843, .T. ) ;
#6039=CARTESIAN_POINT ( 'NONE',  ( -10.00000000000000000, -5.773502691896251982, -19.50000000409676915 ) ) ;
#6050=ORIENTED_EDGE ( 'NONE', *, *, #33285, .T. ) ;
#6054=CARTESIAN_POINT ( 'NONE',  ( -2.293366432827344421E-15, -12.48450537969573659, -183.4062500020483810 ) ) ;
#6056=CARTESIAN_POINT ( 'NONE',  ( -9.999999999999998224, 1.224646799147353059E-15, -161.7500000000000000 ) ) ;
#6059=CARTESIAN_POINT ( 'NONE',  ( 5.405949406249999534, 9.363379034771803333, -104.5937500020483810 ) ) ;
#6061=CARTESIAN_POINT ( 'NONE',  ( 10.81189881249999907, 6.242252689847868297, -109.4062500020483952 ) ) ;
#6063=CARTESIAN_POINT ( 'NONE',  ( -2.293366432827344421E-15, -12.48450537969573659, -121.7187500020483952 ) ) ;
#6065=EDGE_CURVE ( 'NONE', #32933, #16776, #12966, .T. ) ;
#6067=CARTESIAN_POINT ( 'NONE',  ( 9.999999999999998224, 0.000000000000000000, -135.5000000000000000 ) ) ;
#6068=CARTESIAN_POINT ( 'NONE',  ( -5.000000000000003553, -8.660254037844383745, -8.499999999999952038 ) ) ;
#6072=CARTESIAN_POINT ( 'NONE',  ( 4.999999999999992006, -8.660254037844389075, -178.1250000040968189 ) ) ;
#6075=CARTESIAN_POINT ( 'NONE',  ( -5.405949406250003975, -9.363379034771801557, -25.84375000204835970 ) ) ;
#6076=CARTESIAN_POINT ( 'NONE',  ( 9.999999999999998224, 0.000000000000000000, -117.5000000000000000 ) ) ;
#6077=CARTESIAN_POINT ( 'NONE',  ( -10.81189881249999907, -6.242252689847864744, -139.9687500020483810 ) ) ;
#6081=CARTESIAN_POINT ( 'NONE',  ( -4.999999999999996447, 8.660254037844387298, -67.49999999999997158 ) ) ;
#6082=CARTESIAN_POINT ( 'NONE',  ( -10.81189881249999907, -6.242252689847864744, -143.1562500020484094 ) ) ;
#6086=CARTESIAN_POINT ( 'NONE',  ( 10.00000000000000000, 5.773502691896255534, -119.2500000040967905 ) ) ;
#6088=CARTESIAN_POINT ( 'NONE',  ( 7.644554776091147741E-16, 12.48450537969573659, -72.96875000204835260 ) ) ;
#6093=CARTESIAN_POINT ( 'NONE',  ( -9.999999999999998224, 5.773502691896259087, -46.75000000409676915 ) ) ;
#6094=CARTESIAN_POINT ( 'NONE',  ( 10.81189881249999729, 0.000000000000000000, -33.03125000204837391 ) ) ;
#6095=DIRECTION ( 'NONE',  ( -0.000000000000000000, -0.000000000000000000, -1.000000000000000000 ) ) ;
#6101=ORIENTED_EDGE ( 'NONE', *, *, #26161, .F. ) ;
#6103=ORIENTED_EDGE ( 'NONE', *, *, #1721, .F. ) ;
#6110=CARTESIAN_POINT ( 'NONE',  ( -10.81189881249999729, 1.324075727343319199E-15, -128.0937500020483810 ) ) ;
#6111=CARTESIAN_POINT ( 'NONE',  ( -10.81189881249999907, -6.242252689847864744, -131.1562500020483810 ) ) ;
#6113=CARTESIAN_POINT ( 'NONE',  ( -5.405949406249996869, 9.363379034771805109, -147.8437500020483810 ) ) ;
#6114=LINE ( 'NONE', #39961, #12282 ) ;
#6117=CARTESIAN_POINT ( 'NONE',  ( -5.000000000000003553, -8.660254037844383745, -166.0000000000000000 ) ) ;
#6120=CARTESIAN_POINT ( 'NONE',  ( 7.644554776091147741E-16, 12.48450537969573659, -63.96875000204837391 ) ) ;
#6121=CARTESIAN_POINT ( 'NONE',  ( -2.121150477449813534E-15, -11.54700538379251284, -174.8750000000000000 ) ) ;
#6122=CARTESIAN_POINT ( 'NONE',  ( 7.644554776091147741E-16, 12.48450537969573659, -171.9687500020483810 ) ) ;
#6125=DIRECTION ( 'NONE',  ( -0.000000000000000000, -0.000000000000000000, -1.000000000000000000 ) ) ;
#6127=CARTESIAN_POINT ( 'NONE',  ( 5.000000000000000000, 8.660254037844385522, -94.74999999999998579 ) ) ;
#6130=CARTESIAN_POINT ( 'NONE',  ( -2.293366432827344421E-15, -12.48450537969573659, -120.4062500020483952 ) ) ;
#6131=CARTESIAN_POINT ( 'NONE',  ( 7.070501591499377789E-16, 11.54700538379251284, -143.0000000040967905 ) ) ;
#6132=CARTESIAN_POINT ( 'NONE',  ( 9.999999999999998224, 0.000000000000000000, -152.0000000000000000 ) ) ;
#6136=DIRECTION ( 'NONE',  ( -1.000000000000000000, 0.000000000000000000, 0.000000000000000000 ) ) ;
#6137=CARTESIAN_POINT ( 'NONE',  ( 10.81189881249999551, -6.242252689847874514, -58.65625000204838813 ) ) ;
#6148=VECTOR ( 'NONE', #2459, 1000.000000000000000 ) ;
#6159=CARTESIAN_POINT ( 'NONE',  ( 4.999999999999992006, -8.660254037844389075, -30.74999999999997158 ) ) ;
#6163=CARTESIAN_POINT ( 'NONE',  ( 10.81189881249999729, 0.000000000000000000, -155.8437500020483810 ) ) ;
#6164=CARTESIAN_POINT ( 'NONE',  ( 10.81189881249999729, 6.242252689847867408, -172.2187500020483810 ) ) ;
#6165=DIRECTION ( 'NONE',  ( -1.000000000000000000, 0.000000000000000000, 0.000000000000000000 ) ) ;
#6166=CARTESIAN_POINT ( 'NONE',  ( -9.999999999999998224, 1.224646799147353059E-15, -162.1250000040967905 ) ) ;
#6167=CARTESIAN_POINT ( 'NONE',  ( 9.999999999999998224, 0.000000000000000000, -189.5000000000000000 ) ) ;
#6173=EDGE_CURVE ( 'NONE', #9851, #8327, #35073, .T. ) ;
#6174=CARTESIAN_POINT ( 'NONE',  ( -10.81189881249999729, 1.324075727343319199E-15, -63.78125000204837391 ) ) ;
#6176=CARTESIAN_POINT ( 'NONE',  ( -9.999999999999998224, 5.773502691896259087, -116.8750000000000000 ) ) ;
#6179=CARTESIAN_POINT ( 'NONE',  ( 5.405949406249999534, 9.363379034771803333, -145.2812500020483810 ) ) ;
#6180=CARTESIAN_POINT ( 'NONE',  ( -10.81189881249999729, 6.242252689847871849, -156.9062500020483810 ) ) ;
#6183=CARTESIAN_POINT ( 'NONE',  ( 7.644554776091147741E-16, 12.48450537969573659, -87.96875000204838102 ) ) ;
#6186=CARTESIAN_POINT ( 'NONE',  ( 5.405949406249999534, 9.363379034771803333, -191.5937500020484094 ) ) ;
#6189=CARTESIAN_POINT ( 'NONE',  ( 5.000000000000000000, 8.660254037844385522, -140.1250000040967905 ) ) ;
#6190=CARTESIAN_POINT ( 'NONE',  ( -2.293366432827344421E-15, -12.48450537969573659, -84.40625000204838102 ) ) ;
#6192=CARTESIAN_POINT ( 'NONE',  ( 7.070501591499377789E-16, 11.54700538379251284, -62.00000000409678336 ) ) ;
#6193=CARTESIAN_POINT ( 'NONE',  ( 10.81189881249999729, 0.000000000000000000, -19.34375000204835260 ) ) ;
#6196=CARTESIAN_POINT ( 'NONE',  ( 7.644554776091147741E-16, 12.48450537969573659, -14.65625000204837214 ) ) ;
#6198=CARTESIAN_POINT ( 'NONE',  ( -9.999999999999998224, 1.224646799147353059E-15, -160.2500000000000000 ) ) ;
#6208=ORIENTED_EDGE ( 'NONE', *, *, #9328, .F. ) ;
#6209=CARTESIAN_POINT ( 'NONE',  ( -9.999999999999998224, 1.224646799147353059E-15, -169.6250000040967905 ) ) ;
#6210=VERTEX_POINT ( 'NONE', #4669 ) ;
#6211=EDGE_LOOP ( 'NONE', ( #7741, #33440, #25469, #31095 ) ) ;
#6217=CARTESIAN_POINT ( 'NONE',  ( 10.25440575037869273, 0.6849317685095945851, -100.0000000000000142 ) ) ;
#6221=CARTESIAN_POINT ( 'NONE',  ( -10.81189881249999907, -6.242252689847864744, -155.1562500020484094 ) ) ;
#6227=CARTESIAN_POINT ( 'NONE',  ( -5.405949406249996869, 9.363379034771805109, -80.34375000204838102 ) ) ;
#6228=CARTESIAN_POINT ( 'NONE',  ( -10.81189881249999729, 6.242252689847871849, -87.90625000204838102 ) ) ;
#6231=CARTESIAN_POINT ( 'NONE',  ( -10.81189881249999729, -6.242252689847864744, -165.6562500020483810 ) ) ;
#6232=CARTESIAN_POINT ( 'NONE',  ( -10.81189881249999907, -6.242252689847864744, -179.1562500020484094 ) ) ;
#6234=CARTESIAN_POINT ( 'NONE',  ( 5.000000000000000000, 8.660254037844385522, -156.6250000040967905 ) ) ;
#6236=CARTESIAN_POINT ( 'NONE',  ( 10.81189881249999551, -6.242252689847874514, -8.968750002048359704 ) ) ;
#6238=CARTESIAN_POINT ( 'NONE',  ( 5.405949406249999534, 9.363379034771803333, -112.0937500020483810 ) ) ;
#6240=CARTESIAN_POINT ( 'NONE',  ( -10.81189881249999729, 1.324075727343319199E-15, -14.28125000204835615 ) ) ;
#6243=CARTESIAN_POINT ( 'NONE',  ( -10.81189881249999907, -6.242252689847864744, -108.6562500020483952 ) ) ;
#6247=CARTESIAN_POINT ( 'NONE',  ( 4.999999999999992006, -8.660254037844389075, -82.12500000409676204 ) ) ;
#6249=CARTESIAN_POINT ( 'NONE',  ( 7.644554776091147741E-16, 12.48450537969573659, -41.46875000204835970 ) ) ;
#6253=CARTESIAN_POINT ( 'NONE',  ( 7.070501591499377789E-16, 11.54700538379251284, -11.00000000409676026 ) ) ;
#6255=ORIENTED_EDGE ( 'NONE', *, *, #37201, .F. ) ;
#6263=VERTEX_POINT ( 'NONE', #20428 ) ;
#6268=CARTESIAN_POINT ( 'NONE',  ( -2.293366432827344421E-15, -12.48450537969573659, -177.4062500020483810 ) ) ;
#6269=CYLINDRICAL_SURFACE ( 'NONE', #35105, 9.999999999999998224 ) ;
#6271=CARTESIAN_POINT ( 'NONE',  ( -10.81189881249999729, 6.242252689847871849, -101.2187500020483810 ) ) ;
#6273=CARTESIAN_POINT ( 'NONE',  ( 10.81189881249999729, 0.000000000000000000, -106.5312500020483810 ) ) ;
#6275=CARTESIAN_POINT ( 'NONE',  ( 7.644554776091147741E-16, 12.48450537969573659, -116.4687500020483668 ) ) ;
#6279=CARTESIAN_POINT ( 'NONE',  ( -5.000000000000003553, -8.660254037844383745, -136.0000000000000000 ) ) ;
#6280=CARTESIAN_POINT ( 'NONE',  ( -9.999999999999998224, 1.224646799147353059E-15, -4.249999999999976019 ) ) ;
#6284=CARTESIAN_POINT ( 'NONE',  ( -4.999999999999996447, 8.660254037844387298, -177.3750000040967905 ) ) ;
#6286=CARTESIAN_POINT ( 'NONE',  ( -2.293366432827344421E-15, -12.48450537969573659, -30.21875000204835260 ) ) ;
#6287=CARTESIAN_POINT ( 'NONE',  ( 4.999999999999992006, -8.660254037844389075, -107.6250000040967763 ) ) ;
#6288=CARTESIAN_POINT ( 'NONE',  ( -2.293366432827344421E-15, -12.48450537969573659, -135.2187500020483810 ) ) ;
#6290=CARTESIAN_POINT ( 'NONE',  ( 4.999999999999992006, -8.660254037844389075, -147.7500000000000000 ) ) ;
#6291=CARTESIAN_POINT ( 'NONE',  ( -9.999999999999998224, 1.224646799147353059E-15, -70.24999999999998579 ) ) ;
#6292=CARTESIAN_POINT ( 'NONE',  ( 10.81189881249999551, -6.242252689847874514, -133.6562500020483810 ) ) ;
#6296=CARTESIAN_POINT ( 'NONE',  ( -9.999999999999998224, 1.224646799147353059E-15, -167.7500000000000000 ) ) ;
#6297=CARTESIAN_POINT ( 'NONE',  ( 9.999999999999998224, 0.000000000000000000, -104.3750000040967763 ) ) ;
#6298=CARTESIAN_POINT ( 'NONE',  ( -10.81189881249999729, 1.324075727343319199E-15, -65.09375000204836681 ) ) ;
#6299=VERTEX_POINT ( 'NONE', #30587 ) ;
#6303=CARTESIAN_POINT ( 'NONE',  ( -5.000000000000003553, -8.660254037844383745, -43.37500000409677625 ) ) ;
#6304=CARTESIAN_POINT ( 'NONE',  ( 10.81189881249999551, -6.242252689847874514, -34.65625000204835970 ) ) ;
#6305=CARTESIAN_POINT ( 'NONE',  ( 7.070501591499376803E-16, 11.54700538379251284, -166.6250000000000000 ) ) ;
#6314=CARTESIAN_POINT ( 'NONE',  ( 4.999999999999992006, -8.660254037844389075, -104.2499999999999858 ) ) ;
#6321=EDGE_CURVE ( 'NONE', #24042, #30761, #808, .T. ) ;
#6324=CARTESIAN_POINT ( 'NONE',  ( 10.81189881249999907, 6.242252689847868297, -127.2187500020483668 ) ) ;
#6325=CARTESIAN_POINT ( 'NONE',  ( 10.81189881249999729, 0.000000000000000000, -130.5312500020484094 ) ) ;
#6327=CARTESIAN_POINT ( 'NONE',  ( 7.644554776091147741E-16, 12.48450537969573659, -144.9687500020484094 ) ) ;
#6328=CARTESIAN_POINT ( 'NONE',  ( 10.70731569305653252, 1.500182182591227154, -180.0000000000000284 ) ) ;
#6330=CARTESIAN_POINT ( 'NONE',  ( 5.000000000000000000, 8.660254037844385522, -160.7500000000000000 ) ) ;
#6331=CARTESIAN_POINT ( 'NONE',  ( -5.405949406249996869, 9.363379034771805109, 0.4687499979516285276 ) ) ;
#6335=CARTESIAN_POINT ( 'NONE',  ( 5.405949406249992428, -9.363379034771808662, -51.09375000204835260 ) ) ;
#6337=CARTESIAN_POINT ( 'NONE',  ( -2.293366432827344421E-15, -12.48450537969573659, -160.7187500020483810 ) ) ;
#6342=CARTESIAN_POINT ( 'NONE',  ( 4.999999999999992006, -8.660254037844389075, -95.24999999999998579 ) ) ;
#6343=ORIENTED_EDGE ( 'NONE', *, *, #42516, .F. ) ;
#6344=CARTESIAN_POINT ( 'NONE',  ( -10.81189881249999729, 6.242252689847871849, -114.9062500020483952 ) ) ;
#6345=CARTESIAN_POINT ( 'NONE',  ( -9.999999999999998224, 1.224646799147353059E-15, -136.6250000040967620 ) ) ;
#6349=CARTESIAN_POINT ( 'NONE',  ( -2.121150477449813534E-15, -11.54700538379251284, -159.8750000000000000 ) ) ;
#6350=CARTESIAN_POINT ( 'NONE',  ( 10.81189881249999907, 6.242252689847868297, -62.90625000204838813 ) ) ;
#6370=CARTESIAN_POINT ( 'NONE',  ( -4.999999999999996447, 8.660254037844387298, -31.49999999999997158 ) ) ;
#6373=CARTESIAN_POINT ( 'NONE',  ( 5.405949406249992428, -9.363379034771808662, -150.0937500020483810 ) ) ;
#6374=CARTESIAN_POINT ( 'NONE',  ( 5.405949406249992428, -9.363379034771808662, -168.0937500020484094 ) ) ;
#6378=CARTESIAN_POINT ( 'NONE',  ( -9.999999999999998224, 5.773502691896259087, -185.8750000000000000 ) ) ;
#6384=CARTESIAN_POINT ( 'NONE',  ( -10.81189881249999907, -6.242252689847864744, -183.4687500020484379 ) ) ;
#6387=CARTESIAN_POINT ( 'NONE',  ( -10.81189881249999729, 6.242252689847871849, -62.40625000204838813 ) ) ;
#6389=CARTESIAN_POINT ( 'NONE',  ( 7.070501591499377789E-16, 11.54700538379251284, -112.6249999999999858 ) ) ;
#6391=CARTESIAN_POINT ( 'NONE',  ( -5.405949406250003975, -9.363379034771801557, -141.5312500020483810 ) ) ;
#6392=CARTESIAN_POINT ( 'NONE',  ( 10.81189881249999729, 0.000000000000000000, -157.5312500020484094 ) ) ;
#6395=CARTESIAN_POINT ( 'NONE',  ( -10.81189881249999907, -6.242252689847864744, -93.46875000204836681 ) ) ;
#6398=CARTESIAN_POINT ( 'NONE',  ( 5.405949406249999534, 9.363379034771803333, -190.0937500020483810 ) ) ;
#6400=CARTESIAN_POINT ( 'NONE',  ( 10.00000000000025402, -5.773502691896113426, -116.5000000040967763 ) ) ;
#6402=CARTESIAN_POINT ( 'NONE',  ( 7.644554776091147741E-16, 12.48450537969573659, -82.15625000204838102 ) ) ;
#6404=CARTESIAN_POINT ( 'NONE',  ( 9.999999999999996447, -5.773502691896262640, -61.00000000409677625 ) ) ;
#6405=CARTESIAN_POINT ( 'NONE',  ( 10.81189881249999551, -6.242252689847874514, -17.96875000204836681 ) ) ;
#6408=CARTESIAN_POINT ( 'NONE',  ( -10.81189881249999729, 1.324075727343319199E-15, -11.28125000204835438 ) ) ;
#6409=DIRECTION ( 'NONE',  ( -1.000000000000000000, 0.000000000000000000, 0.000000000000000000 ) ) ;
#6412=DIRECTION ( 'NONE',  ( -0.000000000000000000, -0.000000000000000000, -1.000000000000000000 ) ) ;
#6419=VERTEX_POINT ( 'NONE', #17179 ) ;
#6428=CARTESIAN_POINT ( 'NONE',  ( -10.81189881249999729, 1.324075727343319199E-15, -153.7812500020484094 ) ) ;
#6435=CARTESIAN_POINT ( 'NONE',  ( -10.81189881249999729, 6.242252689847871849, -75.71875000204836681 ) ) ;
#6436=CARTESIAN_POINT ( 'NONE',  ( -5.405949406249996869, 9.363379034771805109, -82.03125000204839523 ) ) ;
#6438=EDGE_CURVE ( 'NONE', #3489, #3790, #603, .T. ) ;
#6440=CARTESIAN_POINT ( 'NONE',  ( -10.81189881249999729, 6.242252689847871849, -168.9062500020484094 ) ) ;
#6441=CARTESIAN_POINT ( 'NONE',  ( 10.81189881249999907, 6.242252689847868297, -176.9062500020484094 ) ) ;
#6443=CARTESIAN_POINT ( 'NONE',  ( 5.000000000000000000, 8.660254037844385522, -153.6250000040967905 ) ) ;
#6445=CARTESIAN_POINT ( 'NONE',  ( -10.81189881249999729, 1.324075727343319199E-15, -5.093750002048369474 ) ) ;
#6447=CARTESIAN_POINT ( 'NONE',  ( -10.81189881249999729, 1.324075727343319199E-15, -116.0937500020483810 ) ) ;
#6449=CARTESIAN_POINT ( 'NONE',  ( 10.81189881249999729, 0.000000000000000000, -12.03125000204835438 ) ) ;
#6454=CARTESIAN_POINT ( 'NONE',  ( -10.81189881249999729, 1.324075727343319199E-15, -107.2812500020483810 ) ) ;
#6457=CARTESIAN_POINT ( 'NONE',  ( -9.999999999999998224, 1.224646799147353059E-15, -81.12500000409677625 ) ) ;
#6459=CARTESIAN_POINT ( 'NONE',  ( 5.405949406249992428, -9.363379034771808662, -39.09375000204837391 ) ) ;
#6463=CARTESIAN_POINT ( 'NONE',  ( -5.000000000000003553, -8.660254037844383745, -11.87500000409674783 ) ) ;
#6464=ADVANCED_FACE ( 'NONE', ( #17390 ), #11341, .T. ) ;
#6469=VERTEX_POINT ( 'NONE', #32871 ) ;
#6475=CARTESIAN_POINT ( 'NONE',  ( -4.999999999999996447, 8.660254037844387298, -127.8750000040967905 ) ) ;
#6476=CARTESIAN_POINT ( 'NONE',  ( -5.405949406249996869, 9.363379034771805109, -178.0312500020483810 ) ) ;
#6480=CARTESIAN_POINT ( 'NONE',  ( 10.81189881249999907, 6.242252689847868297, -104.7187500020483810 ) ) ;
#6482=CARTESIAN_POINT ( 'NONE',  ( -10.81189881249999729, 1.324075727343319199E-15, -108.7812500020483810 ) ) ;
#6484=CARTESIAN_POINT ( 'NONE',  ( 7.644554776091147741E-16, 12.48450537969573659, -117.9687500020483668 ) ) ;
#6486=( BOUNDED_CURVE ( )  B_SPLINE_CURVE ( 2, ( #29062, #39185, #32516, #42200, #2318, #22575, #35754 ),
 .UNSPECIFIED., .F., .F. ) 
 B_SPLINE_CURVE_WITH_KNOTS ( ( 3, 2, 2, 3 ),
 ( 0.1007462686567163757, 0.1019900497512437887, 0.1032338308457712017, 0.1044776119402986148 ),
 .UNSPECIFIED. ) 
 CURVE ( )  GEOMETRIC_REPRESENTATION_ITEM ( )  RATIONAL_B_SPLINE_CURVE ( ( 1.000000000000004441, 0.8660254037844342667, 1.000000000000000000, 0.8660254037844387076, 1.000000000000000000, 0.8660254037844267172, 1.000000000000011990 ) ) 
 REPRESENTATION_ITEM ( '' )  );
#6487=CARTESIAN_POINT ( 'NONE',  ( -2.121150477449813534E-15, -11.54700538379251284, -143.3750000000000000 ) ) ;
#6488=CARTESIAN_POINT ( 'NONE',  ( 9.999999999999996447, -5.773502691896262640, -5.124999999999963585 ) ) ;
#6491=CARTESIAN_POINT ( 'NONE',  ( 7.070501591499377789E-16, 11.54700538379251284, -183.5000000040968189 ) ) ;
#6493=CARTESIAN_POINT ( 'NONE',  ( 10.81189881249999551, -6.242252689847874514, -26.96875000204837391 ) ) ;
#6494=CARTESIAN_POINT ( 'NONE',  ( -5.405949406249996869, 9.363379034771805109, -134.3437500020484094 ) ) ;
#6496=CARTESIAN_POINT ( 'NONE',  ( 10.81189881249999907, 6.242252689847868297, -38.90625000204836681 ) ) ;
#6498=CARTESIAN_POINT ( 'NONE',  ( -5.000000000000003553, -8.660254037844383745, -68.49999999999997158 ) ) ;
#6499=CARTESIAN_POINT ( 'NONE',  ( -10.81189881249999907, -6.242252689847864744, -132.6562500020484094 ) ) ;
#6503=CARTESIAN_POINT ( 'NONE',  ( -2.121150477449813534E-15, -11.54700538379251284, -107.7500000040967763 ) ) ;
#6505=CARTESIAN_POINT ( 'NONE',  ( 5.405949406249999534, 9.363379034771803333, -64.09375000204836681 ) ) ;
#6511=CARTESIAN_POINT ( 'NONE',  ( 9.999999999999998224, 0.000000000000000000, -119.3750000040967905 ) ) ;
#6512=CARTESIAN_POINT ( 'NONE',  ( -5.000000000000003553, -8.660254037844383745, -32.87500000409676915 ) ) ;
#6520=LINE ( 'NONE', #16201, #18710 ) ;
#6527=CARTESIAN_POINT ( 'NONE',  ( 10.81189881249999907, 6.242252689847868297, -128.7187500020483810 ) ) ;
#6528=CARTESIAN_POINT ( 'NONE',  ( 7.644554776091147741E-16, 12.48450537969573659, -136.1562500020483810 ) ) ;
#6530=CARTESIAN_POINT ( 'NONE',  ( -10.81189881249999729, 6.242252689847871849, -140.2187500020483810 ) ) ;
#6533=CARTESIAN_POINT ( 'NONE',  ( 9.999999999999998224, 0.000000000000000000, -167.0000000000000000 ) ) ;
#6534=CARTESIAN_POINT ( 'NONE',  ( 10.81189881249999729, 0.000000000000000000, -0.03125000204837191653 ) ) ;
#6537=CARTESIAN_POINT ( 'NONE',  ( -10.81189881249999907, -6.242252689847864744, -55.96875000204836681 ) ) ;
#6538=CARTESIAN_POINT ( 'NONE',  ( 0.000000000000000000, 0.000000000000000000, -99.99999999999998579 ) ) ;
#6539=CARTESIAN_POINT ( 'NONE',  ( -10.81189881249999907, -6.242252689847864744, -165.4687500020484094 ) ) ;
#6544=CARTESIAN_POINT ( 'NONE',  ( 4.999999999999992006, -8.660254037844389075, -87.74999999999998579 ) ) ;
#6546=CARTESIAN_POINT ( 'NONE',  ( 5.405949406249999534, 9.363379034771803333, -119.7812500020483952 ) ) ;
#6547=CARTESIAN_POINT ( 'NONE',  ( 10.00000000000000000, 5.773502691896255534, -135.7500000040967905 ) ) ;
#6552=CARTESIAN_POINT ( 'NONE',  ( 5.405949406249992428, -9.363379034771808662, -57.28125000204836681 ) ) ;
#6570=CYLINDRICAL_SURFACE ( 'NONE', #41200, 9.999999999999998224 ) ;
#6571=CARTESIAN_POINT ( 'NONE',  ( 10.00000000000000000, 5.773502691896255534, -30.37499999999995737 ) ) ;
#6574=CARTESIAN_POINT ( 'NONE',  ( -10.81189881249999729, 6.242252689847871849, -150.7187500020483810 ) ) ;
#6575=CARTESIAN_POINT ( 'NONE',  ( -5.405949406250003975, -9.363379034771801557, -160.8437500020484094 ) ) ;
#6578=CARTESIAN_POINT ( 'NONE',  ( -2.121150477449813534E-15, -11.54700538379251284, -191.3750000000000284 ) ) ;
#6581=CARTESIAN_POINT ( 'NONE',  ( 9.999999999999998224, 0.000000000000000000, -123.8750000040967905 ) ) ;
#6584=CARTESIAN_POINT ( 'NONE',  ( 5.405949406249999534, 9.363379034771803333, -188.5937500020483810 ) ) ;
#6586=CARTESIAN_POINT ( 'NONE',  ( -10.81189881249999907, -6.242252689847864744, -62.15625000204838102 ) ) ;
#6588=CARTESIAN_POINT ( 'NONE',  ( -4.999999999999996447, 8.660254037844387298, -118.5000000000000000 ) ) ;
#6590=CARTESIAN_POINT ( 'NONE',  ( -2.293366432827344421E-15, -12.48450537969573659, -144.4062500020484094 ) ) ;
#6591=CARTESIAN_POINT ( 'NONE',  ( 5.405949406249999534, 9.363379034771803333, -152.7812500020484094 ) ) ;
#6593=CYLINDRICAL_SURFACE ( 'NONE', #8913, 9.999999999999998224 ) ;
#6594=CARTESIAN_POINT ( 'NONE',  ( 10.81189881249999729, 0.000000000000000000, -89.84375000204838102 ) ) ;
#6597=CARTESIAN_POINT ( 'NONE',  ( 10.81189881249999907, 6.242252689847868297, -190.2187500020484094 ) ) ;
#6601=CARTESIAN_POINT ( 'NONE',  ( 10.81189881249999907, 6.242252689847868297, -83.90625000204836681 ) ) ;
#6605=CARTESIAN_POINT ( 'NONE',  ( -9.999999999999998224, 5.773502691896259087, -60.25000000409677625 ) ) ;
#6606=CARTESIAN_POINT ( 'NONE',  ( -5.405949406249996869, 9.363379034771805109, -18.84375000204835260 ) ) ;
#6609=CARTESIAN_POINT ( 'NONE',  ( -5.405949406249996869, 9.363379034771805109, -14.53125000204835615 ) ) ;
#6611=CARTESIAN_POINT ( 'NONE',  ( -9.999999999999742428, -5.773502691896402084, -161.6250000000000284 ) ) ;
#6613=CARTESIAN_POINT ( 'NONE',  ( 7.070501591499376803E-16, 11.54700538379251284, -114.5000000040967905 ) ) ;
#6614=CARTESIAN_POINT ( 'NONE',  ( -9.999999999999804601, 5.773502691896371886, -177.2500000040967905 ) ) ;
#6626=( BOUNDED_CURVE ( )  B_SPLINE_CURVE ( 2, ( #15770, #39086, #25312, #2846, #5873, #32632, #12737 ),
 .UNSPECIFIED., .F., .F. ) 
 B_SPLINE_CURVE_WITH_KNOTS ( ( 3, 2, 2, 3 ),
 ( 0.1492537313432835966, 0.1504975124378109819, 0.1517412935323383116, 0.1529850746268656692 ),
 .UNSPECIFIED. ) 
 CURVE ( )  GEOMETRIC_REPRESENTATION_ITEM ( )  RATIONAL_B_SPLINE_CURVE ( ( 0.9999999999999970024, 0.8660254037844417052, 1.000000000000000000, 0.8660254037844387076, 1.000000000000000000, 0.8660254037844387076, 1.000000000000000000 ) ) 
 REPRESENTATION_ITEM ( '' )  );
#6634=CARTESIAN_POINT ( 'NONE',  ( 10.81189881249999551, -6.242252689847874514, -153.1562500020484379 ) ) ;
#6636=CARTESIAN_POINT ( 'NONE',  ( 9.999999999999998224, 0.000000000000000000, -179.0000000000000000 ) ) ;
#6640=CARTESIAN_POINT ( 'NONE',  ( -10.81189881249999729, 6.242252689847871849, -78.71875000204838102 ) ) ;
#6641=CARTESIAN_POINT ( 'NONE',  ( 10.81189881249999907, 6.242252689847868297, -80.90625000204839523 ) ) ;
#6644=CARTESIAN_POINT ( 'NONE',  ( 5.405949406249992428, -9.363379034771808662, -163.7812500020484094 ) ) ;
#6645=CARTESIAN_POINT ( 'NONE',  ( -10.81189881249999907, -6.242252689847864744, -183.6562500020483810 ) ) ;
#6646=CARTESIAN_POINT ( 'NONE',  ( 7.070501591499377789E-16, 11.54700538379251284, -155.0000000040968189 ) ) ;
#6647=DIRECTION ( 'NONE',  ( -0.000000000000000000, -0.000000000000000000, -1.000000000000000000 ) ) ;
#6648=CARTESIAN_POINT ( 'NONE',  ( 10.81189881249999551, -6.242252689847874514, -2.968750002048353931 ) ) ;
#6650=CARTESIAN_POINT ( 'NONE',  ( -10.81189881249999729, 6.242252689847871849, -111.7187500020483810 ) ) ;
#6652=CARTESIAN_POINT ( 'NONE',  ( 7.644554776091147741E-16, 12.48450537969573659, -10.15625000204836681 ) ) ;
#6655=CARTESIAN_POINT ( 'NONE',  ( -2.293366432827344421E-15, -12.48450537969573659, -106.9062500020483952 ) ) ;
#6658=CARTESIAN_POINT ( 'NONE',  ( 10.00000000000000000, 5.773502691896255534, -80.25000000409679046 ) ) ;
#6660=CARTESIAN_POINT ( 'NONE',  ( -10.81189881249999729, 6.242252689847871849, -44.21875000204836681 ) ) ;
#6665=CARTESIAN_POINT ( 'NONE',  ( 10.00000000000000000, 5.773502691896255534, -12.75000000409676204 ) ) ;
#6668=ORIENTED_EDGE ( 'NONE', *, *, #13828, .F. ) ;
#6670=ADVANCED_FACE ( 'NONE', ( #32455 ), #32661, .F. ) ;
#6680=CARTESIAN_POINT ( 'NONE',  ( -10.81189881249999907, -6.242252689847864744, -180.6562500020484094 ) ) ;
#6685=CARTESIAN_POINT ( 'NONE',  ( 10.81189881249999551, -6.242252689847874514, -98.96875000204838102 ) ) ;
#6687=CARTESIAN_POINT ( 'NONE',  ( 5.405949406249999534, 9.363379034771803333, -110.7812500020483810 ) ) ;
#6689=CARTESIAN_POINT ( 'NONE',  ( -10.81189881249999729, 6.242252689847871849, -114.7187500020483810 ) ) ;
#6693=CARTESIAN_POINT ( 'NONE',  ( 5.000000000000000000, 8.660254037844385522, -132.2499999999999716 ) ) ;
#6694=CARTESIAN_POINT ( 'NONE',  ( -5.000000000000003553, -8.660254037844383745, -3.999999999999976019 ) ) ;
#6698=CARTESIAN_POINT ( 'NONE',  ( -2.121150477449813534E-15, -11.54700538379251284, -178.2500000040967620 ) ) ;
#6700=CARTESIAN_POINT ( 'NONE',  ( 10.81189881249999907, 6.242252689847868297, -28.21875000204838102 ) ) ;
#6702=CARTESIAN_POINT ( 'NONE',  ( -5.405949406249996869, 9.363379034771805109, -140.3437500020484094 ) ) ;
#6704=CARTESIAN_POINT ( 'NONE',  ( 10.81189881249999551, -6.242252689847874514, -33.15625000204835970 ) ) ;
#6706=DIRECTION ( 'NONE',  ( -0.000000000000000000, -0.000000000000000000, -1.000000000000000000 ) ) ;
#6707=CARTESIAN_POINT ( 'NONE',  ( 5.000000000000000000, 8.660254037844385522, -66.24999999999997158 ) ) ;
#6708=CARTESIAN_POINT ( 'NONE',  ( -10.81189881249999907, -6.242252689847864744, -129.6562500020483810 ) ) ;
#6710=ORIENTED_EDGE ( 'NONE', *, *, #33868, .F. ) ;
#6712=CARTESIAN_POINT ( 'NONE',  ( -9.999999999999998224, 1.224646799147353059E-15, -111.1250000040967763 ) ) ;
#6714=CARTESIAN_POINT ( 'NONE',  ( -2.293366432827344421E-15, -12.48450537969573659, -63.21875000204838102 ) ) ;
#6720=FACE_OUTER_BOUND ( 'NONE', #27467, .T. ) ;
#6721=CARTESIAN_POINT ( 'NONE',  ( 7.070501591499377789E-16, 11.54700538379251284, -39.50000000409675494 ) ) ;
#6722=CARTESIAN_POINT ( 'NONE',  ( -9.999999999999998224, 1.224646799147353059E-15, -166.2500000000000000 ) ) ;
#6737=CARTESIAN_POINT ( 'NONE',  ( -10.81189881249999729, 1.324075727343319199E-15, -125.0937500020483668 ) ) ;
#6738=CARTESIAN_POINT ( 'NONE',  ( -5.405949406249996869, 9.363379034771805109, -130.0312500020484094 ) ) ;
#6740=CARTESIAN_POINT ( 'NONE',  ( 10.81189881249999551, -6.242252689847874514, -140.9687500020483810 ) ) ;
#6742=DIRECTION ( 'NONE',  ( -1.000000000000000000, 0.000000000000000000, 0.000000000000000000 ) ) ;
#6744=CARTESIAN_POINT ( 'NONE',  ( 7.070501591499377789E-16, 11.54700538379251284, -160.6250000000000284 ) ) ;
#6748=CARTESIAN_POINT ( 'NONE',  ( 5.405949406249992428, -9.363379034771808662, -57.09375000204835970 ) ) ;
#6749=CARTESIAN_POINT ( 'NONE',  ( -10.81189881249999729, 6.242252689847871849, -164.2187500020483810 ) ) ;
#6754=CARTESIAN_POINT ( 'NONE',  ( -9.999999999999998224, 1.224646799147353059E-15, -92.74999999999998579 ) ) ;
#6756=CARTESIAN_POINT ( 'NONE',  ( 10.81189881249999729, 6.242252689847867408, -112.4062500020483952 ) ) ;
#6757=CARTESIAN_POINT ( 'NONE',  ( 4.999999999999992006, -8.660254037844389075, -133.1250000040967620 ) ) ;
#6758=CARTESIAN_POINT ( 'NONE',  ( 9.999999999999998224, 0.000000000000000000, -111.4999999999999858 ) ) ;
#6762=CARTESIAN_POINT ( 'NONE',  ( 5.405949406249992428, -9.363379034771808662, -52.78125000204836681 ) ) ;
#6767=CARTESIAN_POINT ( 'NONE',  ( 9.999999999999998224, 0.000000000000000000, -174.5000000000000284 ) ) ;
#6772=ORIENTED_EDGE ( 'NONE', *, *, #9853, .F. ) ;
#6775=ORIENTED_EDGE ( 'NONE', *, *, #56, .T. ) ;
#6776=VERTEX_POINT ( 'NONE', #14023 ) ;
#6779=SHAPE_REPRESENTATION ( 'reaction body', ( #39998 ), #29026 ) ;
#6783=CARTESIAN_POINT ( 'NONE',  ( 7.070501591499377789E-16, 11.54700538379251284, -30.12499999999995737 ) ) ;
#6786=CARTESIAN_POINT ( 'NONE',  ( 10.81189881249999551, -6.242252689847874514, -146.9687500020484094 ) ) ;
#6787=CARTESIAN_POINT ( 'NONE',  ( -10.81189881249999729, -6.242252689847864744, -160.9687500020484094 ) ) ;
#6790=CARTESIAN_POINT ( 'NONE',  ( 9.999999999999996447, -5.773502691896262640, -186.6250000000000284 ) ) ;
#6795=CARTESIAN_POINT ( 'NONE',  ( -10.81189881249999729, 1.324075727343319199E-15, -186.5937500020483810 ) ) ;
#6800=CARTESIAN_POINT ( 'NONE',  ( 7.644554776091147741E-16, 12.48450537969573659, -55.15625000204838102 ) ) ;
#6802=CARTESIAN_POINT ( 'NONE',  ( 7.070501591499377789E-16, 11.54700538379251284, -115.6249999999999858 ) ) ;
#6805=CARTESIAN_POINT ( 'NONE',  ( -10.81189881249999729, 1.324075727343319199E-15, -134.2812500020483810 ) ) ;
#6806=CARTESIAN_POINT ( 'NONE',  ( 7.644554776091147741E-16, 12.48450537969573659, -149.6562500020484094 ) ) ;
#6809=CARTESIAN_POINT ( 'NONE',  ( -5.405949406250003975, -9.363379034771801557, -82.84375000204836681 ) ) ;
#6812=CARTESIAN_POINT ( 'NONE',  ( -2.293366432827344421E-15, -12.48450537969573659, -187.7187500020484094 ) ) ;
#6816=CARTESIAN_POINT ( 'NONE',  ( 5.405949406249992428, -9.363379034771808662, -84.28125000204838102 ) ) ;
#6818=CARTESIAN_POINT ( 'NONE',  ( -5.000000000000003553, -8.660254037844383745, -62.87500000409676204 ) ) ;
#6819=CARTESIAN_POINT ( 'NONE',  ( 10.81189881249999907, 6.242252689847868297, -19.21875000204836681 ) ) ;
#6822=CARTESIAN_POINT ( 'NONE',  ( -10.81189881249999729, 1.324075727343319199E-15, -15.78125000204835793 ) ) ;
#6833=EDGE_CURVE ( 'NONE', #1591, #19597, #32, .T. ) ;
#6837=VECTOR ( 'NONE', #13942, 1000.000000000000000 ) ;
#6842=DIRECTION ( 'NONE',  ( -0.000000000000000000, -0.000000000000000000, -1.000000000000000000 ) ) ;
#6845=CARTESIAN_POINT ( 'NONE',  ( -5.405949406249996869, 9.363379034771805109, -148.0312500020483810 ) ) ;
#6852=CARTESIAN_POINT ( 'NONE',  ( -2.293366432827344421E-15, -12.48450537969573659, -67.71875000204838102 ) ) ;
#6853=CARTESIAN_POINT ( 'NONE',  ( 10.81189881249999551, -6.242252689847874514, -78.15625000204838102 ) ) ;
#6857=CARTESIAN_POINT ( 'NONE',  ( -10.81189881249999729, 1.324075727343319199E-15, -168.7812500020484094 ) ) ;
#6858=CARTESIAN_POINT ( 'NONE',  ( -5.405949406250003975, -9.363379034771801557, -182.0312500020483810 ) ) ;
#6859=CARTESIAN_POINT ( 'NONE',  ( 0.000000000000000000, 0.000000000000000000, -99.99999999999998579 ) ) ;
#6860=CARTESIAN_POINT ( 'NONE',  ( 10.81189881249999729, 0.000000000000000000, -2.843750002048367698 ) ) ;
#6862=CARTESIAN_POINT ( 'NONE',  ( -10.81189881249999729, 1.324075727343319199E-15, -114.5937500020483810 ) ) ;
#6865=CARTESIAN_POINT ( 'NONE',  ( -10.81189881249999907, -6.242252689847864744, -9.656250002048366810 ) ) ;
#6868=CARTESIAN_POINT ( 'NONE',  ( -2.293366432827344421E-15, -12.48450537969573659, -105.4062500020483810 ) ) ;
#6871=CARTESIAN_POINT ( 'NONE',  ( 4.999999999999992006, -8.660254037844389075, -83.62500000409677625 ) ) ;
#6873=CARTESIAN_POINT ( 'NONE',  ( 5.405949406249999534, 9.363379034771803333, -46.09375000204838102 ) ) ;
#6879=CARTESIAN_POINT ( 'NONE',  ( -5.000000000000003553, -8.660254037844383745, -13.37500000409674783 ) ) ;
#6883=ORIENTED_EDGE ( 'NONE', *, *, #4462, .F. ) ;
#6893=CARTESIAN_POINT ( 'NONE',  ( -10.81189881249999729, 6.242252689847871849, -176.4062500020484094 ) ) ;
#6897=CARTESIAN_POINT ( 'NONE',  ( -10.81189881249999729, 1.324075727343319199E-15, -104.0937500020483810 ) ) ;
#6899=CARTESIAN_POINT ( 'NONE',  ( 10.81189881249999907, 6.242252689847868297, -104.9062500020483952 ) ) ;
#6901=CARTESIAN_POINT ( 'NONE',  ( 10.81189881249999551, -6.242252689847874514, -116.9687500020483810 ) ) ;
#6904=CARTESIAN_POINT ( 'NONE',  ( 5.000000000000000000, 8.660254037844385522, -130.7499999999999716 ) ) ;
#6905=CARTESIAN_POINT ( 'NONE',  ( -9.999999999999998224, 1.224646799147353059E-15, -1.249999999999973355 ) ) ;
#6908=CARTESIAN_POINT ( 'NONE',  ( 9.999999999999996447, -5.773502691896262640, -184.0000000040968189 ) ) ;
#6910=CARTESIAN_POINT ( 'NONE',  ( -5.405949406250003975, -9.363379034771801557, -27.34375000204835970 ) ) ;
#6911=DIRECTION ( 'NONE',  ( -0.000000000000000000, -0.000000000000000000, -1.000000000000000000 ) ) ;
#6912=CARTESIAN_POINT ( 'NONE',  ( -5.405949406249996869, 9.363379034771805109, -135.8437500020484094 ) ) ;
#6913=EDGE_CURVE ( 'NONE', #25998, #5147, #23979, .T. ) ;
#6915=CARTESIAN_POINT ( 'NONE',  ( 7.644554776091147741E-16, 12.48450537969573659, -38.65625000204836681 ) ) ;
#6916=CARTESIAN_POINT ( 'NONE',  ( 9.999999999999998224, 0.000000000000000000, -111.4999999999999858 ) ) ;
#6918=CARTESIAN_POINT ( 'NONE',  ( 4.999999999999992006, -8.660254037844389075, -59.24999999999997158 ) ) ;
#6919=CARTESIAN_POINT ( 'NONE',  ( -5.405949406250003975, -9.363379034771801557, -135.5312500020484094 ) ) ;
#6922=CARTESIAN_POINT ( 'NONE',  ( -9.999999999998969713, -5.773502691896847949, -131.6250000000000000 ) ) ;
#6923=CARTESIAN_POINT ( 'NONE',  ( 5.000000000000000000, 8.660254037844385522, -107.1250000040967763 ) ) ;
#6925=CARTESIAN_POINT ( 'NONE',  ( 5.405949406249992428, -9.363379034771808662, -64.59375000204836681 ) ) ;
#6930=CARTESIAN_POINT ( 'NONE',  ( 9.999999999999742428, 5.773502691896404748, -125.2500000040967478 ) ) ;
#6931=CARTESIAN_POINT ( 'NONE',  ( -4.999999999999996447, 8.660254037844387298, -33.37500000409676915 ) ) ;
#6932=CARTESIAN_POINT ( 'NONE',  ( 9.999999999999998224, 1.224646799147353059E-15, -99.99999999999998579 ) ) ;
#6936=CYLINDRICAL_SURFACE ( 'NONE', #24525, 9.999999999999998224 ) ;
#6939=ORIENTED_EDGE ( 'NONE', *, *, #17487, .F. ) ;
#6940=EDGE_CURVE ( 'NONE', #31885, #31861, #4426, .T. ) ;
#6946=CARTESIAN_POINT ( 'NONE',  ( -9.999999999999998224, 1.224646799147353059E-15, -111.1250000040967763 ) ) ;
#6951=CARTESIAN_POINT ( 'NONE',  ( -10.81189881249999729, 1.324075727343319199E-15, -122.0937500020483952 ) ) ;
#6952=CARTESIAN_POINT ( 'NONE',  ( -10.81189881249999907, -6.242252689847864744, -132.6562500020484094 ) ) ;
#6954=CARTESIAN_POINT ( 'NONE',  ( -2.293366432827344421E-15, -12.48450537969573659, -136.7187500020483810 ) ) ;
#6956=CARTESIAN_POINT ( 'NONE',  ( -10.00000000000051337, 5.773502691895962435, -141.2500000040967905 ) ) ;
#6957=CARTESIAN_POINT ( 'NONE',  ( -5.000000000000003553, -8.660254037844383745, -155.5000000000000000 ) ) ;
#6958=DIRECTION ( 'NONE',  ( -1.000000000000000000, 0.000000000000000000, 0.000000000000000000 ) ) ;
#6963=CARTESIAN_POINT ( 'NONE',  ( -10.81189881249999907, -6.242252689847864744, -52.96875000204837391 ) ) ;
#6965=CARTESIAN_POINT ( 'NONE',  ( 10.81189881249999907, 6.242252689847868297, -164.7187500020483810 ) ) ;
#6970=CARTESIAN_POINT ( 'NONE',  ( 10.00000000000000000, 5.773502691896255534, -94.87499999999998579 ) ) ;
#6972=EDGE_LOOP ( 'NONE', ( #41467, #38685, #6101, #19751 ) ) ;
#6973=CARTESIAN_POINT ( 'NONE',  ( 5.405949406249999534, 9.363379034771803333, -107.7812500020483810 ) ) ;
#6974=CARTESIAN_POINT ( 'NONE',  ( -10.00000000000000000, -5.773502691896251982, -132.0000000040967905 ) ) ;
#6975=CARTESIAN_POINT ( 'NONE',  ( -2.121150477449813534E-15, -11.54700538379251284, -177.8750000000000000 ) ) ;
#6980=CARTESIAN_POINT ( 'NONE',  ( -5.405949406250003975, -9.363379034771801557, -56.03125000204836681 ) ) ;
#6998=UNCERTAINTY_MEASURE_WITH_UNIT (LENGTH_MEASURE( 1.000000000000000082E-05 ), #1003, 'distance_accuracy_value', 'NONE');
#7006=CARTESIAN_POINT ( 'NONE',  ( 7.644554776091147741E-16, 12.48450537969573659, -147.9687500020484094 ) ) ;
#7007=CARTESIAN_POINT ( 'NONE',  ( 10.81189881249999729, 0.000000000000000000, -160.3437500020484094 ) ) ;
#7008=DIRECTION ( 'NONE',  ( -0.000000000000000000, -0.000000000000000000, -1.000000000000000000 ) ) ;
#7010=CARTESIAN_POINT ( 'NONE',  ( 5.000000000000000000, 8.660254037844385522, -178.7500000000000284 ) ) ;
#7015=CARTESIAN_POINT ( 'NONE',  ( -10.81189881249999907, -6.242252689847864744, -184.9687500020484094 ) ) ;
#7018=CARTESIAN_POINT ( 'NONE',  ( 10.81189881249999729, 0.000000000000000000, -52.53125000204835970 ) ) ;
#7020=CARTESIAN_POINT ( 'NONE',  ( 9.999999999999996447, -5.773502691896262640, -117.6250000000000000 ) ) ;
#7021=AXIS2_PLACEMENT_3D ( 'NONE', #23524, #20691, #36673 ) ;
#7023=CARTESIAN_POINT ( 'NONE',  ( 10.81189881249999729, 6.242252689847867408, -137.9062500020484094 ) ) ;
#7024=CARTESIAN_POINT ( 'NONE',  ( -10.81189881249999729, 6.242252689847871849, -149.4062500020484094 ) ) ;
#7027=CARTESIAN_POINT ( 'NONE',  ( 5.405949406249999534, 9.363379034771803333, -82.09375000204836681 ) ) ;
#7030=CARTESIAN_POINT ( 'NONE',  ( -10.81189881249999729, 6.242252689847871849, -179.2187500020483810 ) ) ;
#7034=CARTESIAN_POINT ( 'NONE',  ( -2.293366432827344421E-15, -12.48450537969573659, -75.40625000204838102 ) ) ;
#7036=CARTESIAN_POINT ( 'NONE',  ( 9.999999999999996447, -5.773502691896262640, -49.00000000409676915 ) ) ;
#7037=CARTESIAN_POINT ( 'NONE',  ( -10.81189881249999729, 6.242252689847871849, -11.21875000204835970 ) ) ;
#7038=CARTESIAN_POINT ( 'NONE',  ( 4.999999999999992006, -8.660254037844389075, -137.6250000040967620 ) ) ;
#7040=VECTOR ( 'NONE', #402, 1000.000000000000000 ) ;
#7042=CARTESIAN_POINT ( 'NONE',  ( 10.81189881249999551, -6.242252689847874514, -1.656250002048359482 ) ) ;
#7045=CARTESIAN_POINT ( 'NONE',  ( -4.999999999999996447, 8.660254037844387298, -114.3750000040967763 ) ) ;
#7052=ORIENTED_EDGE ( 'NONE', *, *, #22537, .T. ) ;
#7053=EDGE_LOOP ( 'NONE', ( #15204, #33064 ) ) ;
#7059=CARTESIAN_POINT ( 'NONE',  ( 4.999999999999992006, -8.660254037844389075, -41.24999999999997868 ) ) ;
#7062=LINE ( 'NONE', #39431, #29485 ) ;
#7063=LINE ( 'NONE', #16317, #16352 ) ;
#7064=CARTESIAN_POINT ( 'NONE',  ( -10.81189881249999729, 6.242252689847871849, -152.4062500020483810 ) ) ;
#7072=CARTESIAN_POINT ( 'NONE',  ( 10.81189881249999729, 0.000000000000000000, -71.84375000204836681 ) ) ;
#7073=CARTESIAN_POINT ( 'NONE',  ( 7.644554776091147741E-16, 12.48450537969573659, -73.15625000204836681 ) ) ;
#7075=CARTESIAN_POINT ( 'NONE',  ( 5.405949406249999534, 9.363379034771803333, -161.7812500020484094 ) ) ;
#7076=CARTESIAN_POINT ( 'NONE',  ( -10.81189881249999729, 1.324075727343319199E-15, -176.2812500020484094 ) ) ;
#7080=CARTESIAN_POINT ( 'NONE',  ( -5.405949406249996869, 9.363379034771805109, -104.3437500020483810 ) ) ;
#7082=CARTESIAN_POINT ( 'NONE',  ( 5.405949406249992428, -9.363379034771808662, -4.781250002048375691 ) ) ;
#7085=CARTESIAN_POINT ( 'NONE',  ( 10.81189881249999729, 0.000000000000000000, -103.5312500020483810 ) ) ;
#7088=CARTESIAN_POINT ( 'NONE',  ( 10.00000000000000000, 5.773502691896255534, -84.75000000409677625 ) ) ;
#7090=CARTESIAN_POINT ( 'NONE',  ( 10.81189881249999551, -6.242252689847874514, -32.96875000204835260 ) ) ;
#7093=CARTESIAN_POINT ( 'NONE',  ( 10.81189881249999907, 6.242252689847868297, -35.90625000204835970 ) ) ;
#7095=CARTESIAN_POINT ( 'NONE',  ( -4.999999999999996447, 8.660254037844387298, -12.37500000409674783 ) ) ;
#7097=CARTESIAN_POINT ( 'NONE',  ( 10.00000000000038369, -5.773502691896038819, -155.5000000040967905 ) ) ;
#7099=EDGE_LOOP ( 'NONE', ( #31859, #8534, #41414, #34019 ) ) ;
#7107=CARTESIAN_POINT ( 'NONE',  ( -9.999999999999998224, 1.224646799147353059E-15, -153.1250000040967905 ) ) ;
#7109=( BOUNDED_CURVE ( )  B_SPLINE_CURVE ( 2, ( #10932, #20228, #21079, #33417, #34267, #40077, #37057 ),
 .UNSPECIFIED., .F., .F. ) 
 B_SPLINE_CURVE_WITH_KNOTS ( ( 3, 2, 2, 3 ),
 ( 0.2649253731343284568, 0.2661691542288558421, 0.2674129353233831718, 0.2686567164179105571 ),
 .UNSPECIFIED. ) 
 CURVE ( )  GEOMETRIC_REPRESENTATION_ITEM ( )  RATIONAL_B_SPLINE_CURVE ( ( 0.9999999999999880096, 0.8660254037844506980, 1.000000000000000000, 0.8660254037844387076, 1.000000000000000000, 0.8660254037844267172, 1.000000000000011990 ) ) 
 REPRESENTATION_ITEM ( '' )  );
#7110=CARTESIAN_POINT ( 'NONE',  ( 10.81189881249999551, -6.242252689847874514, -169.6562500020484094 ) ) ;
#7111=CARTESIAN_POINT ( 'NONE',  ( -9.999999999999998224, 1.224646799147353059E-15, -147.1250000040967905 ) ) ;
#7113=CARTESIAN_POINT ( 'NONE',  ( -2.293366432827344421E-15, -12.48450537969573659, -90.21875000204838102 ) ) ;
#7115=CARTESIAN_POINT ( 'NONE',  ( -10.81189881249999729, 6.242252689847871849, -102.9062500020483810 ) ) ;
#7117=CARTESIAN_POINT ( 'NONE',  ( 5.405949406249992428, -9.363379034771808662, -114.0937500020483810 ) ) ;
#7121=CARTESIAN_POINT ( 'NONE',  ( 7.644554776091147741E-16, 12.48450537969573659, -197.6562500020484379 ) ) ;
#7124=CARTESIAN_POINT ( 'NONE',  ( 10.00000000000000000, 5.773502691896255534, -171.7500000040967905 ) ) ;
#7126=CARTESIAN_POINT ( 'NONE',  ( -10.81189881249999729, 6.242252689847871849, -18.71875000204837036 ) ) ;
#7128=CARTESIAN_POINT ( 'NONE',  ( -10.81189881249999729, 1.324075727343319199E-15, -134.0937500020483810 ) ) ;
#7130=CARTESIAN_POINT ( 'NONE',  ( -5.405949406250003975, -9.363379034771801557, -27.53125000204836681 ) ) ;
#7132=CARTESIAN_POINT ( 'NONE',  ( 5.000000000000000000, 8.660254037844385522, -58.74999999999997158 ) ) ;
#7133=CARTESIAN_POINT ( 'NONE',  ( -10.81189881249999729, 1.324075727343319199E-15, -132.7812500020483810 ) ) ;
#7137=CARTESIAN_POINT ( 'NONE',  ( -9.999999999999998224, 5.773502691896259087, -108.2500000040967763 ) ) ;
#7138=CARTESIAN_POINT ( 'NONE',  ( 9.999999999999998224, 0.000000000000000000, -101.3750000040967905 ) ) ;
#7139=CARTESIAN_POINT ( 'NONE',  ( 10.81189881249999907, 6.242252689847868297, -67.21875000204838102 ) ) ;
#7144=CARTESIAN_POINT ( 'NONE',  ( 4.999999999999992006, -8.660254037844389075, -34.12500000409676915 ) ) ;
#7148=ORIENTED_EDGE ( 'NONE', *, *, #20142, .T. ) ;
#7152=ADVANCED_FACE ( 'NONE', ( #31116, #35788 ), #39011, .T. ) ;
#7153=CARTESIAN_POINT ( 'NONE',  ( -9.999999999999227285, -5.773502691896698735, -104.6249999999999574 ) ) ;
#7155=CARTESIAN_POINT ( 'NONE',  ( 10.81189881249999907, 6.242252689847868297, -199.4062500020484094 ) ) ;
#7160=CARTESIAN_POINT ( 'NONE',  ( -9.999999999999998224, 1.224646799147353059E-15, -119.7500000000000000 ) ) ;
#7161=CARTESIAN_POINT ( 'NONE',  ( -2.293366432827344421E-15, -12.48450537969573659, -120.2187500020483952 ) ) ;
#7162=CARTESIAN_POINT ( 'NONE',  ( -2.121150477449813534E-15, -11.54700538379251284, -193.2500000040968473 ) ) ;
#7163=CARTESIAN_POINT ( 'NONE',  ( -10.81189881249999729, 6.242252689847871849, -126.9062500020483810 ) ) ;
#7165=CARTESIAN_POINT ( 'NONE',  ( 5.405949406249999534, 9.363379034771803333, -140.5937500020483810 ) ) ;
#7168=CARTESIAN_POINT ( 'NONE',  ( 9.999999999999996447, -5.773502691896262640, -152.1250000000000284 ) ) ;
#7169=CARTESIAN_POINT ( 'NONE',  ( 7.644554776091147741E-16, 12.48450537969573659, 0.3437499979516422943 ) ) ;
#7173=CARTESIAN_POINT ( 'NONE',  ( -10.81189881249999907, -6.242252689847864744, -54.46875000204836681 ) ) ;
#7175=CARTESIAN_POINT ( 'NONE',  ( -10.81189881249999907, -6.242252689847864744, -154.9687500020484094 ) ) ;
#7179=CARTESIAN_POINT ( 'NONE',  ( 9.999999999999998224, 0.000000000000000000, -85.99999999999998579 ) ) ;
#7181=ORIENTED_EDGE ( 'NONE', *, *, #14541, .T. ) ;
#7182=CARTESIAN_POINT ( 'NONE',  ( 10.81189881249999729, 0.000000000000000000, -109.5312500020483810 ) ) ;
#7183=CARTESIAN_POINT ( 'NONE',  ( -9.999999999999998224, 5.773502691896259087, -130.7500000040967905 ) ) ;
#7186=LINE ( 'NONE', #20770, #12491 ) ;
#7187=CARTESIAN_POINT ( 'NONE',  ( -5.405949406250003975, -9.363379034771801557, -51.53125000204835970 ) ) ;
#7201=VERTEX_POINT ( 'NONE', #19154 ) ;
#7211=CARTESIAN_POINT ( 'NONE',  ( 10.81189881249999551, -6.242252689847874514, -149.9687500020483810 ) ) ;
#7212=CARTESIAN_POINT ( 'NONE',  ( -5.405949406250003975, -9.363379034771801557, -159.3437500020484094 ) ) ;
#7213=CARTESIAN_POINT ( 'NONE',  ( 9.999999999999742428, 5.773502691896404748, -123.7500000040967763 ) ) ;
#7215=CARTESIAN_POINT ( 'NONE',  ( -10.00000000000000000, -5.773502691896251982, -176.6250000000000284 ) ) ;
#7220=CARTESIAN_POINT ( 'NONE',  ( 10.81189881249999907, 6.242252689847868297, -185.7187500020483810 ) ) ;
#7224=CARTESIAN_POINT ( 'NONE',  ( -10.81189881249999907, -6.242252689847864744, -50.15625000204837391 ) ) ;
#7226=CARTESIAN_POINT ( 'NONE',  ( 9.999999999999996447, -5.773502691896262640, -110.1250000000000000 ) ) ;
#7228=CARTESIAN_POINT ( 'NONE',  ( -5.405949406250003975, -9.363379034771801557, -131.0312500020484094 ) ) ;
#7229=CARTESIAN_POINT ( 'NONE',  ( 10.81189881249999729, 0.000000000000000000, -147.0312500020483810 ) ) ;
#7232=CARTESIAN_POINT ( 'NONE',  ( -5.405949406249996869, 9.363379034771805109, -84.84375000204836681 ) ) ;
#7235=CARTESIAN_POINT ( 'NONE',  ( 7.644554776091147741E-16, 12.48450537969573659, -180.9687500020484094 ) ) ;
#7238=CARTESIAN_POINT ( 'NONE',  ( 10.00000000000051159, -5.773502691895965988, -175.0000000040968189 ) ) ;
#7239=CARTESIAN_POINT ( 'NONE',  ( -5.405949406250003975, -9.363379034771801557, -78.53125000204838102 ) ) ;
#7242=CARTESIAN_POINT ( 'NONE',  ( -5.000000000000003553, -8.660254037844383745, -49.37500000409678336 ) ) ;
#7243=CARTESIAN_POINT ( 'NONE',  ( -5.405949406250003975, -9.363379034771801557, -6.343750002048370362 ) ) ;
#7246=CARTESIAN_POINT ( 'NONE',  ( -10.81189881249999907, -6.242252689847864744, -3.656250002048361036 ) ) ;
#7249=EDGE_CURVE ( 'NONE', #19560, #27517, #7063, .T. ) ;
#7250=DIRECTION ( 'NONE',  ( -0.000000000000000000, -0.000000000000000000, -1.000000000000000000 ) ) ;
#7256=ORIENTED_EDGE ( 'NONE', *, *, #35980, .T. ) ;
#7258=CARTESIAN_POINT ( 'NONE',  ( 7.644554776091147741E-16, 12.48450537969573659, -101.4687500020483668 ) ) ;
#7266=CARTESIAN_POINT ( 'NONE',  ( 10.00000000000000000, 5.773502691896255534, -43.87499999999996447 ) ) ;
#7269=LINE ( 'NONE', #32394, #26832 ) ;
#7271=CARTESIAN_POINT ( 'NONE',  ( 9.999999999999998224, 0.000000000000000000, -174.5000000000000284 ) ) ;
#7274=ADVANCED_FACE ( 'NONE', ( #26280 ), #18473, .T. ) ;
#7279=CARTESIAN_POINT ( 'NONE',  ( -10.81189881249999907, -6.242252689847864744, -67.96875000204838102 ) ) ;
#7280=VECTOR ( 'NONE', #22507, 1000.000000000000000 ) ;
#7281=CARTESIAN_POINT ( 'NONE',  ( -5.405949406250003975, -9.363379034771801557, -78.53125000204838102 ) ) ;
#7283=CARTESIAN_POINT ( 'NONE',  ( 10.81189881249999729, 0.000000000000000000, -159.0312500020484094 ) ) ;
#7284=CARTESIAN_POINT ( 'NONE',  ( 10.81189881249999907, 6.242252689847868297, -173.9062500020484094 ) ) ;
#7286=CARTESIAN_POINT ( 'NONE',  ( -24.99999999999999645, 0.000000000000000000, -99.99999999999998579 ) ) ;
#7288=CARTESIAN_POINT ( 'NONE',  ( -2.293366432827344421E-15, -12.48450537969573659, -103.7187500020483668 ) ) ;
#7291=CARTESIAN_POINT ( 'NONE',  ( -2.293366432827344421E-15, -12.48450537969573659, -7.906250002048365921 ) ) ;
#7295=CARTESIAN_POINT ( 'NONE',  ( 5.405949406249999534, 9.363379034771803333, -100.2812500020483952 ) ) ;
#7297=CARTESIAN_POINT ( 'NONE',  ( -4.999999999999996447, 8.660254037844387298, -73.87500000409677625 ) ) ;
#7299=CARTESIAN_POINT ( 'NONE',  ( 5.405949406249999534, 9.363379034771803333, -31.09375000204836326 ) ) ;
#7302=CARTESIAN_POINT ( 'NONE',  ( 5.405949406249999534, 9.363379034771803333, -26.78125000204836681 ) ) ;
#7305=CARTESIAN_POINT ( 'NONE',  ( -10.00000000000000000, -5.773502691896251982, -7.500000004096757600 ) ) ;
#7311=VERTEX_POINT ( 'NONE', #7271 ) ;
#7313=ORIENTED_EDGE ( 'NONE', *, *, #1727, .F. ) ;
#7319=AXIS2_PLACEMENT_3D ( 'NONE', #33453, #10, #3881 ) ;
#7321=DIRECTION ( 'NONE',  ( -1.000000000000000000, 0.000000000000000000, 0.000000000000000000 ) ) ;
#7323=CARTESIAN_POINT ( 'NONE',  ( -10.81189881249999907, -6.242252689847864744, -171.6562500020484094 ) ) ;
#7327=PRODUCT_DEFINITION_SHAPE ( 'NONE', 'NONE',  #14057 ) ;
#7328=CARTESIAN_POINT ( 'NONE',  ( -5.405949406249996869, 9.363379034771805109, -96.84375000204838102 ) ) ;
#7329=CARTESIAN_POINT ( 'NONE',  ( -5.405949406250003975, -9.363379034771801557, -198.3437500020484094 ) ) ;
#7330=CARTESIAN_POINT ( 'NONE',  ( -5.405949406250003975, -9.363379034771801557, -99.53125000204839523 ) ) ;
#7332=CARTESIAN_POINT ( 'NONE',  ( -5.405949406250003975, -9.363379034771801557, -109.8437500020483810 ) ) ;
#7336=CARTESIAN_POINT ( 'NONE',  ( -5.405949406249996869, 9.363379034771805109, -193.0312500020484094 ) ) ;
#7339=CARTESIAN_POINT ( 'NONE',  ( 5.000000000000000000, 8.660254037844385522, -168.6250000040967905 ) ) ;
#7341=CARTESIAN_POINT ( 'NONE',  ( -2.293366432827344421E-15, -12.48450537969573659, -18.21875000204836681 ) ) ;
#7343=CARTESIAN_POINT ( 'NONE',  ( 10.81189881249999729, 0.000000000000000000, -130.3437500020484094 ) ) ;
#7345=CARTESIAN_POINT ( 'NONE',  ( 10.81189881249999551, -6.242252689847874514, -25.65625000204838102 ) ) ;
#7348=CARTESIAN_POINT ( 'NONE',  ( -9.999999999999998224, 1.224646799147353059E-15, -58.24999999999997158 ) ) ;
#7349=CARTESIAN_POINT ( 'NONE',  ( 7.644554776091147741E-16, 12.48450537969573659, -122.6562500020483952 ) ) ;
#7351=EDGE_CURVE ( 'NONE', #7904, #11384, #30159, .T. ) ;
#7354=CARTESIAN_POINT ( 'NONE',  ( 5.000000000000000000, 8.660254037844385522, -104.1250000040967763 ) ) ;
#7356=CARTESIAN_POINT ( 'NONE',  ( -5.405949406249996869, 9.363379034771805109, -54.84375000204835970 ) ) ;
#7360=CARTESIAN_POINT ( 'NONE',  ( -9.999999999999998224, 0.000000000000000000, -99.99999999999998579 ) ) ;
#7361=CARTESIAN_POINT ( 'NONE',  ( 9.999999999999996447, -5.773502691896262640, -40.00000000409676204 ) ) ;
#7364=EDGE_LOOP ( 'NONE', ( #25566, #16658, #11441, #32016 ) ) ;
#7368=LINE ( 'NONE', #26794, #12770 ) ;
#7372=CARTESIAN_POINT ( 'NONE',  ( 10.81189881249999907, 6.242252689847868297, -196.4062500020484379 ) ) ;
#7378=CARTESIAN_POINT ( 'NONE',  ( -10.81189881249999907, -6.242252689847864744, -115.9687500020483810 ) ) ;
#7379=CARTESIAN_POINT ( 'NONE',  ( 9.999999999999998224, 0.000000000000000000, -195.8750000040967905 ) ) ;
#7380=CARTESIAN_POINT ( 'NONE',  ( -2.293366432827344421E-15, -12.48450537969573659, -121.9062500020483952 ) ) ;
#7382=CARTESIAN_POINT ( 'NONE',  ( -5.405949406250003975, -9.363379034771801557, -133.8437500020484094 ) ) ;
#7384=CARTESIAN_POINT ( 'NONE',  ( 7.070501591499376803E-16, 11.54700538379251284, -110.0000000040968047 ) ) ;
#7385=CARTESIAN_POINT ( 'NONE',  ( 4.999999999999992006, -8.660254037844389075, -155.2500000000000000 ) ) ;
#7386=CARTESIAN_POINT ( 'NONE',  ( 9.999999999999996447, -5.773502691896262640, -18.62499999999997868 ) ) ;
#7391=CARTESIAN_POINT ( 'NONE',  ( -10.81189881249999729, 6.242252689847871849, -48.71875000204836681 ) ) ;
#7392=CARTESIAN_POINT ( 'NONE',  ( -5.000000000000003553, -8.660254037844383745, -142.0000000000000000 ) ) ;
#7393=CARTESIAN_POINT ( 'NONE',  ( -5.405949406250003975, -9.363379034771801557, -150.3437500020483810 ) ) ;
#7397=CARTESIAN_POINT ( 'NONE',  ( 9.999999999999996447, -5.773502691896262640, -83.12499999999998579 ) ) ;
#7400=CARTESIAN_POINT ( 'NONE',  ( -10.81189881249999729, -6.242252689847864744, -110.1562500020483952 ) ) ;
#7401=CARTESIAN_POINT ( 'NONE',  ( 10.00000000000000000, 5.773502691896255534, -122.2500000040968047 ) ) ;
#7404=EDGE_CURVE ( 'NONE', #10629, #33014, #37570, .T. ) ;
#7406=CARTESIAN_POINT ( 'NONE',  ( -5.405949406249996869, 9.363379034771805109, -50.53125000204835970 ) ) ;
#7415=VERTEX_POINT ( 'NONE', #10493 ) ;
#7423=CARTESIAN_POINT ( 'NONE',  ( -10.81189881249999907, -6.242252689847864744, -138.4687500020484094 ) ) ;
#7424=CARTESIAN_POINT ( 'NONE',  ( 10.81189881249999729, 0.000000000000000000, -166.3437500020484094 ) ) ;
#7427=CARTESIAN_POINT ( 'NONE',  ( 9.999999999999998224, 0.000000000000000000, -176.0000000000000000 ) ) ;
#7431=CARTESIAN_POINT ( 'NONE',  ( -2.121150477449813534E-15, -11.54700538379251284, -124.2500000040967763 ) ) ;
#7432=CARTESIAN_POINT ( 'NONE',  ( -5.405949406249996869, 9.363379034771805109, -174.8437500020484094 ) ) ;
#7435=CARTESIAN_POINT ( 'NONE',  ( -10.81189881249999729, 1.324075727343319199E-15, -51.78125000204835970 ) ) ;
#7437=CARTESIAN_POINT ( 'NONE',  ( 9.999999999999998224, 0.000000000000000000, -109.9999999999999858 ) ) ;
#7439=CARTESIAN_POINT ( 'NONE',  ( 10.81189881249999729, 0.000000000000000000, -135.0312500020484094 ) ) ;
#7440=CARTESIAN_POINT ( 'NONE',  ( -9.999999999999998224, 5.773502691896259087, -154.7500000040967620 ) ) ;
#7441=CARTESIAN_POINT ( 'NONE',  ( 10.81189881249999551, -6.242252689847874514, -151.6562500020484094 ) ) ;
#7443=CARTESIAN_POINT ( 'NONE',  ( -5.405949406250003975, -9.363379034771801557, -81.34375000204838102 ) ) ;
#7447=CARTESIAN_POINT ( 'NONE',  ( 10.81189881249999907, 6.242252689847868297, -181.2187500020484094 ) ) ;
#7455=CARTESIAN_POINT ( 'NONE',  ( -10.81189881249999729, 6.242252689847871849, -72.90625000204838102 ) ) ;
#7457=CARTESIAN_POINT ( 'NONE',  ( -10.00000000000000000, -5.773502691896251982, -52.50000000409676915 ) ) ;
#7458=CARTESIAN_POINT ( 'NONE',  ( -10.81189881249999729, 1.324075727343319199E-15, -6.593750002048370362 ) ) ;
#7461=CARTESIAN_POINT ( 'NONE',  ( -10.81189881249999729, 6.242252689847871849, -5.406250002048363257 ) ) ;
#7463=CARTESIAN_POINT ( 'NONE',  ( 10.00000000000012257, -5.773502691896187144, -161.1250000000000568 ) ) ;
#7466=CARTESIAN_POINT ( 'NONE',  ( -9.999999999999998224, 1.224646799147353059E-15, -139.2499999999999716 ) ) ;
#7468=ORIENTED_EDGE ( 'NONE', *, *, #37933, .T. ) ;
#7470=VERTEX_POINT ( 'NONE', #41112 ) ;
#7476=CARTESIAN_POINT ( 'NONE',  ( 7.070501591499377789E-16, 11.54700538379251284, -46.62499999999997158 ) ) ;
#7480=CARTESIAN_POINT ( 'NONE',  ( -5.405949406249996869, 9.363379034771805109, -167.3437500020484094 ) ) ;
#7489=CARTESIAN_POINT ( 'NONE',  ( 10.81189881249999729, 0.000000000000000000, -65.84375000204836681 ) ) ;
#7490=CARTESIAN_POINT ( 'NONE',  ( 5.405949406249999534, 9.363379034771803333, -73.28125000204838102 ) ) ;
#7493=CARTESIAN_POINT ( 'NONE',  ( 7.644554776091147741E-16, 12.48450537969573659, -160.1562500020484094 ) ) ;
#7494=CARTESIAN_POINT ( 'NONE',  ( -10.81189881249999729, 1.324075727343319199E-15, -168.7812500020484094 ) ) ;
#7495=CARTESIAN_POINT ( 'NONE',  ( 7.644554776091147741E-16, 12.48450537969573659, 0.5312499979516493998 ) ) ;
#7497=CARTESIAN_POINT ( 'NONE',  ( -10.81189881249999907, -6.242252689847864744, -109.9687500020483668 ) ) ;
#7500=CARTESIAN_POINT ( 'NONE',  ( -10.81189881249999729, 6.242252689847871849, -2.406250002048360592 ) ) ;
#7503=CARTESIAN_POINT ( 'NONE',  ( -2.121150477449813534E-15, -11.54700538379251284, -168.8750000000000000 ) ) ;
#7504=CARTESIAN_POINT ( 'NONE',  ( -10.81189881249999729, 6.242252689847871849, -99.90625000204838102 ) ) ;
#7506=EDGE_CURVE ( 'NONE', #41312, #7415, #24538, .T. ) ;
#7508=CARTESIAN_POINT ( 'NONE',  ( 9.999999999999996447, -5.773502691896262640, -73.00000000409676204 ) ) ;
#7510=CARTESIAN_POINT ( 'NONE',  ( 5.405949406249999534, 9.363379034771803333, -32.59375000204836681 ) ) ;
#7514=CARTESIAN_POINT ( 'NONE',  ( -5.405949406250003975, -9.363379034771801557, -29.03125000204837036 ) ) ;
#7517=CARTESIAN_POINT ( 'NONE',  ( -2.121150477449813534E-15, -11.54700538379251284, -2.750000004096753159 ) ) ;
#7520=CARTESIAN_POINT ( 'NONE',  ( -4.999999999999996447, 8.660254037844387298, -123.0000000000000000 ) ) ;
#7523=CARTESIAN_POINT ( 'NONE',  ( -9.999999999999998224, 0.000000000000000000, -99.99999999999998579 ) ) ;
#7526=EDGE_CURVE ( 'NONE', #30761, #22978, #18542, .T. ) ;
#7530=CARTESIAN_POINT ( 'NONE',  ( -9.999999999999998224, 0.000000000000000000, -99.99999999999998579 ) ) ;
#7533=CARTESIAN_POINT ( 'NONE',  ( -5.405949406249996869, 9.363379034771805109, -170.5312500020484094 ) ) ;
#7536=CARTESIAN_POINT ( 'NONE',  ( 5.405949406249992428, -9.363379034771808662, -97.59375000204838102 ) ) ;
#7538=CARTESIAN_POINT ( 'NONE',  ( -5.405949406249996869, 9.363379034771805109, -103.0312500020483952 ) ) ;
#7540=CARTESIAN_POINT ( 'NONE',  ( -5.405949406249996869, 9.363379034771805109, -107.3437500020483810 ) ) ;
#7544=CARTESIAN_POINT ( 'NONE',  ( 10.81189881249999729, 0.000000000000000000, -196.5312500020484094 ) ) ;
#7548=CARTESIAN_POINT ( 'NONE',  ( -10.00000000000000000, -5.773502691896251982, -171.0000000040967905 ) ) ;
#7550=CARTESIAN_POINT ( 'NONE',  ( 5.405949406249999534, 9.363379034771803333, -22.09375000204835615 ) ) ;
#7551=DIRECTION ( 'NONE',  ( -1.000000000000000000, 0.000000000000000000, 0.000000000000000000 ) ) ;
#7552=CARTESIAN_POINT ( 'NONE',  ( 10.81189881249999907, 6.242252689847868297, -128.7187500020483810 ) ) ;
#7554=CARTESIAN_POINT ( 'NONE',  ( 5.405949406249992428, -9.363379034771808662, -28.78125000204837036 ) ) ;
#7557=CARTESIAN_POINT ( 'NONE',  ( -9.999999999999998224, 1.224646799147353059E-15, -59.74999999999997158 ) ) ;
#7558=CARTESIAN_POINT ( 'NONE',  ( -10.81189881249999729, 6.242252689847871849, -122.4062500020483952 ) ) ;
#7562=CARTESIAN_POINT ( 'NONE',  ( -5.000000000000003553, -8.660254037844383745, -100.3750000040967905 ) ) ;
#7563=DIRECTION ( 'NONE',  ( -1.000000000000000000, 0.000000000000000000, 0.000000000000000000 ) ) ;
#7564=CARTESIAN_POINT ( 'NONE',  ( -2.293366432827344421E-15, -12.48450537969573659, -55.71875000204837391 ) ) ;
#7565=ORIENTED_EDGE ( 'NONE', *, *, #28598, .F. ) ;
#7570=CARTESIAN_POINT ( 'NONE',  ( -9.999999999999998224, 1.224646799147353059E-15, -25.62500000409675849 ) ) ;
#7571=ADVANCED_FACE ( 'NONE', ( #17598 ), #23899, .F. ) ;
#7573=( BOUNDED_CURVE ( )  B_SPLINE_CURVE ( 2, ( #38902, #22294, #2023, #25540, #2445, #25748, #15786 ),
 .UNSPECIFIED., .F., .F. ) 
 B_SPLINE_CURVE_WITH_KNOTS ( ( 3, 2, 2, 3 ),
 ( 0.1082089552238805485, 0.1094527363184079616, 0.1106965174129353746, 0.1119402985074627876 ),
 .UNSPECIFIED. ) 
 CURVE ( )  GEOMETRIC_REPRESENTATION_ITEM ( )  RATIONAL_B_SPLINE_CURVE ( ( 1.000000000000004441, 0.8660254037844343777, 1.000000000000000000, 0.8660254037844387076, 1.000000000000000000, 0.8660254037844282715, 1.000000000000010436 ) ) 
 REPRESENTATION_ITEM ( '' )  );
#7579=DIRECTION ( 'NONE',  ( -1.000000000000000000, 0.000000000000000000, 0.000000000000000000 ) ) ;
#7583=CARTESIAN_POINT ( 'NONE',  ( -10.81189881249999729, 1.324075727343319199E-15, -194.2812500020484094 ) ) ;
#7589=CARTESIAN_POINT ( 'NONE',  ( -5.405949406249996869, 9.363379034771805109, -120.8437500020483952 ) ) ;
#7590=CARTESIAN_POINT ( 'NONE',  ( 7.070501591499377789E-16, 11.54700538379251284, -198.5000000040968189 ) ) ;
#7591=CARTESIAN_POINT ( 'NONE',  ( -10.81189881249999729, 1.324075727343319199E-15, -126.7812500020483668 ) ) ;
#7593=CARTESIAN_POINT ( 'NONE',  ( 5.405949406249999534, 9.363379034771803333, -130.0937500020483810 ) ) ;
#7596=CARTESIAN_POINT ( 'NONE',  ( -4.999999999999996447, 8.660254037844387298, -154.5000000000000000 ) ) ;
#7597=CARTESIAN_POINT ( 'NONE',  ( 7.070501591499377789E-16, 11.54700538379251284, -24.12499999999997868 ) ) ;
#7602=CARTESIAN_POINT ( 'NONE',  ( -5.405949406250003975, -9.363379034771801557, -42.34375000204837391 ) ) ;
#7604=CARTESIAN_POINT ( 'NONE',  ( 5.405949406249999534, 9.363379034771803333, -154.0937500020483810 ) ) ;
#7607=CARTESIAN_POINT ( 'NONE',  ( 10.63231620283895396, 1.921144686730597462, -180.0000000000000000 ) ) ;
#7608=CARTESIAN_POINT ( 'NONE',  ( 5.000000000000000000, 8.660254037844385522, -85.74999999999998579 ) ) ;
#7610=ORIENTED_EDGE ( 'NONE', *, *, #33066, .T. ) ;
#7611=CARTESIAN_POINT ( 'NONE',  ( 10.81189881249999729, 6.242252689847867408, -109.4062500020483952 ) ) ;
#7612=CARTESIAN_POINT ( 'NONE',  ( -4.999999999999996447, 8.660254037844387298, -127.8750000040967905 ) ) ;
#7617=CARTESIAN_POINT ( 'NONE',  ( 10.81189881249999551, -6.242252689847874514, -55.65625000204837391 ) ) ;
#7624=LINE ( 'NONE', #20994, #2469 ) ;
#7628=ORIENTED_EDGE ( 'NONE', *, *, #29925, .F. ) ;
#7629=EDGE_CURVE ( 'NONE', #17140, #40199, #30407, .T. ) ;
#7635=CARTESIAN_POINT ( 'NONE',  ( -9.999999999999998224, 1.224646799147353059E-15, -179.7500000000000284 ) ) ;
#7640=CARTESIAN_POINT ( 'NONE',  ( -10.81189881249999729, 1.324075727343319199E-15, -141.5937500020483810 ) ) ;
#7641=CARTESIAN_POINT ( 'NONE',  ( 5.405949406249992428, -9.363379034771808662, -153.0937500020483810 ) ) ;
#7644=CARTESIAN_POINT ( 'NONE',  ( -4.999999999999996447, 8.660254037844387298, -175.5000000000000284 ) ) ;
#7646=CARTESIAN_POINT ( 'NONE',  ( -3.547780718846140324, 10.23789773687130733, -99.99999999999994316 ) ) ;
#7649=CARTESIAN_POINT ( 'NONE',  ( 5.405949406249999534, 9.363379034771803333, -178.0937500020484094 ) ) ;
#7652=CARTESIAN_POINT ( 'NONE',  ( -4.999999999999996447, 8.660254037844387298, -115.4999999999999858 ) ) ;
#7653=CARTESIAN_POINT ( 'NONE',  ( -2.293366432827344421E-15, -12.48450537969573659, -51.40625000204837391 ) ) ;
#7655=CARTESIAN_POINT ( 'NONE',  ( 9.999999999999996447, -5.773502691896262640, -104.1249999999999858 ) ) ;
#7657=CARTESIAN_POINT ( 'NONE',  ( 5.405949406249992428, -9.363379034771808662, -133.7812500020483810 ) ) ;
#7658=CARTESIAN_POINT ( 'NONE',  ( 4.999999999999992006, -8.660254037844389075, -145.1250000040967905 ) ) ;
#7659=CARTESIAN_POINT ( 'NONE',  ( -10.81189881249999729, 1.324075727343319199E-15, -150.7812500020483810 ) ) ;
#7661=ORIENTED_EDGE ( 'NONE', *, *, #6173, .F. ) ;
#7663=CARTESIAN_POINT ( 'NONE',  ( 10.81189881249999551, -6.242252689847874514, -181.4687500020484094 ) ) ;
#7666=DIRECTION ( 'NONE',  ( -1.000000000000000000, 0.000000000000000000, 0.000000000000000000 ) ) ;
#7667=CARTESIAN_POINT ( 'NONE',  ( 10.81189881249999551, -6.242252689847874514, -79.65625000204838102 ) ) ;
#7669=AXIS2_PLACEMENT_3D ( 'NONE', #22746, #35913, #6136 ) ;
#7670=CARTESIAN_POINT ( 'NONE',  ( 9.999999999999996447, -5.773502691896262640, -50.50000000409676915 ) ) ;
#7671=CARTESIAN_POINT ( 'NONE',  ( -5.405949406249996869, 9.363379034771805109, -9.843750002048345493 ) ) ;
#7675=CARTESIAN_POINT ( 'NONE',  ( -5.405949406249996869, 9.363379034771805109, -5.531250002048376579 ) ) ;
#7676=DIRECTION ( 'NONE',  ( -1.000000000000000000, 0.000000000000000000, 0.000000000000000000 ) ) ;
#7677=DIRECTION ( 'NONE',  ( -0.000000000000000000, -0.000000000000000000, -1.000000000000000000 ) ) ;
#7678=DIRECTION ( 'NONE',  ( -0.000000000000000000, -0.000000000000000000, -1.000000000000000000 ) ) ;
#7691=EDGE_CURVE ( 'NONE', #17801, #23753, #40688, .T. ) ;
#7692=CARTESIAN_POINT ( 'NONE',  ( -4.999999999999996447, 8.660254037844387298, -44.99999999999998579 ) ) ;
#7695=CARTESIAN_POINT ( 'NONE',  ( 5.405949406249999534, 9.363379034771803333, -169.0937500020484094 ) ) ;
#7697=CARTESIAN_POINT ( 'NONE',  ( -10.81189881249999729, 6.242252689847871849, -174.7187500020484379 ) ) ;
#7700=CARTESIAN_POINT ( 'NONE',  ( 9.999999999999998224, 0.000000000000000000, -104.3750000040967763 ) ) ;
#7705=CYLINDRICAL_SURFACE ( 'NONE', #1809, 9.999999999999998224 ) ;
#7708=( BOUNDED_CURVE ( )  B_SPLINE_CURVE ( 2, ( #15777, #28974, #9320, #40351, #34501, #27206, #33489 ),
 .UNSPECIFIED., .F., .F. ) 
 B_SPLINE_CURVE_WITH_KNOTS ( ( 3, 2, 2, 3 ),
 ( 0.3022388059701494045, 0.3034825870646767343, 0.3047263681592040085, 0.3059701492537313383 ),
 .UNSPECIFIED. ) 
 CURVE ( )  GEOMETRIC_REPRESENTATION_ITEM ( )  RATIONAL_B_SPLINE_CURVE ( ( 0.9999999999999820144, 0.8660254037844566932, 1.000000000000000000, 0.8660254037844387076, 1.000000000000000000, 0.8660254037844387076, 1.000000000000000000 ) ) 
 REPRESENTATION_ITEM ( '' )  );
#7709=CARTESIAN_POINT ( 'NONE',  ( -10.81189881249999907, -6.242252689847864744, -69.46875000204838102 ) ) ;
#7710=CARTESIAN_POINT ( 'NONE',  ( -10.81189881249999907, -6.242252689847864744, -77.15625000204836681 ) ) ;
#7712=CARTESIAN_POINT ( 'NONE',  ( -9.999999999999998224, 5.773502691896259087, -128.8749999999999716 ) ) ;
#7713=CARTESIAN_POINT ( 'NONE',  ( 10.81189881249999729, 6.242252689847867408, -160.4062500020483810 ) ) ;
#7714=CARTESIAN_POINT ( 'NONE',  ( 10.81189881249999907, 6.242252689847868297, -170.9062500020484094 ) ) ;
#7716=DIRECTION ( 'NONE',  ( 1.000000000000000000, 0.000000000000000000, -0.000000000000000000 ) ) ;
#7717=PLANE ( 'NONE',  #14392 ) ;
#7718=CARTESIAN_POINT ( 'NONE',  ( 5.405949406249992428, -9.363379034771808662, -106.5937500020483810 ) ) ;
#7721=CARTESIAN_POINT ( 'NONE',  ( 10.81189881249999729, 0.000000000000000000, -1.531250002048373249 ) ) ;
#7723=CARTESIAN_POINT ( 'NONE',  ( -9.999999999999998224, 1.224646799147353059E-15, -169.2500000000000000 ) ) ;
#7724=CARTESIAN_POINT ( 'NONE',  ( -10.81189881249999729, 1.324075727343319199E-15, -98.28125000204839523 ) ) ;
#7726=CARTESIAN_POINT ( 'NONE',  ( 9.999999999999996447, -5.773502691896262640, -77.50000000409677625 ) ) ;
#7727=CARTESIAN_POINT ( 'NONE',  ( -10.81189881249999907, -6.242252689847864744, -34.96875000204835260 ) ) ;
#7728=ORIENTED_EDGE ( 'NONE', *, *, #12285, .T. ) ;
#7730=CARTESIAN_POINT ( 'NONE',  ( -10.81189881249999907, -6.242252689847864744, -30.65625000204835970 ) ) ;
#7733=CARTESIAN_POINT ( 'NONE',  ( -2.121150477449813534E-15, -11.54700538379251284, -1.250000004096751827 ) ) ;
#7739=EDGE_LOOP ( 'NONE', ( #17673, #41789, #9274, #16614 ) ) ;
#7741=ORIENTED_EDGE ( 'NONE', *, *, #41735, .T. ) ;
#7742=ORIENTED_EDGE ( 'NONE', *, *, #8237, .F. ) ;
#7748=EDGE_CURVE ( 'NONE', #36438, #8116, #902, .T. ) ;
#7753=CARTESIAN_POINT ( 'NONE',  ( -10.81189881249999907, -6.242252689847864744, -168.6562500020483810 ) ) ;
#7758=CARTESIAN_POINT ( 'NONE',  ( 7.644554776091147741E-16, 12.48450537969573659, -96.96875000204838102 ) ) ;
#7760=FACE_OUTER_BOUND ( 'NONE', #38550, .T. ) ;
#7761=CARTESIAN_POINT ( 'NONE',  ( 5.405949406249999534, 9.363379034771803333, -97.28125000204839523 ) ) ;
#7763=CARTESIAN_POINT ( 'NONE',  ( -10.81189881249999729, 1.324075727343319199E-15, -110.0937500020483810 ) ) ;
#7768=CARTESIAN_POINT ( 'NONE',  ( -2.293366432827344421E-15, -12.48450537969573659, -196.9062500020484094 ) ) ;
#7771=CARTESIAN_POINT ( 'NONE',  ( 9.999999999999996447, -5.773502691896262640, -173.5000000040968189 ) ) ;
#7773=CARTESIAN_POINT ( 'NONE',  ( 10.81189881249999729, 0.000000000000000000, -17.84375000204835260 ) ) ;
#7775=CARTESIAN_POINT ( 'NONE',  ( -10.81189881249999729, 1.324075727343319199E-15, -128.0937500020483810 ) ) ;
#7777=CARTESIAN_POINT ( 'NONE',  ( -10.81189881249999907, -6.242252689847864744, -26.15625000204838102 ) ) ;
#7780=CARTESIAN_POINT ( 'NONE',  ( -5.000000000000003553, -8.660254037844383745, -62.49999999999997158 ) ) ;
#7781=CARTESIAN_POINT ( 'NONE',  ( 7.644554776091147741E-16, 12.48450537969573659, -121.1562500020483952 ) ) ;
#7785=CARTESIAN_POINT ( 'NONE',  ( -4.999999999999996447, 8.660254037844387298, -99.37500000409679046 ) ) ;
#7786=CARTESIAN_POINT ( 'NONE',  ( 10.00000000000076916, -5.773502691895816774, -113.1249999999999716 ) ) ;
#7788=CARTESIAN_POINT ( 'NONE',  ( 5.405949406249999534, 9.363379034771803333, -58.09375000204835970 ) ) ;
#7790=EDGE_CURVE ( 'NONE', #17641, #25374, #8560, .T. ) ;
#7796=CARTESIAN_POINT ( 'NONE',  ( -9.999999999999998224, 5.773502691896259087, -25.75000000409677625 ) ) ;
#7805=CARTESIAN_POINT ( 'NONE',  ( -10.81189881249999729, 6.242252689847871849, -195.9062500020484094 ) ) ;
#7811=CARTESIAN_POINT ( 'NONE',  ( 10.81189881249999907, 6.242252689847868297, -116.7187500020483810 ) ) ;
#7812=CARTESIAN_POINT ( 'NONE',  ( 10.00000000000000000, 5.773502691896255534, -198.7500000040968189 ) ) ;
#7813=CARTESIAN_POINT ( 'NONE',  ( -5.405949406250003975, -9.363379034771801557, -123.5312500020483952 ) ) ;
#7815=CARTESIAN_POINT ( 'NONE',  ( 10.81189881249999551, -6.242252689847874514, -127.4687500020483810 ) ) ;
#7816=CARTESIAN_POINT ( 'NONE',  ( 9.999999999999998224, 0.000000000000000000, -174.8750000040967905 ) ) ;
#7818=CARTESIAN_POINT ( 'NONE',  ( 10.00000000000000000, 5.773502691896255534, -157.8749999999999716 ) ) ;
#7819=CARTESIAN_POINT ( 'NONE',  ( 9.999999999999998224, 0.000000000000000000, -16.99999999999996092 ) ) ;
#7825=CARTESIAN_POINT ( 'NONE',  ( 5.405949406249999534, 9.363379034771803333, -44.59375000204837391 ) ) ;
#7826=CARTESIAN_POINT ( 'NONE',  ( -2.121150477449813534E-15, -11.54700538379251284, -110.7500000040967620 ) ) ;
#7827=CARTESIAN_POINT ( 'NONE',  ( 10.81189881249999729, 0.000000000000000000, -157.3437500020483810 ) ) ;
#7831=CARTESIAN_POINT ( 'NONE',  ( 9.999999999999996447, -5.773502691896262640, -86.12499999999998579 ) ) ;
#7834=CARTESIAN_POINT ( 'NONE',  ( 10.81189881249999729, 0.000000000000000000, -105.0312500020483810 ) ) ;
#7835=CARTESIAN_POINT ( 'NONE',  ( 10.00000000000000000, 5.773502691896255534, -120.7500000040967905 ) ) ;
#7840=CARTESIAN_POINT ( 'NONE',  ( -10.81189881249999729, 1.324075727343319199E-15, -42.78125000204838102 ) ) ;
#7848=VERTEX_POINT ( 'NONE', #9182 ) ;
#7854=CARTESIAN_POINT ( 'NONE',  ( -9.999999999999998224, 1.224646799147353059E-15, -153.1250000040967905 ) ) ;
#7859=CARTESIAN_POINT ( 'NONE',  ( 10.81189881249999551, -6.242252689847874514, -145.4687500020483810 ) ) ;
#7860=CARTESIAN_POINT ( 'NONE',  ( 10.81189881249999729, 0.000000000000000000, -151.5312500020484094 ) ) ;
#7861=CARTESIAN_POINT ( 'NONE',  ( -10.81189881249999729, 1.324075727343319199E-15, -152.0937500020483810 ) ) ;
#7863=DIRECTION ( 'NONE',  ( -0.000000000000000000, -0.000000000000000000, -1.000000000000000000 ) ) ;
#7864=CARTESIAN_POINT ( 'NONE',  ( -9.999999999999998224, 1.224646799147353059E-15, -179.7500000000000284 ) ) ;
#7866=LINE ( 'NONE', #34626, #3124 ) ;
#7869=CARTESIAN_POINT ( 'NONE',  ( 10.81189881249999729, 0.000000000000000000, -179.8437500020483810 ) ) ;
#7872=FACE_OUTER_BOUND ( 'NONE', #13813, .T. ) ;
#7873=CARTESIAN_POINT ( 'NONE',  ( 5.405949406249999534, 9.363379034771803333, -47.78125000204838813 ) ) ;
#7875=CARTESIAN_POINT ( 'NONE',  ( -9.999999999999998224, 5.773502691896259087, -106.3749999999999858 ) ) ;
#7876=( BOUNDED_CURVE ( )  B_SPLINE_CURVE ( 2, ( #37147, #27228, #709, #17928, #36941, #34150, #31126 ),
 .UNSPECIFIED., .F., .F. ) 
 B_SPLINE_CURVE_WITH_KNOTS ( ( 3, 2, 2, 3 ),
 ( 0.1791044776119403437, 0.1803482587064677289, 0.1815920398009950587, 0.1828358208955224162 ),
 .UNSPECIFIED. ) 
 CURVE ( )  GEOMETRIC_REPRESENTATION_ITEM ( )  RATIONAL_B_SPLINE_CURVE ( ( 0.9999999999999940048, 0.8660254037844447028, 1.000000000000000000, 0.8660254037844387076, 1.000000000000000000, 0.8660254037844357100, 1.000000000000003109 ) ) 
 REPRESENTATION_ITEM ( '' )  );
#7878=CARTESIAN_POINT ( 'NONE',  ( -10.81189881249999729, 6.242252689847871849, -125.4062500020483810 ) ) ;
#7879=CARTESIAN_POINT ( 'NONE',  ( -5.000000000000003553, -8.660254037844383745, -145.3750000040967905 ) ) ;
#7883=CARTESIAN_POINT ( 'NONE',  ( -5.405949406249996869, 9.363379034771805109, -170.3437500020484094 ) ) ;
#7887=CARTESIAN_POINT ( 'NONE',  ( -2.293366432827344421E-15, -12.48450537969573659, -72.40625000204836681 ) ) ;
#7889=ADVANCED_FACE ( 'NONE', ( #21711 ), #35529, .F. ) ;
#7890=CARTESIAN_POINT ( 'NONE',  ( 7.070501591499377789E-16, 11.54700538379251284, -50.00000000409676204 ) ) ;
#7891=CARTESIAN_POINT ( 'NONE',  ( -10.81189881249999907, -6.242252689847864744, -7.968750002048358816 ) ) ;
#7894=CARTESIAN_POINT ( 'NONE',  ( -10.81189881249999729, 1.324075727343319199E-15, -8.281250002048350822 ) ) ;
#7897=LINE ( 'NONE', #14336, #25641 ) ;
#7901=CARTESIAN_POINT ( 'NONE',  ( 9.999999999999998224, 0.000000000000000000, -141.8750000040967905 ) ) ;
#7903=VERTEX_POINT ( 'NONE', #35738 ) ;
#7904=VERTEX_POINT ( 'NONE', #18469 ) ;
#7911=CARTESIAN_POINT ( 'NONE',  ( 4.999999999999992006, -8.660254037844389075, -42.74999999999998579 ) ) ;
#7913=CARTESIAN_POINT ( 'NONE',  ( -2.293366432827344421E-15, -12.48450537969573659, -165.2187500020484094 ) ) ;
#7914=CARTESIAN_POINT ( 'NONE',  ( -5.405949406249996869, 9.363379034771805109, -174.8437500020484094 ) ) ;
#7923=CARTESIAN_POINT ( 'NONE',  ( -5.405949406250003975, -9.363379034771801557, -64.84375000204836681 ) ) ;
#7924=CARTESIAN_POINT ( 'NONE',  ( 5.405949406249999534, 9.363379034771803333, -65.78125000204838102 ) ) ;
#7926=CARTESIAN_POINT ( 'NONE',  ( 9.999999999999996447, -5.773502691896262640, -132.6249999999999716 ) ) ;
#7927=CARTESIAN_POINT ( 'NONE',  ( 5.405949406249992428, -9.363379034771808662, -147.2812500020483810 ) ) ;
#7928=CARTESIAN_POINT ( 'NONE',  ( 7.644554776091147741E-16, 12.48450537969573659, -173.6562500020483810 ) ) ;
#7929=FACE_OUTER_BOUND ( 'NONE', #10994, .T. ) ;
#7931=CARTESIAN_POINT ( 'NONE',  ( -2.293366432827344421E-15, -12.48450537969573659, -96.21875000204839523 ) ) ;
#7932=CARTESIAN_POINT ( 'NONE',  ( -9.999999999999998224, 1.224646799147353059E-15, -155.7500000000000000 ) ) ;
#7934=CARTESIAN_POINT ( 'NONE',  ( 10.81189881249999551, -6.242252689847874514, -6.156250002048363257 ) ) ;
#7937=CARTESIAN_POINT ( 'NONE',  ( -10.81189881249999729, 6.242252689847871849, -96.90625000204838102 ) ) ;
#7939=CARTESIAN_POINT ( 'NONE',  ( 7.070501591499377789E-16, 11.54700538379251284, -78.50000000409677625 ) ) ;
#7940=CARTESIAN_POINT ( 'NONE',  ( 7.644554776091147741E-16, 12.48450537969573659, -35.46875000204835260 ) ) ;
#7943=CARTESIAN_POINT ( 'NONE',  ( 7.644554776091147741E-16, 12.48450537969573659, -31.15625000204835970 ) ) ;
#7947=CARTESIAN_POINT ( 'NONE',  ( 9.999999999999996447, -5.773502691896262640, -4.000000004096754047 ) ) ;
#7951=CARTESIAN_POINT ( 'NONE',  ( -10.00000000000051337, 5.773502691895962435, -119.8749999999999858 ) ) ;
#7955=ORIENTED_EDGE ( 'NONE', *, *, #9727, .T. ) ;
#7964=CARTESIAN_POINT ( 'NONE',  ( -4.999999999999996447, 8.660254037844387298, -105.3750000040967763 ) ) ;
#7965=CARTESIAN_POINT ( 'NONE',  ( -2.293366432827344421E-15, -12.48450537969573659, -160.9062500020483810 ) ) ;
#7967=CARTESIAN_POINT ( 'NONE',  ( -2.293366432827344421E-15, -12.48450537969573659, -93.21875000204838102 ) ) ;
#7969=CARTESIAN_POINT ( 'NONE',  ( -10.81189881249999729, 6.242252689847871849, -194.2187500020483810 ) ) ;
#7970=CARTESIAN_POINT ( 'NONE',  ( -2.293366432827344421E-15, -12.48450537969573659, -102.4062500020483952 ) ) ;
#7972=CARTESIAN_POINT ( 'NONE',  ( 5.405949406249999534, 9.363379034771803333, -107.5937500020483810 ) ) ;
#7975=CARTESIAN_POINT ( 'NONE',  ( -10.81189881249999907, -6.242252689847864744, -197.1562500020484379 ) ) ;
#7977=CARTESIAN_POINT ( 'NONE',  ( -4.999999999999996447, 8.660254037844387298, -171.3750000040968189 ) ) ;
#7979=CARTESIAN_POINT ( 'NONE',  ( -2.293366432827344421E-15, -12.48450537969573659, -22.71875000204837391 ) ) ;
#7981=CARTESIAN_POINT ( 'NONE',  ( -10.81189881249999907, -6.242252689847864744, -130.9687500020483810 ) ) ;
#7983=CARTESIAN_POINT ( 'NONE',  ( 7.644554776091147741E-16, 12.48450537969573659, -31.15625000204835970 ) ) ;
#7986=CARTESIAN_POINT ( 'NONE',  ( -10.00000000000000000, -5.773502691896251982, -50.62499999999997158 ) ) ;
#7987=CARTESIAN_POINT ( 'NONE',  ( -5.405949406250003975, -9.363379034771801557, -125.0312500020483952 ) ) ;
#7990=CARTESIAN_POINT ( 'NONE',  ( 9.999999999999996447, -5.773502691896262640, -103.0000000040967620 ) ) ;
#7992=CARTESIAN_POINT ( 'NONE',  ( 5.405949406249999534, 9.363379034771803333, -55.09375000204835970 ) ) ;
#7999=CARTESIAN_POINT ( 'NONE',  ( -9.999999999999998224, 5.773502691896259087, -24.25000000409677270 ) ) ;
#8000=EDGE_CURVE ( 'NONE', #41312, #25900, #9706, .T. ) ;
#8006=CIRCLE ( 'NONE', #13489, 22.00000000000000711 ) ;
#8008=EDGE_LOOP ( 'NONE', ( #41565, #5511, #29074, #28291 ) ) ;
#8014=FACE_OUTER_BOUND ( 'NONE', #41321, .T. ) ;
#8015=CARTESIAN_POINT ( 'NONE',  ( -9.999999999999998224, 1.224646799147353059E-15, -174.1250000040968189 ) ) ;
#8018=ADVANCED_FACE ( 'NONE', ( #30106 ), #42394, .F. ) ;
#8019=CARTESIAN_POINT ( 'NONE',  ( -5.405949406249996869, 9.363379034771805109, -193.0312500020484094 ) ) ;
#8021=ADVANCED_FACE ( 'NONE', ( #331 ), #29463, .F. ) ;
#8025=CARTESIAN_POINT ( 'NONE',  ( -2.293366432827344421E-15, -12.48450537969573659, -114.2187500020483668 ) ) ;
#8026=CARTESIAN_POINT ( 'NONE',  ( -10.81189881249999907, -6.242252689847864744, -0.4687500020483514329 ) ) ;
#8027=CARTESIAN_POINT ( 'NONE',  ( 5.405949406249999534, 9.363379034771803333, -125.7812500020483668 ) ) ;
#8029=CARTESIAN_POINT ( 'NONE',  ( 5.405949406249992428, -9.363379034771808662, -132.0937500020483810 ) ) ;
#8030=CARTESIAN_POINT ( 'NONE',  ( -2.121150477449813534E-15, -11.54700538379251284, -166.2500000040968189 ) ) ;
#8031=CARTESIAN_POINT ( 'NONE',  ( 9.999999999999998224, 0.000000000000000000, -110.3750000040967763 ) ) ;
#8032=CARTESIAN_POINT ( 'NONE',  ( -2.121150477449813534E-15, -11.54700538379251284, -147.8750000000000000 ) ) ;
#8033=CARTESIAN_POINT ( 'NONE',  ( -4.999999999999996447, 8.660254037844387298, -23.99999999999996447 ) ) ;
#8038=CARTESIAN_POINT ( 'NONE',  ( 7.644554776091147741E-16, 12.48450537969573659, -48.96875000204836681 ) ) ;
#8039=DIRECTION ( 'NONE',  ( 0.000000000000000000, 0.000000000000000000, -1.000000000000000000 ) ) ;
#8040=CARTESIAN_POINT ( 'NONE',  ( 7.644554776091147741E-16, 12.48450537969573659, -155.4687500020484094 ) ) ;
#8043=CARTESIAN_POINT ( 'NONE',  ( -1.048820568758768168, 10.15334972493218757, -180.0000000000000000 ) ) ;
#8044=CARTESIAN_POINT ( 'NONE',  ( 9.999999999999998224, 0.000000000000000000, -76.99999999999998579 ) ) ;
#8047=CARTESIAN_POINT ( 'NONE',  ( 5.405949406249999534, 9.363379034771803333, -101.7812500020483952 ) ) ;
#8048=CARTESIAN_POINT ( 'NONE',  ( 9.999999999999996447, -5.773502691896262640, -124.0000000040967763 ) ) ;
#8051=CARTESIAN_POINT ( 'NONE',  ( -9.999999999999998224, 1.224646799147353059E-15, -130.2499999999999716 ) ) ;
#8052=CARTESIAN_POINT ( 'NONE',  ( -5.405949406250003975, -9.363379034771801557, -45.53125000204838102 ) ) ;
#8053=EDGE_CURVE ( 'NONE', #33176, #36280, #5313, .T. ) ;
#8057=CARTESIAN_POINT ( 'NONE',  ( 9.999999999999998224, 0.000000000000000000, -109.9999999999999858 ) ) ;
#8058=EDGE_LOOP ( 'NONE', ( #5118, #16560, #17375, #27245 ) ) ;
#8061=ORIENTED_EDGE ( 'NONE', *, *, #23971, .F. ) ;
#8067=CARTESIAN_POINT ( 'NONE',  ( 5.000000000000000000, 8.660254037844385522, -153.6250000040967905 ) ) ;
#8071=CARTESIAN_POINT ( 'NONE',  ( -5.405949406249996869, 9.363379034771805109, -143.3437500020483810 ) ) ;
#8072=CARTESIAN_POINT ( 'NONE',  ( 5.405949406249992428, -9.363379034771808662, -145.7812500020483810 ) ) ;
#8073=CARTESIAN_POINT ( 'NONE',  ( -5.405949406250003975, -9.363379034771801557, -151.8437500020483810 ) ) ;
#8076=CARTESIAN_POINT ( 'NONE',  ( -9.999999999999998224, 1.224646799147353059E-15, -169.2500000000000000 ) ) ;
#8078=CARTESIAN_POINT ( 'NONE',  ( 9.999999999999998224, 0.000000000000000000, -103.9999999999999858 ) ) ;
#8080=DIRECTION ( 'NONE',  ( -0.000000000000000000, -0.000000000000000000, -1.000000000000000000 ) ) ;
#8081=CARTESIAN_POINT ( 'NONE',  ( 10.81189881249999907, 6.242252689847868297, -176.7187500020483810 ) ) ;
#8085=DIRECTION ( 'NONE',  ( -1.000000000000000000, 0.000000000000000000, 0.000000000000000000 ) ) ;
#8086=CARTESIAN_POINT ( 'NONE',  ( 10.81189881249999729, 0.000000000000000000, -48.03125000204838813 ) ) ;
#8088=CARTESIAN_POINT ( 'NONE',  ( 9.999999999999996447, -5.773502691896262640, -105.6249999999999858 ) ) ;
#8090=CARTESIAN_POINT ( 'NONE',  ( 10.81189881249999729, 0.000000000000000000, -127.5312500020483952 ) ) ;
#8091=CARTESIAN_POINT ( 'NONE',  ( 10.00000000000000000, 5.773502691896255534, -146.2500000040967905 ) ) ;
#8095=CARTESIAN_POINT ( 'NONE',  ( -5.405949406249996869, 9.363379034771805109, -174.8437500020484094 ) ) ;
#8099=CARTESIAN_POINT ( 'NONE',  ( 5.405949406249992428, -9.363379034771808662, -72.28125000204838102 ) ) ;
#8101=CARTESIAN_POINT ( 'NONE',  ( 9.999999999999998224, 0.000000000000000000, -42.87500000409677625 ) ) ;
#8102=CARTESIAN_POINT ( 'NONE',  ( 10.81189881249999551, -6.242252689847874514, -2.968750002048353931 ) ) ;
#8105=CARTESIAN_POINT ( 'NONE',  ( 9.999999999999998224, 0.000000000000000000, -128.0000000000000000 ) ) ;
#8107=ORIENTED_EDGE ( 'NONE', *, *, #37289, .T. ) ;
#8109=LINE ( 'NONE', #17577, #42420 ) ;
#8116=VERTEX_POINT ( 'NONE', #33351 ) ;
#8121=EDGE_LOOP ( 'NONE', ( #2733, #26895, #18228, #32065 ) ) ;
#8123=CARTESIAN_POINT ( 'NONE',  ( -10.00000000000000000, -5.773502691896251982, -40.12499999999996447 ) ) ;
#8125=CARTESIAN_POINT ( 'NONE',  ( -10.81189881249999729, 1.324075727343319199E-15, -165.5937500020484094 ) ) ;
#8139=CARTESIAN_POINT ( 'NONE',  ( 5.405949406249999534, 9.363379034771803333, -64.09375000204836681 ) ) ;
#8140=CARTESIAN_POINT ( 'NONE',  ( -5.405949406249996869, 9.363379034771805109, -68.53125000204838102 ) ) ;
#8142=CARTESIAN_POINT ( 'NONE',  ( 9.999999999999998224, 0.000000000000000000, -131.0000000000000000 ) ) ;
#8143=CARTESIAN_POINT ( 'NONE',  ( 5.405949406249992428, -9.363379034771808662, -150.2812500020483810 ) ) ;
#8144=CARTESIAN_POINT ( 'NONE',  ( 5.405949406249992428, -9.363379034771808662, -162.2812500020484094 ) ) ;
#8147=CARTESIAN_POINT ( 'NONE',  ( -10.81189881249999907, -6.242252689847864744, -97.96875000204838102 ) ) ;
#8150=CARTESIAN_POINT ( 'NONE',  ( -10.81189881249999907, -6.242252689847864744, -198.4687500020484379 ) ) ;
#8153=CARTESIAN_POINT ( 'NONE',  ( -2.293366432827344421E-15, -12.48450537969573659, -93.40625000204839523 ) ) ;
#8155=CARTESIAN_POINT ( 'NONE',  ( 10.00000000000000000, 5.773502691896255534, -66.75000000409677625 ) ) ;
#8157=CARTESIAN_POINT ( 'NONE',  ( 5.405949406249999534, 9.363379034771803333, -26.59375000204835970 ) ) ;
#8160=CARTESIAN_POINT ( 'NONE',  ( 10.81189881249999907, 6.242252689847868297, -28.40625000204838457 ) ) ;
#8163=CARTESIAN_POINT ( 'NONE',  ( -9.999999999999998224, 1.224646799147353059E-15, -7.625000004096743389 ) ) ;
#8181=CARTESIAN_POINT ( 'NONE',  ( -5.405949406249996869, 9.363379034771805109, -167.5312500020484094 ) ) ;
#8183=EDGE_CURVE ( 'NONE', #36337, #3574, #28774, .T. ) ;
#8185=CARTESIAN_POINT ( 'NONE',  ( 10.81189881249999551, -6.242252689847874514, -83.96875000204838102 ) ) ;
#8187=CARTESIAN_POINT ( 'NONE',  ( 7.644554776091147741E-16, 12.48450537969573659, -195.9687500020484094 ) ) ;
#8188=CARTESIAN_POINT ( 'NONE',  ( 10.81189881249999551, -6.242252689847874514, -91.65625000204838102 ) ) ;
#8192=CARTESIAN_POINT ( 'NONE',  ( 10.81189881249999729, 0.000000000000000000, -172.5312500020484094 ) ) ;
#8193=CARTESIAN_POINT ( 'NONE',  ( 5.405949406249999534, 9.363379034771803333, -188.7812500020484094 ) ) ;
#8195=CARTESIAN_POINT ( 'NONE',  ( -4.999999999999996447, 8.660254037844387298, -163.8750000040967905 ) ) ;
#8197=CARTESIAN_POINT ( 'NONE',  ( 5.405949406249992428, -9.363379034771808662, -10.59375000204834727 ) ) ;
#8198=DIRECTION ( 'NONE',  ( -0.000000000000000000, -0.000000000000000000, -1.000000000000000000 ) ) ;
#8199=CARTESIAN_POINT ( 'NONE',  ( -5.405949406250003975, -9.363379034771801557, -124.8437500020483810 ) ) ;
#8201=CARTESIAN_POINT ( 'NONE',  ( 5.405949406249992428, -9.363379034771808662, -19.78125000204836326 ) ) ;
#8205=CARTESIAN_POINT ( 'NONE',  ( -4.999999999999996447, 8.660254037844387298, -53.99999999999996447 ) ) ;
#8206=CARTESIAN_POINT ( 'NONE',  ( 10.81189881249999729, 0.000000000000000000, -124.5312500020483952 ) ) ;
#8209=B_SPLINE_CURVE_WITH_KNOTS ( 'NONE', 3,
 ( #27599, #5152, #33869, #1277, #11182, #14628, #24378, #40948, #38581, #41808, #42234, #34940, #25854, #15051, #25021, #21762, #38802, #28248, #6217, #12450, #9024, #31922, #22190, #28471, #2350, #19153, #15272, #8608 ),
 .UNSPECIFIED., .F., .F.,
 ( 4, 2, 2, 2, 2, 2, 2, 2, 2, 2, 2, 2, 2, 4 ),
 ( 1.019784333705586920E-15, 0.001286352574010762471, 0.002572705148020504925, 0.005145410296039989832, 0.006431762870049733370, 0.007718115444059476908, 0.009004468018069223048, 0.01029082059207896659, 0.01286352574009845713, 0.01543623088811794594, 0.01672258346212769295, 0.01800893603613743649, 0.01929528861014718349, 0.02058164118415692703 ),
 .UNSPECIFIED. ) ;
#8210=CARTESIAN_POINT ( 'NONE',  ( -10.00000000000000000, -5.773502691896251982, -97.50000000409679046 ) ) ;
#8211=CARTESIAN_POINT ( 'NONE',  ( 9.999999999999998224, 1.224646799147353059E-15, -99.99999999999998579 ) ) ;
#8213=CARTESIAN_POINT ( 'NONE',  ( 7.644554776091147741E-16, 12.48450537969573659, -56.46875000204837391 ) ) ;
#8214=ORIENTED_EDGE ( 'NONE', *, *, #36718, .T. ) ;
#8219=CARTESIAN_POINT ( 'NONE',  ( -9.999999999999998224, 1.224646799147353059E-15, -27.12500000409676204 ) ) ;
#8232=CARTESIAN_POINT ( 'NONE',  ( -10.81189881249999729, 6.242252689847871849, -185.4062500020484094 ) ) ;
#8235=ADVANCED_FACE ( 'NONE', ( #33982 ), #11072, .F. ) ;
#8237=EDGE_CURVE ( 'NONE', #15924, #21752, #16877, .T. ) ;
#8239=CARTESIAN_POINT ( 'NONE',  ( -5.405949406249996869, 9.363379034771805109, -108.8437500020483810 ) ) ;
#8241=CARTESIAN_POINT ( 'NONE',  ( -5.405949406250003975, -9.363379034771801557, -114.5312500020483952 ) ) ;
#8243=CARTESIAN_POINT ( 'NONE',  ( 7.644554776091147741E-16, 12.48450537969573659, -128.4687500020483810 ) ) ;
#8246=CARTESIAN_POINT ( 'NONE',  ( 0.000000000000000000, 0.000000000000000000, -99.99999999999998579 ) ) ;
#8247=CARTESIAN_POINT ( 'NONE',  ( -5.000000000000003553, -8.660254037844383745, -151.0000000000000000 ) ) ;
#8248=CARTESIAN_POINT ( 'NONE',  ( -2.121150477449813534E-15, -11.54700538379251284, -12.87499999999996803 ) ) ;
#8253=CARTESIAN_POINT ( 'NONE',  ( 10.81189881249999907, 6.242252689847868297, -49.21875000204835970 ) ) ;
#8255=CARTESIAN_POINT ( 'NONE',  ( 7.644554776091147741E-16, 12.48450537969573659, -144.9687500020483810 ) ) ;
#8258=CARTESIAN_POINT ( 'NONE',  ( 4.999999999999992006, -8.660254037844389075, -72.74999999999998579 ) ) ;
#8260=( BOUNDED_CURVE ( )  B_SPLINE_CURVE ( 2, ( #37508, #11379, #17635, #21538, #30829, #7951, #15259 ),
 .UNSPECIFIED., .F., .F. ) 
 B_SPLINE_CURVE_WITH_KNOTS ( ( 3, 2, 2, 3 ),
 ( 0.3955223880597015795, 0.3967661691542289648, 0.3980099502487563501, 0.3992537313432836799 ),
 .UNSPECIFIED. ) 
 CURVE ( )  GEOMETRIC_REPRESENTATION_ITEM ( )  RATIONAL_B_SPLINE_CURVE ( ( 0.9999999999999880096, 0.8660254037844506980, 1.000000000000000000, 0.8660254037844387076, 1.000000000000000000, 0.8660254037844267172, 1.000000000000011990 ) ) 
 REPRESENTATION_ITEM ( '' )  );
#8262=CARTESIAN_POINT ( 'NONE',  ( 10.81189881249999551, -6.242252689847874514, -100.6562500020483952 ) ) ;
#8263=CARTESIAN_POINT ( 'NONE',  ( 5.000000000000000000, 8.660254037844385522, -122.1250000040967905 ) ) ;
#8264=CARTESIAN_POINT ( 'NONE',  ( 7.644554776091147741E-16, 12.48450537969573659, -80.46875000204838102 ) ) ;
#8267=CARTESIAN_POINT ( 'NONE',  ( 10.81189881249999551, -6.242252689847874514, -48.15625000204837391 ) ) ;
#8279=CARTESIAN_POINT ( 'NONE',  ( -9.999999999999998224, 1.224646799147353059E-15, -103.2500000000000000 ) ) ;
#8282=CARTESIAN_POINT ( 'NONE',  ( 9.999999999999998224, 1.224646799147353059E-15, -99.99999999999998579 ) ) ;
#8287=CARTESIAN_POINT ( 'NONE',  ( -9.999999999999998224, 1.224646799147353059E-15, -112.2499999999999858 ) ) ;
#8288=CARTESIAN_POINT ( 'NONE',  ( 7.644554776091147741E-16, 12.48450537969573659, -141.9687500020483810 ) ) ;
#8289=CARTESIAN_POINT ( 'NONE',  ( 5.405949406249999534, 9.363379034771803333, -148.2812500020483810 ) ) ;
#8290=CARTESIAN_POINT ( 'NONE',  ( 5.405949406249999534, 9.363379034771803333, -157.0937500020483810 ) ) ;
#8294=CARTESIAN_POINT ( 'NONE',  ( 7.070501591499377789E-16, 11.54700538379251284, -171.1250000000000000 ) ) ;
#8300=CARTESIAN_POINT ( 'NONE',  ( -2.293366432827344421E-15, -12.48450537969573659, -177.2187500020484094 ) ) ;
#8305=CARTESIAN_POINT ( 'NONE',  ( 5.405949406249992428, -9.363379034771808662, -40.78125000204838102 ) ) ;
#8307=CARTESIAN_POINT ( 'NONE',  ( 10.00000000000000000, 5.773502691896255534, -99.37499999999998579 ) ) ;
#8309=CARTESIAN_POINT ( 'NONE',  ( -2.293366432827344421E-15, -12.48450537969573659, -124.9062500020483810 ) ) ;
#8310=CARTESIAN_POINT ( 'NONE',  ( -2.121150477449813534E-15, -11.54700538379251284, -145.2500000040967905 ) ) ;
#8311=LINE ( 'NONE', #23694, #26376 ) ;
#8314=CARTESIAN_POINT ( 'NONE',  ( -10.81189881249999729, 6.242252689847871849, -174.7187500020483810 ) ) ;
#8318=CARTESIAN_POINT ( 'NONE',  ( 10.81189881249999907, 6.242252689847868297, -67.40625000204839523 ) ) ;
#8321=CARTESIAN_POINT ( 'NONE',  ( 9.999999999999996447, -5.773502691896262640, -41.50000000409676204 ) ) ;
#8322=CARTESIAN_POINT ( 'NONE',  ( 5.405949406249999534, 9.363379034771803333, -5.593750002048370362 ) ) ;
#8327=VERTEX_POINT ( 'NONE', #24275 ) ;
#8335=ORIENTED_EDGE ( 'NONE', *, *, #16447, .T. ) ;
#8343=CARTESIAN_POINT ( 'NONE',  ( -4.999999999999996447, 8.660254037844387298, -38.99999999999997868 ) ) ;
#8347=CARTESIAN_POINT ( 'NONE',  ( 7.644554776091147741E-16, 12.48450537969573659, -165.9687500020483810 ) ) ;
#8348=CARTESIAN_POINT ( 'NONE',  ( 5.405949406249992428, -9.363379034771808662, -175.5937500020484094 ) ) ;
#8351=CARTESIAN_POINT ( 'NONE',  ( -5.000000000000003553, -8.660254037844383745, -197.5000000000000000 ) ) ;
#8356=CARTESIAN_POINT ( 'NONE',  ( -10.81189881249999729, 1.324075727343319199E-15, -60.59375000204836681 ) ) ;
#8357=CARTESIAN_POINT ( 'NONE',  ( 10.81189881249999551, -6.242252689847874514, -72.15625000204836681 ) ) ;
#8359=CARTESIAN_POINT ( 'NONE',  ( -10.00000000000000000, -5.773502691896251982, -125.6249999999999858 ) ) ;
#8360=CARTESIAN_POINT ( 'NONE',  ( -5.405949406250003975, -9.363379034771801557, -149.0312500020483810 ) ) ;
#8361=CARTESIAN_POINT ( 'NONE',  ( 10.81189881249999907, 6.242252689847868297, -161.9062500020484094 ) ) ;
#8363=ADVANCED_FACE ( 'NONE', ( #27497 ), #40631, .F. ) ;
#8366=CARTESIAN_POINT ( 'NONE',  ( -5.405949406250003975, -9.363379034771801557, -94.84375000204838102 ) ) ;
#8367=ORIENTED_EDGE ( 'NONE', *, *, #29665, .T. ) ;
#8369=CARTESIAN_POINT ( 'NONE',  ( -5.405949406249996869, 9.363379034771805109, -198.8437500020484094 ) ) ;
#8372=CARTESIAN_POINT ( 'NONE',  ( -5.405949406249996869, 9.363379034771805109, -95.53125000204838102 ) ) ;
#8374=CARTESIAN_POINT ( 'NONE',  ( 9.999999999999998224, 0.000000000000000000, -68.37500000409677625 ) ) ;
#8376=CARTESIAN_POINT ( 'NONE',  ( 7.644554776091147741E-16, 12.48450537969573659, -26.46875000204837391 ) ) ;
#8377=ORIENTED_EDGE ( 'NONE', *, *, #3654, .F. ) ;
#8379=CARTESIAN_POINT ( 'NONE',  ( 7.644554776091147741E-16, 12.48450537969573659, -17.65625000204837391 ) ) ;
#8381=CARTESIAN_POINT ( 'NONE',  ( -9.999999999999479527, -5.773502691896549521, -118.5000000040967763 ) ) ;
#8384=DIRECTION ( 'NONE',  ( -0.000000000000000000, -0.000000000000000000, -1.000000000000000000 ) ) ;
#8389=ORIENTED_EDGE ( 'NONE', *, *, #39645, .F. ) ;
#8401=CARTESIAN_POINT ( 'NONE',  ( -5.405949406250003975, -9.363379034771801557, -164.0312500020484094 ) ) ;
#8404=CARTESIAN_POINT ( 'NONE',  ( -10.81189881249999729, 1.324075727343319199E-15, -89.09375000204838102 ) ) ;
#8406=CARTESIAN_POINT ( 'NONE',  ( -2.293366432827344421E-15, -12.48450537969573659, -196.7187500020484094 ) ) ;
#8407=CARTESIAN_POINT ( 'NONE',  ( 10.81189881249999729, 0.000000000000000000, -94.53125000204838102 ) ) ;
#8411=CARTESIAN_POINT ( 'NONE',  ( 5.405949406249999534, 9.363379034771803333, -176.7812500020484094 ) ) ;
#8412=CARTESIAN_POINT ( 'NONE',  ( -10.81189881249999729, 1.324075727343319199E-15, -189.7812500020484094 ) ) ;
#8414=CARTESIAN_POINT ( 'NONE',  ( -10.00000000000000000, -5.773502691896251982, -166.5000000040967905 ) ) ;
#8416=CARTESIAN_POINT ( 'NONE',  ( -5.405949406249996869, 9.363379034771805109, -11.34375000204834727 ) ) ;
#8418=CARTESIAN_POINT ( 'NONE',  ( 10.81189881249999907, 6.242252689847868297, -121.2187500020483952 ) ) ;
#8420=CARTESIAN_POINT ( 'NONE',  ( -10.81189881249999729, 1.324075727343319199E-15, -18.78125000204835970 ) ) ;
#8423=CARTESIAN_POINT ( 'NONE',  ( -4.999999999999996447, 8.660254037844387298, -49.49999999999998579 ) ) ;
#8424=CARTESIAN_POINT ( 'NONE',  ( -5.405949406250003975, -9.363379034771801557, -119.0312500020483952 ) ) ;
#8427=CARTESIAN_POINT ( 'NONE',  ( 4.999999999999992006, -8.660254037844389075, -94.12500000409677625 ) ) ;
#8430=CARTESIAN_POINT ( 'NONE',  ( 10.81189881249999907, 6.242252689847868297, -46.21875000204837391 ) ) ;
#8436=CARTESIAN_POINT ( 'NONE',  ( -2.121150477449813534E-15, -11.54700538379251284, -28.25000000409675138 ) ) ;
#8438=VECTOR ( 'NONE', #41845, 1000.000000000000000 ) ;
#8439=CARTESIAN_POINT ( 'NONE',  ( 7.070501591499376803E-16, 11.54700538379251284, -168.1250000000000000 ) ) ;
#8448=FACE_OUTER_BOUND ( 'NONE', #4796, .T. ) ;
#8450=DIRECTION ( 'NONE',  ( -0.000000000000000000, -0.000000000000000000, -1.000000000000000000 ) ) ;
#8452=CARTESIAN_POINT ( 'NONE',  ( 10.81189881249999729, 0.000000000000000000, -189.0312500020484094 ) ) ;
#8456=CARTESIAN_POINT ( 'NONE',  ( 5.405949406249999534, 9.363379034771803333, -113.5937500020483810 ) ) ;
#8458=CARTESIAN_POINT ( 'NONE',  ( -10.81189881249999729, 6.242252689847871849, -116.4062500020483810 ) ) ;
#8460=CARTESIAN_POINT ( 'NONE',  ( 5.405949406249999534, 9.363379034771803333, -125.5937500020483668 ) ) ;
#8462=CARTESIAN_POINT ( 'NONE',  ( -4.999999999999996447, 8.660254037844387298, -178.8750000040967905 ) ) ;
#8463=CARTESIAN_POINT ( 'NONE',  ( 4.999999999999992006, -8.660254037844389075, -144.7500000000000000 ) ) ;
#8464=CARTESIAN_POINT ( 'NONE',  ( 9.999999999999998224, 0.000000000000000000, -15.49999999999995737 ) ) ;
#8465=AXIS2_PLACEMENT_3D ( 'NONE', #17676, #14218, #7563 ) ;
#8468=CARTESIAN_POINT ( 'NONE',  ( 9.999999999999998224, 0.000000000000000000, -189.8750000040967905 ) ) ;
#8470=CARTESIAN_POINT ( 'NONE',  ( 5.405949406249999534, 9.363379034771803333, -34.09375000204836681 ) ) ;
#8471=CARTESIAN_POINT ( 'NONE',  ( -5.405949406249996869, 9.363379034771805109, -146.3437500020483810 ) ) ;
#8473=CARTESIAN_POINT ( 'NONE',  ( 10.00000000000000000, 5.773502691896255534, -78.37499999999998579 ) ) ;
#8474=CARTESIAN_POINT ( 'NONE',  ( -5.405949406250003975, -9.363379034771801557, -141.5312500020483810 ) ) ;
#8476=ORIENTED_EDGE ( 'NONE', *, *, #27218, .T. ) ;
#8477=CARTESIAN_POINT ( 'NONE',  ( 4.999999999999992006, -8.660254037844389075, -164.2500000000000000 ) ) ;
#8478=CARTESIAN_POINT ( 'NONE',  ( -5.000000000000003553, -8.660254037844383745, -113.8750000040967763 ) ) ;
#8480=CARTESIAN_POINT ( 'NONE',  ( 5.405949406249992428, -9.363379034771808662, -78.09375000204838102 ) ) ;
#8483=CARTESIAN_POINT ( 'NONE',  ( -10.81189881249999907, -6.242252689847864744, -41.15625000204836681 ) ) ;
#8484=CARTESIAN_POINT ( 'NONE',  ( -9.999999999999227285, -5.773502691896698735, -137.6249999999999716 ) ) ;
#8499=CARTESIAN_POINT ( 'NONE',  ( -2.293366432827344421E-15, -12.48450537969573659, -130.7187500020483810 ) ) ;
#8500=CARTESIAN_POINT ( 'NONE',  ( 10.81189881249999551, -6.242252689847874514, -142.6562500020484094 ) ) ;
#8502=CARTESIAN_POINT ( 'NONE',  ( 10.81189881249999729, 6.242252689847867408, -155.7187500020483810 ) ) ;
#8503=CARTESIAN_POINT ( 'NONE',  ( 5.000000000000000000, 8.660254037844385522, -127.7499999999999716 ) ) ;
#8504=CARTESIAN_POINT ( 'NONE',  ( 9.999999999999996447, -5.773502691896262640, -170.1250000000000000 ) ) ;
#8508=CARTESIAN_POINT ( 'NONE',  ( -10.41934351496823830, 1.167130642714232946, -100.0000000000000142 ) ) ;
#8509=CARTESIAN_POINT ( 'NONE',  ( -10.81189881249999729, 1.324075727343319199E-15, -167.0937500020484094 ) ) ;
#8513=CARTESIAN_POINT ( 'NONE',  ( -10.81189881249999729, 1.324075727343319199E-15, -47.28125000204838813 ) ) ;
#8515=CARTESIAN_POINT ( 'NONE',  ( 10.00000000000000000, 5.773502691896255534, -96.37499999999998579 ) ) ;
#8517=CARTESIAN_POINT ( 'NONE',  ( 10.81189881249999551, -6.242252689847874514, -123.1562500020483952 ) ) ;
#8518=CARTESIAN_POINT ( 'NONE',  ( 10.00000000000000000, 5.773502691896255534, -147.7500000040967905 ) ) ;
#8521=EDGE_LOOP ( 'NONE', ( #12703, #31423, #32673, #30203, #40185 ) ) ;
#8522=CARTESIAN_POINT ( 'NONE',  ( 7.644554776091147741E-16, 12.48450537969573659, -170.4687500020483810 ) ) ;
#8524=CARTESIAN_POINT ( 'NONE',  ( -5.000000000000003553, -8.660254037844383745, -166.0000000000000000 ) ) ;
#8525=DIRECTION ( 'NONE',  ( 0.000000000000000000, 0.000000000000000000, 1.000000000000000000 ) ) ;
#8526=CARTESIAN_POINT ( 'NONE',  ( 5.405949406249992428, -9.363379034771808662, -66.28125000204838102 ) ) ;
#8527=CARTESIAN_POINT ( 'NONE',  ( 10.00000000000000000, 5.773502691896255534, -45.75000000409676204 ) ) ;
#8528=CARTESIAN_POINT ( 'NONE',  ( -2.293366432827344421E-15, -12.48450537969573659, -3.218750002048353931 ) ) ;
#8534=ORIENTED_EDGE ( 'NONE', *, *, #7404, .T. ) ;
#8535=CARTESIAN_POINT ( 'NONE',  ( 0.000000000000000000, 0.000000000000000000, -99.99999999999998579 ) ) ;
#8537=LINE ( 'NONE', #22542, #28664 ) ;
#8538=EDGE_CURVE ( 'NONE', #9539, #34380, #41501, .T. ) ;
#8541=EDGE_LOOP ( 'NONE', ( #35824, #22345, #25279, #36449 ) ) ;
#8552=CARTESIAN_POINT ( 'NONE',  ( 0.000000000000000000, 0.000000000000000000, -99.99999999999998579 ) ) ;
#8553=CARTESIAN_POINT ( 'NONE',  ( -4.999999999999996447, 8.660254037844387298, -37.49999999999997868 ) ) ;
#8557=CARTESIAN_POINT ( 'NONE',  ( 5.405949406249999534, 9.363379034771803333, -154.0937500020483810 ) ) ;
#8558=DIRECTION ( 'NONE',  ( -1.000000000000000000, 0.000000000000000000, 0.000000000000000000 ) ) ;
#8560=LINE ( 'NONE', #32080, #21927 ) ;
#8562=CARTESIAN_POINT ( 'NONE',  ( -9.999999999999998224, 1.224646799147353059E-15, -193.2500000000000000 ) ) ;
#8564=CARTESIAN_POINT ( 'NONE',  ( 9.999999999999998224, 1.224646799147353059E-15, -99.99999999999998579 ) ) ;
#8567=CARTESIAN_POINT ( 'NONE',  ( -10.81189881249999729, 6.242252689847871849, -66.90625000204839523 ) ) ;
#8569=CARTESIAN_POINT ( 'NONE',  ( 7.070501591499377789E-16, 11.54700538379251284, -126.1249999999999858 ) ) ;
#8570=CARTESIAN_POINT ( 'NONE',  ( 5.405949406249999534, 9.363379034771803333, -154.2812500020484094 ) ) ;
#8571=CARTESIAN_POINT ( 'NONE',  ( -2.293366432827344421E-15, -12.48450537969573659, -160.9062500020483810 ) ) ;
#8573=CARTESIAN_POINT ( 'NONE',  ( 0.000000000000000000, 0.000000000000000000, -169.9999999999999716 ) ) ;
#8574=CARTESIAN_POINT ( 'NONE',  ( -10.81189881249999907, -6.242252689847864744, -100.9687500020483810 ) ) ;
#8577=CARTESIAN_POINT ( 'NONE',  ( 7.644554776091147741E-16, 12.48450537969573659, -197.4687500020484094 ) ) ;
#8582=CARTESIAN_POINT ( 'NONE',  ( 10.81189881249999907, 6.242252689847868297, -95.90625000204839523 ) ) ;
#8584=CARTESIAN_POINT ( 'NONE',  ( 10.00000000000000000, 5.773502691896255534, -65.25000000409677625 ) ) ;
#8586=CARTESIAN_POINT ( 'NONE',  ( 10.81189881249999551, -6.242252689847874514, -26.96875000204837391 ) ) ;
#8587=CARTESIAN_POINT ( 'NONE',  ( -4.999999999999996447, 8.660254037844387298, -100.4999999999999858 ) ) ;
#8589=CARTESIAN_POINT ( 'NONE',  ( 5.405949406249992428, -9.363379034771808662, -19.78125000204836326 ) ) ;
#8591=CARTESIAN_POINT ( 'NONE',  ( 9.999999999999998224, 0.000000000000000000, -117.8750000040967905 ) ) ;
#8594=CARTESIAN_POINT ( 'NONE',  ( 9.999999999999612754, 5.773502691896477579, -152.2500000040967336 ) ) ;
#8600=ORIENTED_EDGE ( 'NONE', *, *, #14833, .F. ) ;
#8601=( BOUNDED_CURVE ( )  B_SPLINE_CURVE ( 2, ( #27138, #4048, #17192, #4263, #37270, #30810, #7932 ),
 .UNSPECIFIED., .F., .F. ) 
 B_SPLINE_CURVE_WITH_KNOTS ( ( 3, 2, 2, 3 ),
 ( 0.2164179104477612636, 0.2176616915422886489, 0.2189054726368160064, 0.2201492537313433639 ),
 .UNSPECIFIED. ) 
 CURVE ( )  GEOMETRIC_REPRESENTATION_ITEM ( )  RATIONAL_B_SPLINE_CURVE ( ( 0.9999999999999910072, 0.8660254037844477004, 1.000000000000000000, 0.8660254037844387076, 1.000000000000000000, 0.8660254037844297148, 1.000000000000008882 ) ) 
 REPRESENTATION_ITEM ( '' )  );
#8608=CARTESIAN_POINT ( 'NONE',  ( 8.660254119780192994, -4.999999858083012505, -99.99999999999998579 ) ) ;
#8609=CARTESIAN_POINT ( 'NONE',  ( 9.999999999999227285, 5.773502691896701400, -105.7500000040967620 ) ) ;
#8610=CARTESIAN_POINT ( 'NONE',  ( 10.81189881249999729, 0.000000000000000000, -166.5312500020484094 ) ) ;
#8613=CARTESIAN_POINT ( 'NONE',  ( 10.81189881249999551, -6.242252689847874514, -86.96875000204838102 ) ) ;
#8615=CARTESIAN_POINT ( 'NONE',  ( -10.81189881249999729, 6.242252689847871849, -195.7187500020484379 ) ) ;
#8616=CARTESIAN_POINT ( 'NONE',  ( 10.81189881249999729, 0.000000000000000000, -96.03125000204838102 ) ) ;
#8620=CARTESIAN_POINT ( 'NONE',  ( -10.81189881249999729, 1.324075727343319199E-15, -174.7812500020484094 ) ) ;
#8621=CARTESIAN_POINT ( 'NONE',  ( -10.81189881249999907, -6.242252689847864744, -185.1562500020484094 ) ) ;
#8623=CARTESIAN_POINT ( 'NONE',  ( -9.999999999999998224, 5.773502691896259087, -166.7500000040967905 ) ) ;
#8625=CARTESIAN_POINT ( 'NONE',  ( 10.81189881249999551, -6.242252689847874514, -13.46875000204836503 ) ) ;
#8627=CARTESIAN_POINT ( 'NONE',  ( 10.81189881249999551, -6.242252689847874514, -124.4687500020483952 ) ) ;
#8629=CARTESIAN_POINT ( 'NONE',  ( 5.405949406249999534, 9.363379034771803333, -17.78125000204835970 ) ) ;
#8631=FACE_OUTER_BOUND ( 'NONE', #20079, .T. ) ;
#8632=CARTESIAN_POINT ( 'NONE',  ( 10.00000000000000000, 5.773502691896255534, -51.37499999999997868 ) ) ;
#8633=CARTESIAN_POINT ( 'NONE',  ( -10.81189881249999907, -6.242252689847864744, -116.1562500020483952 ) ) ;
#8637=CARTESIAN_POINT ( 'NONE',  ( -10.00000000000000000, -5.773502691896251982, -94.50000000409677625 ) ) ;
#8640=CARTESIAN_POINT ( 'NONE',  ( 5.405949406249992428, -9.363379034771808662, -49.59375000204838102 ) ) ;
#8641=ORIENTED_EDGE ( 'NONE', *, *, #56, .F. ) ;
#8645=CARTESIAN_POINT ( 'NONE',  ( -5.000000000000003553, -8.660254037844383745, -20.87500000409675494 ) ) ;
#8650=DIRECTION ( 'NONE',  ( -0.000000000000000000, -0.000000000000000000, -1.000000000000000000 ) ) ;
#8652=ORIENTED_EDGE ( 'NONE', *, *, #25059, .T. ) ;
#8653=( BOUNDED_CURVE ( )  B_SPLINE_CURVE ( 2, ( #7160, #10594, #20106, #35886, #19468, #32653, #42550 ),
 .UNSPECIFIED., .F., .F. ) 
 B_SPLINE_CURVE_WITH_KNOTS ( ( 3, 2, 2, 3 ),
 ( 0.3992537313432836799, 0.4004975124378110651, 0.4017412935323383949, 0.4029850746268657802 ),
 .UNSPECIFIED. ) 
 CURVE ( )  GEOMETRIC_REPRESENTATION_ITEM ( )  RATIONAL_B_SPLINE_CURVE ( ( 0.9999999999999880096, 0.8660254037844506980, 1.000000000000000000, 0.8660254037844387076, 1.000000000000000000, 0.8660254037844267172, 1.000000000000011990 ) ) 
 REPRESENTATION_ITEM ( '' )  );
#8660=DIRECTION ( 'NONE',  ( -0.000000000000000000, -0.000000000000000000, -1.000000000000000000 ) ) ;
#8662=CARTESIAN_POINT ( 'NONE',  ( -10.81189881249999907, -6.242252689847864744, -188.1562500020484094 ) ) ;
#8665=CARTESIAN_POINT ( 'NONE',  ( -10.81189881249999907, -6.242252689847864744, -108.4687500020483810 ) ) ;
#8667=CARTESIAN_POINT ( 'NONE',  ( 5.405949406249999534, 9.363379034771803333, -119.7812500020483952 ) ) ;
#8669=CARTESIAN_POINT ( 'NONE',  ( -5.405949406249996869, 9.363379034771805109, -125.3437500020483952 ) ) ;
#8672=CARTESIAN_POINT ( 'NONE',  ( -4.999999999999996447, 8.660254037844387298, -157.5000000000000000 ) ) ;
#8673=CARTESIAN_POINT ( 'NONE',  ( 7.070501591499377789E-16, 11.54700538379251284, -145.6250000000000284 ) ) ;
#8674=CARTESIAN_POINT ( 'NONE',  ( -9.999999999999998224, 5.773502691896259087, -8.874999999999966249 ) ) ;
#8677=CARTESIAN_POINT ( 'NONE',  ( -4.999999999999996447, 8.660254037844387298, -184.8750000040967905 ) ) ;
#8679=CARTESIAN_POINT ( 'NONE',  ( 10.81189881249999551, -6.242252689847874514, -40.46875000204835970 ) ) ;
#8680=CARTESIAN_POINT ( 'NONE',  ( 10.00000000000025402, -5.773502691896113426, -163.0000000040967905 ) ) ;
#8681=CARTESIAN_POINT ( 'NONE',  ( -10.81189881249999907, -6.242252689847864744, -142.9687500020484094 ) ) ;
#8685=CARTESIAN_POINT ( 'NONE',  ( 9.999999999999996447, -5.773502691896262640, -72.62499999999995737 ) ) ;
#8686=CARTESIAN_POINT ( 'NONE',  ( 10.81189881249999551, -6.242252689847874514, -138.1562500020484094 ) ) ;
#8688=ORIENTED_EDGE ( 'NONE', *, *, #8000, .F. ) ;
#8690=CARTESIAN_POINT ( 'NONE',  ( 7.070501591499377789E-16, 11.54700538379251284, -113.0000000040967905 ) ) ;
#8692=CARTESIAN_POINT ( 'NONE',  ( 10.81189881249999729, 0.000000000000000000, -76.34375000204838102 ) ) ;
#8697=CARTESIAN_POINT ( 'NONE',  ( 7.644554776091147741E-16, 12.48450537969573659, -41.65625000204837391 ) ) ;
#8702=CARTESIAN_POINT ( 'NONE',  ( 10.00000000000051159, -5.773502691895965988, -120.6250000000000000 ) ) ;
#8714=CARTESIAN_POINT ( 'NONE',  ( -2.293366432827344421E-15, -12.48450537969573659, -135.2187500020483810 ) ) ;
#8715=CARTESIAN_POINT ( 'NONE',  ( -5.405949406249996869, 9.363379034771805109, -142.0312500020483810 ) ) ;
#8716=CARTESIAN_POINT ( 'NONE',  ( -5.405949406249996869, 9.363379034771805109, -149.3437500020483810 ) ) ;
#8719=CARTESIAN_POINT ( 'NONE',  ( 10.00000000000000000, 5.773502691896255534, -174.3750000000000000 ) ) ;
#8723=CARTESIAN_POINT ( 'NONE',  ( -9.999999999999998224, 1.224646799147353059E-15, -133.2499999999999716 ) ) ;
#8725=CARTESIAN_POINT ( 'NONE',  ( -10.81189881249999729, 6.242252689847871849, -167.2187500020483810 ) ) ;
#8729=CARTESIAN_POINT ( 'NONE',  ( 7.644554776091147741E-16, 12.48450537969573659, -47.65625000204837391 ) ) ;
#8731=CARTESIAN_POINT ( 'NONE',  ( 9.999999999999996447, -5.773502691896262640, -99.62500000000000000 ) ) ;
#8733=CARTESIAN_POINT ( 'NONE',  ( -10.81189881249999729, -6.242252689847864744, -128.1562500020483810 ) ) ;
#8734=CARTESIAN_POINT ( 'NONE',  ( -10.00000000000000000, -5.773502691896251982, -142.5000000040967905 ) ) ;
#8738=CARTESIAN_POINT ( 'NONE',  ( -5.405949406249996869, 9.363379034771805109, -173.3437500020484094 ) ) ;
#8741=CARTESIAN_POINT ( 'NONE',  ( 10.81189881249999729, 0.000000000000000000, -72.03125000204838102 ) ) ;
#8742=CARTESIAN_POINT ( 'NONE',  ( -9.999999999999998224, 5.773502691896259087, -42.25000000409676204 ) ) ;
#8743=DIRECTION ( 'NONE',  ( -0.000000000000000000, -0.000000000000000000, -1.000000000000000000 ) ) ;
#8751=ORIENTED_EDGE ( 'NONE', *, *, #30651, .F. ) ;
#8761=CARTESIAN_POINT ( 'NONE',  ( 10.00000000000000000, 5.773502691896255534, -36.37499999999996447 ) ) ;
#8764=CARTESIAN_POINT ( 'NONE',  ( -2.293366432827344421E-15, -12.48450537969573659, -159.2187500020483810 ) ) ;
#8765=CARTESIAN_POINT ( 'NONE',  ( 5.405949406249992428, -9.363379034771808662, -171.0937500020484094 ) ) ;
#8766=FACE_OUTER_BOUND ( 'NONE', #7099, .T. ) ;
#8767=CARTESIAN_POINT ( 'NONE',  ( 9.999999999999998224, 0.000000000000000000, -132.5000000000000000 ) ) ;
#8768=CARTESIAN_POINT ( 'NONE',  ( 10.00000000000000000, 5.773502691896255534, -195.3750000000000284 ) ) ;
#8775=CARTESIAN_POINT ( 'NONE',  ( -5.405949406249996869, 9.363379034771805109, -71.53125000204838102 ) ) ;
#8777=CARTESIAN_POINT ( 'NONE',  ( 5.000000000000000000, 8.660254037844385522, -123.2500000000000000 ) ) ;
#8778=CARTESIAN_POINT ( 'NONE',  ( 10.81189881249999729, 0.000000000000000000, -151.5312500020484094 ) ) ;
#8779=CARTESIAN_POINT ( 'NONE',  ( 7.644554776091147741E-16, 12.48450537969573659, -166.1562500020483810 ) ) ;
#8782=CARTESIAN_POINT ( 'NONE',  ( 5.405949406249992428, -9.363379034771808662, -96.09375000204838102 ) ) ;
#8783=EDGE_LOOP ( 'NONE', ( #25068, #30998, #1304, #11437 ) ) ;
#8785=CARTESIAN_POINT ( 'NONE',  ( 7.644554776091147741E-16, 12.48450537969573659, -195.9687500020484094 ) ) ;
#8788=CARTESIAN_POINT ( 'NONE',  ( 5.405949406249999534, 9.363379034771803333, -89.78125000204838102 ) ) ;
#8790=CARTESIAN_POINT ( 'NONE',  ( 9.999999999999996447, -5.773502691896262640, -68.50000000409677625 ) ) ;
#8791=DIRECTION ( 'NONE',  ( -0.000000000000000000, -0.000000000000000000, -1.000000000000000000 ) ) ;
#8792=CARTESIAN_POINT ( 'NONE',  ( -5.405949406250003975, -9.363379034771801557, -27.34375000204835970 ) ) ;
#8795=CARTESIAN_POINT ( 'NONE',  ( -2.293366432827344421E-15, -12.48450537969573659, -16.90625000204837391 ) ) ;
#8805=CARTESIAN_POINT ( 'NONE',  ( 7.070501591499376803E-16, 11.54700538379251284, -170.0000000040967905 ) ) ;
#8813=CIRCLE ( 'NONE', #35678, 35.00000000000000711 ) ;
#8816=CARTESIAN_POINT ( 'NONE',  ( -5.000000000000003553, -8.660254037844383745, -127.3750000040967905 ) ) ;
#8817=CARTESIAN_POINT ( 'NONE',  ( 7.644554776091147741E-16, 12.48450537969573659, -164.6562500020484094 ) ) ;
#8821=EDGE_CURVE ( 'NONE', #15268, #12639, #21051, .T. ) ;
#8823=CARTESIAN_POINT ( 'NONE',  ( -2.293366432827344421E-15, -12.48450537969573659, -85.71875000204838102 ) ) ;
#8824=CARTESIAN_POINT ( 'NONE',  ( -2.293366432827344421E-15, -12.48450537969573659, -193.7187500020484094 ) ) ;
#8825=CARTESIAN_POINT ( 'NONE',  ( 7.644554776091147741E-16, 12.48450537969573659, -89.65625000204839523 ) ) ;
#8830=CARTESIAN_POINT ( 'NONE',  ( -10.81189881249999729, 1.324075727343319199E-15, -171.7812500020484094 ) ) ;
#8831=CARTESIAN_POINT ( 'NONE',  ( -5.405949406250003975, -9.363379034771801557, -191.0312500020484094 ) ) ;
#8834=CARTESIAN_POINT ( 'NONE',  ( -10.00000000000000000, -5.773502691896251982, -168.0000000040967905 ) ) ;
#8836=CARTESIAN_POINT ( 'NONE',  ( -10.81189881249999729, 1.324075727343319199E-15, -11.09375000204834727 ) ) ;
#8837=CARTESIAN_POINT ( 'NONE',  ( 0.000000000000000000, 0.000000000000000000, -99.99999999999998579 ) ) ;
#8838=CARTESIAN_POINT ( 'NONE',  ( 5.405949406249992428, -9.363379034771808662, -124.5937500020483952 ) ) ;
#8840=CARTESIAN_POINT ( 'NONE',  ( 7.644554776091147741E-16, 12.48450537969573659, -23.65625000204838102 ) ) ;
#8843=CARTESIAN_POINT ( 'NONE',  ( 10.81189881249999729, 0.000000000000000000, -120.0312500020483952 ) ) ;
#8846=CARTESIAN_POINT ( 'NONE',  ( 7.070501591499377789E-16, 11.54700538379251284, -95.00000000409677625 ) ) ;
#8849=CARTESIAN_POINT ( 'NONE',  ( -5.405949406250003975, -9.363379034771801557, -48.34375000204838102 ) ) ;
#8854=VECTOR ( 'NONE', #7008, 1000.000000000000000 ) ;
#8856=CARTESIAN_POINT ( 'NONE',  ( -9.999999999999998224, 1.224646799147353059E-15, -16.62500000409675138 ) ) ;
#8857=EDGE_CURVE ( 'NONE', #30728, #33393, #2044, .T. ) ;
#8867=ORIENTED_EDGE ( 'NONE', *, *, #30852, .F. ) ;
#8871=CARTESIAN_POINT ( 'NONE',  ( 10.81189881249999551, -6.242252689847874514, -192.1562500020484094 ) ) ;
#8876=CARTESIAN_POINT ( 'NONE',  ( 10.81189881249999907, 6.242252689847868297, -109.2187500020483810 ) ) ;
#8877=CARTESIAN_POINT ( 'NONE',  ( 5.405949406249992428, -9.363379034771808662, -118.7812500020483952 ) ) ;
#8879=CARTESIAN_POINT ( 'NONE',  ( -2.293366432827344421E-15, -12.48450537969573659, -123.2187500020483952 ) ) ;
#8882=CARTESIAN_POINT ( 'NONE',  ( -9.999999999999998224, 5.773502691896259087, -146.8750000000000000 ) ) ;
#8883=CARTESIAN_POINT ( 'NONE',  ( 10.00000000000000000, 5.773502691896255534, -15.37499999999997335 ) ) ;
#8886=CARTESIAN_POINT ( 'NONE',  ( 9.999999999999998224, 0.000000000000000000, -186.8750000040967905 ) ) ;
#8888=CARTESIAN_POINT ( 'NONE',  ( -10.81189881249999907, -6.242252689847864744, -36.46875000204835260 ) ) ;
#8889=CARTESIAN_POINT ( 'NONE',  ( 0.000000000000000000, 0.000000000000000000, -169.9999999999999716 ) ) ;
#8890=CARTESIAN_POINT ( 'NONE',  ( -5.405949406249996869, 9.363379034771805109, -147.8437500020483810 ) ) ;
#8892=CARTESIAN_POINT ( 'NONE',  ( -9.999999999999998224, 1.224646799147353059E-15, -77.74999999999998579 ) ) ;
#8893=CARTESIAN_POINT ( 'NONE',  ( -10.81189881249999907, -6.242252689847864744, -138.6562500020484094 ) ) ;
#8896=( BOUNDED_SURFACE ( )  B_SPLINE_SURFACE ( 1, 2, ( 
 ( #20904, #10547, #40114, #33879, #27607, #40747, #23732, #36883, #7329, #33665, #14635, #31714, #21118, #42400, #5374, #1931, #28478, #4722, #31501, #25028, #40957, #8406, #31288, #34523, #38171, #17871, #12043, #8187, #2935, #8615, #2145, #11400, #29256, #16064, #34307, #31067, #15280, #41609, #18311, #24594, #37743, #7969, #25239, #21334, #38383, #8824, #21771, #27823, #34949, #1501, #24387, #5159, #41393, #21981, #4946, #18093, #1717, #14846, #37961, #35159, #18525, #5585, #28042, #41169, #11608, #15058, #24816, #18738, #31930, #37528, #21557, #34737, #28256, #11828, #13038, #16486, #22995, #3567, #13457, #3143, #26232, #39174, #19740, #10233, #10023, #3776, #6584, #22781, #17126, #550, #12831, #26437, #9608, #23203, #39588, #19951, #20372, #26651, #39801, #13250, #16701, #33357, #6795, #36362, #26022, #29897, #23420, #33139, #9815, #7220, #36569, #33561, #3353, #3985, #36784, #7015, #19526, #32920, #30329, #36151, #40016, #128, #35942, #336, #29685, #20167, #32710, #6384, #16911, #30113, #13669, #16270, #26862, #29469, #10446, #23638, #42611, #39380, #970, #11508, #14525, #37426, #14087, #1395, #1182, #21017, #40424, #14303, #31182, #27288, #20584, #27934, #14741, #36997, #40638, #10868, #7869, #40855, #24059, #5055, #27719, #37202, #34207, #27503, #11295, #30963, #41063, #37642, #34418, #10655, #7649, #24710, #20800, #24489, #37856, #33988, #4195, #8300, #18203, #11079, #1612, #8081, #21232, #21445, #4836, #34629, #17982, #759, #13882, #33773, #27078, #4409, #4623, #40221, #17548, #23847, #7432, #17339, #30542, #30749, #24281, #17769, #9144, #18635, #15807, #25767, #2673, #5485, #34844, #38491, #41713, #9351, #18857, #35273, #5706, #24924, #21663, #38710, #28153, #6122, #12361, #8935, #35485, #11726, #22099, #32037, #5267, #15386, #38278, #41508, #2466, #38068, #19065, #15172, #22520, #15596, #22312, #18419, #35693, #31393, #32246, #28798, #35057, #5912, #1827, #38920, #28584, #29002, #42143, #12574, #2265, #31829, #14955, #28369, #25132, #41930, #41287, #8725, #8509, #21879, #31609, #11940, #25558, #2041, #12152, #25345, #39755, #13412, #39545, #510, #12783, #6539, #9976, #30068, #3515, #19692, #26184, #6965, #42563, #16223, #29423, #6749, #26394, #16865, #3307, #26605, #3095, #13625, #29212, #39331, #29634, #20122, #33087, #19903, #33310, #10190, #3735, #16652, #23375, #29853, #39126, #2886, #32666, #13201, #32460, #19480, #26818, #16016, #39970, #6337, #35900, #9560, #16435, #36525, #32876, #10400, #23590, #36737, #36105, #22734, #23155, #77, #19267, #291, #36318, #42351, #25975, #12987, #9771, #22951, #24667, #30915, #27461, #11253, #30281, #14258, #7827, #23796, #33947, #14042, #17295, #20974, #720, #37596, #33729, #27889, #34159, #14480, #36951, #11466, #41022, #8040, #4579, #10823, #40813, #7175, #14700, #4369, #21184, #34374, #4790, #20758, #7604, #20327, #4152, #926, #17720, #17938, #27238, #33521, #40381, #3944, #30500, #1350, #31137, #24016, #27675, #24450, #1570, #40596, #17082, #13839, #37157, #11039, #27033, #40177, #17508, #30703, #10609, #1135, #24233, #37384, #7393, #20540, #35435, #21835, #2419, #21623, #5863, #5017, #15125, #15343, #38236, #35226, #25303, #22266, #31993, #28753, #18158, #18378, #19017, #38028, #8890, #9098, #31567, #41240, #32202, #12529, #2629, #15551, #41880, #31353, #1999, #15761, #8471, #22053, #28959, #28320, #11678, #42095, #37810, #5444, #25514, #5657, #38447, #8255, #12316, #38662, #18805, #21401, #34587, #14913, #1783, #34802, #31782, #28113, #5222, #24878, #41461, #11896, #25091, #8681, #35015, #18595, #2212, #28541, #41673, #12108, #39706, #42512, #29166, #32827, #36060, #3687, #13152, #29586, #29, #19224, #15970, #33038, #22470, #460, #6702, #3258, #29805, #6077, #16385, #26346, #42306, #9721, #32623, #35854, #39499, #32414, #13367, #9516, #16815, #9930, #3467, #12728, #30014, #25722, #26559, #23109, #29371, #16602, #38871, #33261, #22904, #10143, #23323, #36478, #39287, #26135, #9300, #22686, #19432, #36271, #6912, #3048, #35647, #16176, #2836, #6288, #19854, #20066, #12939, #245, #25925, #39077, #6494, #19643, #7128, #876, #4315, #24400, #40542, #13992, #20492, #1296, #36899, #10560, #23746, #1081, #20705, #11202, #40333, #20918, #40130, #37541, #23538, #33677, #33893, #27189, #10986, #14207, #21131, #7981, #24181, #20282, #4104, #31081, #7343, #40760, #10775, #39920, #17454, #17245, #27406, #33471, #34320, #37108, #30445, #23964, #4737, #7552, #17032, #30650, #37328, #17883, #7775, #13789, #13576, #34100, #4522, #26972, #17666, #30860, #14427, #27620, #26767, #10350, #36688, #3897, #30231, #671, #37754, #41406, #41181, #38183, #41621, #28055, #5810, #2157, #11620, #11412, #8199, #35172, #8838, #8627, #18105, #31300, #27837, #31941, #14858, #21994, #18750, #12055, #34534, #25251, #21348, #22210, #25041, #18537, #5597, #24606, #24828, #4958, #1732, #15068, #41828, #15292, #2369, #37974, #34750, #8418, #21783, #21569, #28489, #15495, #28701, #28269, #5170, #18324, #31513, #1943, #11840, #34963, #5386, #38396, #31728, #12265, #40969, #25461, #38606, #9045, #35385, #18963, #1514, #14648, #19800, #32150, #2998, #15709, #29320, #16123, #39237, #39653, #32772, #3208, #32572, #36010, #9884, #26086, #42463, #2580, #6447, #16334, #9675, #29117, #26506, #42675, #10090, #22633, #32987, #29533, #35806, #23058, #6862, #23268, #12892, #3416, #16553, #29751, #22848, #19589, #36427, #15916, #25874, #13101, #196, #39029, #28908, #9464, #42045, #42253, #26300, #13317, #6238, #39449, #36214, #6650, #12471, #25666, #38820, #19382, #9248, #22418, #35596, #6024, #19174, #32363, #12678, #2787, #16980, #7497, #27137, #17614, #4047, #27353, #3845, #30809, #29965, #40079, #40280, #20440, #17403, #20650, #4472, #14153, #10934, #405, #616, #1248, #20230, #33837, #34050, #13732, #23485, #14372, #37487, #30390, #7718, #4262, #30601, #27569, #40488, #20866, #1030, #24127, #37269, #39865, #3638, #33419, #13944, #33207, #30178, #40704, #16765, #11147, #7080, #36634, #10299, #17191, #24346, #7288, #20014, #13526, #26713, #36845, #26921, #10721, #823, #10510, #23697, #23914, #37058, #33625, #40918, #15237, #4685, #25403, #31672, #28217, #12004, #31029, #15018, #8574, #24555, #34697, #14803, #18052, #21724, #1460, #38340, #34483, #28646, #34907, #28435, #37705, #12210, #41776, #41350, #4905, #5329, #21939, #41571, #21516, #14593, #27783, #11360, #8147, #11569, #31247, #11787, #18484, #21295, #1675, #34269, #27999, #2106, #5117, #25199, #41129, #17833, #7931, #8782, #21081, #18266, #24775, #31455, #1889, #24989, #15448, #35119, #5543, #8366, #38131, #18695, #31891, #2319, #37920, #12842, #39186, #16074, #35543, #32931, #6395, #3364, #29063, #16497, #19750, #35954, #2529, #15862, #13262, #19124, #23007, #25821, #22158, #29267, #2731, #9620, #15654, #29695, #19322, #42201, #5973, #141, #38976, #41990, #12627, #22792, #36161, #9412, #38771, #6594, #19536, #32517, #9197, #32720, #22576, #42411, #32309, #35755, #26244, #22366, #28854, #38549, #9825, #32096, #6183, #2946, #26033, #3153, #16282, #8990, #29479, #42620, #5760, #12419, #13050, #39393, #35333, #25613, #18913, #10034, #14709, #39812, #33784, #981, #23860, #16714, #37008, #3580, #5027, #7232, #769, #4207, #36373, #23432, #19964, #13470, #40027, #24676, #40231, #27899, #10244, #16923, #26662, #27088, #36580, #6809, #33150, #17350, #30554, #20382, #348, #7027, #23216, #41032, #20179, #11475, #37822, #7443, #29909, #20597, #33369, #18168, #33573, #13895, #8264, #3789, #30124, #560, #13681, #10457, #21410, #10666, #34596, #26872, #23648, #36794, #3995, #17139, #31362, #1793, #26448, #30340, #39600, #8480, #21634, #15136, #18604, #25101, #5666, #15563, #5235, #28333, #41250, #21845, #12326, #12121, #5874, #8692, #24888, #19235, #2640, #14923, #28551, #11692, #25313, #41683, #22064, #22481, #28764, #41892, #15353, #18819, #35448, #8899, #38458, #28122, #32003, #25524, #35236, #11906, #9313, #38673, #35657, #5454, #6088, #38882, #9108, #34812, #35024, #32423, #38247, #42105, #2226, #38037, #2428, #31792, #22276, #18387, #31577, #19028, #32212, #15771, #2009, #28968, #41471, #12540, #25732, #472, #16398, #3060, #13587, #16613, #39511, #16185, #3478, #3268, #23119, #42525, #29598, #33272, #29382, #22696, #30026, #16827, #39087, #41, #12950, #9940, #257, #26145, #7139, #39296, #12738, #9526, #36488, #10155, #36284, #19441, #32633, #29177, #3698, #9733, #23336, #20078, #13378, #35865, #26570, #6298, #23551, #26358, #19866, #6925, #25938, #22914, #36069, #6505, #13164, #26780, #29816, #39932, #19655, #32840, #6714, #33052, #39719, #10359, #36699, #20292, #2847, #15980, #42316, #26984, #33690, #37120, #886, #24194, #34114, #23757, #4116, #17043, #40344, #30873, #30665, #24413, #27200, #683, #37768, #21145, #33483, #4328, #30243, #1093, #17466, #40556, #40982, #4536, #17678, #33906, #37342, #11213, #27420, #14220, #3909, #7788, #1308, #11000, #30459, #27849, #14441, #11425, #23976, #24620, #14660, #27633, #40143, #10787, #8213, #14005, #17895, #20716, #13800, #20932, #7564, #40772, #10571, #36910, #37554, #7992, #34331, #7356, #4749, #20503, #31094, #1527, #17256, #34975, #21583, #32161, #35182, #15305, #34761, #22007, #21795, #41632, #18337, #5399, #9055, #5183, #41193, #5821, #35397, #14870, #18551, #31526, #28502, #18763, #1955, #25678, #5608, #28281, #12483, #15081, #31952, #2591, #41418, #2381, #41839, #15508, #12068, #15720, #28067, #8640, #25262, #28918, #28713, #31741, #11854, #22222, #25053, #38196, #2170, #8849, #38407, #18976, #12277, #25473, #38618, #42055, #31312, #38830, #21362, #34545, #4971, #18117, #1744, #11634, #24839, #37986, #8430, #6873, #9476, #23069, #23278, #32584, #12688, #33217, #26723, #19601, #39665, #36225, #9894, #36437, #29761, #10101, #6660, #207, #19810, #29128, #35607, #22644, #3219, #22428, #35816, #3648, #6034, #20025, #39039, #25885, #42263, #36021, #13327, #39247, #16775, #29975, #418, #26097, #6249, #16344, #32782, #13538, #39460, #13111, #26310, #2797, #19392, #16564, #19184, #9260, #32998, #29543, #26517, #32373, #42686, #3426, #3009, #6459, #16133, #29331, #15927, #42473, #12901, #9684, #22858, #40499, #4483, #26931, #1471, #17843, #40716, #24139, #832, #30820, #14605, #4694, #37068, #11157, #24356, #37498, #10732, #40290, #39876, #23705, #33636, #37280, #7940, #4058, #10309, #21091, #7727, #3856, #17200, #23497, #20449, #34279, #27147, #36645, #30611, #30401, #10944, #16991, #31039, #20660, #13954, #36856, #7090, #23924, #625, #7510, #20875, #20240, #33848, #40089, #33429, #34061, #4272, #10520, #17625, #17413, #1039, #7299, #14164, #27579, #27363, #30189, #13741, #1258, #14382, #25001, #24786, #21739, #25210, #11578, #32108, #28447, #37930, #37715, #34493, #18707, #35131, #34918, #1685, #14814, #11369, #15459, #41139, #5554, #2330, #38353, #18063, #8792, #4915, #5771, #8586, #2117, #31901, #8157, #8376, #21305, #28011, #41361, #25415, #41582, #28658, #21526, #18276, #34708, #5340, #5129, #12014, #41788, #12223, #11798, #31259, #31466, #1899, #15028, #28228, #38143, #18495, #21950, #31683, #15247, #24566, #38560, #9001, #22169, #35343, #18924, #2540, #27795, #40926, #15666, #29278, #42001, #12852, #42422, #22802, #23226, #16293, #29491, #16083, #19546, #36171, #9631, #26044, #28867, #32730, #42630, #35967, #12638, #10046, #26254, #36386, #6193, #6819, #13060, #19337, #6606, #33160, #19974, #39196, #16508, #29706, #13272, #6405, #3166, #12429, #42211, #9422, #39403, #151, #22588, #25625, #35765, #38782, #25831, #9839, #26461, #32527, #23017, #19760, #32943, #3373, #39610, #9208, #2956, #22378, #35555, #5983, #19134, #32319, #2745, #38986, #15871, #29073, #33794, #10677, #1205, #30350, #10891, #30134, #14329, #13483, #23657, #23870, #4006, #991, #4219, #30771, #40447, #37223, #26672, #26882, #27526, #3799, #17361, #17570, #40037, #7037, #40660, #21038, #13905, #34010, #30562, #14109, #11100, #24084, #4431, #27312, #7671, #20823, #23442, #29919, #16937, #40240, #16724, #572, #24303, #361, #37447, #33379, #20190, #36590, #780, #7891, #33585, #3592, #39823, #10256, #20393, #13690, #37018, #27098, #10467, #36805, #7458, #20608, #7243, #17149, #28173, #17792, #15192, #1849, #8322, #11745, #1417, #37878, #5077, #11317, #41085, #4860, #21253, #18223, #30989, #38088, #37663, #31630, #31413, #41307, #24510, #34228, #2063, #8528, #14549, #8102, #21467, #4644, #18002, #27740, #34441, #40877, #34649, #14975, #11528, #21683, #31204, #24945, #1632, #14761, #27956, #34865, #5287, #24731, #18439, #8026, #17495, #33931, #4354, #23576, #20314, #37369, #26805, #4776, #11024 ),
 ( #40583, #7812, #24218, #7590, #11239, #36723, #17279, #20743, #40798, #14244, #30484, #36936, #17706, #10596, #27017, #40164, #30688, #37142, #27657, #14028, #20960, #13824, #24438, #39956, #7379, #1120, #913, #27447, #34146, #14467, #4564, #30901, #10387, #23782, #37581, #30266, #1336, #21170, #20525, #33507, #34360, #30052, #40368, #498, #13613, #7162, #3931, #17069, #705, #33713, #4138, #27224, #10809, #24002, #5218, #32198, #38658, #19013, #2415, #9095, #31989, #38024, #1779, #31563, #12104, #31349, #18374, #42092, #14909, #28955, #1996, #34798, #8468, #2208, #22262, #5440, #2625, #12525, #15757, #35010, #21619, #25299, #28537, #38867, #5653, #22049, #35222, #11674, #15121, #25510, #28108, #35643, #41875, #38442, #35431, #41236, #8886, #18801, #28316, #15340, #25087, #41457, #15547, #24874, #5859, #11892, #9296, #28749, #25718, #38232, #22466, #18154, #8677, #12312, #21831, #18592, #31778, #41669, #3254, #6908, #20062, #3683, #19639, #6491, #10346, #32619, #42508, #3463, #33257, #12934, #23534, #26131, #39916, #3044, #16598, #16811, #39284, #29801, #26555, #241, #26343, #30010, #42302, #36056, #39495, #456, #33034, #32823, #9717, #36474, #29367, #16172, #22900, #36267, #13148, #13572, #16380, #13363, #29582, #26763, #15966, #25, #9926, #23105, #39703, #6698, #6072, #10139, #23319, #29162, #19849, #19220, #6284, #32410, #2832, #12724, #9511, #25921, #39073, #22682, #35850, #19429, #1077, #4311, #14644, #24177, #40538, #10982, #30227, #26968, #1293, #33467, #11408, #17662, #14203, #40756, #17028, #27402, #37324, #10556, #20701, #872, #4100, #7771, #667, #24396, #20488, #27833, #20914, #14423, #23742, #40965, #36684, #37537, #34097, #40329, #27616, #7124, #1510, #33889, #7977, #21127, #34316, #7548, #37104, #20279, #33674, #30441, #4518, #4733, #13988, #3893, #27185, #13785, #17241, #30856, #17880, #10771, #11198, #31077, #40126, #36895, #7339, #23960, #17450, #30646, #35381, #8834, #25037, #31509, #12261, #5167, #21565, #34746, #12051, #31724, #22206, #8623, #31938, #8414, #5806, #34530, #1939, #2153, #38179, #21990, #25247, #9041, #18746, #15492, #4954, #18320, #18959, #24824, #38392, #38602, #15065, #28051, #32146, #42041, #8195, #2365, #5593, #11616, #2576, #28697, #25457, #35168, #41824, #15705, #1728, #21344, #37970, #18533, #37751, #28265, #28904, #18101, #24602, #41402, #41177, #14854, #21779, #31296, #11836, #34959, #5382, #15288, #28485, #41617, #29113, #39234, #19379, #22629, #26296, #35592, #192, #39025, #33781, #13097, #19796, #42249, #17347, #4204, #13313, #39445, #16119, #3412, #30551, #20593, #9671, #26502, #39649, #10663, #26082, #12888, #12468, #9461, #6234, #9880, #23856, #32568, #25662, #2994, #38817, #35802, #23054, #37005, #29316, #36210, #32983, #6646, #32768, #7440, #6020, #42460, #3204, #9244, #16549, #22844, #36006, #22414, #6443, #19585, #16330, #42671, #29529, #19170, #29747, #32359, #2783, #15912, #12674, #25870, #21242, #1404, #41072, #31191, #28162, #37865, #34639, #10877, #24292, #41296, #1191, #14750, #14964, #37436, #4418, #24934, #18429, #27298, #21455, #24719, #30758, #11735, #5065, #1838, #27945, #18213, #11517, #20811, #40433, #14313, #37651, #14096, #27513, #38078, #24069, #8518, #40647, #17558, #33997, #27728, #31403, #30974, #21671, #34854, #5276, #17778, #11089, #8091, #11305, #978, #1621, #4847, #17991, #37211, #7879, #8310, #7658, #21026, #34216, #34427, #4632, #14534, #40864, #24499, #22529, #38928, #25568, #5494, #18644, #15182, #19274, #2275, #9360, #6131, #29011, #21888, #42151, #8734, #9568, #12370, #5922, #35702, #41520, #28593, #25141, #31838, #2476, #29220, #2681, #32470, #15396, #22108, #41724, #9154, #12162, #28378, #32047, #38501, #2894, #25354, #8944, #35282, #19073, #38720, #42359, #15605, #16024, #5715, #12792, #11950, #18867, #22321, #28807, #12582, #32254, #25984, #25775, #39136, #38288, #41939, #22742, #35496, #15815, #35908, #6345, #35067, #31618, #2051, #3104, #39978, #518, #6547, #33529, #10409, #20337, #3742, #23601, #33317, #39340, #16232, #32884, #13420, #32675, #19701, #728, #29432, #30289, #3315, #36114, #9779, #3524, #36746, #6757, #3952, #13847, #17090, #36326, #22959, #26615, #29861, #40187, #6974, #23384, #36533, #12996, #16445, #26825, #42573, #36959, #13633, #39764, #7183, #26192, #10198, #20129, #29643, #16660, #26403, #87, #16872, #13209, #27043, #39553, #10617, #30077, #23805, #9984, #19488, #23163, #19911, #33098, #299, #1358, #20549, #7612, #31360, #4159, #18166, #37165, #24025, #27247, #34169, #27897, #37392, #34594, #1791, #21408, #24241, #10831, #14488, #17728, #28120, #37605, #11261, #24458, #935, #40388, #14707, #17304, #24886, #31145, #27683, #11473, #30508, #40821, #8048, #20766, #4589, #14267, #17517, #21195, #14052, #37820, #33955, #41248, #34382, #41030, #4377, #11690, #7401, #8263, #4798, #11047, #24674, #33738, #14921, #30923, #5025, #30715, #1143, #20983, #7835, #27469, #40604, #17947, #1578, #38880, #31790, #12736, #2224, #29175, #21843, #5872, #6086, #15351, #19026, #15769, #32210, #15561, #19233, #31575, #2638, #12538, #25730, #21632, #38456, #28549, #9311, #18602, #35022, #5452, #25522, #2427, #35655, #22062, #28966, #41681, #32422, #5233, #12119, #28762, #8897, #35446, #38671, #22479, #42103, #2845, #18385, #25311, #15978, #38245, #9106, #42314, #35234, #41469, #38035, #8478, #34810, #2007, #15134, #25099, #28331, #11904, #8690, #22274, #5665, #18817, #32001, #41890, #12324, #10358, #13162, #9524, #16612, #32838, #26568, #3058, #33481, #6712, #16396, #22912, #20291, #26356, #29380, #29596, #10153, #23549, #39509, #26143, #36697, #39717, #19864, #39295, #23334, #9939, #3476, #36067, #23117, #13585, #9731, #16183, #7137, #39930, #19439, #36282, #6503, #33050, #36487, #19653, #30241, #6923, #3267, #35863, #32631, #16825, #33270, #29814, #42523, #12948, #22694, #26778, #39, #3696, #470, #20076, #255, #30023, #13376, #3907, #17041, #681, #25936, #6297, #39085, #7354, #884, #27417, #11422, #27630, #14657, #40342, #4326, #34111, #7990, #31091, #14003, #27846, #34328, #40553, #20501, #33688, #4114, #27198, #17464, #23974, #4533, #14438, #17254, #10784, #40141, #20714, #11211, #10997, #4746, #7562, #23755, #18114, #1524, #13798, #24191, #10569, #37339, #7785, #20929, #21359, #40769, #24410, #14217, #30663, #30870, #17675, #30457, #26982, #1306, #37551, #21142, #37118, #8210, #17892, #34542, #1091, #4968, #37765, #40979, #33904, #24616, #31309, #36908, #37983, #34759, #9052, #41190, #19182, #25470, #22004, #5818, #24837, #8846, #2378, #18334, #28499, #8637, #11851, #15505, #8427, #32158, #28279, #22426, #28710, #22219, #31523, #6032, #35605, #2588, #41836, #5396, #35394, #1741, #9258, #41629, #15717, #28916, #42053, #15302, #2167, #14867, #41415, #38193, #12274, #12481, #21792, #28064, #34972, #11631, #25050, #38615, #25676, #18548, #18973, #38828, #21580, #35180, #5180, #1952, #15078, #31738, #12065, #25259, #38404, #5605, #18760, #31949, #29329, #42472, #19808, #39458, #29973, #16343, #39663, #16131, #416, #42261, #9683, #9892, #32780, #29759, #32996, #16773, #26515, #23276, #12686, #12899, #13536, #32582, #3424, #3646, #26095, #35814, #26721, #7088, #15925, #10099, #13325, #19390, #39874, #36435, #33215, #16562, #6871, #205, #9474, #29126, #3007, #26308, #2795, #39245, #10307, #25884, #23495, #22856, #6247, #22642, #29541, #20023, #19599, #36643, #32371, #39037, #6457, #36019, #23067, #42684, #3217, #13109, #36223, #6658, #11368, #4056, #30818, #31037, #13952, #1256, #40714, #14380, #40497, #1469, #13739, #27577, #37496, #7939, #3854, #20658, #27145, #21089, #831, #17198, #30399, #7726, #27361, #17841, #4270, #11155, #40288, #14603, #30187, #10730, #10942, #33846, #17623, #20873, #4692, #24354, #34277, #623, #23922, #27793, #20447, #34059, #40925, #37066, #23704, #24564, #37713, #16989, #20238, #33427, #7297, #26929, #40087, #10518, #4481, #36854, #33634, #7508, #17411, #30609, #14162, #1037, #24137, #37278, #4913, #18922, #37928, #24784, #28009, #34916, #28656, #38141, #35341, #2538, #22167, #24999, #11577, #15245, #18493, #28865, #38351, #12012, #25208, #1683, #41137, #15457, #18061, #25623, #31900, #28445, #12221, #31257, #41580, #8790, #8374, #5338, #15026, #18274, #21948, #14812, #38558, #34706, #41999, #35129, #41786, #21524, #12428, #8155, #8999, #5552, #11796, #25413, #21303, #15664, #31681, #5769, #32106, #34492, #21737, #8584, #5127, #31464, #1897, #18705, #28226, #41359, #2115, #2328, #29277, #35764, #33159, #39195, #42210, #42421, #23016, #36385, #9630, #38985, #6818, #9838, #32729, #9421, #39402, #22801, #16292, #6192, #35966, #26460, #22587, #15870, #23225, #10045, #32318, #6404, #19336, #3165, #36170, #32526, #360, #6605, #2955, #5982, #2744, #29705, #3372, #29490, #12637, #25830, #22376, #39609, #16082, #16507, #13271, #19759, #29072, #32942, #12851, #16723, #19545, #13059, #150, #19133, #26043, #42629, #26252, #19973, #3591, #29918, #13482, #38780, #9206, #35553, #20822, #1203, #26881, #40659, #4430, #40239, #20189, #33378, #3798, #40036, #30349, #36804, #17360, #27311, #16936, #10466, #10255, #33584, #24082, #23869, #17569, #20392, #36589, #30987, #14328, #26671, #10676, #23441, #37017, #7457, #33793, #34227, #40446, #10890, #27097, #779, #990, #30561, #30133, #39822, #14108, #37222, #4218, #23656, #21037, #7670, #4643, #17148, #17791, #7890, #34009, #571, #4005, #1416, #7242, #11099, #13904, #7036, #30770, #20606, #27524, #13689, #24302, #37446, #28389, #29182, #37876, #18001, #39093, #32639, #40876, #35662, #38297, #1631, #42322, #6093, #15986, #41529, #19240, #11959, #34439, #11316, #27955, #8527, #27739, #14760, #9532, #24509, #25944, #41084, #31203, #4859, #41306, #32429, #1848, #12745, #22702, #35870, #31412, #11527, #21682, #24944, #6303, #2061, #18438, #31629, #8101, #24730, #22487, #37662, #14548, #8742, #34864, #2853, #21252, #5286, #15191, #8321, #11744, #21466, #34648, #25149, #5076, #19448, #18222, #14974, #28172, #38087, #32847, #7361, #23762, #3914, #30033, #6721, #36705, #20509, #10576, #263, #17048, #30249, #687, #16620, #3484, #3066, #29604, #39517, #478, #13805, #9946, #16192, #23126, #36916, #47, #13594, #26994, #36290, #26785, #23557, #39936, #23344, #40148, #39302, #10366, #20297, #33488, #29390, #29823, #19873, #42531, #26365, #13171, #33058, #33279, #10161, #12956, #13384, #7144, #26576, #26151, #9740, #39726, #36495, #6931, #22921, #3704, #36075, #6512, #19661, #3275, #20085, #16404, #16833, #34122, #40562, #21368, #14226, #30671, #1099, #21151, #40779, #31318, #17684, #40989, #17474, #1750, #892, #11006, #11220, #4542, #31100, #34338, #18123, #27855, #24628, #14010, #27428, #14878, #33914, #4755, #4977, #24200, #37125, #28074, #8436, #17261, #11431, #14666, #20723, #41202, #37775, #34551, #17904, #8219, #1533, #10793, #30465, #4333, #27639, #4122, #37349, #11641, #27205, #24845, #7796, #7570, #23983, #30881, #37992, #20939, #33694, #40349, #1315, #14447, #24420, #37560, #7999, #42267, #9060, #25478, #38625, #15089, #11861, #28924, #18343, #39043, #2596, #41844, #25683, #1961, #28718, #22228, #38201, #5614, #28507, #31747, #35402, #28286, #9265, #5408, #12693, #5827, #42061, #8645, #25889, #21589, #22433, #18981, #25267, #12490, #34768, #29133, #18768, #35612, #6039, #19189, #35187, #22015, #5189, #18557, #15310, #32166, #32378, #41637, #31532, #12073, #41423, #2175, #15725, #2803, #38413, #38836, #15932, #25058, #12283, #21800, #34980, #8856, #31957, #2386, #15513, #26938, #33222, #29766, #13543, #32588, #16569, #10107, #26101, #36232, #16348, #19606, #23283, #3014, #39882, #36025, #30195, #36444, #16780, #39252, #13748, #633, #10317, #6879, #13115, #423, #9480, #16998, #6665, #23503, #36652, #7095, #23074, #9899, #22648, #6463, #3224, #20031, #20246, #29548, #35821, #40775, #6253, #32786, #3653, #33436, #26314, #29980, #26729, #3862, #212, #19396, #16137, #29336, #42478, #12905, #9688, #19815, #39465, #22862, #33004, #3432, #13332, #39670, #26522, #37721, #24147, #4699, #23930, #8163, #7305, #17420, #17631, #40505, #37504, #27585, #24573, #34284, #31046, #20455, #20667, #21312, #40295, #11164, #11375, #33854, #839, #34500, #14819, #23711, #17849, #21097, #27153, #4921, #1477, #40933, #24363, #14612, #7947, #17206, #36862, #10738, #34068, #10527, #37074, #18069, #33643, #31266, #7517, #13960, #30408, #37287, #27801, #27370, #1692, #40095, #4065, #14170, #4278, #4489, #7733, #30617, #40723, #1264, #14388, #1045, #10951, #20881, #30826, #37938, #32325, #15672, #28017, #41589, #11585, #25217, #12021, #35137, #35562, #28665 ) ),
 .UNSPECIFIED., .F., .F., .F. ) 
 B_SPLINE_SURFACE_WITH_KNOTS ( ( 2, 2 ),
 ( 3, 2, 2, 2, 2, 2, 2, 2, 2, 2, 2, 2, 2, 2, 2, 2, 2, 2, 2, 2, 2, 2, 2, 2, 2, 2, 2, 2, 2, 2, 2, 2, 2, 2, 2, 2, 2, 2, 2, 2, 2, 2, 2, 2, 2, 2, 2, 2, 2, 2, 2, 2, 2, 2, 2, 2, 2, 2, 2, 2, 2, 2, 2, 2, 2, 2, 2, 2, 2, 2, 2, 2, 2, 2, 2, 2, 2, 2, 2, 2, 2, 2, 2, 2, 2, 2, 2, 2, 2, 2, 2, 2, 2, 2, 2, 2, 2, 2, 2, 2, 2, 2, 2, 2, 2, 2, 2, 2, 2, 2, 2, 2, 2, 2, 2, 2, 2, 2, 2, 2, 2, 2, 2, 2, 2, 2, 2, 2, 2, 2, 2, 2, 2, 2, 2, 2, 2, 2, 2, 2, 2, 2, 2, 2, 2, 2, 2, 2, 2, 2, 2, 2, 2, 2, 2, 2, 2, 2, 2, 2, 2, 2, 2, 2, 2, 2, 2, 2, 2, 2, 2, 2, 2, 2, 2, 2, 2, 2, 2, 2, 2, 2, 2, 2, 2, 2, 2, 2, 2, 2, 2, 2, 2, 2, 2, 2, 2, 2, 2, 2, 2, 2, 2, 2, 2, 2, 2, 2, 2, 2, 2, 2, 2, 2, 2, 2, 2, 2, 2, 2, 2, 2, 2, 2, 2, 2, 2, 2, 2, 2, 2, 2, 2, 2, 2, 2, 2, 2, 2, 2, 2, 2, 2, 2, 2, 2, 2, 2, 2, 2, 2, 2, 2, 2, 2, 2, 2, 2, 2, 2, 2, 2, 2, 2, 2, 2, 2, 2, 2, 2, 2, 2, 2, 2, 2, 2, 2, 2, 2, 2, 2, 2, 2, 2, 2, 2, 2, 2, 2, 2, 2, 2, 2, 2, 2, 2, 2, 2, 2, 2, 2, 2, 2, 2, 2, 2, 2, 2, 2, 2, 2, 2, 2, 2, 2, 2, 2, 2, 2, 2, 2, 2, 2, 2, 2, 2, 2, 2, 2, 2, 2, 2, 2, 2, 2, 2, 2, 2, 2, 2, 2, 2, 2, 2, 2, 2, 2, 2, 2, 2, 2, 2, 2, 2, 2, 2, 2, 2, 2, 2, 2, 2, 2, 2, 2, 2, 2, 2, 2, 2, 2, 2, 2, 2, 2, 2, 2, 2, 2, 2, 2, 2, 2, 2, 2, 2, 2, 2, 2, 2, 2, 2, 2, 2, 2, 2, 2, 2, 2, 2, 2, 2, 2, 2, 2, 2, 2, 2, 2, 2, 2, 2, 2, 2, 2, 2, 2, 2, 2, 2, 2, 2, 2, 2, 2, 2, 2, 2, 2, 2, 2, 2, 2, 2, 2, 2, 2, 2, 2, 2, 2, 2, 2, 2, 2, 2, 2, 2, 2, 2, 2, 2, 2, 2, 2, 2, 2, 2, 2, 2, 2, 2, 2, 2, 2, 2, 2, 2, 2, 2, 2, 2, 2, 2, 2, 2, 2, 2, 2, 2, 2, 2, 2, 2, 2, 2, 2, 2, 2, 2, 2, 2, 2, 2, 2, 2, 2, 2, 2, 2, 2, 2, 2, 2, 2, 2, 2, 2, 2, 2, 2, 2, 2, 2, 2, 2, 2, 2, 2, 2, 2, 2, 2, 2, 2, 2, 2, 2, 2, 2, 2, 2, 2, 2, 2, 2, 2, 2, 2, 2, 2, 2, 2, 2, 2, 2, 2, 2, 2, 2, 2, 2, 2, 2, 2, 2, 2, 2, 2, 2, 2, 2, 2, 2, 2, 2, 2, 2, 2, 2, 2, 2, 2, 2, 2, 2, 2, 2, 2, 2, 2, 2, 2, 2, 2, 2, 2, 2, 2, 2, 2, 2, 2, 2, 2, 2, 2, 2, 2, 2, 2, 2, 2, 2, 2, 2, 2, 2, 2, 2, 2, 2, 2, 2, 2, 2, 2, 2, 2, 2, 2, 2, 2, 2, 2, 2, 2, 2, 2, 2, 2, 2, 2, 2, 2, 2, 2, 2, 2, 2, 2, 2, 2, 2, 2, 2, 2, 2, 2, 2, 2, 2, 2, 2, 2, 2, 2, 2, 2, 2, 2, 2, 2, 2, 2, 2, 2, 2, 2, 2, 2, 2, 2, 2, 2, 2, 2, 2, 2, 2, 2, 2, 2, 2, 2, 2, 2, 2, 2, 2, 2, 2, 2, 2, 2, 2, 2, 2, 2, 2, 2, 2, 2, 2, 2, 2, 2, 2, 2, 2, 2, 2, 2, 2, 2, 2, 2, 2, 2, 2, 2, 2, 2, 2, 2, 2, 2, 2, 2, 2, 2, 2, 2, 2, 2, 2, 2, 2, 2, 2, 2, 2, 2, 2, 2, 2, 2, 2, 2, 2, 2, 2, 2, 2, 2, 2, 2, 2, 2, 2, 2, 2, 2, 2, 2, 2, 2, 2, 2, 2, 2, 2, 2, 2, 2, 2, 2, 2, 2, 2, 2, 2, 2, 2, 2, 2, 2, 2, 2, 2, 2, 2, 2, 2, 2, 2, 2, 2, 2, 2, 3 ),
 ( 0.000000000000000000, 1.000000000000000000 ),
 ( 0.000000000000000000, 0.001243781094527363160, 0.002487562189054726321, 0.003731343283582089481, 0.004975124378109452641, 0.006218905472636816235, 0.007462686567164178962, 0.008706467661691542556, 0.009950248756218905283, 0.01119402985074626801, 0.01243781094527363247, 0.01368159203980099520, 0.01492537313432835792, 0.01616915422885572065, 0.01741293532338308511, 0.01865671641791044610, 0.01990049751243781057, 0.02114427860696517503, 0.02238805970149253602, 0.02363184079601990048, 0.02487562189054726494, 0.02611940298507462593, 0.02736318407960199039, 0.02860696517412935486, 0.02985074626865671585, 0.03109452736318408031, 0.03233830845771144130, 0.03358208955223880576, 0.03482587064676617022, 0.03606965174129353469, 0.03731343283582089221, 0.03855721393034825667, 0.03980099502487562113, 0.04104477611940298559, 0.04228855721393035005, 0.04353233830845771452, 0.04477611940298507204, 0.04601990049751243650, 0.04726368159203980096, 0.04850746268656716542, 0.04975124378109452988, 0.05099502487562188741, 0.05223880597014925187, 0.05348258706467661633, 0.05472636815920398079, 0.05597014925373134525, 0.05721393034825870971, 0.05845771144278606724, 0.05970149253731343170, 0.06094527363184079616, 0.06218905472636816062, 0.06343283582089552508, 0.06467661691542288260, 0.06592039800995025400, 0.06716417910447761153, 0.06840796019900496905, 0.06965174129353234045, 0.07089552238805969797, 0.07213930348258706937, 0.07338308457711442689, 0.07462686567164178442, 0.07587064676616915582, 0.07711442786069651334, 0.07835820895522388474, 0.07960199004975124226, 0.08084577114427861366, 0.08208955223880597118, 0.08333333333333332871, 0.08457711442786070011, 0.08582089552238805763, 0.08706467661691542903, 0.08830845771144278655, 0.08955223880597014408, 0.09079601990049751548, 0.09203980099502487300, 0.09328358208955224440, 0.09452736318407960192, 0.09577114427860695944, 0.09701492537313433084, 0.09825870646766168837, 0.09950248756218905977, 0.1007462686567164173, 0.1019900497512437748, 0.1032338308457711462, 0.1044776119402985037, 0.1057213930348258751, 0.1069651741293532327, 0.1082089552238805902, 0.1094527363184079616, 0.1106965174129353191, 0.1119402985074626905, 0.1131840796019900480, 0.1144278606965174194, 0.1156716417910447769, 0.1169154228855721345, 0.1181592039800995059, 0.1194029850746268634, 0.1206467661691542348, 0.1218905472636815923, 0.1231343283582089498, 0.1243781094527363212, 0.1256218905472636926, 0.1268656716417910502, 0.1281094527363184077, 0.1293532338308457652, 0.1305970149253731227, 0.1318407960199005080, 0.1330845771144278655, 0.1343283582089552231, 0.1355721393034825806, 0.1368159203980099381, 0.1380597014925373234, 0.1393034825870646809, 0.1405472636815920384, 0.1417910447761193959, 0.1430348258706467535, 0.1442786069651741387, 0.1455223880597014963, 0.1467661691542288538, 0.1480099502487562113, 0.1492537313432835688, 0.1504975124378109541, 0.1517412935323383116, 0.1529850746268656692, 0.1542288557213930267, 0.1554726368159203842, 0.1567164179104477695, 0.1579601990049751270, 0.1592039800995024845, 0.1604477611940298420, 0.1616915422885572273, 0.1629353233830845848, 0.1641791044776119424, 0.1654228855721392999, 0.1666666666666666574, 0.1679104477611940427, 0.1691542288557214002, 0.1703980099502487577, 0.1716417910447761153, 0.1728855721393034728, 0.1741293532338308581, 0.1753731343283582156, 0.1766169154228855731, 0.1778606965174129306, 0.1791044776119402882, 0.1803482587064676734, 0.1815920398009950310, 0.1828358208955223885, 0.1840796019900497460, 0.1853233830845771035, 0.1865671641791044888, 0.1878109452736318463, 0.1890547263681592038, 0.1902985074626865614, 0.1915422885572139189, 0.1927860696517413042, 0.1940298507462686617, 0.1952736318407960192, 0.1965174129353233767, 0.1977611940298507343, 0.1990049751243781195, 0.2002487562189054771, 0.2014925373134328346, 0.2027363184079601921, 0.2039800995024875496, 0.2052238805970149349, 0.2064676616915422924, 0.2077114427860696499, 0.2089552238805970075, 0.2101990049751243650, 0.2114427860696517503, 0.2126865671641791078, 0.2139303482587064653, 0.2151741293532338228, 0.2164179104477611804, 0.2176616915422885656, 0.2189054726368159232, 0.2201492537313432807, 0.2213930348258706382, 0.2226368159203980235, 0.2238805970149253810, 0.2251243781094527385, 0.2263681592039800961, 0.2276119402985074536, 0.2288557213930348389, 0.2300995024875621964, 0.2313432835820895539, 0.2325870646766169114, 0.2338308457711442689, 0.2350746268656716542, 0.2363184079601990117, 0.2375621890547263693, 0.2388059701492537268, 0.2400497512437810843, 0.2412935323383084696, 0.2425373134328358271, 0.2437810945273631846, 0.2450248756218905422, 0.2462686567164178997, 0.2475124378109452850, 0.2487562189054726425, 0.2500000000000000000, 0.2512437810945273853, 0.2524875621890547150, 0.2537313432835821003, 0.2549751243781094301, 0.2562189054726368154, 0.2574626865671642006, 0.2587064676616915304, 0.2599502487562189157, 0.2611940298507462455, 0.2624378109452736307, 0.2636815920398010160, 0.2649253731343283458, 0.2661691542288557311, 0.2674129353233830608, 0.2686567164179104461, 0.2699004975124378314, 0.2711442786069651611, 0.2723880597014925464, 0.2736318407960198762, 0.2748756218905472615, 0.2761194029850746468, 0.2773631840796019765, 0.2786069651741293618, 0.2798507462686566916, 0.2810945273631840768, 0.2823383084577114621, 0.2835820895522387919, 0.2848258706467661772, 0.2860696517412935069, 0.2873134328358208922, 0.2885572139303482775, 0.2898009950248756073, 0.2910447761194029925, 0.2922885572139303223, 0.2935323383084577076, 0.2947761194029850929, 0.2960199004975124226, 0.2972636815920398079, 0.2985074626865671377, 0.2997512437810945229, 0.3009950248756219082, 0.3022388059701492380, 0.3034825870646766233, 0.3047263681592039530, 0.3059701492537313383, 0.3072139303482587236, 0.3084577114427860534, 0.3097014925373134386, 0.3109452736318407684, 0.3121890547263681537, 0.3134328358208955390, 0.3146766169154228687, 0.3159203980099502540, 0.3171641791044776393, 0.3184079601990049690, 0.3196517412935323543, 0.3208955223880596841, 0.3221393034825870694, 0.3233830845771144546, 0.3246268656716417844, 0.3258706467661691697, 0.3271144278606964995, 0.3283582089552238847, 0.3296019900497512700, 0.3308457711442785998, 0.3320895522388059851, 0.3333333333333333148, 0.3345771144278607001, 0.3358208955223880854, 0.3370646766169154152, 0.3383084577114428004, 0.3395522388059701302, 0.3407960199004975155, 0.3420398009950249008, 0.3432835820895522305, 0.3445273631840796158, 0.3457711442786069456, 0.3470149253731343308, 0.3482587064676617161, 0.3495024875621890459, 0.3507462686567164312, 0.3519900497512437609, 0.3532338308457711462, 0.3544776119402985315, 0.3557213930348258613, 0.3569651741293532465, 0.3582089552238805763, 0.3594527363184079616, 0.3606965174129353469, 0.3619402985074626766, 0.3631840796019900619, 0.3644278606965173917, 0.3656716417910447769, 0.3669154228855721622, 0.3681592039800994920, 0.3694029850746268773, 0.3706467661691542070, 0.3718905472636815923, 0.3731343283582089776, 0.3743781094527363074, 0.3756218905472636926, 0.3768656716417910224, 0.3781094527363184077, 0.3793532338308457930, 0.3805970149253731227, 0.3818407960199005080, 0.3830845771144278378, 0.3843283582089552231, 0.3855721393034826083, 0.3868159203980099381, 0.3880597014925373234, 0.3893034825870646531, 0.3905472636815920384, 0.3917910447761194237, 0.3930348258706467535, 0.3942786069651741387, 0.3955223880597014685, 0.3967661691542288538, 0.3980099502487562391, 0.3992537313432835688, 0.4004975124378109541, 0.4017412935323382839, 0.4029850746268656692, 0.4042288557213930544, 0.4054726368159203842, 0.4067164179104477695, 0.4079601990049750992, 0.4092039800995024845, 0.4104477611940298698, 0.4116915422885571996, 0.4129353233830845848, 0.4141791044776119146, 0.4154228855721392999, 0.4166666666666666852, 0.4179104477611940149, 0.4191542288557214002, 0.4203980099502487300, 0.4216417910447761153, 0.4228855721393035005, 0.4241293532338308303, 0.4253731343283582156, 0.4266169154228855454, 0.4278606965174129306, 0.4291044776119403159, 0.4303482587064676457, 0.4315920398009950310, 0.4328358208955223607, 0.4340796019900497460, 0.4353233830845771313, 0.4365671641791044610, 0.4378109452736318463, 0.4390547263681592316, 0.4402985074626865614, 0.4415422885572139466, 0.4427860696517412764, 0.4440298507462686617, 0.4452736318407960470, 0.4465174129353233767, 0.4477611940298507620, 0.4490049751243780918, 0.4502487562189054771, 0.4514925373134328623, 0.4527363184079601921, 0.4539800995024875774, 0.4552238805970149071, 0.4564676616915422924, 0.4577114427860696777, 0.4589552238805970075, 0.4601990049751243927, 0.4614427860696517225, 0.4626865671641791078, 0.4639303482587064931, 0.4651741293532338228, 0.4664179104477612081, 0.4676616915422885379, 0.4689054726368159232, 0.4701492537313433084, 0.4713930348258706382, 0.4726368159203980235, 0.4738805970149253532, 0.4751243781094527385, 0.4763681592039801238, 0.4776119402985074536, 0.4788557213930348389, 0.4800995024875621686, 0.4813432835820895539, 0.4825870646766169392, 0.4838308457711442689, 0.4850746268656716542, 0.4863184079601989840, 0.4875621890547263693, 0.4888059701492537545, 0.4900497512437810843, 0.4912935323383084696, 0.4925373134328357994, 0.4937810945273631846, 0.4950248756218905699, 0.4962686567164178997, 0.4975124378109452850, 0.4987562189054726147, 0.5000000000000000000, 0.5012437810945273853, 0.5024875621890547706, 0.5037313432835820448, 0.5049751243781094301, 0.5062189054726368154, 0.5074626865671642006, 0.5087064676616915859, 0.5099502487562188602, 0.5111940298507462455, 0.5124378109452736307, 0.5136815920398010160, 0.5149253731343284013, 0.5161691542288556755, 0.5174129353233830608, 0.5186567164179104461, 0.5199004975124378314, 0.5211442786069652167, 0.5223880597014924909, 0.5236318407960198762, 0.5248756218905472615, 0.5261194029850746468, 0.5273631840796020320, 0.5286069651741293063, 0.5298507462686566916, 0.5310945273631840768, 0.5323383084577114621, 0.5335820895522388474, 0.5348258706467661217, 0.5360696517412935069, 0.5373134328358208922, 0.5385572139303482775, 0.5398009950248756628, 0.5410447761194029370, 0.5422885572139303223, 0.5435323383084577076, 0.5447761194029850929, 0.5460199004975124781, 0.5472636815920397524, 0.5485074626865671377, 0.5497512437810945229, 0.5509950248756219082, 0.5522388059701492935, 0.5534825870646765678, 0.5547263681592039530, 0.5559701492537313383, 0.5572139303482587236, 0.5584577114427861089, 0.5597014925373133831, 0.5609452736318407684, 0.5621890547263681537, 0.5634328358208955390, 0.5646766169154229242, 0.5659203980099501985, 0.5671641791044775838, 0.5684079601990049690, 0.5696517412935323543, 0.5708955223880597396, 0.5721393034825870139, 0.5733830845771143991, 0.5746268656716417844, 0.5758706467661691697, 0.5771144278606965550, 0.5783582089552238292, 0.5796019900497512145, 0.5808457711442785998, 0.5820895522388059851, 0.5833333333333333703, 0.5845771144278606446, 0.5858208955223880299, 0.5870646766169154152, 0.5883084577114428004, 0.5895522388059701857, 0.5907960199004974600, 0.5920398009950248452, 0.5932835820895522305, 0.5945273631840796158, 0.5957711442786070011, 0.5970149253731342753, 0.5982587064676616606, 0.5995024875621890459, 0.6007462686567164312, 0.6019900497512438164, 0.6032338308457710907, 0.6044776119402984760, 0.6057213930348258613, 0.6069651741293532465, 0.6082089552238806318, 0.6094527363184079061, 0.6106965174129352913, 0.6119402985074626766, 0.6131840796019900619, 0.6144278606965174472, 0.6156716417910447214, 0.6169154228855721067, 0.6181592039800994920, 0.6194029850746268773, 0.6206467661691542625, 0.6218905472636815368, 0.6231343283582089221, 0.6243781094527363074, 0.6256218905472636926, 0.6268656716417910779, 0.6281094527363184632, 0.6293532338308457375, 0.6305970149253731227, 0.6318407960199005080, 0.6330845771144278933, 0.6343283582089552786, 0.6355721393034825528, 0.6368159203980099381, 0.6380597014925373234, 0.6393034825870647087, 0.6405472636815920939, 0.6417910447761193682, 0.6430348258706467535, 0.6442786069651741387, 0.6455223880597015240, 0.6467661691542289093, 0.6480099502487561836, 0.6492537313432835688, 0.6504975124378109541, 0.6517412935323383394, 0.6529850746268657247, 0.6542288557213929989, 0.6554726368159203842, 0.6567164179104477695, 0.6579601990049751548, 0.6592039800995025400, 0.6604477611940298143, 0.6616915422885571996, 0.6629353233830845848, 0.6641791044776119701, 0.6654228855721393554, 0.6666666666666666297, 0.6679104477611940149, 0.6691542288557214002, 0.6703980099502487855, 0.6716417910447761708, 0.6728855721393034450, 0.6741293532338308303, 0.6753731343283582156, 0.6766169154228856009, 0.6778606965174129861, 0.6791044776119402604, 0.6803482587064676457, 0.6815920398009950310, 0.6828358208955224162, 0.6840796019900498015, 0.6853233830845770758, 0.6865671641791044610, 0.6878109452736318463, 0.6890547263681592316, 0.6902985074626866169, 0.6915422885572138911, 0.6927860696517412764, 0.6940298507462686617, 0.6952736318407960470, 0.6965174129353234322, 0.6977611940298507065, 0.6990049751243780918, 0.7002487562189054771, 0.7014925373134328623, 0.7027363184079602476, 0.7039800995024875219, 0.7052238805970149071, 0.7064676616915422924, 0.7077114427860696777, 0.7089552238805970630, 0.7101990049751243372, 0.7114427860696517225, 0.7126865671641791078, 0.7139303482587064931, 0.7151741293532338783, 0.7164179104477611526, 0.7176616915422885379, 0.7189054726368159232, 0.7201492537313433084, 0.7213930348258706937, 0.7226368159203979680, 0.7238805970149253532, 0.7251243781094527385, 0.7263681592039801238, 0.7276119402985075091, 0.7288557213930347833, 0.7300995024875621686, 0.7313432835820895539, 0.7325870646766169392, 0.7338308457711443245, 0.7350746268656715987, 0.7363184079601989840, 0.7375621890547263693, 0.7388059701492537545, 0.7400497512437811398, 0.7412935323383084141, 0.7425373134328357994, 0.7437810945273631846, 0.7450248756218905699, 0.7462686567164179552, 0.7475124378109452294, 0.7487562189054726147, 0.7500000000000000000, 0.7512437810945273853, 0.7524875621890547706, 0.7537313432835820448, 0.7549751243781094301, 0.7562189054726368154, 0.7574626865671642006, 0.7587064676616915859, 0.7599502487562188602, 0.7611940298507462455, 0.7624378109452736307, 0.7636815920398010160, 0.7649253731343284013, 0.7661691542288556755, 0.7674129353233830608, 0.7686567164179104461, 0.7699004975124378314, 0.7711442786069652167, 0.7723880597014924909, 0.7736318407960198762, 0.7748756218905472615, 0.7761194029850746468, 0.7773631840796020320, 0.7786069651741293063, 0.7798507462686566916, 0.7810945273631840768, 0.7823383084577114621, 0.7835820895522388474, 0.7848258706467661217, 0.7860696517412935069, 0.7873134328358208922, 0.7885572139303482775, 0.7898009950248756628, 0.7910447761194029370, 0.7922885572139303223, 0.7935323383084577076, 0.7947761194029850929, 0.7960199004975124781, 0.7972636815920397524, 0.7985074626865671377, 0.7997512437810945229, 0.8009950248756219082, 0.8022388059701492935, 0.8034825870646765678, 0.8047263681592039530, 0.8059701492537313383, 0.8072139303482587236, 0.8084577114427861089, 0.8097014925373133831, 0.8109452736318407684, 0.8121890547263681537, 0.8134328358208955390, 0.8146766169154229242, 0.8159203980099501985, 0.8171641791044775838, 0.8184079601990049690, 0.8196517412935323543, 0.8208955223880597396, 0.8221393034825870139, 0.8233830845771143991, 0.8246268656716417844, 0.8258706467661691697, 0.8271144278606965550, 0.8283582089552238292, 0.8296019900497512145, 0.8308457711442785998, 0.8320895522388059851, 0.8333333333333333703, 0.8345771144278606446, 0.8358208955223880299, 0.8370646766169154152, 0.8383084577114428004, 0.8395522388059701857, 0.8407960199004974600, 0.8420398009950248452, 0.8432835820895522305, 0.8445273631840796158, 0.8457711442786070011, 0.8470149253731342753, 0.8482587064676616606, 0.8495024875621890459, 0.8507462686567164312, 0.8519900497512438164, 0.8532338308457710907, 0.8544776119402984760, 0.8557213930348258613, 0.8569651741293532465, 0.8582089552238806318, 0.8594527363184079061, 0.8606965174129352913, 0.8619402985074626766, 0.8631840796019900619, 0.8644278606965174472, 0.8656716417910447214, 0.8669154228855721067, 0.8681592039800994920, 0.8694029850746268773, 0.8706467661691542625, 0.8718905472636815368, 0.8731343283582089221, 0.8743781094527363074, 0.8756218905472636926, 0.8768656716417910779, 0.8781094527363184632, 0.8793532338308457375, 0.8805970149253731227, 0.8818407960199005080, 0.8830845771144278933, 0.8843283582089552786, 0.8855721393034825528, 0.8868159203980099381, 0.8880597014925373234, 0.8893034825870647087, 0.8905472636815920939, 0.8917910447761193682, 0.8930348258706467535, 0.8942786069651741387, 0.8955223880597015240, 0.8967661691542289093, 0.8980099502487561836, 0.8992537313432835688, 0.9004975124378109541, 0.9017412935323383394, 0.9029850746268657247, 0.9042288557213929989, 0.9054726368159203842, 0.9067164179104477695, 0.9079601990049751548, 0.9092039800995025400, 0.9104477611940298143, 0.9116915422885571996, 0.9129353233830845848, 0.9141791044776119701, 0.9154228855721393554, 0.9166666666666666297, 0.9179104477611940149, 0.9191542288557214002, 0.9203980099502487855, 0.9216417910447761708, 0.9228855721393034450, 0.9241293532338308303, 0.9253731343283582156, 0.9266169154228856009, 0.9278606965174129861, 0.9291044776119402604, 0.9303482587064676457, 0.9315920398009950310, 0.9328358208955224162, 0.9340796019900498015, 0.9353233830845770758, 0.9365671641791044610, 0.9378109452736318463, 0.9390547263681592316, 0.9402985074626866169, 0.9415422885572138911, 0.9427860696517412764, 0.9440298507462686617, 0.9452736318407960470, 0.9465174129353234322, 0.9477611940298507065, 0.9490049751243780918, 0.9502487562189054771, 0.9514925373134328623, 0.9527363184079602476, 0.9539800995024875219, 0.9552238805970149071, 0.9564676616915422924, 0.9577114427860696777, 0.9589552238805970630, 0.9601990049751243372, 0.9614427860696517225, 0.9626865671641791078, 0.9639303482587064931, 0.9651741293532338783, 0.9664179104477611526, 0.9676616915422885379, 0.9689054726368159232, 0.9701492537313433084, 0.9713930348258706937, 0.9726368159203979680, 0.9738805970149253532, 0.9751243781094527385, 0.9763681592039801238, 0.9776119402985075091, 0.9788557213930347833, 0.9800995024875621686, 0.9813432835820895539, 0.9825870646766169392, 0.9838308457711443245, 0.9850746268656715987, 0.9863184079601989840, 0.9875621890547263693, 0.9888059701492537545, 0.9900497512437811398, 0.9912935323383084141, 0.9925373134328357994, 0.9937810945273631846, 0.9950248756218905699 ),
 .UNSPECIFIED. ) 
 GEOMETRIC_REPRESENTATION_ITEM ( )  RATIONAL_B_SPLINE_SURFACE ( (
 ( 1.000000000000000000, 0.8660254037844387076, 1.000000000000000000, 0.8660254037844387076, 1.000000000000000000, 0.8660254037844387076, 1.000000000000000000, 0.8660254037844387076, 1.000000000000000000, 0.8660254037844387076, 1.000000000000000000, 0.8660254037844387076, 1.000000000000000000, 0.8660254037844387076, 1.000000000000000000, 0.8660254037844387076, 1.000000000000000000, 0.8660254037844387076, 1.000000000000000000, 0.8660254037844387076, 1.000000000000000000, 0.8660254037844387076, 1.000000000000000000, 0.8660254037844387076, 1.000000000000000000, 0.8660254037844387076, 1.000000000000000000, 0.8660254037844387076, 1.000000000000000000, 0.8660254037844387076, 1.000000000000000000, 0.8660254037844387076, 1.000000000000000000, 0.8660254037844387076, 1.000000000000000000, 0.8660254037844387076, 1.000000000000000000, 0.8660254037844387076, 1.000000000000000000, 0.8660254037844387076, 1.000000000000000000, 0.8660254037844387076, 1.000000000000000000, 0.8660254037844387076, 1.000000000000000000, 0.8660254037844387076, 1.000000000000000000, 0.8660254037844387076, 1.000000000000000000, 0.8660254037844387076, 1.000000000000000000, 0.8660254037844387076, 1.000000000000000000, 0.8660254037844387076, 1.000000000000000000, 0.8660254037844387076, 1.000000000000000000, 0.8660254037844387076, 1.000000000000000000, 0.8660254037844387076, 1.000000000000000000, 0.8660254037844387076, 1.000000000000000000, 0.8660254037844387076, 1.000000000000000000, 0.8660254037844387076, 1.000000000000000000, 0.8660254037844387076, 1.000000000000000000, 0.8660254037844387076, 1.000000000000000000, 0.8660254037844387076, 1.000000000000000000, 0.8660254037844387076, 1.000000000000000000, 0.8660254037844387076, 1.000000000000000000, 0.8660254037844387076, 1.000000000000000000, 0.8660254037844387076, 1.000000000000000000, 0.8660254037844387076, 1.000000000000000000, 0.8660254037844387076, 1.000000000000000000, 0.8660254037844387076, 1.000000000000000000, 0.8660254037844387076, 1.000000000000000000, 0.8660254037844387076, 1.000000000000000000, 0.8660254037844387076, 1.000000000000000000, 0.8660254037844387076, 1.000000000000000000, 0.8660254037844387076, 1.000000000000000000, 0.8660254037844387076, 1.000000000000000000, 0.8660254037844387076, 1.000000000000000000, 0.8660254037844387076, 1.000000000000000000, 0.8660254037844387076, 1.000000000000000000, 0.8660254037844387076, 1.000000000000000000, 0.8660254037844387076, 1.000000000000000000, 0.8660254037844387076, 1.000000000000000000, 0.8660254037844387076, 1.000000000000000000, 0.8660254037844387076, 1.000000000000000000, 0.8660254037844387076, 1.000000000000000000, 0.8660254037844387076, 1.000000000000000000, 0.8660254037844387076, 1.000000000000000000, 0.8660254037844387076, 1.000000000000000000, 0.8660254037844387076, 1.000000000000000000, 0.8660254037844387076, 1.000000000000000000, 0.8660254037844387076, 1.000000000000000000, 0.8660254037844387076, 1.000000000000000000, 0.8660254037844387076, 1.000000000000000000, 0.8660254037844387076, 1.000000000000000000, 0.8660254037844387076, 1.000000000000000000, 0.8660254037844387076, 1.000000000000000000, 0.8660254037844387076, 1.000000000000000000, 0.8660254037844387076, 1.000000000000000000, 0.8660254037844387076, 1.000000000000000000, 0.8660254037844387076, 1.000000000000000000, 0.8660254037844387076, 1.000000000000000000, 0.8660254037844387076, 1.000000000000000000, 0.8660254037844387076, 1.000000000000000000, 0.8660254037844387076, 1.000000000000000000, 0.8660254037844387076, 1.000000000000000000, 0.8660254037844387076, 1.000000000000000000, 0.8660254037844387076, 1.000000000000000000, 0.8660254037844387076, 1.000000000000000000, 0.8660254037844387076, 1.000000000000000000, 0.8660254037844387076, 1.000000000000000000, 0.8660254037844387076, 1.000000000000000000, 0.8660254037844387076, 1.000000000000000000, 0.8660254037844387076, 1.000000000000000000, 0.8660254037844387076, 1.000000000000000000, 0.8660254037844387076, 1.000000000000000000, 0.8660254037844387076, 1.000000000000000000, 0.8660254037844387076, 1.000000000000000000, 0.8660254037844387076, 1.000000000000000000, 0.8660254037844387076, 1.000000000000000000, 0.8660254037844387076, 1.000000000000000000, 0.8660254037844387076, 1.000000000000000000, 0.8660254037844387076, 1.000000000000000000, 0.8660254037844387076, 1.000000000000000000, 0.8660254037844387076, 1.000000000000000000, 0.8660254037844387076, 1.000000000000000000, 0.8660254037844387076, 1.000000000000000000, 0.8660254037844387076, 1.000000000000000000, 0.8660254037844387076, 1.000000000000000000, 0.8660254037844387076, 1.000000000000000000, 0.8660254037844387076, 1.000000000000000000, 0.8660254037844387076, 1.000000000000000000, 0.8660254037844387076, 1.000000000000000000, 0.8660254037844387076, 1.000000000000000000, 0.8660254037844387076, 1.000000000000000000, 0.8660254037844387076, 1.000000000000000000, 0.8660254037844387076, 1.000000000000000000, 0.8660254037844387076, 1.000000000000000000, 0.8660254037844387076, 1.000000000000000000, 0.8660254037844387076, 1.000000000000000000, 0.8660254037844387076, 1.000000000000000000, 0.8660254037844387076, 1.000000000000000000, 0.8660254037844387076, 1.000000000000000000, 0.8660254037844387076, 1.000000000000000000, 0.8660254037844387076, 1.000000000000000000, 0.8660254037844387076, 1.000000000000000000, 0.8660254037844387076, 1.000000000000000000, 0.8660254037844387076, 1.000000000000000000, 0.8660254037844387076, 1.000000000000000000, 0.8660254037844387076, 1.000000000000000000, 0.8660254037844387076, 1.000000000000000000, 0.8660254037844387076, 1.000000000000000000, 0.8660254037844387076, 1.000000000000000000, 0.8660254037844387076, 1.000000000000000000, 0.8660254037844387076, 1.000000000000000000, 0.8660254037844387076, 1.000000000000000000, 0.8660254037844387076, 1.000000000000000000, 0.8660254037844387076, 1.000000000000000000, 0.8660254037844387076, 1.000000000000000000, 0.8660254037844387076, 1.000000000000000000, 0.8660254037844387076, 1.000000000000000000, 0.8660254037844387076, 1.000000000000000000, 0.8660254037844387076, 1.000000000000000000, 0.8660254037844387076, 1.000000000000000000, 0.8660254037844387076, 1.000000000000000000, 0.8660254037844387076, 1.000000000000000000, 0.8660254037844387076, 1.000000000000000000, 0.8660254037844387076, 1.000000000000000000, 0.8660254037844387076, 1.000000000000000000, 0.8660254037844387076, 1.000000000000000000, 0.8660254037844387076, 1.000000000000000000, 0.8660254037844387076, 1.000000000000000000, 0.8660254037844387076, 1.000000000000000000, 0.8660254037844387076, 1.000000000000000000, 0.8660254037844387076, 1.000000000000000000, 0.8660254037844387076, 1.000000000000000000, 0.8660254037844387076, 1.000000000000000000, 0.8660254037844387076, 1.000000000000000000, 0.8660254037844387076, 1.000000000000000000, 0.8660254037844387076, 1.000000000000000000, 0.8660254037844387076, 1.000000000000000000, 0.8660254037844387076, 1.000000000000000000, 0.8660254037844387076, 1.000000000000000000, 0.8660254037844387076, 1.000000000000000000, 0.8660254037844387076, 1.000000000000000000, 0.8660254037844387076, 1.000000000000000000, 0.8660254037844387076, 1.000000000000000000, 0.8660254037844387076, 1.000000000000000000, 0.8660254037844387076, 1.000000000000000000, 0.8660254037844387076, 1.000000000000000000, 0.8660254037844387076, 1.000000000000000000, 0.8660254037844387076, 1.000000000000000000, 0.8660254037844387076, 1.000000000000000000, 0.8660254037844387076, 1.000000000000000000, 0.8660254037844387076, 1.000000000000000000, 0.8660254037844387076, 1.000000000000000000, 0.8660254037844387076, 1.000000000000000000, 0.8660254037844387076, 1.000000000000000000, 0.8660254037844387076, 1.000000000000000000, 0.8660254037844387076, 1.000000000000000000, 0.8660254037844387076, 1.000000000000000000, 0.8660254037844387076, 1.000000000000000000, 0.8660254037844387076, 1.000000000000000000, 0.8660254037844387076, 1.000000000000000000, 0.8660254037844387076, 1.000000000000000000, 0.8660254037844387076, 1.000000000000000000, 0.8660254037844387076, 1.000000000000000000, 0.8660254037844387076, 1.000000000000000000, 0.8660254037844387076, 1.000000000000000000, 0.8660254037844387076, 1.000000000000000000, 0.8660254037844387076, 1.000000000000000000, 0.8660254037844387076, 1.000000000000000000, 0.8660254037844387076, 1.000000000000000000, 0.8660254037844387076, 1.000000000000000000, 0.8660254037844387076, 1.000000000000000000, 0.8660254037844387076, 1.000000000000000000, 0.8660254037844387076, 1.000000000000000000, 0.8660254037844387076, 1.000000000000000000, 0.8660254037844387076, 1.000000000000000000, 0.8660254037844387076, 1.000000000000000000, 0.8660254037844387076, 1.000000000000000000, 0.8660254037844387076, 1.000000000000000000, 0.8660254037844387076, 1.000000000000000000, 0.8660254037844387076, 1.000000000000000000, 0.8660254037844387076, 1.000000000000000000, 0.8660254037844387076, 1.000000000000000000, 0.8660254037844387076, 1.000000000000000000, 0.8660254037844387076, 1.000000000000000000, 0.8660254037844387076, 1.000000000000000000, 0.8660254037844387076, 1.000000000000000000, 0.8660254037844387076, 1.000000000000000000, 0.8660254037844387076, 1.000000000000000000, 0.8660254037844387076, 1.000000000000000000, 0.8660254037844387076, 1.000000000000000000, 0.8660254037844387076, 1.000000000000000000, 0.8660254037844387076, 1.000000000000000000, 0.8660254037844387076, 1.000000000000000000, 0.8660254037844387076, 1.000000000000000000, 0.8660254037844387076, 1.000000000000000000, 0.8660254037844387076, 1.000000000000000000, 0.8660254037844387076, 1.000000000000000000, 0.8660254037844387076, 1.000000000000000000, 0.8660254037844387076, 1.000000000000000000, 0.8660254037844387076, 1.000000000000000000, 0.8660254037844387076, 1.000000000000000000, 0.8660254037844387076, 1.000000000000000000, 0.8660254037844387076, 1.000000000000000000, 0.8660254037844387076, 1.000000000000000000, 0.8660254037844387076, 1.000000000000000000, 0.8660254037844387076, 1.000000000000000000, 0.8660254037844387076, 1.000000000000000000, 0.8660254037844387076, 1.000000000000000000, 0.8660254037844387076, 1.000000000000000000, 0.8660254037844387076, 1.000000000000000000, 0.8660254037844387076, 1.000000000000000000, 0.8660254037844387076, 1.000000000000000000, 0.8660254037844387076, 1.000000000000000000, 0.8660254037844387076, 1.000000000000000000, 0.8660254037844387076, 1.000000000000000000, 0.8660254037844387076, 1.000000000000000000, 0.8660254037844387076, 1.000000000000000000, 0.8660254037844387076, 1.000000000000000000, 0.8660254037844387076, 1.000000000000000000, 0.8660254037844387076, 1.000000000000000000, 0.8660254037844387076, 1.000000000000000000, 0.8660254037844387076, 1.000000000000000000, 0.8660254037844387076, 1.000000000000000000, 0.8660254037844387076, 1.000000000000000000, 0.8660254037844387076, 1.000000000000000000, 0.8660254037844387076, 1.000000000000000000, 0.8660254037844387076, 1.000000000000000000, 0.8660254037844387076, 1.000000000000000000, 0.8660254037844387076, 1.000000000000000000, 0.8660254037844387076, 1.000000000000000000, 0.8660254037844387076, 1.000000000000000000, 0.8660254037844387076, 1.000000000000000000, 0.8660254037844387076, 1.000000000000000000, 0.8660254037844387076, 1.000000000000000000, 0.8660254037844387076, 1.000000000000000000, 0.8660254037844387076, 1.000000000000000000, 0.8660254037844387076, 1.000000000000000000, 0.8660254037844387076, 1.000000000000000000, 0.8660254037844387076, 1.000000000000000000, 0.8660254037844387076, 1.000000000000000000, 0.8660254037844387076, 1.000000000000000000, 0.8660254037844387076, 1.000000000000000000, 0.8660254037844387076, 1.000000000000000000, 0.8660254037844387076, 1.000000000000000000, 0.8660254037844387076, 1.000000000000000000, 0.8660254037844387076, 1.000000000000000000, 0.8660254037844387076, 1.000000000000000000, 0.8660254037844387076, 1.000000000000000000, 0.8660254037844387076, 1.000000000000000000, 0.8660254037844387076, 1.000000000000000000, 0.8660254037844387076, 1.000000000000000000, 0.8660254037844387076, 1.000000000000000000, 0.8660254037844387076, 1.000000000000000000, 0.8660254037844387076, 1.000000000000000000, 0.8660254037844387076, 1.000000000000000000, 0.8660254037844387076, 1.000000000000000000, 0.8660254037844387076, 1.000000000000000000, 0.8660254037844387076, 1.000000000000000000, 0.8660254037844387076, 1.000000000000000000, 0.8660254037844387076, 1.000000000000000000, 0.8660254037844387076, 1.000000000000000000, 0.8660254037844387076, 1.000000000000000000, 0.8660254037844387076, 1.000000000000000000, 0.8660254037844387076, 1.000000000000000000, 0.8660254037844387076, 1.000000000000000000, 0.8660254037844387076, 1.000000000000000000, 0.8660254037844387076, 1.000000000000000000, 0.8660254037844387076, 1.000000000000000000, 0.8660254037844387076, 1.000000000000000000, 0.8660254037844387076, 1.000000000000000000, 0.8660254037844387076, 1.000000000000000000, 0.8660254037844387076, 1.000000000000000000, 0.8660254037844387076, 1.000000000000000000, 0.8660254037844387076, 1.000000000000000000, 0.8660254037844387076, 1.000000000000000000, 0.8660254037844387076, 1.000000000000000000, 0.8660254037844387076, 1.000000000000000000, 0.8660254037844387076, 1.000000000000000000, 0.8660254037844387076, 1.000000000000000000, 0.8660254037844387076, 1.000000000000000000, 0.8660254037844387076, 1.000000000000000000, 0.8660254037844387076, 1.000000000000000000, 0.8660254037844387076, 1.000000000000000000, 0.8660254037844387076, 1.000000000000000000, 0.8660254037844387076, 1.000000000000000000, 0.8660254037844387076, 1.000000000000000000, 0.8660254037844387076, 1.000000000000000000, 0.8660254037844387076, 1.000000000000000000, 0.8660254037844387076, 1.000000000000000000, 0.8660254037844387076, 1.000000000000000000, 0.8660254037844387076, 1.000000000000000000, 0.8660254037844387076, 1.000000000000000000, 0.8660254037844387076, 1.000000000000000000, 0.8660254037844387076, 1.000000000000000000, 0.8660254037844387076, 1.000000000000000000, 0.8660254037844387076, 1.000000000000000000, 0.8660254037844387076, 1.000000000000000000, 0.8660254037844387076, 1.000000000000000000, 0.8660254037844387076, 1.000000000000000000, 0.8660254037844387076, 1.000000000000000000, 0.8660254037844387076, 1.000000000000000000, 0.8660254037844387076, 1.000000000000000000, 0.8660254037844387076, 1.000000000000000000, 0.8660254037844387076, 1.000000000000000000, 0.8660254037844387076, 1.000000000000000000, 0.8660254037844387076, 1.000000000000000000, 0.8660254037844387076, 1.000000000000000000, 0.8660254037844387076, 1.000000000000000000, 0.8660254037844387076, 1.000000000000000000, 0.8660254037844387076, 1.000000000000000000, 0.8660254037844387076, 1.000000000000000000, 0.8660254037844387076, 1.000000000000000000, 0.8660254037844387076, 1.000000000000000000, 0.8660254037844387076, 1.000000000000000000, 0.8660254037844387076, 1.000000000000000000, 0.8660254037844387076, 1.000000000000000000, 0.8660254037844387076, 1.000000000000000000, 0.8660254037844387076, 1.000000000000000000, 0.8660254037844387076, 1.000000000000000000, 0.8660254037844387076, 1.000000000000000000, 0.8660254037844387076, 1.000000000000000000, 0.8660254037844387076, 1.000000000000000000, 0.8660254037844387076, 1.000000000000000000, 0.8660254037844387076, 1.000000000000000000, 0.8660254037844387076, 1.000000000000000000, 0.8660254037844387076, 1.000000000000000000, 0.8660254037844387076, 1.000000000000000000, 0.8660254037844387076, 1.000000000000000000, 0.8660254037844387076, 1.000000000000000000, 0.8660254037844387076, 1.000000000000000000, 0.8660254037844387076, 1.000000000000000000, 0.8660254037844387076, 1.000000000000000000, 0.8660254037844387076, 1.000000000000000000, 0.8660254037844387076, 1.000000000000000000, 0.8660254037844387076, 1.000000000000000000, 0.8660254037844387076, 1.000000000000000000, 0.8660254037844387076, 1.000000000000000000, 0.8660254037844387076, 1.000000000000000000, 0.8660254037844387076, 1.000000000000000000, 0.8660254037844387076, 1.000000000000000000, 0.8660254037844387076, 1.000000000000000000, 0.8660254037844387076, 1.000000000000000000, 0.8660254037844387076, 1.000000000000000000, 0.8660254037844387076, 1.000000000000000000, 0.8660254037844387076, 1.000000000000000000, 0.8660254037844387076, 1.000000000000000000, 0.8660254037844387076, 1.000000000000000000, 0.8660254037844387076, 1.000000000000000000, 0.8660254037844387076, 1.000000000000000000, 0.8660254037844387076, 1.000000000000000000, 0.8660254037844387076, 1.000000000000000000, 0.8660254037844387076, 1.000000000000000000, 0.8660254037844387076, 1.000000000000000000, 0.8660254037844387076, 1.000000000000000000, 0.8660254037844387076, 1.000000000000000000, 0.8660254037844387076, 1.000000000000000000, 0.8660254037844387076, 1.000000000000000000, 0.8660254037844387076, 1.000000000000000000, 0.8660254037844387076, 1.000000000000000000, 0.8660254037844387076, 1.000000000000000000, 0.8660254037844387076, 1.000000000000000000, 0.8660254037844387076, 1.000000000000000000, 0.8660254037844387076, 1.000000000000000000, 0.8660254037844387076, 1.000000000000000000, 0.8660254037844387076, 1.000000000000000000, 0.8660254037844387076, 1.000000000000000000, 0.8660254037844387076, 1.000000000000000000, 0.8660254037844387076, 1.000000000000000000, 0.8660254037844387076, 1.000000000000000000, 0.8660254037844387076, 1.000000000000000000, 0.8660254037844387076, 1.000000000000000000, 0.8660254037844387076, 1.000000000000000000, 0.8660254037844387076, 1.000000000000000000, 0.8660254037844387076, 1.000000000000000000, 0.8660254037844387076, 1.000000000000000000, 0.8660254037844387076, 1.000000000000000000, 0.8660254037844387076, 1.000000000000000000, 0.8660254037844387076, 1.000000000000000000, 0.8660254037844387076, 1.000000000000000000, 0.8660254037844387076, 1.000000000000000000, 0.8660254037844387076, 1.000000000000000000, 0.8660254037844387076, 1.000000000000000000, 0.8660254037844387076, 1.000000000000000000, 0.8660254037844387076, 1.000000000000000000, 0.8660254037844387076, 1.000000000000000000, 0.8660254037844387076, 1.000000000000000000, 0.8660254037844387076, 1.000000000000000000, 0.8660254037844387076, 1.000000000000000000, 0.8660254037844387076, 1.000000000000000000, 0.8660254037844387076, 1.000000000000000000, 0.8660254037844387076, 1.000000000000000000, 0.8660254037844387076, 1.000000000000000000, 0.8660254037844387076, 1.000000000000000000, 0.8660254037844387076, 1.000000000000000000, 0.8660254037844387076, 1.000000000000000000, 0.8660254037844387076, 1.000000000000000000, 0.8660254037844387076, 1.000000000000000000, 0.8660254037844387076, 1.000000000000000000, 0.8660254037844387076, 1.000000000000000000, 0.8660254037844387076, 1.000000000000000000, 0.8660254037844387076, 1.000000000000000000, 0.8660254037844387076, 1.000000000000000000, 0.8660254037844387076, 1.000000000000000000, 0.8660254037844387076, 1.000000000000000000, 0.8660254037844387076, 1.000000000000000000, 0.8660254037844387076, 1.000000000000000000, 0.8660254037844387076, 1.000000000000000000, 0.8660254037844387076, 1.000000000000000000, 0.8660254037844387076, 1.000000000000000000, 0.8660254037844387076, 1.000000000000000000, 0.8660254037844387076, 1.000000000000000000, 0.8660254037844387076, 1.000000000000000000, 0.8660254037844387076, 1.000000000000000000, 0.8660254037844387076, 1.000000000000000000, 0.8660254037844387076, 1.000000000000000000, 0.8660254037844387076, 1.000000000000000000, 0.8660254037844387076, 1.000000000000000000, 0.8660254037844387076, 1.000000000000000000, 0.8660254037844387076, 1.000000000000000000, 0.8660254037844387076, 1.000000000000000000, 0.8660254037844387076, 1.000000000000000000, 0.8660254037844387076, 1.000000000000000000, 0.8660254037844387076, 1.000000000000000000, 0.8660254037844387076, 1.000000000000000000, 0.8660254037844387076, 1.000000000000000000, 0.8660254037844387076, 1.000000000000000000, 0.8660254037844387076, 1.000000000000000000, 0.8660254037844387076, 1.000000000000000000, 0.8660254037844387076, 1.000000000000000000, 0.8660254037844387076, 1.000000000000000000, 0.8660254037844387076, 1.000000000000000000, 0.8660254037844387076, 1.000000000000000000, 0.8660254037844387076, 1.000000000000000000, 0.8660254037844387076, 1.000000000000000000, 0.8660254037844387076, 1.000000000000000000, 0.8660254037844387076, 1.000000000000000000, 0.8660254037844387076, 1.000000000000000000, 0.8660254037844387076, 1.000000000000000000, 0.8660254037844387076, 1.000000000000000000, 0.8660254037844387076, 1.000000000000000000, 0.8660254037844387076, 1.000000000000000000, 0.8660254037844387076, 1.000000000000000000, 0.8660254037844387076, 1.000000000000000000, 0.8660254037844387076, 1.000000000000000000, 0.8660254037844387076, 1.000000000000000000, 0.8660254037844387076, 1.000000000000000000, 0.8660254037844387076, 1.000000000000000000, 0.8660254037844387076, 1.000000000000000000, 0.8660254037844387076, 1.000000000000000000, 0.8660254037844387076, 1.000000000000000000, 0.8660254037844387076, 1.000000000000000000, 0.8660254037844387076, 1.000000000000000000, 0.8660254037844387076, 1.000000000000000000, 0.8660254037844387076, 1.000000000000000000, 0.8660254037844387076, 1.000000000000000000, 0.8660254037844387076, 1.000000000000000000, 0.8660254037844387076, 1.000000000000000000, 0.8660254037844387076, 1.000000000000000000, 0.8660254037844387076, 1.000000000000000000, 0.8660254037844387076, 1.000000000000000000, 0.8660254037844387076, 1.000000000000000000, 0.8660254037844387076, 1.000000000000000000, 0.8660254037844387076, 1.000000000000000000, 0.8660254037844387076, 1.000000000000000000, 0.8660254037844387076, 1.000000000000000000, 0.8660254037844387076, 1.000000000000000000, 0.8660254037844387076, 1.000000000000000000, 0.8660254037844387076, 1.000000000000000000, 0.8660254037844387076, 1.000000000000000000, 0.8660254037844387076, 1.000000000000000000, 0.8660254037844387076, 1.000000000000000000, 0.8660254037844387076, 1.000000000000000000, 0.8660254037844387076, 1.000000000000000000, 0.8660254037844387076, 1.000000000000000000, 0.8660254037844387076, 1.000000000000000000, 0.8660254037844387076, 1.000000000000000000, 0.8660254037844387076, 1.000000000000000000, 0.8660254037844387076, 1.000000000000000000, 0.8660254037844387076, 1.000000000000000000, 0.8660254037844387076, 1.000000000000000000, 0.8660254037844387076, 1.000000000000000000, 0.8660254037844387076, 1.000000000000000000, 0.8660254037844387076, 1.000000000000000000, 0.8660254037844387076, 1.000000000000000000, 0.8660254037844387076, 1.000000000000000000, 0.8660254037844387076, 1.000000000000000000, 0.8660254037844387076, 1.000000000000000000, 0.8660254037844387076, 1.000000000000000000, 0.8660254037844387076, 1.000000000000000000, 0.8660254037844387076, 1.000000000000000000, 0.8660254037844387076, 1.000000000000000000, 0.8660254037844387076, 1.000000000000000000, 0.8660254037844387076, 1.000000000000000000, 0.8660254037844387076, 1.000000000000000000, 0.8660254037844387076, 1.000000000000000000, 0.8660254037844387076, 1.000000000000000000, 0.8660254037844387076, 1.000000000000000000, 0.8660254037844387076, 1.000000000000000000, 0.8660254037844387076, 1.000000000000000000, 0.8660254037844387076, 1.000000000000000000, 0.8660254037844387076, 1.000000000000000000, 0.8660254037844387076, 1.000000000000000000, 0.8660254037844387076, 1.000000000000000000, 0.8660254037844387076, 1.000000000000000000, 0.8660254037844387076, 1.000000000000000000, 0.8660254037844387076, 1.000000000000000000, 0.8660254037844387076, 1.000000000000000000, 0.8660254037844387076, 1.000000000000000000, 0.8660254037844387076, 1.000000000000000000, 0.8660254037844387076, 1.000000000000000000, 0.8660254037844387076, 1.000000000000000000, 0.8660254037844387076, 1.000000000000000000, 0.8660254037844387076, 1.000000000000000000, 0.8660254037844387076, 1.000000000000000000, 0.8660254037844387076, 1.000000000000000000, 0.8660254037844387076, 1.000000000000000000, 0.8660254037844387076, 1.000000000000000000, 0.8660254037844387076, 1.000000000000000000, 0.8660254037844387076, 1.000000000000000000, 0.8660254037844387076, 1.000000000000000000, 0.8660254037844387076, 1.000000000000000000, 0.8660254037844387076, 1.000000000000000000, 0.8660254037844387076, 1.000000000000000000, 0.8660254037844387076, 1.000000000000000000, 0.8660254037844387076, 1.000000000000000000, 0.8660254037844387076, 1.000000000000000000, 0.8660254037844387076, 1.000000000000000000, 0.8660254037844387076, 1.000000000000000000, 0.8660254037844387076, 1.000000000000000000, 0.8660254037844387076, 1.000000000000000000, 0.8660254037844387076, 1.000000000000000000, 0.8660254037844387076, 1.000000000000000000, 0.8660254037844387076, 1.000000000000000000, 0.8660254037844387076, 1.000000000000000000, 0.8660254037844387076, 1.000000000000000000, 0.8660254037844387076, 1.000000000000000000, 0.8660254037844387076, 1.000000000000000000, 0.8660254037844387076, 1.000000000000000000, 0.8660254037844387076, 1.000000000000000000, 0.8660254037844387076, 1.000000000000000000, 0.8660254037844387076, 1.000000000000000000, 0.8660254037844387076, 1.000000000000000000, 0.8660254037844387076, 1.000000000000000000, 0.8660254037844387076, 1.000000000000000000, 0.8660254037844387076, 1.000000000000000000, 0.8660254037844387076, 1.000000000000000000, 0.8660254037844387076, 1.000000000000000000, 0.8660254037844387076, 1.000000000000000000, 0.8660254037844387076, 1.000000000000000000, 0.8660254037844387076, 1.000000000000000000, 0.8660254037844387076, 1.000000000000000000, 0.8660254037844387076, 1.000000000000000000, 0.8660254037844387076, 1.000000000000000000, 0.8660254037844387076, 1.000000000000000000, 0.8660254037844387076, 1.000000000000000000, 0.8660254037844387076, 1.000000000000000000, 0.8660254037844387076, 1.000000000000000000, 0.8660254037844387076, 1.000000000000000000, 0.8660254037844387076, 1.000000000000000000, 0.8660254037844387076, 1.000000000000000000, 0.8660254037844387076, 1.000000000000000000, 0.8660254037844387076, 1.000000000000000000, 0.8660254037844387076, 1.000000000000000000, 0.8660254037844387076, 1.000000000000000000, 0.8660254037844387076, 1.000000000000000000, 0.8660254037844387076, 1.000000000000000000, 0.8660254037844387076, 1.000000000000000000, 0.8660254037844387076, 1.000000000000000000, 0.8660254037844387076, 1.000000000000000000, 0.8660254037844387076, 1.000000000000000000, 0.8660254037844387076, 1.000000000000000000, 0.8660254037844387076, 1.000000000000000000, 0.8660254037844387076, 1.000000000000000000, 0.8660254037844387076, 1.000000000000000000, 0.8660254037844387076, 1.000000000000000000, 0.8660254037844387076, 1.000000000000000000, 0.8660254037844387076, 1.000000000000000000, 0.8660254037844387076, 1.000000000000000000, 0.8660254037844387076, 1.000000000000000000, 0.8660254037844387076, 1.000000000000000000, 0.8660254037844387076, 1.000000000000000000, 0.8660254037844387076, 1.000000000000000000, 0.8660254037844387076, 1.000000000000000000, 0.8660254037844387076, 1.000000000000000000, 0.8660254037844387076, 1.000000000000000000, 0.8660254037844387076, 1.000000000000000000, 0.8660254037844387076, 1.000000000000000000, 0.8660254037844387076, 1.000000000000000000, 0.8660254037844387076, 1.000000000000000000, 0.8660254037844387076, 1.000000000000000000, 0.8660254037844387076, 1.000000000000000000, 0.8660254037844387076, 1.000000000000000000, 0.8660254037844387076, 1.000000000000000000, 0.8660254037844387076, 1.000000000000000000, 0.8660254037844387076, 1.000000000000000000, 0.8660254037844387076, 1.000000000000000000, 0.8660254037844387076, 1.000000000000000000, 0.8660254037844387076, 1.000000000000000000, 0.8660254037844387076, 1.000000000000000000, 0.8660254037844387076, 1.000000000000000000, 0.8660254037844387076, 1.000000000000000000, 0.8660254037844387076, 1.000000000000000000, 0.8660254037844387076, 1.000000000000000000, 0.8660254037844387076, 1.000000000000000000, 0.8660254037844387076, 1.000000000000000000, 0.8660254037844387076, 1.000000000000000000, 0.8660254037844387076, 1.000000000000000000, 0.8660254037844387076, 1.000000000000000000, 0.8660254037844387076, 1.000000000000000000, 0.8660254037844387076, 1.000000000000000000, 0.8660254037844387076, 1.000000000000000000, 0.8660254037844387076, 1.000000000000000000, 0.8660254037844387076, 1.000000000000000000, 0.8660254037844387076, 1.000000000000000000, 0.8660254037844387076, 1.000000000000000000, 0.8660254037844387076, 1.000000000000000000, 0.8660254037844387076, 1.000000000000000000, 0.8660254037844387076, 1.000000000000000000, 0.8660254037844387076, 1.000000000000000000, 0.8660254037844387076, 1.000000000000000000, 0.8660254037844387076, 1.000000000000000000, 0.8660254037844387076, 1.000000000000000000, 0.8660254037844387076, 1.000000000000000000, 0.8660254037844387076, 1.000000000000000000, 0.8660254037844387076, 1.000000000000000000, 0.8660254037844387076, 1.000000000000000000, 0.8660254037844387076, 1.000000000000000000, 0.8660254037844387076, 1.000000000000000000, 0.8660254037844387076, 1.000000000000000000, 0.8660254037844387076, 1.000000000000000000, 0.8660254037844387076, 1.000000000000000000, 0.8660254037844387076, 1.000000000000000000, 0.8660254037844387076, 1.000000000000000000, 0.8660254037844387076, 1.000000000000000000, 0.8660254037844387076, 1.000000000000000000, 0.8660254037844387076, 1.000000000000000000, 0.8660254037844387076, 1.000000000000000000, 0.8660254037844387076, 1.000000000000000000, 0.8660254037844387076, 1.000000000000000000, 0.8660254037844387076, 1.000000000000000000, 0.8660254037844387076, 1.000000000000000000, 0.8660254037844387076, 1.000000000000000000, 0.8660254037844387076, 1.000000000000000000, 0.8660254037844387076, 1.000000000000000000, 0.8660254037844387076, 1.000000000000000000, 0.8660254037844387076, 1.000000000000000000, 0.8660254037844387076, 1.000000000000000000, 0.8660254037844387076, 1.000000000000000000, 0.8660254037844387076, 1.000000000000000000, 0.8660254037844387076, 1.000000000000000000, 0.8660254037844387076, 1.000000000000000000, 0.8660254037844387076, 1.000000000000000000, 0.8660254037844387076, 1.000000000000000000, 0.8660254037844387076, 1.000000000000000000, 0.8660254037844387076, 1.000000000000000000, 0.8660254037844387076, 1.000000000000000000, 0.8660254037844387076, 1.000000000000000000, 0.8660254037844387076, 1.000000000000000000, 0.8660254037844387076, 1.000000000000000000, 0.8660254037844387076, 1.000000000000000000, 0.8660254037844387076, 1.000000000000000000, 0.8660254037844387076, 1.000000000000000000, 0.8660254037844387076, 1.000000000000000000, 0.8660254037844387076, 1.000000000000000000, 0.8660254037844387076, 1.000000000000000000, 0.8660254037844387076, 1.000000000000000000, 0.8660254037844387076, 1.000000000000000000, 0.8660254037844387076, 1.000000000000000000, 0.8660254037844387076, 1.000000000000000000, 0.8660254037844387076, 1.000000000000000000, 0.8660254037844387076, 1.000000000000000000, 0.8660254037844387076, 1.000000000000000000, 0.8660254037844387076, 1.000000000000000000, 0.8660254037844387076, 1.000000000000000000, 0.8660254037844387076, 1.000000000000000000, 0.8660254037844387076, 1.000000000000000000, 0.8660254037844387076, 1.000000000000000000, 0.8660254037844387076, 1.000000000000000000, 0.8660254037844387076, 1.000000000000000000, 0.8660254037844387076, 1.000000000000000000, 0.8660254037844387076, 1.000000000000000000, 0.8660254037844387076, 1.000000000000000000, 0.8660254037844387076, 1.000000000000000000, 0.8660254037844387076, 1.000000000000000000, 0.8660254037844387076, 1.000000000000000000, 0.8660254037844387076, 1.000000000000000000, 0.8660254037844387076, 1.000000000000000000, 0.8660254037844387076, 1.000000000000000000, 0.8660254037844387076, 1.000000000000000000, 0.8660254037844387076, 1.000000000000000000, 0.8660254037844387076, 1.000000000000000000, 0.8660254037844387076, 1.000000000000000000, 0.8660254037844387076, 1.000000000000000000, 0.8660254037844387076, 1.000000000000000000, 0.8660254037844387076, 1.000000000000000000, 0.8660254037844387076, 1.000000000000000000, 0.8660254037844387076, 1.000000000000000000, 0.8660254037844387076, 1.000000000000000000, 0.8660254037844387076, 1.000000000000000000, 0.8660254037844387076, 1.000000000000000000, 0.8660254037844387076, 1.000000000000000000, 0.8660254037844387076, 1.000000000000000000, 0.8660254037844387076, 1.000000000000000000, 0.8660254037844387076, 1.000000000000000000, 0.8660254037844387076, 1.000000000000000000, 0.8660254037844387076, 1.000000000000000000, 0.8660254037844387076, 1.000000000000000000, 0.8660254037844387076, 1.000000000000000000, 0.8660254037844387076, 1.000000000000000000, 0.8660254037844387076, 1.000000000000000000, 0.8660254037844387076, 1.000000000000000000, 0.8660254037844387076, 1.000000000000000000, 0.8660254037844387076, 1.000000000000000000, 0.8660254037844387076, 1.000000000000000000, 0.8660254037844387076, 1.000000000000000000, 0.8660254037844387076, 1.000000000000000000, 0.8660254037844387076, 1.000000000000000000, 0.8660254037844387076, 1.000000000000000000, 0.8660254037844387076, 1.000000000000000000, 0.8660254037844387076, 1.000000000000000000, 0.8660254037844387076, 1.000000000000000000, 0.8660254037844387076, 1.000000000000000000, 0.8660254037844387076, 1.000000000000000000, 0.8660254037844387076, 1.000000000000000000, 0.8660254037844387076, 1.000000000000000000, 0.8660254037844387076, 1.000000000000000000, 0.8660254037844387076, 1.000000000000000000, 0.8660254037844387076, 1.000000000000000000, 0.8660254037844387076, 1.000000000000000000, 0.8660254037844387076, 1.000000000000000000, 0.8660254037844387076, 1.000000000000000000, 0.8660254037844387076, 1.000000000000000000, 0.8660254037844387076, 1.000000000000000000, 0.8660254037844387076, 1.000000000000000000, 0.8660254037844387076, 1.000000000000000000, 0.8660254037844387076, 1.000000000000000000, 0.8660254037844387076, 1.000000000000000000, 0.8660254037844387076, 1.000000000000000000, 0.8660254037844387076, 1.000000000000000000, 0.8660254037844387076, 1.000000000000000000, 0.8660254037844387076, 1.000000000000000000, 0.8660254037844387076, 1.000000000000000000, 0.8660254037844387076, 1.000000000000000000, 0.8660254037844387076, 1.000000000000000000, 0.8660254037844387076, 1.000000000000000000, 0.8660254037844387076, 1.000000000000000000, 0.8660254037844387076, 1.000000000000000000, 0.8660254037844387076, 1.000000000000000000, 0.8660254037844387076, 1.000000000000000000, 0.8660254037844387076, 1.000000000000000000, 0.8660254037844387076, 1.000000000000000000, 0.8660254037844387076, 1.000000000000000000, 0.8660254037844387076, 1.000000000000000000, 0.8660254037844387076, 1.000000000000000000, 0.8660254037844387076, 1.000000000000000000, 0.8660254037844387076, 1.000000000000000000, 0.8660254037844387076, 1.000000000000000000, 0.8660254037844387076, 1.000000000000000000, 0.8660254037844387076, 1.000000000000000000, 0.8660254037844387076, 1.000000000000000000, 0.8660254037844387076, 1.000000000000000000, 0.8660254037844387076, 1.000000000000000000, 0.8660254037844387076, 1.000000000000000000, 0.8660254037844387076, 1.000000000000000000, 0.8660254037844387076, 1.000000000000000000, 0.8660254037844387076, 1.000000000000000000, 0.8660254037844387076, 1.000000000000000000, 0.8660254037844387076, 1.000000000000000000, 0.8660254037844387076, 1.000000000000000000, 0.8660254037844387076, 1.000000000000000000, 0.8660254037844387076, 1.000000000000000000, 0.8660254037844387076, 1.000000000000000000, 0.8660254037844387076, 1.000000000000000000, 0.8660254037844387076, 1.000000000000000000, 0.8660254037844387076, 1.000000000000000000, 0.8660254037844387076, 1.000000000000000000, 0.8660254037844387076, 1.000000000000000000, 0.8660254037844387076, 1.000000000000000000, 0.8660254037844387076, 1.000000000000000000, 0.8660254037844387076, 1.000000000000000000, 0.8660254037844387076, 1.000000000000000000, 0.8660254037844387076, 1.000000000000000000, 0.8660254037844387076, 1.000000000000000000, 0.8660254037844387076, 1.000000000000000000),
 ( 1.000000000000000000, 0.8660254037844387076, 1.000000000000000000, 0.8660254037844387076, 1.000000000000000000, 0.8660254037844387076, 1.000000000000000000, 0.8660254037844387076, 1.000000000000000000, 0.8660254037844387076, 1.000000000000000000, 0.8660254037844387076, 1.000000000000000000, 0.8660254037844387076, 1.000000000000000000, 0.8660254037844387076, 1.000000000000000000, 0.8660254037844387076, 1.000000000000000000, 0.8660254037844387076, 1.000000000000000000, 0.8660254037844387076, 1.000000000000000000, 0.8660254037844387076, 1.000000000000000000, 0.8660254037844387076, 1.000000000000000000, 0.8660254037844387076, 1.000000000000000000, 0.8660254037844387076, 1.000000000000000000, 0.8660254037844387076, 1.000000000000000000, 0.8660254037844387076, 1.000000000000000000, 0.8660254037844387076, 1.000000000000000000, 0.8660254037844387076, 1.000000000000000000, 0.8660254037844387076, 1.000000000000000000, 0.8660254037844387076, 1.000000000000000000, 0.8660254037844387076, 1.000000000000000000, 0.8660254037844387076, 1.000000000000000000, 0.8660254037844387076, 1.000000000000000000, 0.8660254037844387076, 1.000000000000000000, 0.8660254037844387076, 1.000000000000000000, 0.8660254037844387076, 1.000000000000000000, 0.8660254037844387076, 1.000000000000000000, 0.8660254037844387076, 1.000000000000000000, 0.8660254037844387076, 1.000000000000000000, 0.8660254037844387076, 1.000000000000000000, 0.8660254037844387076, 1.000000000000000000, 0.8660254037844387076, 1.000000000000000000, 0.8660254037844387076, 1.000000000000000000, 0.8660254037844387076, 1.000000000000000000, 0.8660254037844387076, 1.000000000000000000, 0.8660254037844387076, 1.000000000000000000, 0.8660254037844387076, 1.000000000000000000, 0.8660254037844387076, 1.000000000000000000, 0.8660254037844387076, 1.000000000000000000, 0.8660254037844387076, 1.000000000000000000, 0.8660254037844387076, 1.000000000000000000, 0.8660254037844387076, 1.000000000000000000, 0.8660254037844387076, 1.000000000000000000, 0.8660254037844387076, 1.000000000000000000, 0.8660254037844387076, 1.000000000000000000, 0.8660254037844387076, 1.000000000000000000, 0.8660254037844387076, 1.000000000000000000, 0.8660254037844387076, 1.000000000000000000, 0.8660254037844387076, 1.000000000000000000, 0.8660254037844387076, 1.000000000000000000, 0.8660254037844387076, 1.000000000000000000, 0.8660254037844387076, 1.000000000000000000, 0.8660254037844387076, 1.000000000000000000, 0.8660254037844387076, 1.000000000000000000, 0.8660254037844387076, 1.000000000000000000, 0.8660254037844387076, 1.000000000000000000, 0.8660254037844387076, 1.000000000000000000, 0.8660254037844387076, 1.000000000000000000, 0.8660254037844387076, 1.000000000000000000, 0.8660254037844387076, 1.000000000000000000, 0.8660254037844387076, 1.000000000000000000, 0.8660254037844387076, 1.000000000000000000, 0.8660254037844387076, 1.000000000000000000, 0.8660254037844387076, 1.000000000000000000, 0.8660254037844387076, 1.000000000000000000, 0.8660254037844387076, 1.000000000000000000, 0.8660254037844387076, 1.000000000000000000, 0.8660254037844387076, 1.000000000000000000, 0.8660254037844387076, 1.000000000000000000, 0.8660254037844387076, 1.000000000000000000, 0.8660254037844387076, 1.000000000000000000, 0.8660254037844387076, 1.000000000000000000, 0.8660254037844387076, 1.000000000000000000, 0.8660254037844387076, 1.000000000000000000, 0.8660254037844387076, 1.000000000000000000, 0.8660254037844387076, 1.000000000000000000, 0.8660254037844387076, 1.000000000000000000, 0.8660254037844387076, 1.000000000000000000, 0.8660254037844387076, 1.000000000000000000, 0.8660254037844387076, 1.000000000000000000, 0.8660254037844387076, 1.000000000000000000, 0.8660254037844387076, 1.000000000000000000, 0.8660254037844387076, 1.000000000000000000, 0.8660254037844387076, 1.000000000000000000, 0.8660254037844387076, 1.000000000000000000, 0.8660254037844387076, 1.000000000000000000, 0.8660254037844387076, 1.000000000000000000, 0.8660254037844387076, 1.000000000000000000, 0.8660254037844387076, 1.000000000000000000, 0.8660254037844387076, 1.000000000000000000, 0.8660254037844387076, 1.000000000000000000, 0.8660254037844387076, 1.000000000000000000, 0.8660254037844387076, 1.000000000000000000, 0.8660254037844387076, 1.000000000000000000, 0.8660254037844387076, 1.000000000000000000, 0.8660254037844387076, 1.000000000000000000, 0.8660254037844387076, 1.000000000000000000, 0.8660254037844387076, 1.000000000000000000, 0.8660254037844387076, 1.000000000000000000, 0.8660254037844387076, 1.000000000000000000, 0.8660254037844387076, 1.000000000000000000, 0.8660254037844387076, 1.000000000000000000, 0.8660254037844387076, 1.000000000000000000, 0.8660254037844387076, 1.000000000000000000, 0.8660254037844387076, 1.000000000000000000, 0.8660254037844387076, 1.000000000000000000, 0.8660254037844387076, 1.000000000000000000, 0.8660254037844387076, 1.000000000000000000, 0.8660254037844387076, 1.000000000000000000, 0.8660254037844387076, 1.000000000000000000, 0.8660254037844387076, 1.000000000000000000, 0.8660254037844387076, 1.000000000000000000, 0.8660254037844387076, 1.000000000000000000, 0.8660254037844387076, 1.000000000000000000, 0.8660254037844387076, 1.000000000000000000, 0.8660254037844387076, 1.000000000000000000, 0.8660254037844387076, 1.000000000000000000, 0.8660254037844387076, 1.000000000000000000, 0.8660254037844387076, 1.000000000000000000, 0.8660254037844387076, 1.000000000000000000, 0.8660254037844387076, 1.000000000000000000, 0.8660254037844387076, 1.000000000000000000, 0.8660254037844387076, 1.000000000000000000, 0.8660254037844387076, 1.000000000000000000, 0.8660254037844387076, 1.000000000000000000, 0.8660254037844387076, 1.000000000000000000, 0.8660254037844387076, 1.000000000000000000, 0.8660254037844387076, 1.000000000000000000, 0.8660254037844387076, 1.000000000000000000, 0.8660254037844387076, 1.000000000000000000, 0.8660254037844387076, 1.000000000000000000, 0.8660254037844387076, 1.000000000000000000, 0.8660254037844387076, 1.000000000000000000, 0.8660254037844387076, 1.000000000000000000, 0.8660254037844387076, 1.000000000000000000, 0.8660254037844387076, 1.000000000000000000, 0.8660254037844387076, 1.000000000000000000, 0.8660254037844387076, 1.000000000000000000, 0.8660254037844387076, 1.000000000000000000, 0.8660254037844387076, 1.000000000000000000, 0.8660254037844387076, 1.000000000000000000, 0.8660254037844387076, 1.000000000000000000, 0.8660254037844387076, 1.000000000000000000, 0.8660254037844387076, 1.000000000000000000, 0.8660254037844387076, 1.000000000000000000, 0.8660254037844387076, 1.000000000000000000, 0.8660254037844387076, 1.000000000000000000, 0.8660254037844387076, 1.000000000000000000, 0.8660254037844387076, 1.000000000000000000, 0.8660254037844387076, 1.000000000000000000, 0.8660254037844387076, 1.000000000000000000, 0.8660254037844387076, 1.000000000000000000, 0.8660254037844387076, 1.000000000000000000, 0.8660254037844387076, 1.000000000000000000, 0.8660254037844387076, 1.000000000000000000, 0.8660254037844387076, 1.000000000000000000, 0.8660254037844387076, 1.000000000000000000, 0.8660254037844387076, 1.000000000000000000, 0.8660254037844387076, 1.000000000000000000, 0.8660254037844387076, 1.000000000000000000, 0.8660254037844387076, 1.000000000000000000, 0.8660254037844387076, 1.000000000000000000, 0.8660254037844387076, 1.000000000000000000, 0.8660254037844387076, 1.000000000000000000, 0.8660254037844387076, 1.000000000000000000, 0.8660254037844387076, 1.000000000000000000, 0.8660254037844387076, 1.000000000000000000, 0.8660254037844387076, 1.000000000000000000, 0.8660254037844387076, 1.000000000000000000, 0.8660254037844387076, 1.000000000000000000, 0.8660254037844387076, 1.000000000000000000, 0.8660254037844387076, 1.000000000000000000, 0.8660254037844387076, 1.000000000000000000, 0.8660254037844387076, 1.000000000000000000, 0.8660254037844387076, 1.000000000000000000, 0.8660254037844387076, 1.000000000000000000, 0.8660254037844387076, 1.000000000000000000, 0.8660254037844387076, 1.000000000000000000, 0.8660254037844387076, 1.000000000000000000, 0.8660254037844387076, 1.000000000000000000, 0.8660254037844387076, 1.000000000000000000, 0.8660254037844387076, 1.000000000000000000, 0.8660254037844387076, 1.000000000000000000, 0.8660254037844387076, 1.000000000000000000, 0.8660254037844387076, 1.000000000000000000, 0.8660254037844387076, 1.000000000000000000, 0.8660254037844387076, 1.000000000000000000, 0.8660254037844387076, 1.000000000000000000, 0.8660254037844387076, 1.000000000000000000, 0.8660254037844387076, 1.000000000000000000, 0.8660254037844387076, 1.000000000000000000, 0.8660254037844387076, 1.000000000000000000, 0.8660254037844387076, 1.000000000000000000, 0.8660254037844387076, 1.000000000000000000, 0.8660254037844387076, 1.000000000000000000, 0.8660254037844387076, 1.000000000000000000, 0.8660254037844387076, 1.000000000000000000, 0.8660254037844387076, 1.000000000000000000, 0.8660254037844387076, 1.000000000000000000, 0.8660254037844387076, 1.000000000000000000, 0.8660254037844387076, 1.000000000000000000, 0.8660254037844387076, 1.000000000000000000, 0.8660254037844387076, 1.000000000000000000, 0.8660254037844387076, 1.000000000000000000, 0.8660254037844387076, 1.000000000000000000, 0.8660254037844387076, 1.000000000000000000, 0.8660254037844387076, 1.000000000000000000, 0.8660254037844387076, 1.000000000000000000, 0.8660254037844387076, 1.000000000000000000, 0.8660254037844387076, 1.000000000000000000, 0.8660254037844387076, 1.000000000000000000, 0.8660254037844387076, 1.000000000000000000, 0.8660254037844387076, 1.000000000000000000, 0.8660254037844387076, 1.000000000000000000, 0.8660254037844387076, 1.000000000000000000, 0.8660254037844387076, 1.000000000000000000, 0.8660254037844387076, 1.000000000000000000, 0.8660254037844387076, 1.000000000000000000, 0.8660254037844387076, 1.000000000000000000, 0.8660254037844387076, 1.000000000000000000, 0.8660254037844387076, 1.000000000000000000, 0.8660254037844387076, 1.000000000000000000, 0.8660254037844387076, 1.000000000000000000, 0.8660254037844387076, 1.000000000000000000, 0.8660254037844387076, 1.000000000000000000, 0.8660254037844387076, 1.000000000000000000, 0.8660254037844387076, 1.000000000000000000, 0.8660254037844387076, 1.000000000000000000, 0.8660254037844387076, 1.000000000000000000, 0.8660254037844387076, 1.000000000000000000, 0.8660254037844387076, 1.000000000000000000, 0.8660254037844387076, 1.000000000000000000, 0.8660254037844387076, 1.000000000000000000, 0.8660254037844387076, 1.000000000000000000, 0.8660254037844387076, 1.000000000000000000, 0.8660254037844387076, 1.000000000000000000, 0.8660254037844387076, 1.000000000000000000, 0.8660254037844387076, 1.000000000000000000, 0.8660254037844387076, 1.000000000000000000, 0.8660254037844387076, 1.000000000000000000, 0.8660254037844387076, 1.000000000000000000, 0.8660254037844387076, 1.000000000000000000, 0.8660254037844387076, 1.000000000000000000, 0.8660254037844387076, 1.000000000000000000, 0.8660254037844387076, 1.000000000000000000, 0.8660254037844387076, 1.000000000000000000, 0.8660254037844387076, 1.000000000000000000, 0.8660254037844387076, 1.000000000000000000, 0.8660254037844387076, 1.000000000000000000, 0.8660254037844387076, 1.000000000000000000, 0.8660254037844387076, 1.000000000000000000, 0.8660254037844387076, 1.000000000000000000, 0.8660254037844387076, 1.000000000000000000, 0.8660254037844387076, 1.000000000000000000, 0.8660254037844387076, 1.000000000000000000, 0.8660254037844387076, 1.000000000000000000, 0.8660254037844387076, 1.000000000000000000, 0.8660254037844387076, 1.000000000000000000, 0.8660254037844387076, 1.000000000000000000, 0.8660254037844387076, 1.000000000000000000, 0.8660254037844387076, 1.000000000000000000, 0.8660254037844387076, 1.000000000000000000, 0.8660254037844387076, 1.000000000000000000, 0.8660254037844387076, 1.000000000000000000, 0.8660254037844387076, 1.000000000000000000, 0.8660254037844387076, 1.000000000000000000, 0.8660254037844387076, 1.000000000000000000, 0.8660254037844387076, 1.000000000000000000, 0.8660254037844387076, 1.000000000000000000, 0.8660254037844387076, 1.000000000000000000, 0.8660254037844387076, 1.000000000000000000, 0.8660254037844387076, 1.000000000000000000, 0.8660254037844387076, 1.000000000000000000, 0.8660254037844387076, 1.000000000000000000, 0.8660254037844387076, 1.000000000000000000, 0.8660254037844387076, 1.000000000000000000, 0.8660254037844387076, 1.000000000000000000, 0.8660254037844387076, 1.000000000000000000, 0.8660254037844387076, 1.000000000000000000, 0.8660254037844387076, 1.000000000000000000, 0.8660254037844387076, 1.000000000000000000, 0.8660254037844387076, 1.000000000000000000, 0.8660254037844387076, 1.000000000000000000, 0.8660254037844387076, 1.000000000000000000, 0.8660254037844387076, 1.000000000000000000, 0.8660254037844387076, 1.000000000000000000, 0.8660254037844387076, 1.000000000000000000, 0.8660254037844387076, 1.000000000000000000, 0.8660254037844387076, 1.000000000000000000, 0.8660254037844387076, 1.000000000000000000, 0.8660254037844387076, 1.000000000000000000, 0.8660254037844387076, 1.000000000000000000, 0.8660254037844387076, 1.000000000000000000, 0.8660254037844387076, 1.000000000000000000, 0.8660254037844387076, 1.000000000000000000, 0.8660254037844387076, 1.000000000000000000, 0.8660254037844387076, 1.000000000000000000, 0.8660254037844387076, 1.000000000000000000, 0.8660254037844387076, 1.000000000000000000, 0.8660254037844387076, 1.000000000000000000, 0.8660254037844387076, 1.000000000000000000, 0.8660254037844387076, 1.000000000000000000, 0.8660254037844387076, 1.000000000000000000, 0.8660254037844387076, 1.000000000000000000, 0.8660254037844387076, 1.000000000000000000, 0.8660254037844387076, 1.000000000000000000, 0.8660254037844387076, 1.000000000000000000, 0.8660254037844387076, 1.000000000000000000, 0.8660254037844387076, 1.000000000000000000, 0.8660254037844387076, 1.000000000000000000, 0.8660254037844387076, 1.000000000000000000, 0.8660254037844387076, 1.000000000000000000, 0.8660254037844387076, 1.000000000000000000, 0.8660254037844387076, 1.000000000000000000, 0.8660254037844387076, 1.000000000000000000, 0.8660254037844387076, 1.000000000000000000, 0.8660254037844387076, 1.000000000000000000, 0.8660254037844387076, 1.000000000000000000, 0.8660254037844387076, 1.000000000000000000, 0.8660254037844387076, 1.000000000000000000, 0.8660254037844387076, 1.000000000000000000, 0.8660254037844387076, 1.000000000000000000, 0.8660254037844387076, 1.000000000000000000, 0.8660254037844387076, 1.000000000000000000, 0.8660254037844387076, 1.000000000000000000, 0.8660254037844387076, 1.000000000000000000, 0.8660254037844387076, 1.000000000000000000, 0.8660254037844387076, 1.000000000000000000, 0.8660254037844387076, 1.000000000000000000, 0.8660254037844387076, 1.000000000000000000, 0.8660254037844387076, 1.000000000000000000, 0.8660254037844387076, 1.000000000000000000, 0.8660254037844387076, 1.000000000000000000, 0.8660254037844387076, 1.000000000000000000, 0.8660254037844387076, 1.000000000000000000, 0.8660254037844387076, 1.000000000000000000, 0.8660254037844387076, 1.000000000000000000, 0.8660254037844387076, 1.000000000000000000, 0.8660254037844387076, 1.000000000000000000, 0.8660254037844387076, 1.000000000000000000, 0.8660254037844387076, 1.000000000000000000, 0.8660254037844387076, 1.000000000000000000, 0.8660254037844387076, 1.000000000000000000, 0.8660254037844387076, 1.000000000000000000, 0.8660254037844387076, 1.000000000000000000, 0.8660254037844387076, 1.000000000000000000, 0.8660254037844387076, 1.000000000000000000, 0.8660254037844387076, 1.000000000000000000, 0.8660254037844387076, 1.000000000000000000, 0.8660254037844387076, 1.000000000000000000, 0.8660254037844387076, 1.000000000000000000, 0.8660254037844387076, 1.000000000000000000, 0.8660254037844387076, 1.000000000000000000, 0.8660254037844387076, 1.000000000000000000, 0.8660254037844387076, 1.000000000000000000, 0.8660254037844387076, 1.000000000000000000, 0.8660254037844387076, 1.000000000000000000, 0.8660254037844387076, 1.000000000000000000, 0.8660254037844387076, 1.000000000000000000, 0.8660254037844387076, 1.000000000000000000, 0.8660254037844387076, 1.000000000000000000, 0.8660254037844387076, 1.000000000000000000, 0.8660254037844387076, 1.000000000000000000, 0.8660254037844387076, 1.000000000000000000, 0.8660254037844387076, 1.000000000000000000, 0.8660254037844387076, 1.000000000000000000, 0.8660254037844387076, 1.000000000000000000, 0.8660254037844387076, 1.000000000000000000, 0.8660254037844387076, 1.000000000000000000, 0.8660254037844387076, 1.000000000000000000, 0.8660254037844387076, 1.000000000000000000, 0.8660254037844387076, 1.000000000000000000, 0.8660254037844387076, 1.000000000000000000, 0.8660254037844387076, 1.000000000000000000, 0.8660254037844387076, 1.000000000000000000, 0.8660254037844387076, 1.000000000000000000, 0.8660254037844387076, 1.000000000000000000, 0.8660254037844387076, 1.000000000000000000, 0.8660254037844387076, 1.000000000000000000, 0.8660254037844387076, 1.000000000000000000, 0.8660254037844387076, 1.000000000000000000, 0.8660254037844387076, 1.000000000000000000, 0.8660254037844387076, 1.000000000000000000, 0.8660254037844387076, 1.000000000000000000, 0.8660254037844387076, 1.000000000000000000, 0.8660254037844387076, 1.000000000000000000, 0.8660254037844387076, 1.000000000000000000, 0.8660254037844387076, 1.000000000000000000, 0.8660254037844387076, 1.000000000000000000, 0.8660254037844387076, 1.000000000000000000, 0.8660254037844387076, 1.000000000000000000, 0.8660254037844387076, 1.000000000000000000, 0.8660254037844387076, 1.000000000000000000, 0.8660254037844387076, 1.000000000000000000, 0.8660254037844387076, 1.000000000000000000, 0.8660254037844387076, 1.000000000000000000, 0.8660254037844387076, 1.000000000000000000, 0.8660254037844387076, 1.000000000000000000, 0.8660254037844387076, 1.000000000000000000, 0.8660254037844387076, 1.000000000000000000, 0.8660254037844387076, 1.000000000000000000, 0.8660254037844387076, 1.000000000000000000, 0.8660254037844387076, 1.000000000000000000, 0.8660254037844387076, 1.000000000000000000, 0.8660254037844387076, 1.000000000000000000, 0.8660254037844387076, 1.000000000000000000, 0.8660254037844387076, 1.000000000000000000, 0.8660254037844387076, 1.000000000000000000, 0.8660254037844387076, 1.000000000000000000, 0.8660254037844387076, 1.000000000000000000, 0.8660254037844387076, 1.000000000000000000, 0.8660254037844387076, 1.000000000000000000, 0.8660254037844387076, 1.000000000000000000, 0.8660254037844387076, 1.000000000000000000, 0.8660254037844387076, 1.000000000000000000, 0.8660254037844387076, 1.000000000000000000, 0.8660254037844387076, 1.000000000000000000, 0.8660254037844387076, 1.000000000000000000, 0.8660254037844387076, 1.000000000000000000, 0.8660254037844387076, 1.000000000000000000, 0.8660254037844387076, 1.000000000000000000, 0.8660254037844387076, 1.000000000000000000, 0.8660254037844387076, 1.000000000000000000, 0.8660254037844387076, 1.000000000000000000, 0.8660254037844387076, 1.000000000000000000, 0.8660254037844387076, 1.000000000000000000, 0.8660254037844387076, 1.000000000000000000, 0.8660254037844387076, 1.000000000000000000, 0.8660254037844387076, 1.000000000000000000, 0.8660254037844387076, 1.000000000000000000, 0.8660254037844387076, 1.000000000000000000, 0.8660254037844387076, 1.000000000000000000, 0.8660254037844387076, 1.000000000000000000, 0.8660254037844387076, 1.000000000000000000, 0.8660254037844387076, 1.000000000000000000, 0.8660254037844387076, 1.000000000000000000, 0.8660254037844387076, 1.000000000000000000, 0.8660254037844387076, 1.000000000000000000, 0.8660254037844387076, 1.000000000000000000, 0.8660254037844387076, 1.000000000000000000, 0.8660254037844387076, 1.000000000000000000, 0.8660254037844387076, 1.000000000000000000, 0.8660254037844387076, 1.000000000000000000, 0.8660254037844387076, 1.000000000000000000, 0.8660254037844387076, 1.000000000000000000, 0.8660254037844387076, 1.000000000000000000, 0.8660254037844387076, 1.000000000000000000, 0.8660254037844387076, 1.000000000000000000, 0.8660254037844387076, 1.000000000000000000, 0.8660254037844387076, 1.000000000000000000, 0.8660254037844387076, 1.000000000000000000, 0.8660254037844387076, 1.000000000000000000, 0.8660254037844387076, 1.000000000000000000, 0.8660254037844387076, 1.000000000000000000, 0.8660254037844387076, 1.000000000000000000, 0.8660254037844387076, 1.000000000000000000, 0.8660254037844387076, 1.000000000000000000, 0.8660254037844387076, 1.000000000000000000, 0.8660254037844387076, 1.000000000000000000, 0.8660254037844387076, 1.000000000000000000, 0.8660254037844387076, 1.000000000000000000, 0.8660254037844387076, 1.000000000000000000, 0.8660254037844387076, 1.000000000000000000, 0.8660254037844387076, 1.000000000000000000, 0.8660254037844387076, 1.000000000000000000, 0.8660254037844387076, 1.000000000000000000, 0.8660254037844387076, 1.000000000000000000, 0.8660254037844387076, 1.000000000000000000, 0.8660254037844387076, 1.000000000000000000, 0.8660254037844387076, 1.000000000000000000, 0.8660254037844387076, 1.000000000000000000, 0.8660254037844387076, 1.000000000000000000, 0.8660254037844387076, 1.000000000000000000, 0.8660254037844387076, 1.000000000000000000, 0.8660254037844387076, 1.000000000000000000, 0.8660254037844387076, 1.000000000000000000, 0.8660254037844387076, 1.000000000000000000, 0.8660254037844387076, 1.000000000000000000, 0.8660254037844387076, 1.000000000000000000, 0.8660254037844387076, 1.000000000000000000, 0.8660254037844387076, 1.000000000000000000, 0.8660254037844387076, 1.000000000000000000, 0.8660254037844387076, 1.000000000000000000, 0.8660254037844387076, 1.000000000000000000, 0.8660254037844387076, 1.000000000000000000, 0.8660254037844387076, 1.000000000000000000, 0.8660254037844387076, 1.000000000000000000, 0.8660254037844387076, 1.000000000000000000, 0.8660254037844387076, 1.000000000000000000, 0.8660254037844387076, 1.000000000000000000, 0.8660254037844387076, 1.000000000000000000, 0.8660254037844387076, 1.000000000000000000, 0.8660254037844387076, 1.000000000000000000, 0.8660254037844387076, 1.000000000000000000, 0.8660254037844387076, 1.000000000000000000, 0.8660254037844387076, 1.000000000000000000, 0.8660254037844387076, 1.000000000000000000, 0.8660254037844387076, 1.000000000000000000, 0.8660254037844387076, 1.000000000000000000, 0.8660254037844387076, 1.000000000000000000, 0.8660254037844387076, 1.000000000000000000, 0.8660254037844387076, 1.000000000000000000, 0.8660254037844387076, 1.000000000000000000, 0.8660254037844387076, 1.000000000000000000, 0.8660254037844387076, 1.000000000000000000, 0.8660254037844387076, 1.000000000000000000, 0.8660254037844387076, 1.000000000000000000, 0.8660254037844387076, 1.000000000000000000, 0.8660254037844387076, 1.000000000000000000, 0.8660254037844387076, 1.000000000000000000, 0.8660254037844387076, 1.000000000000000000, 0.8660254037844387076, 1.000000000000000000, 0.8660254037844387076, 1.000000000000000000, 0.8660254037844387076, 1.000000000000000000, 0.8660254037844387076, 1.000000000000000000, 0.8660254037844387076, 1.000000000000000000, 0.8660254037844387076, 1.000000000000000000, 0.8660254037844387076, 1.000000000000000000, 0.8660254037844387076, 1.000000000000000000, 0.8660254037844387076, 1.000000000000000000, 0.8660254037844387076, 1.000000000000000000, 0.8660254037844387076, 1.000000000000000000, 0.8660254037844387076, 1.000000000000000000, 0.8660254037844387076, 1.000000000000000000, 0.8660254037844387076, 1.000000000000000000, 0.8660254037844387076, 1.000000000000000000, 0.8660254037844387076, 1.000000000000000000, 0.8660254037844387076, 1.000000000000000000, 0.8660254037844387076, 1.000000000000000000, 0.8660254037844387076, 1.000000000000000000, 0.8660254037844387076, 1.000000000000000000, 0.8660254037844387076, 1.000000000000000000, 0.8660254037844387076, 1.000000000000000000, 0.8660254037844387076, 1.000000000000000000, 0.8660254037844387076, 1.000000000000000000, 0.8660254037844387076, 1.000000000000000000, 0.8660254037844387076, 1.000000000000000000, 0.8660254037844387076, 1.000000000000000000, 0.8660254037844387076, 1.000000000000000000, 0.8660254037844387076, 1.000000000000000000, 0.8660254037844387076, 1.000000000000000000, 0.8660254037844387076, 1.000000000000000000, 0.8660254037844387076, 1.000000000000000000, 0.8660254037844387076, 1.000000000000000000, 0.8660254037844387076, 1.000000000000000000, 0.8660254037844387076, 1.000000000000000000, 0.8660254037844387076, 1.000000000000000000, 0.8660254037844387076, 1.000000000000000000, 0.8660254037844387076, 1.000000000000000000, 0.8660254037844387076, 1.000000000000000000, 0.8660254037844387076, 1.000000000000000000, 0.8660254037844387076, 1.000000000000000000, 0.8660254037844387076, 1.000000000000000000, 0.8660254037844387076, 1.000000000000000000, 0.8660254037844387076, 1.000000000000000000, 0.8660254037844387076, 1.000000000000000000, 0.8660254037844387076, 1.000000000000000000, 0.8660254037844387076, 1.000000000000000000, 0.8660254037844387076, 1.000000000000000000, 0.8660254037844387076, 1.000000000000000000, 0.8660254037844387076, 1.000000000000000000, 0.8660254037844387076, 1.000000000000000000, 0.8660254037844387076, 1.000000000000000000, 0.8660254037844387076, 1.000000000000000000, 0.8660254037844387076, 1.000000000000000000, 0.8660254037844387076, 1.000000000000000000, 0.8660254037844387076, 1.000000000000000000, 0.8660254037844387076, 1.000000000000000000, 0.8660254037844387076, 1.000000000000000000, 0.8660254037844387076, 1.000000000000000000, 0.8660254037844387076, 1.000000000000000000, 0.8660254037844387076, 1.000000000000000000, 0.8660254037844387076, 1.000000000000000000, 0.8660254037844387076, 1.000000000000000000, 0.8660254037844387076, 1.000000000000000000, 0.8660254037844387076, 1.000000000000000000, 0.8660254037844387076, 1.000000000000000000, 0.8660254037844387076, 1.000000000000000000, 0.8660254037844387076, 1.000000000000000000, 0.8660254037844387076, 1.000000000000000000, 0.8660254037844387076, 1.000000000000000000, 0.8660254037844387076, 1.000000000000000000, 0.8660254037844387076, 1.000000000000000000, 0.8660254037844387076, 1.000000000000000000, 0.8660254037844387076, 1.000000000000000000, 0.8660254037844387076, 1.000000000000000000, 0.8660254037844387076, 1.000000000000000000, 0.8660254037844387076, 1.000000000000000000, 0.8660254037844387076, 1.000000000000000000, 0.8660254037844387076, 1.000000000000000000, 0.8660254037844387076, 1.000000000000000000, 0.8660254037844387076, 1.000000000000000000, 0.8660254037844387076, 1.000000000000000000, 0.8660254037844387076, 1.000000000000000000, 0.8660254037844387076, 1.000000000000000000, 0.8660254037844387076, 1.000000000000000000, 0.8660254037844387076, 1.000000000000000000, 0.8660254037844387076, 1.000000000000000000, 0.8660254037844387076, 1.000000000000000000, 0.8660254037844387076, 1.000000000000000000, 0.8660254037844387076, 1.000000000000000000, 0.8660254037844387076, 1.000000000000000000, 0.8660254037844387076, 1.000000000000000000, 0.8660254037844387076, 1.000000000000000000, 0.8660254037844387076, 1.000000000000000000, 0.8660254037844387076, 1.000000000000000000, 0.8660254037844387076, 1.000000000000000000, 0.8660254037844387076, 1.000000000000000000, 0.8660254037844387076, 1.000000000000000000, 0.8660254037844387076, 1.000000000000000000, 0.8660254037844387076, 1.000000000000000000, 0.8660254037844387076, 1.000000000000000000, 0.8660254037844387076, 1.000000000000000000, 0.8660254037844387076, 1.000000000000000000, 0.8660254037844387076, 1.000000000000000000, 0.8660254037844387076, 1.000000000000000000, 0.8660254037844387076, 1.000000000000000000, 0.8660254037844387076, 1.000000000000000000, 0.8660254037844387076, 1.000000000000000000, 0.8660254037844387076, 1.000000000000000000, 0.8660254037844387076, 1.000000000000000000, 0.8660254037844387076, 1.000000000000000000, 0.8660254037844387076, 1.000000000000000000, 0.8660254037844387076, 1.000000000000000000, 0.8660254037844387076, 1.000000000000000000, 0.8660254037844387076, 1.000000000000000000, 0.8660254037844387076, 1.000000000000000000, 0.8660254037844387076, 1.000000000000000000, 0.8660254037844387076, 1.000000000000000000, 0.8660254037844387076, 1.000000000000000000, 0.8660254037844387076, 1.000000000000000000, 0.8660254037844387076, 1.000000000000000000, 0.8660254037844387076, 1.000000000000000000, 0.8660254037844387076, 1.000000000000000000, 0.8660254037844387076, 1.000000000000000000, 0.8660254037844387076, 1.000000000000000000, 0.8660254037844387076, 1.000000000000000000, 0.8660254037844387076, 1.000000000000000000, 0.8660254037844387076, 1.000000000000000000, 0.8660254037844387076, 1.000000000000000000, 0.8660254037844387076, 1.000000000000000000, 0.8660254037844387076, 1.000000000000000000, 0.8660254037844387076, 1.000000000000000000, 0.8660254037844387076, 1.000000000000000000, 0.8660254037844387076, 1.000000000000000000, 0.8660254037844387076, 1.000000000000000000, 0.8660254037844387076, 1.000000000000000000, 0.8660254037844387076, 1.000000000000000000, 0.8660254037844387076, 1.000000000000000000, 0.8660254037844387076, 1.000000000000000000, 0.8660254037844387076, 1.000000000000000000, 0.8660254037844387076, 1.000000000000000000, 0.8660254037844387076, 1.000000000000000000, 0.8660254037844387076, 1.000000000000000000, 0.8660254037844387076, 1.000000000000000000, 0.8660254037844387076, 1.000000000000000000, 0.8660254037844387076, 1.000000000000000000, 0.8660254037844387076, 1.000000000000000000, 0.8660254037844387076, 1.000000000000000000, 0.8660254037844387076, 1.000000000000000000, 0.8660254037844387076, 1.000000000000000000, 0.8660254037844387076, 1.000000000000000000, 0.8660254037844387076, 1.000000000000000000, 0.8660254037844387076, 1.000000000000000000, 0.8660254037844387076, 1.000000000000000000, 0.8660254037844387076, 1.000000000000000000, 0.8660254037844387076, 1.000000000000000000, 0.8660254037844387076, 1.000000000000000000, 0.8660254037844387076, 1.000000000000000000, 0.8660254037844387076, 1.000000000000000000, 0.8660254037844387076, 1.000000000000000000, 0.8660254037844387076, 1.000000000000000000, 0.8660254037844387076, 1.000000000000000000, 0.8660254037844387076, 1.000000000000000000, 0.8660254037844387076, 1.000000000000000000, 0.8660254037844387076, 1.000000000000000000, 0.8660254037844387076, 1.000000000000000000, 0.8660254037844387076, 1.000000000000000000, 0.8660254037844387076, 1.000000000000000000, 0.8660254037844387076, 1.000000000000000000, 0.8660254037844387076, 1.000000000000000000, 0.8660254037844387076, 1.000000000000000000, 0.8660254037844387076, 1.000000000000000000, 0.8660254037844387076, 1.000000000000000000, 0.8660254037844387076, 1.000000000000000000, 0.8660254037844387076, 1.000000000000000000, 0.8660254037844387076, 1.000000000000000000, 0.8660254037844387076, 1.000000000000000000, 0.8660254037844387076, 1.000000000000000000, 0.8660254037844387076, 1.000000000000000000, 0.8660254037844387076, 1.000000000000000000, 0.8660254037844387076, 1.000000000000000000, 0.8660254037844387076, 1.000000000000000000, 0.8660254037844387076, 1.000000000000000000, 0.8660254037844387076, 1.000000000000000000, 0.8660254037844387076, 1.000000000000000000, 0.8660254037844387076, 1.000000000000000000, 0.8660254037844387076, 1.000000000000000000, 0.8660254037844387076, 1.000000000000000000, 0.8660254037844387076, 1.000000000000000000, 0.8660254037844387076, 1.000000000000000000, 0.8660254037844387076, 1.000000000000000000, 0.8660254037844387076, 1.000000000000000000, 0.8660254037844387076, 1.000000000000000000, 0.8660254037844387076, 1.000000000000000000, 0.8660254037844387076, 1.000000000000000000, 0.8660254037844387076, 1.000000000000000000, 0.8660254037844387076, 1.000000000000000000, 0.8660254037844387076, 1.000000000000000000, 0.8660254037844387076, 1.000000000000000000, 0.8660254037844387076, 1.000000000000000000, 0.8660254037844387076, 1.000000000000000000, 0.8660254037844387076, 1.000000000000000000, 0.8660254037844387076, 1.000000000000000000, 0.8660254037844387076, 1.000000000000000000, 0.8660254037844387076, 1.000000000000000000, 0.8660254037844387076, 1.000000000000000000, 0.8660254037844387076, 1.000000000000000000, 0.8660254037844387076, 1.000000000000000000, 0.8660254037844387076, 1.000000000000000000, 0.8660254037844387076, 1.000000000000000000, 0.8660254037844387076, 1.000000000000000000, 0.8660254037844387076, 1.000000000000000000, 0.8660254037844387076, 1.000000000000000000, 0.8660254037844387076, 1.000000000000000000, 0.8660254037844387076, 1.000000000000000000, 0.8660254037844387076, 1.000000000000000000, 0.8660254037844387076, 1.000000000000000000, 0.8660254037844387076, 1.000000000000000000, 0.8660254037844387076, 1.000000000000000000, 0.8660254037844387076, 1.000000000000000000, 0.8660254037844387076, 1.000000000000000000, 0.8660254037844387076, 1.000000000000000000, 0.8660254037844387076, 1.000000000000000000, 0.8660254037844387076, 1.000000000000000000, 0.8660254037844387076, 1.000000000000000000, 0.8660254037844387076, 1.000000000000000000, 0.8660254037844387076, 1.000000000000000000, 0.8660254037844387076, 1.000000000000000000, 0.8660254037844387076, 1.000000000000000000, 0.8660254037844387076, 1.000000000000000000, 0.8660254037844387076, 1.000000000000000000, 0.8660254037844387076, 1.000000000000000000, 0.8660254037844387076, 1.000000000000000000, 0.8660254037844387076, 1.000000000000000000, 0.8660254037844387076, 1.000000000000000000, 0.8660254037844387076, 1.000000000000000000, 0.8660254037844387076, 1.000000000000000000, 0.8660254037844387076, 1.000000000000000000, 0.8660254037844387076, 1.000000000000000000, 0.8660254037844387076, 1.000000000000000000, 0.8660254037844387076, 1.000000000000000000, 0.8660254037844387076, 1.000000000000000000, 0.8660254037844387076, 1.000000000000000000, 0.8660254037844387076, 1.000000000000000000, 0.8660254037844387076, 1.000000000000000000, 0.8660254037844387076, 1.000000000000000000, 0.8660254037844387076, 1.000000000000000000, 0.8660254037844387076, 1.000000000000000000, 0.8660254037844387076, 1.000000000000000000, 0.8660254037844387076, 1.000000000000000000, 0.8660254037844387076, 1.000000000000000000, 0.8660254037844387076, 1.000000000000000000, 0.8660254037844387076, 1.000000000000000000, 0.8660254037844387076, 1.000000000000000000, 0.8660254037844387076, 1.000000000000000000, 0.8660254037844387076, 1.000000000000000000, 0.8660254037844387076, 1.000000000000000000, 0.8660254037844387076, 1.000000000000000000, 0.8660254037844387076, 1.000000000000000000, 0.8660254037844387076, 1.000000000000000000, 0.8660254037844387076, 1.000000000000000000, 0.8660254037844387076, 1.000000000000000000, 0.8660254037844387076, 1.000000000000000000, 0.8660254037844387076, 1.000000000000000000, 0.8660254037844387076, 1.000000000000000000, 0.8660254037844387076, 1.000000000000000000, 0.8660254037844387076, 1.000000000000000000, 0.8660254037844387076, 1.000000000000000000, 0.8660254037844387076, 1.000000000000000000, 0.8660254037844387076, 1.000000000000000000, 0.8660254037844387076, 1.000000000000000000, 0.8660254037844387076, 1.000000000000000000, 0.8660254037844387076, 1.000000000000000000, 0.8660254037844387076, 1.000000000000000000, 0.8660254037844387076, 1.000000000000000000, 0.8660254037844387076, 1.000000000000000000, 0.8660254037844387076, 1.000000000000000000, 0.8660254037844387076, 1.000000000000000000, 0.8660254037844387076, 1.000000000000000000, 0.8660254037844387076, 1.000000000000000000, 0.8660254037844387076, 1.000000000000000000, 0.8660254037844387076, 1.000000000000000000, 0.8660254037844387076, 1.000000000000000000, 0.8660254037844387076, 1.000000000000000000, 0.8660254037844387076, 1.000000000000000000, 0.8660254037844387076, 1.000000000000000000, 0.8660254037844387076, 1.000000000000000000, 0.8660254037844387076, 1.000000000000000000) ) ) 
 REPRESENTATION_ITEM ( '' )  SURFACE ( )  );
#8897=CARTESIAN_POINT ( 'NONE',  ( -9.999999999999998224, 5.773502691896259087, -115.7500000040967763 ) ) ;
#8899=CARTESIAN_POINT ( 'NONE',  ( -5.405949406249996869, 9.363379034771805109, -74.34375000204838102 ) ) ;
#8903=CARTESIAN_POINT ( 'NONE',  ( -10.00000000000051337, 5.773502691895962435, -118.7500000040967763 ) ) ;
#8904=CARTESIAN_POINT ( 'NONE',  ( -5.405949406249996869, 9.363379034771805109, -37.03125000204837391 ) ) ;
#8905=( BOUNDED_CURVE ( )  B_SPLINE_CURVE ( 2, ( #27015, #26803, #13188, #29410, #23361, #13611, #16422 ),
 .UNSPECIFIED., .F., .F. ) 
 B_SPLINE_CURVE_WITH_KNOTS ( ( 3, 2, 2, 3 ),
 ( 0.4141791044776120256, 0.4154228855721394109, 0.4166666666666667962, 0.4179104477611941260 ),
 .UNSPECIFIED. ) 
 CURVE ( )  GEOMETRIC_REPRESENTATION_ITEM ( )  RATIONAL_B_SPLINE_CURVE ( ( 0.9999999999999880096, 0.8660254037844506980, 1.000000000000000000, 0.8660254037844387076, 1.000000000000000000, 0.8660254037844267172, 1.000000000000011990 ) ) 
 REPRESENTATION_ITEM ( '' )  );
#8913=AXIS2_PLACEMENT_3D ( 'NONE', #3363, #16496, #23568 ) ;
#8916=CARTESIAN_POINT ( 'NONE',  ( 7.070501591499376803E-16, 11.54700538379251284, -135.5000000040967905 ) ) ;
#8920=CARTESIAN_POINT ( 'NONE',  ( -9.999999999999998224, 1.224646799147353059E-15, -130.6250000040967620 ) ) ;
#8924=CARTESIAN_POINT ( 'NONE',  ( -2.293366432827344421E-15, -12.48450537969573659, -133.7187500020483810 ) ) ;
#8925=CARTESIAN_POINT ( 'NONE',  ( -10.81189881249999907, -6.242252689847864744, -137.1562500020483810 ) ) ;
#8926=CARTESIAN_POINT ( 'NONE',  ( 7.070501591499376803E-16, 11.54700538379251284, -104.0000000040967763 ) ) ;
#8927=CARTESIAN_POINT ( 'NONE',  ( 5.405949406249999534, 9.363379034771803333, -149.5937500020483810 ) ) ;
#8930=CARTESIAN_POINT ( 'NONE',  ( -10.00000000000000000, -5.773502691896251982, -172.1250000000000284 ) ) ;
#8932=CARTESIAN_POINT ( 'NONE',  ( 4.999999999999992006, -8.660254037844389075, -113.6250000040967763 ) ) ;
#8934=CARTESIAN_POINT ( 'NONE',  ( -9.999999999999998224, 1.224646799147353059E-15, -149.7500000000000000 ) ) ;
#8935=CARTESIAN_POINT ( 'NONE',  ( -10.81189881249999729, 6.242252689847871849, -171.7187500020483810 ) ) ;
#8938=CARTESIAN_POINT ( 'NONE',  ( 0.000000000000000000, 0.000000000000000000, -99.99999999999998579 ) ) ;
#8939=CARTESIAN_POINT ( 'NONE',  ( 5.405949406249999534, 9.363379034771803333, -37.28125000204837391 ) ) ;
#8941=CARTESIAN_POINT ( 'NONE',  ( 9.999999999999998224, 0.000000000000000000, -97.99999999999998579 ) ) ;
#8943=CARTESIAN_POINT ( 'NONE',  ( 10.81189881249999729, 0.000000000000000000, -115.5312500020483952 ) ) ;
#8944=CARTESIAN_POINT ( 'NONE',  ( -9.999999999999998224, 1.224646799147353059E-15, -139.6250000040967905 ) ) ;
#8949=CARTESIAN_POINT ( 'NONE',  ( 10.00000000000025402, -5.773502691896113426, -155.1250000000000000 ) ) ;
#8950=CARTESIAN_POINT ( 'NONE',  ( -2.293366432827344421E-15, -12.48450537969573659, -64.90625000204838102 ) ) ;
#8956=EDGE_CURVE ( 'NONE', #5520, #13539, #22708, .T. ) ;
#8961=VERTEX_POINT ( 'NONE', #14471 ) ;
#8962=EDGE_LOOP ( 'NONE', ( #2746, #9472, #12597, #23988 ) ) ;
#8969=CARTESIAN_POINT ( 'NONE',  ( -9.999999999999998224, 1.224646799147353059E-15, -112.6250000040967763 ) ) ;
#8970=CARTESIAN_POINT ( 'NONE',  ( -5.000000000000003553, -8.660254037844383745, -35.49999999999997868 ) ) ;
#8973=CARTESIAN_POINT ( 'NONE',  ( -5.405949406250003975, -9.363379034771801557, -160.8437500020484094 ) ) ;
#8974=CARTESIAN_POINT ( 'NONE',  ( -10.81189881249999729, 6.242252689847871849, -170.2187500020483810 ) ) ;
#8976=CARTESIAN_POINT ( 'NONE',  ( 10.00000000000000000, 5.773502691896255534, -132.3750000000000000 ) ) ;
#8977=CARTESIAN_POINT ( 'NONE',  ( -9.999999999999998224, 5.773502691896259087, -197.8750000000000000 ) ) ;
#8982=CARTESIAN_POINT ( 'NONE',  ( 10.81189881249999729, 0.000000000000000000, -63.03125000204837391 ) ) ;
#8984=CARTESIAN_POINT ( 'NONE',  ( 9.999999999999998224, 0.000000000000000000, -122.0000000000000000 ) ) ;
#8985=EDGE_LOOP ( 'NONE', ( #26781, #4177, #32898, #19504 ) ) ;
#8986=CARTESIAN_POINT ( 'NONE',  ( -10.81189881249999729, 6.242252689847871849, -140.4062500020484094 ) ) ;
#8987=CARTESIAN_POINT ( 'NONE',  ( 5.405949406249992428, -9.363379034771808662, -159.2812500020484094 ) ) ;
#8990=CARTESIAN_POINT ( 'NONE',  ( -5.405949406250003975, -9.363379034771801557, -87.34375000204836681 ) ) ;
#8993=CARTESIAN_POINT ( 'NONE',  ( 10.81189881249999729, 0.000000000000000000, -194.8437500020484094 ) ) ;
#8997=CARTESIAN_POINT ( 'NONE',  ( 7.644554776091147741E-16, 12.48450537969573659, -95.65625000204838102 ) ) ;
#8999=CARTESIAN_POINT ( 'NONE',  ( 5.000000000000000000, 8.660254037844385522, -66.62500000409676204 ) ) ;
#9000=CARTESIAN_POINT ( 'NONE',  ( 0.000000000000000000, 0.000000000000000000, -99.99999999999998579 ) ) ;
#9001=CARTESIAN_POINT ( 'NONE',  ( -10.81189881249999907, -6.242252689847864744, -22.96875000204837036 ) ) ;
#9005=CARTESIAN_POINT ( 'NONE',  ( 10.81189881249999729, 0.000000000000000000, -22.53125000204836326 ) ) ;
#9008=CARTESIAN_POINT ( 'NONE',  ( 0.000000000000000000, 0.000000000000000000, -99.99999999999998579 ) ) ;
#9014=ORIENTED_EDGE ( 'NONE', *, *, #1558, .T. ) ;
#9019=ORIENTED_EDGE ( 'NONE', *, *, #33581, .F. ) ;
#9024=CARTESIAN_POINT ( 'NONE',  ( 10.13602244787124995, -1.019214064432307332, -99.99999999999994316 ) ) ;
#9026=CARTESIAN_POINT ( 'NONE',  ( -4.999999999999996447, 8.660254037844387298, -129.0000000000000000 ) ) ;
#9027=CARTESIAN_POINT ( 'NONE',  ( 7.644554776091147741E-16, 12.48450537969573659, -152.6562500020484094 ) ) ;
#9029=CARTESIAN_POINT ( 'NONE',  ( 0.000000000000000000, 0.000000000000000000, -99.99999999999998579 ) ) ;
#9033=CARTESIAN_POINT ( 'NONE',  ( 7.644554776091147741E-16, 12.48450537969573659, -81.96875000204839523 ) ) ;
#9034=CARTESIAN_POINT ( 'NONE',  ( -10.81189881249999907, -6.242252689847864744, -92.15625000204839523 ) ) ;
#9038=CARTESIAN_POINT ( 'NONE',  ( -2.293366432827344421E-15, -12.48450537969573659, -177.4062500020484379 ) ) ;
#9039=CARTESIAN_POINT ( 'NONE',  ( -10.81189881249999729, 6.242252689847871849, -185.4062500020484094 ) ) ;
#9041=CARTESIAN_POINT ( 'NONE',  ( 7.070501591499377789E-16, 11.54700538379251284, -165.5000000040967905 ) ) ;
#9043=CARTESIAN_POINT ( 'NONE',  ( 10.81189881249999551, -6.242252689847874514, -11.96875000204836326 ) ) ;
#9045=CARTESIAN_POINT ( 'NONE',  ( -2.293366432827344421E-15, -12.48450537969573659, -118.7187500020483952 ) ) ;
#9047=CARTESIAN_POINT ( 'NONE',  ( 5.405949406249992428, -9.363379034771808662, -16.78125000204835970 ) ) ;
#9049=CARTESIAN_POINT ( 'NONE',  ( -10.81189881249999907, -6.242252689847864744, -119.1562500020484237 ) ) ;
#9052=CARTESIAN_POINT ( 'NONE',  ( -5.000000000000003553, -8.660254037844383745, -95.87500000409677625 ) ) ;
#9055=CARTESIAN_POINT ( 'NONE',  ( -2.293366432827344421E-15, -12.48450537969573659, -52.71875000204837391 ) ) ;
#9056=ORIENTED_EDGE ( 'NONE', *, *, #17227, .T. ) ;
#9060=CARTESIAN_POINT ( 'NONE',  ( -10.00000000000000000, -5.773502691896251982, -24.00000000409677270 ) ) ;
#9062=CARTESIAN_POINT ( 'NONE',  ( -9.999999999999998224, 1.224646799147353059E-15, -120.1250000040967905 ) ) ;
#9076=CARTESIAN_POINT ( 'NONE',  ( 7.070501591499376803E-16, 11.54700538379251284, -171.1250000000000000 ) ) ;
#9078=CARTESIAN_POINT ( 'NONE',  ( 10.81189881249999907, 6.242252689847868297, -190.4062500020484094 ) ) ;
#9080=DIRECTION ( 'NONE',  ( 1.000000000000000000, 0.000000000000000000, 0.000000000000000000 ) ) ;
#9082=CARTESIAN_POINT ( 'NONE',  ( -10.81189881249999729, 6.242252689847871849, -108.7187500020483810 ) ) ;
#9084=CARTESIAN_POINT ( 'NONE',  ( 5.405949406249999534, 9.363379034771803333, -113.7812500020483952 ) ) ;
#9086=CARTESIAN_POINT ( 'NONE',  ( 5.405949406249999534, 9.363379034771803333, -119.5937500020483810 ) ) ;
#9089=CARTESIAN_POINT ( 'NONE',  ( -2.121150477449813534E-15, -11.54700538379251284, -137.3750000000000000 ) ) ;
#9090=CARTESIAN_POINT ( 'NONE',  ( 7.070501591499377789E-16, 11.54700538379251284, -16.62499999999997158 ) ) ;
#9095=CARTESIAN_POINT ( 'NONE',  ( 9.999999999999996447, -5.773502691896262640, -191.5000000040968189 ) ) ;
#9097=CARTESIAN_POINT ( 'NONE',  ( 10.81189881249999729, 0.000000000000000000, -35.84375000204836681 ) ) ;
#9098=CARTESIAN_POINT ( 'NONE',  ( -10.81189881249999729, 6.242252689847871849, -147.7187500020484094 ) ) ;
#9100=( BOUNDED_CURVE ( )  B_SPLINE_CURVE ( 2, ( #20191, #19547, #3167, #3593, #7038, #16725, #26673 ),
 .UNSPECIFIED., .F., .F. ) 
 B_SPLINE_CURVE_WITH_KNOTS ( ( 3, 2, 2, 3 ),
 ( 0.3022388059701494045, 0.3034825870646767343, 0.3047263681592040085, 0.3059701492537313383 ),
 .UNSPECIFIED. ) 
 CURVE ( )  GEOMETRIC_REPRESENTATION_ITEM ( )  RATIONAL_B_SPLINE_CURVE ( ( 0.9999999999999820144, 0.8660254037844566932, 1.000000000000000000, 0.8660254037844387076, 1.000000000000000000, 0.8660254037844387076, 1.000000000000000000 ) ) 
 REPRESENTATION_ITEM ( '' )  );
#9101=CARTESIAN_POINT ( 'NONE',  ( 9.999999999999998224, 0.000000000000000000, -63.49999999999997158 ) ) ;
#9102=CARTESIAN_POINT ( 'NONE',  ( 5.405949406249992428, -9.363379034771808662, -142.7812500020483810 ) ) ;
#9104=ORIENTED_EDGE ( 'NONE', *, *, #4578, .F. ) ;
#9105=CARTESIAN_POINT ( 'NONE',  ( 9.999999999999998224, 0.000000000000000000, -164.0000000000000000 ) ) ;
#9106=CARTESIAN_POINT ( 'NONE',  ( 7.070501591499377789E-16, 11.54700538379251284, -114.5000000040967905 ) ) ;
#9108=CARTESIAN_POINT ( 'NONE',  ( -10.81189881249999729, 6.242252689847871849, -72.71875000204835260 ) ) ;
#9113=CARTESIAN_POINT ( 'NONE',  ( -2.293366432827344421E-15, -12.48450537969573659, -37.90625000204836681 ) ) ;
#9130=LINE ( 'NONE', #18623, #41739 ) ;
#9131=CARTESIAN_POINT ( 'NONE',  ( -5.405949406250003975, -9.363379034771801557, -136.8437500020484094 ) ) ;
#9132=CARTESIAN_POINT ( 'NONE',  ( 10.81189881249999907, 6.242252689847868297, -140.9062500020484094 ) ) ;
#9134=CARTESIAN_POINT ( 'NONE',  ( -5.405949406249996869, 9.363379034771805109, -144.8437500020483810 ) ) ;
#9135=CARTESIAN_POINT ( 'NONE',  ( 0.000000000000000000, 0.000000000000000000, -99.99999999999998579 ) ) ;
#9138=CARTESIAN_POINT ( 'NONE',  ( 10.00000000000000000, 5.773502691896255534, -163.8750000000000000 ) ) ;
#9140=CARTESIAN_POINT ( 'NONE',  ( -2.121150477449813534E-15, -11.54700538379251284, -113.7500000040967763 ) ) ;
#9142=CARTESIAN_POINT ( 'NONE',  ( 10.81189881249999907, 6.242252689847868297, -59.71875000204838102 ) ) ;
#9144=CARTESIAN_POINT ( 'NONE',  ( 5.405949406249992428, -9.363379034771808662, -174.0937500020484094 ) ) ;
#9147=DIRECTION ( 'NONE',  ( -1.000000000000000000, 0.000000000000000000, 0.000000000000000000 ) ) ;
#9148=CARTESIAN_POINT ( 'NONE',  ( -10.81189881249999907, -6.242252689847864744, -38.15625000204835970 ) ) ;
#9150=CARTESIAN_POINT ( 'NONE',  ( -10.00000000000000000, -5.773502691896251982, -98.62499999999998579 ) ) ;
#9153=CARTESIAN_POINT ( 'NONE',  ( 10.81189881249999551, -6.242252689847874514, -115.6562500020483810 ) ) ;
#9154=CARTESIAN_POINT ( 'NONE',  ( 9.999999999999996447, -5.773502691896262640, -140.5000000040967905 ) ) ;
#9157=CARTESIAN_POINT ( 'NONE',  ( -10.81189881249999729, 6.242252689847871849, -63.90625000204838813 ) ) ;
#9160=CARTESIAN_POINT ( 'NONE',  ( -9.999999999999998224, 1.224646799147353059E-15, -106.6250000040967763 ) ) ;
#9164=DIRECTION ( 'NONE',  ( 1.000000000000000000, 0.000000000000000000, 0.000000000000000000 ) ) ;
#9169=ORIENTED_EDGE ( 'NONE', *, *, #36496, .T. ) ;
#9176=CARTESIAN_POINT ( 'NONE',  ( -4.999999999999996447, 8.660254037844387298, -28.49999999999997158 ) ) ;
#9179=CARTESIAN_POINT ( 'NONE',  ( -5.405949406249996869, 9.363379034771805109, -155.3437500020483810 ) ) ;
#9180=CARTESIAN_POINT ( 'NONE',  ( -10.81189881249999729, 1.324075727343319199E-15, -168.5937500020484094 ) ) ;
#9182=CARTESIAN_POINT ( 'NONE',  ( 9.999999999999998224, 0.000000000000000000, -162.8750000040967905 ) ) ;
#9183=CARTESIAN_POINT ( 'NONE',  ( -10.00000000000000000, -5.773502691896251982, -193.1250000000000284 ) ) ;
#9188=CARTESIAN_POINT ( 'NONE',  ( -10.81189881249999729, 1.324075727343319199E-15, -62.28125000204837391 ) ) ;
#9190=CARTESIAN_POINT ( 'NONE',  ( -10.00000000000000000, -5.773502691896251982, -119.6249999999999858 ) ) ;
#9191=EDGE_CURVE ( 'NONE', #31697, #39083, #27112, .T. ) ;
#9193=CARTESIAN_POINT ( 'NONE',  ( 10.81189881249999729, 0.000000000000000000, -144.0312500020483810 ) ) ;
#9194=CARTESIAN_POINT ( 'NONE',  ( 5.405949406249992428, -9.363379034771808662, -157.7812500020484094 ) ) ;
#9196=DIRECTION ( 'NONE',  ( -0.000000000000000000, -0.000000000000000000, -1.000000000000000000 ) ) ;
#9197=CARTESIAN_POINT ( 'NONE',  ( 7.644554776091147741E-16, 12.48450537969573659, -89.46875000204838102 ) ) ;
#9200=CARTESIAN_POINT ( 'NONE',  ( -5.405949406249996869, 9.363379034771805109, -186.8437500020483810 ) ) ;
#9202=CARTESIAN_POINT ( 'NONE',  ( 4.999999999999992006, -8.660254037844389075, -116.6250000040967905 ) ) ;
#9204=CARTESIAN_POINT ( 'NONE',  ( 10.81189881249999551, -6.242252689847874514, -82.65625000204836681 ) ) ;
#9206=CARTESIAN_POINT ( 'NONE',  ( 9.999999999999998224, 0.000000000000000000, -56.37500000409676204 ) ) ;
#9208=CARTESIAN_POINT ( 'NONE',  ( -10.81189881249999907, -6.242252689847864744, -15.46875000204836503 ) ) ;
#9210=CARTESIAN_POINT ( 'NONE',  ( -2.293366432827344421E-15, -12.48450537969573659, -19.90625000204837391 ) ) ;
#9213=( BOUNDED_CURVE ( )  B_SPLINE_CURVE ( 2, ( #36799, #36585, #17355, #29914, #33579, #3585, #13475 ),
 .UNSPECIFIED., .F., .F. ) 
 B_SPLINE_CURVE_WITH_KNOTS ( ( 3, 2, 2, 3 ),
 ( 0.1380597014925373234, 0.1393034825870646809, 0.1405472636815920384, 0.1417910447761193959 ),
 .UNSPECIFIED. ) 
 CURVE ( )  GEOMETRIC_REPRESENTATION_ITEM ( )  RATIONAL_B_SPLINE_CURVE ( ( 1.000000000000000000, 0.8660254037844387076, 1.000000000000000000, 0.8660254037844387076, 1.000000000000000000, 0.8660254037844387076, 1.000000000000000000 ) ) 
 REPRESENTATION_ITEM ( '' )  );
#9223=ORIENTED_EDGE ( 'NONE', *, *, #16683, .T. ) ;
#9228=CARTESIAN_POINT ( 'NONE',  ( 9.999999999999866773, -5.773502691896336358, -173.1250000000000000 ) ) ;
#9232=CARTESIAN_POINT ( 'NONE',  ( 5.405949406249992428, -9.363379034771808662, -154.7812500020484094 ) ) ;
#9238=CARTESIAN_POINT ( 'NONE',  ( -10.81189881249999907, -6.242252689847864744, -79.96875000204836681 ) ) ;
#9239=CARTESIAN_POINT ( 'NONE',  ( -2.293366432827344421E-15, -12.48450537969573659, -82.90625000204838102 ) ) ;
#9241=CARTESIAN_POINT ( 'NONE',  ( 7.644554776091147741E-16, 12.48450537969573659, -164.6562500020484094 ) ) ;
#9242=CARTESIAN_POINT ( 'NONE',  ( -5.405949406250003975, -9.363379034771801557, -179.0312500020483810 ) ) ;
#9244=CARTESIAN_POINT ( 'NONE',  ( -2.121150477449813534E-15, -11.54700538379251284, -154.2500000040967620 ) ) ;
#9246=CARTESIAN_POINT ( 'NONE',  ( -5.405949406250003975, -9.363379034771801557, -7.843750002048343717 ) ) ;
#9248=CARTESIAN_POINT ( 'NONE',  ( 5.405949406249992428, -9.363379034771808662, -111.0937500020483810 ) ) ;
#9249=ADVANCED_FACE ( 'NONE', ( #24658 ), #21614, .F. ) ;
#9251=CARTESIAN_POINT ( 'NONE',  ( 5.405949406249992428, -9.363379034771808662, -9.281250002048352599 ) ) ;
#9253=CARTESIAN_POINT ( 'NONE',  ( 9.999999999999994671, -5.773502691896262640, -170.5000000040967905 ) ) ;
#9254=CARTESIAN_POINT ( 'NONE',  ( -5.405949406250003975, -9.363379034771801557, -117.5312500020483952 ) ) ;
#9256=ORIENTED_EDGE ( 'NONE', *, *, #23486, .T. ) ;
#9257=( BOUNDED_CURVE ( )  B_SPLINE_CURVE ( 2, ( #36270, #29165, #15969, #32622, #32201, #22469, #16384 ),
 .UNSPECIFIED., .F., .F. ) 
 B_SPLINE_CURVE_WITH_KNOTS ( ( 3, 2, 2, 3 ),
 ( 0.2798507462686568026, 0.2810945273631841879, 0.2823383084577115731, 0.2835820895522389029 ),
 .UNSPECIFIED. ) 
 CURVE ( )  GEOMETRIC_REPRESENTATION_ITEM ( )  RATIONAL_B_SPLINE_CURVE ( ( 0.9999999999999880096, 0.8660254037844506980, 1.000000000000000000, 0.8660254037844387076, 1.000000000000000000, 0.8660254037844267172, 1.000000000000011990 ) ) 
 REPRESENTATION_ITEM ( '' )  );
#9258=CARTESIAN_POINT ( 'NONE',  ( 9.999999999999998224, 0.000000000000000000, -92.37500000409677625 ) ) ;
#9260=CARTESIAN_POINT ( 'NONE',  ( 5.405949406249999534, 9.363379034771803333, -40.09375000204837391 ) ) ;
#9265=CARTESIAN_POINT ( 'NONE',  ( 7.070501591499377789E-16, 11.54700538379251284, -21.50000000409676915 ) ) ;
#9266=CARTESIAN_POINT ( 'NONE',  ( -5.000000000000003553, -8.660254037844383745, -119.8750000040967905 ) ) ;
#9274=ORIENTED_EDGE ( 'NONE', *, *, #7790, .T. ) ;
#9279=CARTESIAN_POINT ( 'NONE',  ( -5.405949406249996869, 9.363379034771805109, -179.5312500020483810 ) ) ;
#9283=CARTESIAN_POINT ( 'NONE',  ( 7.644554776091147741E-16, 12.48450537969573659, -104.4687500020483668 ) ) ;
#9285=CARTESIAN_POINT ( 'NONE',  ( -10.81189881249999907, -6.242252689847864744, -107.1562500020483952 ) ) ;
#9287=CARTESIAN_POINT ( 'NONE',  ( 10.81189881249999729, 0.000000000000000000, -125.8437500020483952 ) ) ;
#9291=CARTESIAN_POINT ( 'NONE',  ( -2.121150477449813534E-15, -11.54700538379251284, -135.8750000000000000 ) ) ;
#9292=CARTESIAN_POINT ( 'NONE',  ( 9.999999999999996447, -5.773502691896262640, -2.124999999999960476 ) ) ;
#9296=CARTESIAN_POINT ( 'NONE',  ( 4.999999999999992006, -8.660254037844389075, -185.6250000040967905 ) ) ;
#9298=CARTESIAN_POINT ( 'NONE',  ( -10.81189881249999729, 6.242252689847871849, -39.71875000204835970 ) ) ;
#9299=CARTESIAN_POINT ( 'NONE',  ( 10.00000000000076916, -5.773502691895816774, -107.5000000040967620 ) ) ;
#9300=CARTESIAN_POINT ( 'NONE',  ( 10.81189881249999729, 0.000000000000000000, -136.3437500020484094 ) ) ;
#9305=CARTESIAN_POINT ( 'NONE',  ( 7.070501591499377789E-16, 11.54700538379251284, -69.12500000000000000 ) ) ;
#9306=CARTESIAN_POINT ( 'NONE',  ( -10.81189881249999729, 1.324075727343319199E-15, -140.2812500020483810 ) ) ;
#9311=CARTESIAN_POINT ( 'NONE',  ( 7.070501591499377789E-16, 11.54700538379251284, -117.5000000040967905 ) ) ;
#9313=CARTESIAN_POINT ( 'NONE',  ( 10.81189881249999551, -6.242252689847874514, -73.46875000204835260 ) ) ;
#9318=CARTESIAN_POINT ( 'NONE',  ( 5.405949406249999534, 9.363379034771803333, -35.78125000204837391 ) ) ;
#9320=CARTESIAN_POINT ( 'NONE',  ( -5.000000000000003553, -8.660254037844383745, -139.0000000000000000 ) ) ;
#9325=CARTESIAN_POINT ( 'NONE',  ( -9.999999999999742428, -5.773502691896402084, -121.1250000000000000 ) ) ;
#9328=EDGE_CURVE ( 'NONE', #17257, #24467, #18284, .T. ) ;
#9331=ADVANCED_FACE ( 'NONE', ( #14691 ), #41012, .F. ) ;
#9339=CARTESIAN_POINT ( 'NONE',  ( -2.293366432827344421E-15, -12.48450537969573659, -136.7187500020483810 ) ) ;
#9340=AXIS2_PLACEMENT_3D ( 'NONE', #38004, #37132, #7579 ) ;
#9341=CARTESIAN_POINT ( 'NONE',  ( 10.81189881249999729, 0.000000000000000000, -142.5312500020483810 ) ) ;
#9343=CARTESIAN_POINT ( 'NONE',  ( -5.405949406250003975, -9.363379034771801557, -148.8437500020483810 ) ) ;
#9344=CARTESIAN_POINT ( 'NONE',  ( -9.999999999999998224, 1.224646799147353059E-15, -150.1250000040967905 ) ) ;
#9346=CARTESIAN_POINT ( 'NONE',  ( 7.070501591499377789E-16, 11.54700538379251284, -166.6249999999999716 ) ) ;
#9349=CARTESIAN_POINT ( 'NONE',  ( -10.81189881249999729, 1.324075727343319199E-15, -65.09375000204836681 ) ) ;
#9350=DIRECTION ( 'NONE',  ( -0.000000000000000000, -0.000000000000000000, -1.000000000000000000 ) ) ;
#9351=CARTESIAN_POINT ( 'NONE',  ( -10.81189881249999907, -6.242252689847864744, -172.9687500020484094 ) ) ;
#9356=CARTESIAN_POINT ( 'NONE',  ( 9.999999999999998224, 0.000000000000000000, -93.49999999999998579 ) ) ;
#9359=CARTESIAN_POINT ( 'NONE',  ( -5.405949406250003975, -9.363379034771801557, -122.0312500020483952 ) ) ;
#9360=CARTESIAN_POINT ( 'NONE',  ( 5.000000000000000000, 8.660254037844385522, -143.1250000040967905 ) ) ;
#9365=CARTESIAN_POINT ( 'NONE',  ( 10.81189881249999551, -6.242252689847874514, -60.15625000204838813 ) ) ;
#9388=CARTESIAN_POINT ( 'NONE',  ( -5.000000000000003553, -8.660254037844383745, -109.3750000040967763 ) ) ;
#9389=CARTESIAN_POINT ( 'NONE',  ( -10.00000000000000000, -5.773502691896251982, -25.12499999999997868 ) ) ;
#9392=CARTESIAN_POINT ( 'NONE',  ( -10.81189881249999907, -6.242252689847864744, -160.9687500020484094 ) ) ;
#9393=CARTESIAN_POINT ( 'NONE',  ( -5.405949406249996869, 9.363379034771805109, -170.3437500020484094 ) ) ;
#9395=( BOUNDED_CURVE ( )  B_SPLINE_CURVE ( 2, ( #31576, #5234, #28332, #41470, #11905, #25100, #38246 ),
 .UNSPECIFIED., .F., .F. ) 
 B_SPLINE_CURVE_WITH_KNOTS ( ( 3, 2, 2, 3 ),
 ( 0.2947761194029852039, 0.2960199004975125336, 0.2972636815920398634, 0.2985074626865671932 ),
 .UNSPECIFIED. ) 
 CURVE ( )  GEOMETRIC_REPRESENTATION_ITEM ( )  RATIONAL_B_SPLINE_CURVE ( ( 0.9999999999999880096, 0.8660254037844506980, 1.000000000000000000, 0.8660254037844387076, 1.000000000000000000, 0.8660254037844327124, 1.000000000000005995 ) ) 
 REPRESENTATION_ITEM ( '' )  );
#9397=CARTESIAN_POINT ( 'NONE',  ( 10.00000000000000000, 5.773502691896255534, -190.8750000000000000 ) ) ;
#9404=CARTESIAN_POINT ( 'NONE',  ( 7.644554776091147741E-16, 12.48450537969573659, -64.15625000204838102 ) ) ;
#9406=CARTESIAN_POINT ( 'NONE',  ( -9.999999999999998224, 5.773502691896259087, -112.3749999999999858 ) ) ;
#9408=CARTESIAN_POINT ( 'NONE',  ( -10.81189881249999729, -6.242252689847864744, -144.6562500020484094 ) ) ;
#9409=CARTESIAN_POINT ( 'NONE',  ( -10.81189881249999907, -6.242252689847864744, -153.6562500020484094 ) ) ;
#9412=CARTESIAN_POINT ( 'NONE',  ( 5.405949406249992428, -9.363379034771808662, -90.09375000204838102 ) ) ;
#9415=CARTESIAN_POINT ( 'NONE',  ( -5.405949406250003975, -9.363379034771801557, -187.8437500020483810 ) ) ;
#9419=CARTESIAN_POINT ( 'NONE',  ( 10.81189881249999551, -6.242252689847874514, -87.15625000204838102 ) ) ;
#9421=CARTESIAN_POINT ( 'NONE',  ( 9.999999999999996447, -5.773502691896262640, -62.50000000409677625 ) ) ;
#9422=CARTESIAN_POINT ( 'NONE',  ( 7.644554776091147741E-16, 12.48450537969573659, -17.46875000204836681 ) ) ;
#9426=CARTESIAN_POINT ( 'NONE',  ( 5.405949406249999534, 9.363379034771803333, -10.28125000204835260 ) ) ;
#9429=CARTESIAN_POINT ( 'NONE',  ( -9.999999999999998224, 1.224646799147353059E-15, -112.6250000040967763 ) ) ;
#9437=EDGE_LOOP ( 'NONE', ( #3905, #15681, #18723, #35615 ) ) ;
#9445=CLOSED_SHELL ( 'NONE', ( #21625, #42060, #16461, #24987, #10367, #10628, #28622, #33494, #17007, #36653, #30049, #38001, #11163, #37755, #1666, #33094, #14950, #17703, #6670, #4067, #21424, #36888, #42276, #33633, #35912, #11701, #18512, #10593, #35026, #10523, #12751, #4942, #21461, #18687, #34137, #28640, #17648, #30291, #34981, #16630, #14054, #8021, #8235, #5903, #11135, #34302, #36614, #34953, #34702, #16710, #28498, #15370, #12110, #19328, #7571, #33815, #40184, #22248, #16413, #29870, #7889, #26496, #15639, #20947, #37585, #10528, #9249, #36249, #24861, #16679, #25577, #12446, #25394, #5071, #25526, #20922, #11438, #22938, #4335, #20102, #36642, #2523, #20900, #3810, #29767, #23122, #36670, #415, #4586, #15674, #26474, #2213, #20778, #28027, #26638, #28140, #2685, #8363, #10902, #32793, #37257, #8018, #39413, #33607, #32168, #9331, #35436, #20768, #20188, #893, #4994, #7152, #36749, #2921, #10544, #5365, #36078, #7274, #27396, #36648, #6464, #27283 ) ) ;
#9449=CARTESIAN_POINT ( 'NONE',  ( -5.405949406249996869, 9.363379034771805109, -155.5312500020484094 ) ) ;
#9451=CARTESIAN_POINT ( 'NONE',  ( -4.999999999999996447, 8.660254037844387298, -178.5000000000000000 ) ) ;
#9455=CARTESIAN_POINT ( 'NONE',  ( -10.81189881249999729, 6.242252689847871849, -80.21875000204838102 ) ) ;
#9456=CARTESIAN_POINT ( 'NONE',  ( -5.405949406249996869, 9.363379034771805109, -88.03125000204838102 ) ) ;
#9459=CARTESIAN_POINT ( 'NONE',  ( -2.293366432827344421E-15, -12.48450537969573659, -166.9062500020484379 ) ) ;
#9460=CARTESIAN_POINT ( 'NONE',  ( -10.81189881249999729, 6.242252689847871849, -180.9062500020484094 ) ) ;
#9461=CARTESIAN_POINT ( 'NONE',  ( 10.00000000000000000, 5.773502691896255534, -156.7500000040967905 ) ) ;
#9463=CARTESIAN_POINT ( 'NONE',  ( -10.81189881249999729, 6.242252689847871849, -9.718750002048361480 ) ) ;
#9464=CARTESIAN_POINT ( 'NONE',  ( -2.293366432827344421E-15, -12.48450537969573659, -112.7187500020483952 ) ) ;
#9466=CARTESIAN_POINT ( 'NONE',  ( 7.644554776091147741E-16, 12.48450537969573659, -13.15625000204836859 ) ) ;
#9468=( BOUNDED_CURVE ( )  B_SPLINE_CURVE ( 2, ( #20274, #17023, #4094, #40121, #17236, #10552, #23737 ),
 .UNSPECIFIED., .F., .F. ) 
 B_SPLINE_CURVE_WITH_KNOTS ( ( 3, 2, 2, 3 ),
 ( 0.4664179104477613191, 0.4676616915422886489, 0.4689054726368160342, 0.4701492537313434195 ),
 .UNSPECIFIED. ) 
 CURVE ( )  GEOMETRIC_REPRESENTATION_ITEM ( )  RATIONAL_B_SPLINE_CURVE ( ( 0.9999999999999880096, 0.8660254037844506980, 1.000000000000000000, 0.8660254037844387076, 1.000000000000000000, 0.8660254037844267172, 1.000000000000011990 ) ) 
 REPRESENTATION_ITEM ( '' )  );
#9470=CARTESIAN_POINT ( 'NONE',  ( 10.81189881249999907, 6.242252689847868297, -106.4062500020483952 ) ) ;
#9472=ORIENTED_EDGE ( 'NONE', *, *, #36192, .T. ) ;
#9474=CARTESIAN_POINT ( 'NONE',  ( 9.999999999999998224, 0.000000000000000000, -83.37500000409677625 ) ) ;
#9476=CARTESIAN_POINT ( 'NONE',  ( 7.644554776091147741E-16, 12.48450537969573659, -45.96875000204836681 ) ) ;
#9480=CARTESIAN_POINT ( 'NONE',  ( 9.999999999999996447, -5.773502691896262640, -13.00000000409676204 ) ) ;
#9481=CARTESIAN_POINT ( 'NONE',  ( 0.000000000000000000, 0.000000000000000000, -169.9999999999999716 ) ) ;
#9494=CARTESIAN_POINT ( 'NONE',  ( -9.999999999999998224, 1.224646799147353059E-15, -127.6250000040967620 ) ) ;
#9495=CARTESIAN_POINT ( 'NONE',  ( 5.405949406249999534, 9.363379034771803333, -179.7812500020484094 ) ) ;
#9499=CARTESIAN_POINT ( 'NONE',  ( 5.405949406249992428, -9.363379034771808662, -99.09375000204838102 ) ) ;
#9501=CARTESIAN_POINT ( 'NONE',  ( 5.405949406249992428, -9.363379034771808662, -109.7812500020483810 ) ) ;
#9503=CARTESIAN_POINT ( 'NONE',  ( 5.405949406249992428, -9.363379034771808662, -117.0937500020483810 ) ) ;
#9505=( BOUNDED_CURVE ( )  B_SPLINE_CURVE ( 2, ( #28216, #1888, #4904, #14371, #21515, #34482, #31028 ),
 .UNSPECIFIED., .F., .F. ) 
 B_SPLINE_CURVE_WITH_KNOTS ( ( 3, 2, 2, 3 ),
 ( 0.1940298507462686894, 0.1952736318407960470, 0.1965174129353234322, 0.1977611940298507898 ),
 .UNSPECIFIED. ) 
 CURVE ( )  GEOMETRIC_REPRESENTATION_ITEM ( )  RATIONAL_B_SPLINE_CURVE ( ( 0.9999999999999970024, 0.8660254037844417052, 1.000000000000000000, 0.8660254037844387076, 1.000000000000000000, 0.8660254037844327124, 1.000000000000005995 ) ) 
 REPRESENTATION_ITEM ( '' )  );
#9507=CARTESIAN_POINT ( 'NONE',  ( 7.070501591499377789E-16, 11.54700538379251284, -136.6250000000000000 ) ) ;
#9508=CARTESIAN_POINT ( 'NONE',  ( 5.000000000000000000, 8.660254037844385522, -4.749999999999976907 ) ) ;
#9511=CARTESIAN_POINT ( 'NONE',  ( -5.000000000000003553, -8.660254037844383745, -176.8750000040967905 ) ) ;
#9514=CARTESIAN_POINT ( 'NONE',  ( -10.81189881249999907, -6.242252689847864744, -30.46875000204835260 ) ) ;
#9516=CARTESIAN_POINT ( 'NONE',  ( -10.81189881249999729, 6.242252689847871849, -138.7187500020483810 ) ) ;
#9519=CARTESIAN_POINT ( 'NONE',  ( -4.999999999999996447, 8.660254037844387298, -65.99999999999997158 ) ) ;
#9520=CARTESIAN_POINT ( 'NONE',  ( -10.81189881249999729, 1.324075727343319199E-15, -129.7812500020483810 ) ) ;
#9524=CARTESIAN_POINT ( 'NONE',  ( 9.999999999999998224, 0.000000000000000000, -111.8750000040967763 ) ) ;
#9526=CARTESIAN_POINT ( 'NONE',  ( -5.405949406249996869, 9.363379034771805109, -66.84375000204836681 ) ) ;
#9532=CARTESIAN_POINT ( 'NONE',  ( -4.999999999999996447, 8.660254037844387298, -45.37500000409677625 ) ) ;
#9533=CARTESIAN_POINT ( 'NONE',  ( 10.81189881249999729, 0.000000000000000000, -37.53125000204838102 ) ) ;
#9539=VERTEX_POINT ( 'NONE', #38862 ) ;
#9548=CARTESIAN_POINT ( 'NONE',  ( 5.405949406249999534, 9.363379034771803333, -124.0937500020483952 ) ) ;
#9549=CARTESIAN_POINT ( 'NONE',  ( -10.81189881249999907, -6.242252689847864744, -129.6562500020483810 ) ) ;
#9551=CARTESIAN_POINT ( 'NONE',  ( -10.81189881249999729, 6.242252689847871849, -149.2187500020484379 ) ) ;
#9554=CARTESIAN_POINT ( 'NONE',  ( -2.121150477449813534E-15, -11.54700538379251284, -165.8750000000000000 ) ) ;
#9558=CARTESIAN_POINT ( 'NONE',  ( 7.644554776091147741E-16, 12.48450537969573659, -50.46875000204836681 ) ) ;
#9559=CYLINDRICAL_SURFACE ( 'NONE', #2017, 9.999999999999998224 ) ;
#9560=CARTESIAN_POINT ( 'NONE',  ( 10.81189881249999551, -6.242252689847874514, -160.4687500020484094 ) ) ;
#9565=CARTESIAN_POINT ( 'NONE',  ( 7.070501591499377789E-16, 11.54700538379251284, -91.62500000000000000 ) ) ;
#9567=CARTESIAN_POINT ( 'NONE',  ( 5.405949406249999534, 9.363379034771803333, -118.2812500020483952 ) ) ;
#9568=CARTESIAN_POINT ( 'NONE',  ( -5.000000000000003553, -8.660254037844383745, -142.3750000040967905 ) ) ;
#9573=CARTESIAN_POINT ( 'NONE',  ( 10.81189881249999551, -6.242252689847874514, -57.15625000204837391 ) ) ;
#9578=CARTESIAN_POINT ( 'NONE',  ( 9.999999999999998224, 0.000000000000000000, -167.3750000040967905 ) ) ;
#9594=CARTESIAN_POINT ( 'NONE',  ( 7.070501591499377789E-16, 11.54700538379251284, -28.62499999999998224 ) ) ;
#9598=CARTESIAN_POINT ( 'NONE',  ( 5.405949406249992428, -9.363379034771808662, -153.0937500020483810 ) ) ;
#9599=CARTESIAN_POINT ( 'NONE',  ( -2.293366432827344421E-15, -12.48450537969573659, -171.2187500020483810 ) ) ;
#9600=CARTESIAN_POINT ( 'NONE',  ( 9.999999999999998224, 0.000000000000000000, -107.3750000040967763 ) ) ;
#9602=CARTESIAN_POINT ( 'NONE',  ( 7.070501591499377789E-16, 11.54700538379251284, -187.6250000000000284 ) ) ;
#9608=CARTESIAN_POINT ( 'NONE',  ( -5.405949406250003975, -9.363379034771801557, -187.8437500020483810 ) ) ;
#9610=CARTESIAN_POINT ( 'NONE',  ( -10.81189881249999729, 1.324075727343319199E-15, -57.78125000204836681 ) ) ;
#9612=CARTESIAN_POINT ( 'NONE',  ( 9.999999999999998224, 0.000000000000000000, -119.0000000000000000 ) ) ;
#9614=VECTOR ( 'NONE', #20125, 1000.000000000000000 ) ;
#9615=CARTESIAN_POINT ( 'NONE',  ( 5.405949406249992428, -9.363379034771808662, -144.2812500020483810 ) ) ;
#9616=CARTESIAN_POINT ( 'NONE',  ( -10.81189881249999907, -6.242252689847864744, -159.6562500020484094 ) ) ;
#9620=CARTESIAN_POINT ( 'NONE',  ( 5.405949406249992428, -9.363379034771808662, -91.59375000204838102 ) ) ;
#9621=ORIENTED_EDGE ( 'NONE', *, *, #17219, .T. ) ;
#9623=CARTESIAN_POINT ( 'NONE',  ( -5.405949406249996869, 9.363379034771805109, -188.3437500020483810 ) ) ;
#9626=CARTESIAN_POINT ( 'NONE',  ( -9.999999999999998224, 1.224646799147353059E-15, -139.6250000040967905 ) ) ;
#9627=CARTESIAN_POINT ( 'NONE',  ( -10.81189881249999729, 6.242252689847871849, -83.40625000204836681 ) ) ;
#9630=CARTESIAN_POINT ( 'NONE',  ( -9.999999999999998224, 1.224646799147353059E-15, -63.12500000409676204 ) ) ;
#9631=CARTESIAN_POINT ( 'NONE',  ( 5.405949406249999534, 9.363379034771803333, -20.59375000204835615 ) ) ;
#9634=CARTESIAN_POINT ( 'NONE',  ( -5.405949406250003975, -9.363379034771801557, -9.531250002048352599 ) ) ;
#9645=CARTESIAN_POINT ( 'NONE',  ( 9.999999999999998224, 0.000000000000000000, -159.8750000040967905 ) ) ;
#9646=CARTESIAN_POINT ( 'NONE',  ( -9.999999999999998224, 1.224646799147353059E-15, -154.2500000000000000 ) ) ;
#9648=EDGE_LOOP ( 'NONE', ( #7148, #1482, #5785, #24717 ) ) ;
#9657=CARTESIAN_POINT ( 'NONE',  ( 9.999999999999998224, 0.000000000000000000, -173.0000000000000284 ) ) ;
#9658=CARTESIAN_POINT ( 'NONE',  ( -10.81189881249999729, 1.324075727343319199E-15, -156.7812500020484094 ) ) ;
#9665=CARTESIAN_POINT ( 'NONE',  ( 5.405949406249992428, -9.363379034771808662, -76.59375000204838102 ) ) ;
#9666=CARTESIAN_POINT ( 'NONE',  ( -2.293366432827344421E-15, -12.48450537969573659, -85.90625000204839523 ) ) ;
#9669=CARTESIAN_POINT ( 'NONE',  ( -10.81189881249999729, 1.324075727343319199E-15, -170.2812500020484094 ) ) ;
#9670=CARTESIAN_POINT ( 'NONE',  ( -2.293366432827344421E-15, -12.48450537969573659, -177.4062500020483810 ) ) ;
#9671=CARTESIAN_POINT ( 'NONE',  ( -9.999999999999998224, 1.224646799147353059E-15, -157.6250000040967905 ) ) ;
#9672=CYLINDRICAL_SURFACE ( 'NONE', #33939, 9.999999999999998224 ) ;
#9673=CARTESIAN_POINT ( 'NONE',  ( 5.405949406249999534, 9.363379034771803333, -5.593750002048370362 ) ) ;
#9675=CARTESIAN_POINT ( 'NONE',  ( -5.405949406250003975, -9.363379034771801557, -115.8437500020483810 ) ) ;
#9677=CARTESIAN_POINT ( 'NONE',  ( 10.81189881249999729, 0.000000000000000000, -15.03125000204835793 ) ) ;
#9679=CARTESIAN_POINT ( 'NONE',  ( 9.999999999999998224, 0.000000000000000000, -170.3750000040968189 ) ) ;
#9680=CARTESIAN_POINT ( 'NONE',  ( -5.405949406250003975, -9.363379034771801557, -110.0312500020483810 ) ) ;
#9683=CARTESIAN_POINT ( 'NONE',  ( -5.000000000000003553, -8.660254037844383745, -86.87500000409677625 ) ) ;
#9684=CARTESIAN_POINT ( 'NONE',  ( -5.405949406249996869, 9.363379034771805109, -38.34375000204837391 ) ) ;
#9685=EDGE_LOOP ( 'NONE', ( #34773, #25054, #14933, #23337 ) ) ;
#9688=CARTESIAN_POINT ( 'NONE',  ( -9.999999999999998224, 5.773502691896259087, -9.250000004096760264 ) ) ;
#9691=ORIENTED_EDGE ( 'NONE', *, *, #24327, .T. ) ;
#9698=ORIENTED_EDGE ( 'NONE', *, *, #11181, .T. ) ;
#9700=CARTESIAN_POINT ( 'NONE',  ( 0.000000000000000000, 0.000000000000000000, -99.99999999999998579 ) ) ;
#9702=CARTESIAN_POINT ( 'NONE',  ( -5.405949406250003975, -9.363379034771801557, -182.0312500020483810 ) ) ;
#9706=( BOUNDED_CURVE ( )  B_SPLINE_CURVE ( 2, ( #8767, #8976, #21923, #22143, #35317, #5746, #18899 ),
 .UNSPECIFIED., .F., .F. ) 
 B_SPLINE_CURVE_WITH_KNOTS ( ( 3, 2, 2, 3 ),
 ( 0.3358208955223880854, 0.3370646766169154707, 0.3383084577114429670, 0.3395522388059703522 ),
 .UNSPECIFIED. ) 
 CURVE ( )  GEOMETRIC_REPRESENTATION_ITEM ( )  RATIONAL_B_SPLINE_CURVE ( ( 1.000000000000000000, 0.8660254037844387076, 1.000000000000000000, 0.8660254037844387076, 1.000000000000000000, 0.8660254037844148378, 1.000000000000023981 ) ) 
 REPRESENTATION_ITEM ( '' )  );
#9707=CARTESIAN_POINT ( 'NONE',  ( 5.405949406249999534, 9.363379034771803333, -101.5937500020483810 ) ) ;
#9708=CARTESIAN_POINT ( 'NONE',  ( -2.293366432827344421E-15, -12.48450537969573659, -105.4062500020483810 ) ) ;
#9710=CARTESIAN_POINT ( 'NONE',  ( 7.644554776091147741E-16, 12.48450537969573659, -111.9687500020483668 ) ) ;
#9713=CARTESIAN_POINT ( 'NONE',  ( -5.000000000000003553, -8.660254037844383745, -142.0000000000000000 ) ) ;
#9714=CARTESIAN_POINT ( 'NONE',  ( 7.070501591499377789E-16, 11.54700538379251284, -4.624999999999963585 ) ) ;
#9717=CARTESIAN_POINT ( 'NONE',  ( -4.999999999999996447, 8.660254037844387298, -180.3750000040967905 ) ) ;
#9719=CARTESIAN_POINT ( 'NONE',  ( -2.293366432827344421E-15, -12.48450537969573659, -33.21875000204835260 ) ) ;
#9721=CARTESIAN_POINT ( 'NONE',  ( 10.81189881249999551, -6.242252689847874514, -139.4687500020483810 ) ) ;
#9724=CARTESIAN_POINT ( 'NONE',  ( -2.121150477449813534E-15, -11.54700538379251284, -71.37500000000000000 ) ) ;
#9725=CARTESIAN_POINT ( 'NONE',  ( 5.405949406249992428, -9.363379034771808662, -135.2812500020483810 ) ) ;
#9727=EDGE_CURVE ( 'NONE', #31328, #15306, #31806, .T. ) ;
#9731=CARTESIAN_POINT ( 'NONE',  ( 7.070501591499377789E-16, 11.54700538379251284, -108.5000000040967763 ) ) ;
#9732=CARTESIAN_POINT ( 'NONE',  ( -4.999999999999996447, 8.660254037844387298, -162.0000000000000000 ) ) ;
#9733=CARTESIAN_POINT ( 'NONE',  ( 10.81189881249999729, 0.000000000000000000, -65.84375000204836681 ) ) ;
#9740=CARTESIAN_POINT ( 'NONE',  ( 10.00000000000000000, 5.773502691896255534, -33.75000000409675494 ) ) ;
#9741=CYLINDRICAL_SURFACE ( 'NONE', #36240, 9.999999999999998224 ) ;
#9749=DIRECTION ( 'NONE',  ( -0.000000000000000000, -0.000000000000000000, -1.000000000000000000 ) ) ;
#9758=CARTESIAN_POINT ( 'NONE',  ( 5.405949406249999534, 9.363379034771803333, -125.5937500020483668 ) ) ;
#9759=CARTESIAN_POINT ( 'NONE',  ( 5.405949406249999534, 9.363379034771803333, -131.7812500020483810 ) ) ;
#9761=CARTESIAN_POINT ( 'NONE',  ( 10.81189881249999729, 6.242252689847867408, -134.7187500020483810 ) ) ;
#9764=CARTESIAN_POINT ( 'NONE',  ( 7.070501591499377789E-16, 11.54700538379251284, -162.1250000000000284 ) ) ;
#9765=CARTESIAN_POINT ( 'NONE',  ( 7.644554776091147741E-16, 12.48450537969573659, -1.156250002048359038 ) ) ;
#9769=CARTESIAN_POINT ( 'NONE',  ( 7.644554776091147741E-16, 12.48450537969573659, -53.46875000204836681 ) ) ;
#9771=CARTESIAN_POINT ( 'NONE',  ( -5.405949406249996869, 9.363379034771805109, -158.3437500020483810 ) ) ;
#9776=CARTESIAN_POINT ( 'NONE',  ( -5.000000000000003553, -8.660254037844383745, -87.99999999999998579 ) ) ;
#9778=CARTESIAN_POINT ( 'NONE',  ( 5.405949406249992428, -9.363379034771808662, -117.2812500020483952 ) ) ;
#9779=CARTESIAN_POINT ( 'NONE',  ( -10.00000000000000000, -5.773502691896251982, -133.5000000040967905 ) ) ;
#9785=CARTESIAN_POINT ( 'NONE',  ( -10.81189881249999907, -6.242252689847864744, -57.65625000204838102 ) ) ;
#9786=AXIS2_PLACEMENT_3D ( 'NONE', #40377, #24012, #1347 ) ;
#9791=CARTESIAN_POINT ( 'NONE',  ( 7.070501591499376803E-16, 11.54700538379251284, -174.1250000000000000 ) ) ;
#9792=ORIENTED_EDGE ( 'NONE', *, *, #17580, .F. ) ;
#9796=ORIENTED_EDGE ( 'NONE', *, *, #39140, .F. ) ;
#9798=ORIENTED_EDGE ( 'NONE', *, *, #15572, .T. ) ;
#9799=ORIENTED_EDGE ( 'NONE', *, *, #23824, .F. ) ;
#9804=CARTESIAN_POINT ( 'NONE',  ( -9.999999999999998224, 1.224646799147353059E-15, -29.74999999999997158 ) ) ;
#9807=CARTESIAN_POINT ( 'NONE',  ( -10.81189881249999729, 1.324075727343319199E-15, -150.5937500020483810 ) ) ;
#9809=CARTESIAN_POINT ( 'NONE',  ( -5.405949406249996869, 9.363379034771805109, -161.3437500020484094 ) ) ;
#9810=CARTESIAN_POINT ( 'NONE',  ( -5.000000000000003553, -8.660254037844383745, -161.8750000040967905 ) ) ;
#9811=CARTESIAN_POINT ( 'NONE',  ( 5.000000000000000000, 8.660254037844385522, -184.7500000000000000 ) ) ;
#9815=CARTESIAN_POINT ( 'NONE',  ( 10.81189881249999729, 0.000000000000000000, -185.8437500020483810 ) ) ;
#9817=CARTESIAN_POINT ( 'NONE',  ( 5.405949406249992428, -9.363379034771808662, -63.28125000204837391 ) ) ;
#9819=CARTESIAN_POINT ( 'NONE',  ( -5.000000000000003553, -8.660254037844383745, -118.0000000000000000 ) ) ;
#9820=ORIENTED_EDGE ( 'NONE', *, *, #385, .F. ) ;
#9821=CARTESIAN_POINT ( 'NONE',  ( 5.405949406249992428, -9.363379034771808662, -145.7812500020483810 ) ) ;
#9822=CARTESIAN_POINT ( 'NONE',  ( -2.293366432827344421E-15, -12.48450537969573659, -154.9062500020483810 ) ) ;
#9825=CARTESIAN_POINT ( 'NONE',  ( 10.81189881249999907, 6.242252689847868297, -88.21875000204838102 ) ) ;
#9826=VERTEX_POINT ( 'NONE', #23529 ) ;
#9828=CARTESIAN_POINT ( 'NONE',  ( 10.81189881249999729, 0.000000000000000000, -185.8437500020483810 ) ) ;
#9832=CARTESIAN_POINT ( 'NONE',  ( -9.999999999999998224, 1.224646799147353059E-15, -118.6250000040967905 ) ) ;
#9835=CARTESIAN_POINT ( 'NONE',  ( 10.81189881249999551, -6.242252689847874514, -84.15625000204838102 ) ) ;
#9838=CARTESIAN_POINT ( 'NONE',  ( -2.121150477449813534E-15, -11.54700538379251284, -62.75000000409677625 ) ) ;
#9839=CARTESIAN_POINT ( 'NONE',  ( 10.81189881249999551, -6.242252689847874514, -16.46875000204836681 ) ) ;
#9842=CARTESIAN_POINT ( 'NONE',  ( -5.405949406249996869, 9.363379034771805109, -10.03125000204835260 ) ) ;
#9851=VERTEX_POINT ( 'NONE', #33251 ) ;
#9853=EDGE_CURVE ( 'NONE', #4202, #35880, #9468, .T. ) ;
#9854=CARTESIAN_POINT ( 'NONE',  ( -5.405949406249996869, 9.363379034771805109, -101.3437500020483810 ) ) ;
#9862=LINE ( 'NONE', #3821, #5683 ) ;
#9865=DIRECTION ( 'NONE',  ( -0.000000000000000000, -0.000000000000000000, -1.000000000000000000 ) ) ;
#9866=CARTESIAN_POINT ( 'NONE',  ( -2.293366432827344421E-15, -12.48450537969573659, -154.9062500020483810 ) ) ;
#9873=CARTESIAN_POINT ( 'NONE',  ( 10.81189881249999907, 6.242252689847868297, -74.71875000204838102 ) ) ;
#9874=CARTESIAN_POINT ( 'NONE',  ( -10.81189881249999907, -6.242252689847864744, -84.65625000204836681 ) ) ;
#9878=CARTESIAN_POINT ( 'NONE',  ( -5.405949406249996869, 9.363379034771805109, -169.0312500020484094 ) ) ;
#9879=CARTESIAN_POINT ( 'NONE',  ( 10.81189881249999907, 6.242252689847868297, -179.9062500020484094 ) ) ;
#9880=CARTESIAN_POINT ( 'NONE',  ( 7.070501591499377789E-16, 11.54700538379251284, -156.5000000040968189 ) ) ;
#9881=CARTESIAN_POINT ( 'NONE',  ( -9.999999999999998224, 0.000000000000000000, -99.99999999999998579 ) ) ;
#9882=CARTESIAN_POINT ( 'NONE',  ( 5.405949406249992428, -9.363379034771808662, -3.093750002048367698 ) ) ;
#9884=CARTESIAN_POINT ( 'NONE',  ( 5.405949406249999534, 9.363379034771803333, -116.5937500020483810 ) ) ;
#9886=CARTESIAN_POINT ( 'NONE',  ( 10.81189881249999907, 6.242252689847868297, -10.40625000204836859 ) ) ;
#9888=CARTESIAN_POINT ( 'NONE',  ( -10.00000000000000000, -5.773502691896252870, -171.0000000040967905 ) ) ;
#9889=CARTESIAN_POINT ( 'NONE',  ( 5.405949406249992428, -9.363379034771808662, -106.7812500020483810 ) ) ;
#9891=ORIENTED_EDGE ( 'NONE', *, *, #30774, .T. ) ;
#9892=CARTESIAN_POINT ( 'NONE',  ( -2.121150477449813534E-15, -11.54700538379251284, -86.75000000409677625 ) ) ;
#9894=CARTESIAN_POINT ( 'NONE',  ( 10.81189881249999907, 6.242252689847868297, -44.71875000204835970 ) ) ;
#9895=VERTEX_POINT ( 'NONE', #38175 ) ;
#9898=CARTESIAN_POINT ( 'NONE',  ( 5.000000000000000000, 8.660254037844385522, -139.7499999999999716 ) ) ;
#9899=CARTESIAN_POINT ( 'NONE',  ( -9.999999999999998224, 1.224646799147353059E-15, -12.12500000409674783 ) ) ;
#9912=CARTESIAN_POINT ( 'NONE',  ( -5.405949406250003975, -9.363379034771801557, -179.0312500020483810 ) ) ;
#9916=CARTESIAN_POINT ( 'NONE',  ( 5.405949406249992428, -9.363379034771808662, -100.5937500020483810 ) ) ;
#9917=CARTESIAN_POINT ( 'NONE',  ( -9.999999999999479527, -5.773502691896549521, -143.6250000000000000 ) ) ;
#9918=CARTESIAN_POINT ( 'NONE',  ( -5.405949406249996869, 9.363379034771805109, -107.5312500020483810 ) ) ;
#9920=CARTESIAN_POINT ( 'NONE',  ( -10.81189881249999729, 1.324075727343319199E-15, -114.5937500020483810 ) ) ;
#9922=CARTESIAN_POINT ( 'NONE',  ( 9.999999999999998224, 0.000000000000000000, -141.5000000000000000 ) ) ;
#9923=CARTESIAN_POINT ( 'NONE',  ( -2.121150477449813534E-15, -11.54700538379251284, -6.874999999999964473 ) ) ;
#9926=CARTESIAN_POINT ( 'NONE',  ( -9.999999999999998224, 1.224646799147353059E-15, -178.6250000040968189 ) ) ;
#9928=CARTESIAN_POINT ( 'NONE',  ( -10.81189881249999907, -6.242252689847864744, -33.46875000204835260 ) ) ;
#9929=CARTESIAN_POINT ( 'NONE',  ( 9.999999999999998224, 0.000000000000000000, -107.3750000040967763 ) ) ;
#9930=CARTESIAN_POINT ( 'NONE',  ( -10.81189881249999907, -6.242252689847864744, -138.4687500020484094 ) ) ;
#9932=CARTESIAN_POINT ( 'NONE',  ( -5.405949406250003975, -9.363379034771801557, -39.53125000204838102 ) ) ;
#9934=CARTESIAN_POINT ( 'NONE',  ( -5.000000000000003553, -8.660254037844383745, -69.99999999999998579 ) ) ;
#9935=CARTESIAN_POINT ( 'NONE',  ( 7.644554776091147741E-16, 12.48450537969573659, -130.1562500020483810 ) ) ;
#9939=CARTESIAN_POINT ( 'NONE',  ( 4.999999999999992006, -8.660254037844389075, -109.1250000040967763 ) ) ;
#9940=CARTESIAN_POINT ( 'NONE',  ( 5.405949406249992428, -9.363379034771808662, -67.59375000204836681 ) ) ;
#9946=CARTESIAN_POINT ( 'NONE',  ( -9.999999999999998224, 1.224646799147353059E-15, -37.62500000409676915 ) ) ;
#9953=VERTEX_POINT ( 'NONE', #37533 ) ;
#9956=EDGE_CURVE ( 'NONE', #34592, #1591, #25490, .T. ) ;
#9964=CARTESIAN_POINT ( 'NONE',  ( -10.81189881249999729, 6.242252689847871849, -128.2187500020483810 ) ) ;
#9965=CARTESIAN_POINT ( 'NONE',  ( -2.293366432827344421E-15, -12.48450537969573659, -130.9062500020483810 ) ) ;
#9967=CARTESIAN_POINT ( 'NONE',  ( -10.81189881249999729, -6.242252689847864744, -141.4687500020483810 ) ) ;
#9970=CARTESIAN_POINT ( 'NONE',  ( 4.999999999999992006, -8.660254037844389075, -162.7500000000000000 ) ) ;
#9974=CARTESIAN_POINT ( 'NONE',  ( -5.405949406249996869, 9.363379034771805109, -53.34375000204835970 ) ) ;
#9975=DIRECTION ( 'NONE',  ( -0.000000000000000000, -0.000000000000000000, -1.000000000000000000 ) ) ;
#9976=CARTESIAN_POINT ( 'NONE',  ( -5.405949406250003975, -9.363379034771801557, -165.3437500020484094 ) ) ;
#9981=CARTESIAN_POINT ( 'NONE',  ( 7.070501591499377789E-16, 11.54700538379251284, -94.62499999999997158 ) ) ;
#9983=CARTESIAN_POINT ( 'NONE',  ( 5.405949406249992428, -9.363379034771808662, -114.2812500020483952 ) ) ;
#9984=CARTESIAN_POINT ( 'NONE',  ( -5.000000000000003553, -8.660254037844383745, -128.8750000040967905 ) ) ;
#9989=CARTESIAN_POINT ( 'NONE',  ( 5.405949406249999534, 9.363379034771803333, -59.78125000204836681 ) ) ;
#9994=CARTESIAN_POINT ( 'NONE',  ( 7.070501591499376803E-16, 11.54700538379251284, -171.5000000040967905 ) ) ;
#9999=ORIENTED_EDGE ( 'NONE', *, *, #20684, .T. ) ;
#10007=( BOUNDED_CURVE ( )  B_SPLINE_CURVE ( 2, ( #33287, #15834, #29034, #3712, #30040, #39944, #14678 ),
 .UNSPECIFIED., .F., .F. ) 
 B_SPLINE_CURVE_WITH_KNOTS ( ( 3, 2, 2, 3 ),
 ( 0.3582089552238806873, 0.3594527363184080726, 0.3606965174129355134, 0.3619402985074628432 ),
 .UNSPECIFIED. ) 
 CURVE ( )  GEOMETRIC_REPRESENTATION_ITEM ( )  RATIONAL_B_SPLINE_CURVE ( ( 0.9999999999999880096, 0.8660254037844506980, 1.000000000000000000, 0.8660254037844387076, 1.000000000000000000, 0.8660254037844207220, 1.000000000000017986 ) ) 
 REPRESENTATION_ITEM ( '' )  );
#10009=CARTESIAN_POINT ( 'NONE',  ( -5.000000000000003553, -8.660254037844383745, -134.5000000000000000 ) ) ;
#10011=CARTESIAN_POINT ( 'NONE',  ( 5.000000000000000000, 8.660254037844385522, -27.24999999999996803 ) ) ;
#10015=CARTESIAN_POINT ( 'NONE',  ( 10.81189881249999729, 0.000000000000000000, -149.8437500020483810 ) ) ;
#10016=CARTESIAN_POINT ( 'NONE',  ( 5.405949406249992428, -9.363379034771808662, -165.0937500020484094 ) ) ;
#10018=CARTESIAN_POINT ( 'NONE',  ( 9.999999999999998224, 0.000000000000000000, -102.8750000040967763 ) ) ;
#10019=CARTESIAN_POINT ( 'NONE',  ( -9.999999999999998224, 1.224646799147353059E-15, -187.2500000000000000 ) ) ;
#10021=CARTESIAN_POINT ( 'NONE',  ( 9.999999999999998224, 0.000000000000000000, -152.0000000000000000 ) ) ;
#10023=CARTESIAN_POINT ( 'NONE',  ( 10.81189881249999729, 0.000000000000000000, -188.8437500020483810 ) ) ;
#10026=CARTESIAN_POINT ( 'NONE',  ( -5.405949406250003975, -9.363379034771801557, -53.03125000204836681 ) ) ;
#10028=CARTESIAN_POINT ( 'NONE',  ( -4.999999999999996447, 8.660254037844387298, -117.0000000000000000 ) ) ;
#10030=CARTESIAN_POINT ( 'NONE',  ( 10.81189881249999729, 6.242252689847867408, -133.4062500020483810 ) ) ;
#10031=CARTESIAN_POINT ( 'NONE',  ( -5.405949406250003975, -9.363379034771801557, -146.0312500020483810 ) ) ;
#10034=CARTESIAN_POINT ( 'NONE',  ( -10.81189881249999729, 1.324075727343319199E-15, -86.09375000204836681 ) ) ;
#10037=CARTESIAN_POINT ( 'NONE',  ( -5.405949406249996869, 9.363379034771805109, -185.3437500020483810 ) ) ;
#10041=CARTESIAN_POINT ( 'NONE',  ( -10.81189881249999729, 6.242252689847871849, -87.90625000204838102 ) ) ;
#10045=CARTESIAN_POINT ( 'NONE',  ( -2.121150477449813534E-15, -11.54700538379251284, -61.25000000409677625 ) ) ;
#10046=CARTESIAN_POINT ( 'NONE',  ( -2.293366432827344421E-15, -12.48450537969573659, -19.71875000204837036 ) ) ;
#10049=CARTESIAN_POINT ( 'NONE',  ( 5.405949406249992428, -9.363379034771808662, -10.78125000204835438 ) ) ;
#10051=CARTESIAN_POINT ( 'NONE',  ( -4.999999999999996447, 8.660254037844387298, -175.8750000040967905 ) ) ;
#10054=CARTESIAN_POINT ( 'NONE',  ( -9.999999999999227285, -5.773502691896698735, -135.0000000040967620 ) ) ;
#10059=ORIENTED_EDGE ( 'NONE', *, *, #24680, .F. ) ;
#10061=CARTESIAN_POINT ( 'NONE',  ( -10.81189881249999729, -6.242252689847864744, -102.4687500020483810 ) ) ;
#10075=CARTESIAN_POINT ( 'NONE',  ( 7.070501591499376803E-16, 11.54700538379251284, -172.6249999999999716 ) ) ;
#10076=CARTESIAN_POINT ( 'NONE',  ( -10.81189881249999729, 1.324075727343319199E-15, -152.2812500020484094 ) ) ;
#10082=CARTESIAN_POINT ( 'NONE',  ( -5.405949406250003975, -9.363379034771801557, -81.34375000204838102 ) ) ;
#10083=CARTESIAN_POINT ( 'NONE',  ( 5.405949406249999534, 9.363379034771803333, -80.78125000204838102 ) ) ;
#10086=CARTESIAN_POINT ( 'NONE',  ( -10.81189881249999729, 1.324075727343319199E-15, -167.2812500020484094 ) ) ;
#10087=CARTESIAN_POINT ( 'NONE',  ( -2.293366432827344421E-15, -12.48450537969573659, -181.9062500020483810 ) ) ;
#10088=CARTESIAN_POINT ( 'NONE',  ( 9.999999999999998224, 1.224646799147353059E-15, -99.99999999999998579 ) ) ;
#10089=CARTESIAN_POINT ( 'NONE',  ( -10.81189881249999729, 1.324075727343319199E-15, -6.593750002048370362 ) ) ;
#10090=CARTESIAN_POINT ( 'NONE',  ( 10.81189881249999729, 0.000000000000000000, -115.3437500020483810 ) ) ;
#10092=CARTESIAN_POINT ( 'NONE',  ( 10.81189881249999729, 0.000000000000000000, -10.53125000204835260 ) ) ;
#10095=DIRECTION ( 'NONE',  ( -1.000000000000000000, 0.000000000000000000, 0.000000000000000000 ) ) ;
#10096=CARTESIAN_POINT ( 'NONE',  ( 10.81189881249999907, 6.242252689847868297, -109.4062500020483952 ) ) ;
#10099=CARTESIAN_POINT ( 'NONE',  ( 7.070501591499377789E-16, 11.54700538379251284, -84.50000000409677625 ) ) ;
#10101=CARTESIAN_POINT ( 'NONE',  ( -5.405949406249996869, 9.363379034771805109, -44.34375000204837391 ) ) ;
#10107=CARTESIAN_POINT ( 'NONE',  ( -4.999999999999996447, 8.660254037844387298, -15.37500000409675138 ) ) ;
#10119=ORIENTED_EDGE ( 'NONE', *, *, #7351, .F. ) ;
#10124=CARTESIAN_POINT ( 'NONE',  ( 5.405949406249999534, 9.363379034771803333, -170.7812500020484094 ) ) ;
#10128=CARTESIAN_POINT ( 'NONE',  ( 5.405949406249999534, 9.363379034771803333, -98.59375000204838102 ) ) ;
#10129=CARTESIAN_POINT ( 'NONE',  ( -5.405949406250003975, -9.363379034771801557, -107.0312500020483810 ) ) ;
#10131=CARTESIAN_POINT ( 'NONE',  ( 10.81189881249999551, -6.242252689847874514, -110.9687500020483810 ) ) ;
#10135=CARTESIAN_POINT ( 'NONE',  ( 7.070501591499377789E-16, 11.54700538379251284, -132.1250000000000000 ) ) ;
#10136=CARTESIAN_POINT ( 'NONE',  ( -9.999999999999998224, 5.773502691896259087, -4.374999999999961808 ) ) ;
#10139=CARTESIAN_POINT ( 'NONE',  ( 9.999999999999996447, -5.773502691896262640, -178.0000000040967905 ) ) ;
#10141=CARTESIAN_POINT ( 'NONE',  ( -5.405949406250003975, -9.363379034771801557, -28.84375000204836326 ) ) ;
#10143=CARTESIAN_POINT ( 'NONE',  ( -10.81189881249999907, -6.242252689847864744, -136.9687500020483810 ) ) ;
#10145=CARTESIAN_POINT ( 'NONE',  ( -10.81189881249999907, -6.242252689847864744, -36.65625000204835970 ) ) ;
#10147=CARTESIAN_POINT ( 'NONE',  ( -4.999999999999996447, 8.660254037844387298, -58.49999999999997158 ) ) ;
#10148=CARTESIAN_POINT ( 'NONE',  ( 5.405949406249999534, 9.363379034771803333, -133.2812500020483810 ) ) ;
#10153=CARTESIAN_POINT ( 'NONE',  ( 10.00000000000000000, 5.773502691896255534, -110.2500000040967905 ) ) ;
#10154=CARTESIAN_POINT ( 'NONE',  ( -10.00000000000025580, 5.773502691896109873, -100.7500000040968047 ) ) ;
#10155=CARTESIAN_POINT ( 'NONE',  ( -10.81189881249999729, 1.324075727343319199E-15, -66.59375000204836681 ) ) ;
#10161=CARTESIAN_POINT ( 'NONE',  ( -10.00000000000000000, -5.773502691896251982, -34.50000000409675494 ) ) ;
#10165=ORIENTED_EDGE ( 'NONE', *, *, #26456, .F. ) ;
#10177=CARTESIAN_POINT ( 'NONE',  ( 10.81189881249999729, 0.000000000000000000, -127.3437500020483952 ) ) ;
#10178=CARTESIAN_POINT ( 'NONE',  ( 10.81189881249999907, 6.242252689847868297, -134.9062500020483810 ) ) ;
#10180=CARTESIAN_POINT ( 'NONE',  ( 7.644554776091147741E-16, 12.48450537969573659, -141.9687500020483810 ) ) ;
#10181=CARTESIAN_POINT ( 'NONE',  ( -5.000000000000003553, -8.660254037844383745, -130.0000000000000000 ) ) ;
#10183=CARTESIAN_POINT ( 'NONE',  ( 9.999999999999996447, -5.773502691896262640, -158.1250000000000284 ) ) ;
#10188=CARTESIAN_POINT ( 'NONE',  ( 10.81189881249999729, 0.000000000000000000, -56.84375000204835970 ) ) ;
#10190=CARTESIAN_POINT ( 'NONE',  ( -10.81189881249999907, -6.242252689847864744, -162.4687500020483526 ) ) ;
#10193=DIRECTION ( 'NONE',  ( -1.000000000000000000, 0.000000000000000000, 0.000000000000000000 ) ) ;
#10195=CARTESIAN_POINT ( 'NONE',  ( -9.999999999999998224, 1.224646799147353059E-15, -89.74999999999998579 ) ) ;
#10197=CARTESIAN_POINT ( 'NONE',  ( -10.81189881249999729, 6.242252689847871849, -108.9062500020483810 ) ) ;
#10198=CARTESIAN_POINT ( 'NONE',  ( -10.00000000000000000, -5.773502691896251982, -130.5000000040967905 ) ) ;
#10203=CARTESIAN_POINT ( 'NONE',  ( 10.81189881249999907, 6.242252689847868297, -49.40625000204837391 ) ) ;
#10224=CARTESIAN_POINT ( 'NONE',  ( -5.405949406250003975, -9.363379034771801557, -145.8437500020483810 ) ) ;
#10225=CARTESIAN_POINT ( 'NONE',  ( 10.81189881249999729, 0.000000000000000000, -164.8437500020484094 ) ) ;
#10228=CARTESIAN_POINT ( 'NONE',  ( -5.000000000000003553, -8.660254037844383745, -190.0000000000000000 ) ) ;
#10233=CARTESIAN_POINT ( 'NONE',  ( 10.81189881249999551, -6.242252689847874514, -188.9687500020484094 ) ) ;
#10236=CARTESIAN_POINT ( 'NONE',  ( -2.293366432827344421E-15, -12.48450537969573659, -52.90625000204837391 ) ) ;
#10238=CARTESIAN_POINT ( 'NONE',  ( -9.999999999999998224, 5.773502691896259087, -118.3750000000000000 ) ) ;
#10240=CARTESIAN_POINT ( 'NONE',  ( -2.293366432827344421E-15, -12.48450537969573659, -135.4062500020483810 ) ) ;
#10241=CARTESIAN_POINT ( 'NONE',  ( -5.405949406249996869, 9.363379034771805109, -145.0312500020483810 ) ) ;
#10244=CARTESIAN_POINT ( 'NONE',  ( 7.644554776091147741E-16, 12.48450537969573659, -83.46875000204838102 ) ) ;
#10247=CARTESIAN_POINT ( 'NONE',  ( -10.81189881249999729, 1.324075727343319199E-15, -177.5937500020484094 ) ) ;
#10251=DIRECTION ( 'NONE',  ( -0.000000000000000000, -0.000000000000000000, -1.000000000000000000 ) ) ;
#10252=CARTESIAN_POINT ( 'NONE',  ( -10.81189881249999907, -6.242252689847864744, -80.15625000204839523 ) ) ;
#10255=CARTESIAN_POINT ( 'NONE',  ( -9.999999999999998224, 1.224646799147353059E-15, -54.12500000409675494 ) ) ;
#10256=CARTESIAN_POINT ( 'NONE',  ( 10.81189881249999551, -6.242252689847874514, -7.468750002048357928 ) ) ;
#10257=CARTESIAN_POINT ( 'NONE',  ( 9.999999999999998224, 0.000000000000000000, -177.8750000040967905 ) ) ;
#10259=CARTESIAN_POINT ( 'NONE',  ( 10.81189881249999907, 6.242252689847868297, -8.906250002048366810 ) ) ;
#10261=CARTESIAN_POINT ( 'NONE',  ( 9.999999999999998224, 0.000000000000000000, -176.3750000040967905 ) ) ;
#10277=CARTESIAN_POINT ( 'NONE',  ( -9.999999999999998224, 5.773502691896259087, -41.87499999999997158 ) ) ;
#10283=CARTESIAN_POINT ( 'NONE',  ( 10.81189881249999907, 6.242252689847868297, -148.4062500020484094 ) ) ;
#10287=CARTESIAN_POINT ( 'NONE',  ( 7.070501591499376803E-16, 11.54700538379251284, -141.1250000000000000 ) ) ;
#10290=CARTESIAN_POINT ( 'NONE',  ( 5.405949406249992428, -9.363379034771808662, -73.59375000204838102 ) ) ;
#10291=CARTESIAN_POINT ( 'NONE',  ( 5.405949406249992428, -9.363379034771808662, -73.78125000204838102 ) ) ;
#10293=CARTESIAN_POINT ( 'NONE',  ( 9.999999999999479527, 5.773502691896553074, -115.8749999999999858 ) ) ;
#10294=CARTESIAN_POINT ( 'NONE',  ( -10.81189881249999729, 6.242252689847871849, -158.4062500020483810 ) ) ;
#10295=CARTESIAN_POINT ( 'NONE',  ( 10.81189881249999551, -6.242252689847874514, -172.6562500020484379 ) ) ;
#10296=DIRECTION ( 'NONE',  ( -1.000000000000000000, 0.000000000000000000, 0.000000000000000000 ) ) ;
#10297=CARTESIAN_POINT ( 'NONE',  ( 10.81189881249999551, -6.242252689847874514, 0.03124999795164895566 ) ) ;
#10299=CARTESIAN_POINT ( 'NONE',  ( -10.81189881249999729, 1.324075727343319199E-15, -104.0937500020483810 ) ) ;
#10301=CARTESIAN_POINT ( 'NONE',  ( -5.405949406249996869, 9.363379034771805109, -8.531250002048352599 ) ) ;
#10304=CARTESIAN_POINT ( 'NONE',  ( 10.81189881249999907, 6.242252689847868297, -100.4062500020483952 ) ) ;
#10306=ORIENTED_EDGE ( 'NONE', *, *, #33061, .F. ) ;
#10307=CARTESIAN_POINT ( 'NONE',  ( -9.999999999999998224, 1.224646799147353059E-15, -82.62500000409676204 ) ) ;
#10308=CARTESIAN_POINT ( 'NONE',  ( 7.070501591499376803E-16, 11.54700538379251284, -134.0000000040967905 ) ) ;
#10309=CARTESIAN_POINT ( 'NONE',  ( -10.81189881249999729, 6.242252689847871849, -35.21875000204835260 ) ) ;
#10312=AXIS2_PLACEMENT_3D ( 'NONE', #4442, #27969, #30783 ) ;
#10313=CARTESIAN_POINT ( 'NONE',  ( -10.81189881249999907, -6.242252689847864744, -35.15625000204835970 ) ) ;
#10314=EDGE_CURVE ( 'NONE', #36340, #28518, #5802, .T. ) ;
#10317=CARTESIAN_POINT ( 'NONE',  ( -10.00000000000000000, -5.773502691896251982, -13.50000000409676204 ) ) ;
#10321=ORIENTED_EDGE ( 'NONE', *, *, #27218, .F. ) ;
#10331=CARTESIAN_POINT ( 'NONE',  ( -5.405949406249996869, 9.363379034771805109, -172.0312500020484094 ) ) ;
#10335=CARTESIAN_POINT ( 'NONE',  ( 5.405949406249992428, -9.363379034771808662, -96.09375000204838102 ) ) ;
#10337=CARTESIAN_POINT ( 'NONE',  ( -10.81189881249999729, 1.324075727343319199E-15, -102.7812500020483952 ) ) ;
#10339=CARTESIAN_POINT ( 'NONE',  ( -5.405949406249996869, 9.363379034771805109, -111.8437500020483810 ) ) ;
#10343=CARTESIAN_POINT ( 'NONE',  ( -10.81189881249999907, -6.242252689847864744, -198.6562500020484094 ) ) ;
#10346=CARTESIAN_POINT ( 'NONE',  ( -4.999999999999996447, 8.660254037844387298, -183.3750000040967905 ) ) ;
#10348=CARTESIAN_POINT ( 'NONE',  ( 5.405949406249999534, 9.363379034771803333, -26.59375000204835970 ) ) ;
#10350=CARTESIAN_POINT ( 'NONE',  ( -10.81189881249999729, 6.242252689847871849, -126.7187500020483952 ) ) ;
#10352=CARTESIAN_POINT ( 'NONE',  ( 5.405949406249999534, 9.363379034771803333, -34.28125000204837391 ) ) ;
#10353=CARTESIAN_POINT ( 'NONE',  ( 10.00000000000000000, 5.773502691896255534, -61.87499999999998579 ) ) ;
#10354=CARTESIAN_POINT ( 'NONE',  ( -10.81189881249999729, 1.324075727343319199E-15, -134.2812500020483810 ) ) ;
#10358=CARTESIAN_POINT ( 'NONE',  ( 4.999999999999992006, -8.660254037844389075, -112.1250000040967763 ) ) ;
#10359=CARTESIAN_POINT ( 'NONE',  ( 10.81189881249999729, 0.000000000000000000, -62.84375000204836681 ) ) ;
#10360=ORIENTED_EDGE ( 'NONE', *, *, #4119, .F. ) ;
#10366=CARTESIAN_POINT ( 'NONE',  ( -5.000000000000003553, -8.660254037844383745, -35.87500000409676915 ) ) ;
#10367=ADVANCED_FACE ( 'NONE', ( #24284 ), #3631, .F. ) ;
#10368=CARTESIAN_POINT ( 'NONE',  ( -4.999999999999996447, 8.660254037844387298, -151.8750000040967905 ) ) ;
#10372=ORIENTED_EDGE ( 'NONE', *, *, #24915, .F. ) ;
#10374=ORIENTED_EDGE ( 'NONE', *, *, #26094, .T. ) ;
#10379=CARTESIAN_POINT ( 'NONE',  ( 5.405949406249999534, 9.363379034771803333, -199.2812500020484094 ) ) ;
#10381=CARTESIAN_POINT ( 'NONE',  ( 9.999999999999742428, 5.773502691896404748, -156.7500000040967905 ) ) ;
#10382=CARTESIAN_POINT ( 'NONE',  ( -10.00000000000051337, 5.773502691895962435, -149.8750000000000000 ) ) ;
#10386=CARTESIAN_POINT ( 'NONE',  ( 10.81189881249999729, 0.000000000000000000, -121.3437500020483952 ) ) ;
#10387=CARTESIAN_POINT ( 'NONE',  ( -5.000000000000003553, -8.660254037844383745, -194.8750000040967905 ) ) ;
#10388=CARTESIAN_POINT ( 'NONE',  ( 7.644554776091147741E-16, 12.48450537969573659, -133.1562500020483810 ) ) ;
#10390=CARTESIAN_POINT ( 'NONE',  ( 7.644554776091147741E-16, 12.48450537969573659, -137.4687500020483810 ) ) ;
#10392=CARTESIAN_POINT ( 'NONE',  ( -4.999999999999996447, 8.660254037844387298, -157.5000000000000000 ) ) ;
#10393=CARTESIAN_POINT ( 'NONE',  ( -10.81189881249999907, -6.242252689847864744, -0.6562500020483587049 ) ) ;
#10398=CARTESIAN_POINT ( 'NONE',  ( 7.644554776091147741E-16, 12.48450537969573659, -54.96875000204836681 ) ) ;
#10400=CARTESIAN_POINT ( 'NONE',  ( 7.644554776091147741E-16, 12.48450537969573659, -159.9687500020483810 ) ) ;
#10405=CARTESIAN_POINT ( 'NONE',  ( 7.070501591499377789E-16, 11.54700538379251284, -82.62500000000000000 ) ) ;
#10408=CARTESIAN_POINT ( 'NONE',  ( 7.644554776091147741E-16, 12.48450537969573659, -112.1562500020483952 ) ) ;
#10409=CARTESIAN_POINT ( 'NONE',  ( 7.070501591499377789E-16, 11.54700538379251284, -135.5000000040967905 ) ) ;
#10410=CARTESIAN_POINT ( 'NONE',  ( 10.00000000000044764, -5.773502691896004180, -177.6249999999999716 ) ) ;
#10413=CARTESIAN_POINT ( 'NONE',  ( -10.81189881249999907, -6.242252689847864744, -48.65625000204836681 ) ) ;
#10424=ORIENTED_EDGE ( 'NONE', *, *, #29872, .F. ) ;
#10437=CARTESIAN_POINT ( 'NONE',  ( 5.405949406249999534, 9.363379034771803333, -151.0937500020483810 ) ) ;
#10438=CARTESIAN_POINT ( 'NONE',  ( -10.81189881249999729, 1.324075727343319199E-15, -159.5937500020484094 ) ) ;
#10440=CARTESIAN_POINT ( 'NONE',  ( 0.000000000000000000, 0.000000000000000000, -99.99999999999998579 ) ) ;
#10441=CARTESIAN_POINT ( 'NONE',  ( 5.000000000000000000, 8.660254037844385522, -177.2500000000000284 ) ) ;
#10446=CARTESIAN_POINT ( 'NONE',  ( 5.405949406249999534, 9.363379034771803333, -182.5937500020483810 ) ) ;
#10449=CARTESIAN_POINT ( 'NONE',  ( -10.81189881249999729, 1.324075727343319199E-15, -56.28125000204836681 ) ) ;
#10451=CARTESIAN_POINT ( 'NONE',  ( -9.999999999999998224, 1.224646799147353059E-15, -109.2499999999999858 ) ) ;
#10454=CARTESIAN_POINT ( 'NONE',  ( -5.405949406250003975, -9.363379034771801557, -137.0312500020484094 ) ) ;
#10455=CARTESIAN_POINT ( 'NONE',  ( 5.405949406249992428, -9.363379034771808662, -150.2812500020483810 ) ) ;
#10457=CARTESIAN_POINT ( 'NONE',  ( -5.405949406250003975, -9.363379034771801557, -79.84375000204838102 ) ) ;
#10460=CARTESIAN_POINT ( 'NONE',  ( -10.81189881249999907, -6.242252689847864744, -183.4687500020484379 ) ) ;
#10462=CARTESIAN_POINT ( 'NONE',  ( 9.999999999999998224, 0.000000000000000000, -109.9999999999999858 ) ) ;
#10464=CARTESIAN_POINT ( 'NONE',  ( -10.81189881249999907, -6.242252689847864744, -77.15625000204836681 ) ) ;
#10466=CARTESIAN_POINT ( 'NONE',  ( -9.999999999999998224, 5.773502691896259087, -54.25000000409676915 ) ) ;
#10467=CARTESIAN_POINT ( 'NONE',  ( -5.405949406249996869, 9.363379034771805109, -6.843750002048371250 ) ) ;
#10471=CARTESIAN_POINT ( 'NONE',  ( 10.81189881249999907, 6.242252689847868297, -7.406250002048365033 ) ) ;
#10472=FACE_OUTER_BOUND ( 'NONE', #1427, .T. ) ;
#10474=CYLINDRICAL_SURFACE ( 'NONE', #13481, 9.999999999999998224 ) ;
#10477=EDGE_LOOP ( 'NONE', ( #13499, #30624, #25365, #5091 ) ) ;
#10488=CARTESIAN_POINT ( 'NONE',  ( 9.999999999999998224, 0.000000000000000000, -48.49999999999998579 ) ) ;
#10493=CARTESIAN_POINT ( 'NONE',  ( 9.999999999999998224, 0.000000000000000000, -132.8750000040967905 ) ) ;
#10494=CARTESIAN_POINT ( 'NONE',  ( -10.81189881249999907, -6.242252689847864744, -150.6562500020484094 ) ) ;
#10501=CARTESIAN_POINT ( 'NONE',  ( -2.293366432827344421E-15, -12.48450537969573659, -73.71875000204835260 ) ) ;
#10502=CARTESIAN_POINT ( 'NONE',  ( -10.81189881249999907, -6.242252689847864744, -74.15625000204835260 ) ) ;
#10505=CARTESIAN_POINT ( 'NONE',  ( -5.405949406250003975, -9.363379034771801557, -158.0312500020484094 ) ) ;
#10506=CARTESIAN_POINT ( 'NONE',  ( 5.405949406249999534, 9.363379034771803333, -173.7812500020484094 ) ) ;
#10507=CARTESIAN_POINT ( 'NONE',  ( -9.999999999999998224, 1.224646799147353059E-15, -136.6250000040967620 ) ) ;
#10510=CARTESIAN_POINT ( 'NONE',  ( -10.81189881249999729, 6.242252689847871849, -102.7187500020483810 ) ) ;
#10512=CARTESIAN_POINT ( 'NONE',  ( 5.405949406249999534, 9.363379034771803333, -2.781250002048374359 ) ) ;
#10515=CARTESIAN_POINT ( 'NONE',  ( -10.81189881249999729, 1.324075727343319199E-15, -102.7812500020483952 ) ) ;
#10518=CARTESIAN_POINT ( 'NONE',  ( -10.00000000000000000, -5.773502691896251982, -73.50000000409674783 ) ) ;
#10520=CARTESIAN_POINT ( 'NONE',  ( 5.405949406249992428, -9.363379034771808662, -31.59375000204836681 ) ) ;
#10523=ADVANCED_FACE ( 'NONE', ( #39646 ), #30968, .F. ) ;
#10524=CARTESIAN_POINT ( 'NONE',  ( 10.81189881249999729, 0.000000000000000000, -27.03125000204836681 ) ) ;
#10527=CARTESIAN_POINT ( 'NONE',  ( -4.999999999999996447, 8.660254037844387298, -3.375000004096767370 ) ) ;
#10528=ADVANCED_FACE ( 'NONE', ( #29959 ), #11083, .F. ) ;
#10530=CARTESIAN_POINT ( 'NONE',  ( 4.999999999999992006, -8.660254037844389075, -155.6250000040967905 ) ) ;
#10534=VERTEX_POINT ( 'NONE', #14307 ) ;
#10539=VERTEX_POINT ( 'NONE', #24713 ) ;
#10542=CARTESIAN_POINT ( 'NONE',  ( -10.81189881249999729, 6.242252689847871849, -168.9062500020483810 ) ) ;
#10544=ADVANCED_FACE ( 'NONE', ( #7872 ), #40641, .F. ) ;
#10546=CARTESIAN_POINT ( 'NONE',  ( -10.81189881249999729, 1.324075727343319199E-15, -93.59375000204838102 ) ) ;
#10547=CARTESIAN_POINT ( 'NONE',  ( 10.81189881249999907, 6.242252689847868297, -199.2187500020484094 ) ) ;
#10548=CARTESIAN_POINT ( 'NONE',  ( 10.81189881249999907, 6.242252689847868297, -97.40625000204839523 ) ) ;
#10550=CARTESIAN_POINT ( 'NONE',  ( 5.405949406249999534, 9.363379034771803333, -106.0937500020483810 ) ) ;
#10552=CARTESIAN_POINT ( 'NONE',  ( 10.00000000000051159, -5.773502691895965988, -104.5000000040967620 ) ) ;
#10553=CARTESIAN_POINT ( 'NONE',  ( 7.644554776091147741E-16, 12.48450537969573659, -199.1562500020484094 ) ) ;
#10556=CARTESIAN_POINT ( 'NONE',  ( -10.00000000000000000, -5.773502691896251982, -174.0000000040967905 ) ) ;
#10558=CARTESIAN_POINT ( 'NONE',  ( -2.293366432827344421E-15, -12.48450537969573659, -21.21875000204837036 ) ) ;
#10560=CARTESIAN_POINT ( 'NONE',  ( 7.644554776091147741E-16, 12.48450537969573659, -132.9687500020483810 ) ) ;
#10562=CARTESIAN_POINT ( 'NONE',  ( 5.405949406249992428, -9.363379034771808662, -30.28125000204837036 ) ) ;
#10564=CARTESIAN_POINT ( 'NONE',  ( 4.999999999999992006, -8.660254037844389075, -57.74999999999997158 ) ) ;
#10565=CARTESIAN_POINT ( 'NONE',  ( 10.81189881249999729, 0.000000000000000000, -126.0312500020483952 ) ) ;
#10569=CARTESIAN_POINT ( 'NONE',  ( 5.000000000000000000, 8.660254037844385522, -99.62500000409679046 ) ) ;
#10571=CARTESIAN_POINT ( 'NONE',  ( 10.81189881249999551, -6.242252689847874514, -55.46875000204837391 ) ) ;
#10575=CARTESIAN_POINT ( 'NONE',  ( 0.000000000000000000, 0.000000000000000000, -99.99999999999998579 ) ) ;
#10576=CARTESIAN_POINT ( 'NONE',  ( -9.999999999999998224, 1.224646799147353059E-15, -39.12500000409676915 ) ) ;
#10581=ORIENTED_EDGE ( 'NONE', *, *, #33908, .T. ) ;
#10582=ORIENTED_EDGE ( 'NONE', *, *, #38051, .T. ) ;
#10586=CARTESIAN_POINT ( 'NONE',  ( 5.405949406249999534, 9.363379034771803333, -197.7812500020484094 ) ) ;
#10587=EDGE_CURVE ( 'NONE', #41907, #28187, #2914, .T. ) ;
#10593=ADVANCED_FACE ( 'NONE', ( #17772 ), #1398, .F. ) ;
#10594=CARTESIAN_POINT ( 'NONE',  ( -9.999999999999479527, -5.773502691896549521, -119.6249999999999858 ) ) ;
#10595=CARTESIAN_POINT ( 'NONE',  ( 10.81189881249999729, 0.000000000000000000, -113.8437500020483810 ) ) ;
#10596=CARTESIAN_POINT ( 'NONE',  ( 10.00000000000000000, 5.773502691896255534, -197.2500000040968189 ) ) ;
#10597=CARTESIAN_POINT ( 'NONE',  ( 10.81189881249999907, 6.242252689847868297, -125.9062500020483810 ) ) ;
#10599=CARTESIAN_POINT ( 'NONE',  ( 5.405949406249992428, -9.363379034771808662, -139.5937500020483810 ) ) ;
#10601=CARTESIAN_POINT ( 'NONE',  ( 10.00000000000000000, 5.773502691896255534, -156.3749999999999716 ) ) ;
#10602=CARTESIAN_POINT ( 'NONE',  ( -5.000000000000003553, -8.660254037844383745, -18.99999999999996092 ) ) ;
#10607=CARTESIAN_POINT ( 'NONE',  ( -5.405949406250003975, -9.363379034771801557, -46.84375000204838102 ) ) ;
#10609=CARTESIAN_POINT ( 'NONE',  ( -5.405949406249996869, 9.363379034771805109, -150.8437500020483810 ) ) ;
#10612=CARTESIAN_POINT ( 'NONE',  ( 10.70731569305653252, 1.500182182591227154, -180.0000000000000284 ) ) ;
#10613=CARTESIAN_POINT ( 'NONE',  ( 9.999999999999998224, 0.000000000000000000, -81.49999999999998579 ) ) ;
#10616=CARTESIAN_POINT ( 'NONE',  ( -5.405949406249996869, 9.363379034771805109, -113.5312500020483952 ) ) ;
#10617=CARTESIAN_POINT ( 'NONE',  ( -9.999999999999998224, 5.773502691896259087, -129.2500000040967905 ) ) ;
#10622=CARTESIAN_POINT ( 'NONE',  ( -2.293366432827344421E-15, -12.48450537969573659, -48.40625000204838102 ) ) ;
#10624=DIRECTION ( 'NONE',  ( -0.000000000000000000, -0.000000000000000000, -1.000000000000000000 ) ) ;
#10628=ADVANCED_FACE ( 'NONE', ( #31832 ), #38072, .F. ) ;
#10629=VERTEX_POINT ( 'NONE', #25348 ) ;
#10631=EDGE_LOOP ( 'NONE', ( #10119, #3876, #2758, #8867 ) ) ;
#10640=DIRECTION ( 'NONE',  ( -0.000000000000000000, -0.000000000000000000, -1.000000000000000000 ) ) ;
#10644=CARTESIAN_POINT ( 'NONE',  ( 5.405949406249999534, 9.363379034771803333, -139.0937500020483810 ) ) ;
#10645=CARTESIAN_POINT ( 'NONE',  ( 10.81189881249999729, 0.000000000000000000, -158.8437500020483810 ) ) ;
#10649=CARTESIAN_POINT ( 'NONE',  ( 10.00000000000000000, 5.773502691896255534, -177.3750000000000000 ) ) ;
#10655=CARTESIAN_POINT ( 'NONE',  ( 10.81189881249999907, 6.242252689847868297, -178.2187500020483810 ) ) ;
#10658=CARTESIAN_POINT ( 'NONE',  ( 5.405949406249999534, 9.363379034771803333, -49.28125000204838813 ) ) ;
#10660=CARTESIAN_POINT ( 'NONE',  ( 10.00000000000000000, 5.773502691896255534, -105.3749999999999858 ) ) ;
#10662=CARTESIAN_POINT ( 'NONE',  ( -10.81189881249999729, -6.242252689847864744, -137.1562500020484094 ) ) ;
#10663=CARTESIAN_POINT ( 'NONE',  ( -2.121150477449813534E-15, -11.54700538379251284, -157.2500000040967620 ) ) ;
#10664=CARTESIAN_POINT ( 'NONE',  ( -5.405949406250003975, -9.363379034771801557, -149.0312500020483810 ) ) ;
#10666=CARTESIAN_POINT ( 'NONE',  ( 5.405949406249992428, -9.363379034771808662, -79.59375000204838102 ) ) ;
#10669=CARTESIAN_POINT ( 'NONE',  ( 10.81189881249999907, 6.242252689847868297, -184.2187500020483810 ) ) ;
#10673=CARTESIAN_POINT ( 'NONE',  ( -2.293366432827344421E-15, -12.48450537969573659, -73.90625000204836681 ) ) ;
#10676=CARTESIAN_POINT ( 'NONE',  ( -4.999999999999996447, 8.660254037844387298, -52.87500000409675494 ) ) ;
#10677=CARTESIAN_POINT ( 'NONE',  ( -10.81189881249999907, -6.242252689847864744, -13.96875000204836326 ) ) ;
#10680=CARTESIAN_POINT ( 'NONE',  ( -10.81189881249999729, 6.242252689847871849, -2.406250002048360592 ) ) ;
#10681=CARTESIAN_POINT ( 'NONE',  ( 0.000000000000000000, 0.000000000000000000, -180.0000000000000000 ) ) ;
#10682=CARTESIAN_POINT ( 'NONE',  ( -2.121150477449813534E-15, -11.54700538379251284, -161.3750000000000000 ) ) ;
#10686=FACE_OUTER_BOUND ( 'NONE', #30821, .T. ) ;
#10689=CARTESIAN_POINT ( 'NONE',  ( -5.000000000000003553, -8.660254037844383745, -122.8750000040967905 ) ) ;
#10693=AXIS2_PLACEMENT_3D ( 'NONE', #35903, #2889, #39973 ) ;
#10698=CARTESIAN_POINT ( 'NONE',  ( -5.000000000000003553, -8.660254037844383745, -47.49999999999998579 ) ) ;
#10700=CARTESIAN_POINT ( 'NONE',  ( -2.293366432827344421E-15, -12.48450537969573659, -163.7187500020483810 ) ) ;
#10702=CARTESIAN_POINT ( 'NONE',  ( -9.999999999999742428, -5.773502691896402084, -121.5000000040967905 ) ) ;
#10703=CARTESIAN_POINT ( 'NONE',  ( 5.000000000000000000, 8.660254037844385522, -147.2500000000000000 ) ) ;
#10704=CARTESIAN_POINT ( 'NONE',  ( -10.00000000000051337, 5.773502691895962435, -143.8750000000000000 ) ) ;
#10711=CARTESIAN_POINT ( 'NONE',  ( -10.81189881249999907, -6.242252689847864744, -66.46875000204838102 ) ) ;
#10713=CARTESIAN_POINT ( 'NONE',  ( 7.644554776091147741E-16, 12.48450537969573659, -79.15625000204838102 ) ) ;
#10716=CARTESIAN_POINT ( 'NONE',  ( -10.81189881249999729, -6.242252689847864744, -161.1562500020484094 ) ) ;
#10717=CARTESIAN_POINT ( 'NONE',  ( -10.81189881249999729, 1.324075727343319199E-15, -174.7812500020484094 ) ) ;
#10719=CARTESIAN_POINT ( 'NONE',  ( -2.293366432827344421E-15, -12.48450537969573659, -1.718750002048352377 ) ) ;
#10720=CARTESIAN_POINT ( 'NONE',  ( -9.999999999999998224, 1.224646799147353059E-15, -108.1250000040967763 ) ) ;
#10721=CARTESIAN_POINT ( 'NONE',  ( 7.644554776091147741E-16, 12.48450537969573659, -102.9687500020483952 ) ) ;
#10722=CYLINDRICAL_SURFACE ( 'NONE', #21768, 9.999999999999998224 ) ;
#10724=CARTESIAN_POINT ( 'NONE',  ( -10.81189881249999729, 6.242252689847871849, -5.406250002048363257 ) ) ;
#10728=CARTESIAN_POINT ( 'NONE',  ( 5.405949406249999534, 9.363379034771803333, -101.7812500020483952 ) ) ;
#10730=CARTESIAN_POINT ( 'NONE',  ( -10.00000000000000000, -5.773502691896251982, -76.50000000409677625 ) ) ;
#10731=CARTESIAN_POINT ( 'NONE',  ( -10.00000000000076916, 5.773502691895813221, -134.8750000000000000 ) ) ;
#10732=CARTESIAN_POINT ( 'NONE',  ( -2.293366432827344421E-15, -12.48450537969573659, -36.21875000204835970 ) ) ;
#10735=CARTESIAN_POINT ( 'NONE',  ( 5.405949406249999534, 9.363379034771803333, -25.28125000204836681 ) ) ;
#10738=CARTESIAN_POINT ( 'NONE',  ( 5.000000000000000000, 8.660254037844385522, -3.625000004096767814 ) ) ;
#10751=DIRECTION ( 'NONE',  ( -1.000000000000000000, 0.000000000000000000, 0.000000000000000000 ) ) ;
#10753=( BOUNDED_CURVE ( )  B_SPLINE_CURVE ( 2, ( #10021, #20369, #20164, #4192, #30540, #16908, #39798 ),
 .UNSPECIFIED., .F., .F. ) 
 B_SPLINE_CURVE_WITH_KNOTS ( ( 3, 2, 2, 3 ),
 ( 0.2388059701492538378, 0.2400497512437811953, 0.2412935323383085806, 0.2425373134328359381 ),
 .UNSPECIFIED. ) 
 CURVE ( )  GEOMETRIC_REPRESENTATION_ITEM ( )  RATIONAL_B_SPLINE_CURVE ( ( 0.9999999999999880096, 0.8660254037844506980, 1.000000000000000000, 0.8660254037844387076, 1.000000000000000000, 0.8660254037844267172, 1.000000000000011990 ) ) 
 REPRESENTATION_ITEM ( '' )  );
#10754=CARTESIAN_POINT ( 'NONE',  ( -2.293366432827344421E-15, -12.48450537969573659, -171.4062500020484379 ) ) ;
#10758=CARTESIAN_POINT ( 'NONE',  ( 10.81189881249999551, -6.242252689847874514, -94.46875000204838102 ) ) ;
#10759=CARTESIAN_POINT ( 'NONE',  ( -4.999999999999996447, 8.660254037844387298, -112.8750000040967763 ) ) ;
#10760=CARTESIAN_POINT ( 'NONE',  ( -10.81189881249999729, 6.242252689847871849, -99.90625000204838102 ) ) ;
#10762=CARTESIAN_POINT ( 'NONE',  ( -2.293366432827344421E-15, -12.48450537969573659, -108.2187500020483668 ) ) ;
#10768=CARTESIAN_POINT ( 'NONE',  ( 5.405949406249999534, 9.363379034771803333, -197.7812500020484094 ) ) ;
#10771=CARTESIAN_POINT ( 'NONE',  ( -2.121150477449813534E-15, -11.54700538379251284, -169.2500000040967620 ) ) ;
#10773=CARTESIAN_POINT ( 'NONE',  ( -10.81189881249999907, -6.242252689847864744, -21.46875000204836681 ) ) ;
#10774=CARTESIAN_POINT ( 'NONE',  ( 0.000000000000000000, 0.000000000000000000, -99.99999999999998579 ) ) ;
#10775=CARTESIAN_POINT ( 'NONE',  ( 5.405949406249999534, 9.363379034771803333, -130.0937500020483810 ) ) ;
#10777=CARTESIAN_POINT ( 'NONE',  ( 10.81189881249999907, 6.242252689847868297, -31.40625000204835615 ) ) ;
#10779=CARTESIAN_POINT ( 'NONE',  ( -9.999999999999998224, 1.224646799147353059E-15, -56.74999999999996447 ) ) ;
#10780=CARTESIAN_POINT ( 'NONE',  ( -10.81189881249999729, 1.324075727343319199E-15, -126.7812500020483668 ) ) ;
#10784=CARTESIAN_POINT ( 'NONE',  ( 5.000000000000000000, 8.660254037844385522, -101.1250000040967905 ) ) ;
#10787=CARTESIAN_POINT ( 'NONE',  ( 5.405949406249999534, 9.363379034771803333, -56.59375000204835970 ) ) ;
#10788=EDGE_LOOP ( 'NONE', ( #40676, #7955, #23350, #2541 ) ) ;
#10793=CARTESIAN_POINT ( 'NONE',  ( -5.000000000000003553, -8.660254037844383745, -26.87500000409676204 ) ) ;
#10794=LINE ( 'NONE', #26997, #41741 ) ;
#10797=ORIENTED_EDGE ( 'NONE', *, *, #32796, .T. ) ;
#10800=CARTESIAN_POINT ( 'NONE',  ( -4.999999999999996447, 8.660254037844387298, -174.3750000040968189 ) ) ;
#10802=CARTESIAN_POINT ( 'NONE',  ( -5.405949406250003975, -9.363379034771801557, -197.0312500020484094 ) ) ;
#10808=CARTESIAN_POINT ( 'NONE',  ( -5.405949406249996869, 9.363379034771805109, -117.8437500020483810 ) ) ;
#10809=CARTESIAN_POINT ( 'NONE',  ( -4.999999999999996447, 8.660254037844387298, -192.3750000040967905 ) ) ;
#10810=CARTESIAN_POINT ( 'NONE',  ( 5.405949406249999534, 9.363379034771803333, -122.7812500020483952 ) ) ;
#10812=CARTESIAN_POINT ( 'NONE',  ( -2.293366432827344421E-15, -12.48450537969573659, -132.2187500020483810 ) ) ;
#10814=CARTESIAN_POINT ( 'NONE',  ( 9.999999999999998224, 0.000000000000000000, -179.3750000040967905 ) ) ;
#10815=CARTESIAN_POINT ( 'NONE',  ( -10.00000000000000000, -5.773502691896251982, -158.6250000000000284 ) ) ;
#10816=CARTESIAN_POINT ( 'NONE',  ( 5.000000000000000000, 8.660254037844385522, -18.24999999999996092 ) ) ;
#10819=CYLINDRICAL_SURFACE ( 'NONE', #9786, 9.999999999999998224 ) ;
#10821=CARTESIAN_POINT ( 'NONE',  ( 5.405949406249999534, 9.363379034771803333, -43.09375000204837391 ) ) ;
#10823=CARTESIAN_POINT ( 'NONE',  ( -10.81189881249999729, 6.242252689847871849, -155.2187500020483810 ) ) ;
#10827=CARTESIAN_POINT ( 'NONE',  ( -2.121150477449813534E-15, -11.54700538379251284, -81.87500000000000000 ) ) ;
#10830=CARTESIAN_POINT ( 'NONE',  ( 10.81189881249999729, 0.000000000000000000, -106.5312500020483810 ) ) ;
#10831=CARTESIAN_POINT ( 'NONE',  ( -9.999999999999998224, 1.224646799147353059E-15, -126.1250000040967620 ) ) ;
#10836=CARTESIAN_POINT ( 'NONE',  ( 5.405949406249999534, 9.363379034771803333, -53.78125000204836681 ) ) ;
#10837=CARTESIAN_POINT ( 'NONE',  ( -5.000000000000003553, -8.660254037844383745, -136.0000000000000000 ) ) ;
#10844=CARTESIAN_POINT ( 'NONE',  ( -4.999999999999996447, 8.660254037844387298, -163.8750000040967905 ) ) ;
#10851=CARTESIAN_POINT ( 'NONE',  ( 5.000000000000000000, 8.660254037844385522, -103.7500000000000000 ) ) ;
#10859=CARTESIAN_POINT ( 'NONE',  ( -10.81189881249999907, -6.242252689847864744, -139.9687500020483810 ) ) ;
#10860=CARTESIAN_POINT ( 'NONE',  ( -10.81189881249999729, 1.324075727343319199E-15, -156.5937500020483810 ) ) ;
#10863=CARTESIAN_POINT ( 'NONE',  ( -9.999999999999998224, 1.224646799147353059E-15, -176.7500000000000284 ) ) ;
#10867=CARTESIAN_POINT ( 'NONE',  ( -5.000000000000003553, -8.660254037844383745, -124.3750000040967763 ) ) ;
#10868=CARTESIAN_POINT ( 'NONE',  ( 10.81189881249999551, -6.242252689847874514, -179.9687500020484094 ) ) ;
#10871=CARTESIAN_POINT ( 'NONE',  ( 10.81189881249999551, -6.242252689847874514, -55.65625000204837391 ) ) ;
#10873=CARTESIAN_POINT ( 'NONE',  ( -10.00000000000000000, -5.773502691896251982, -104.6249999999999858 ) ) ;
#10876=CARTESIAN_POINT ( 'NONE',  ( -10.81189881249999729, 1.324075727343319199E-15, -132.7812500020483810 ) ) ;
#10877=CARTESIAN_POINT ( 'NONE',  ( -2.121150477449813534E-15, -11.54700538379251284, -151.2500000040967620 ) ) ;
#10878=CARTESIAN_POINT ( 'NONE',  ( -2.293366432827344421E-15, -12.48450537969573659, -145.9062500020484094 ) ) ;
#10881=ORIENTED_EDGE ( 'NONE', *, *, #17901, .T. ) ;
#10883=CARTESIAN_POINT ( 'NONE',  ( -10.81189881249999729, 1.324075727343319199E-15, -183.5937500020483810 ) ) ;
#10885=AXIS2_PLACEMENT_3D ( 'NONE', #4395, #10640, #11065 ) ;
#10886=CARTESIAN_POINT ( 'NONE',  ( 4.999999999999992006, -8.660254037844389075, -110.2499999999999858 ) ) ;
#10888=CARTESIAN_POINT ( 'NONE',  ( -5.405949406250003975, -9.363379034771801557, -80.03125000204838102 ) ) ;
#10890=CARTESIAN_POINT ( 'NONE',  ( 9.999999999999996447, -5.773502691896262640, -52.00000000409676915 ) ) ;
#10891=CARTESIAN_POINT ( 'NONE',  ( 5.405949406249992428, -9.363379034771808662, -13.59375000204834905 ) ) ;
#10894=CARTESIAN_POINT ( 'NONE',  ( 5.405949406249999534, 9.363379034771803333, -2.781250002048374359 ) ) ;
#10896=CARTESIAN_POINT ( 'NONE',  ( 9.999999999999998224, 0.000000000000000000, -138.8750000040968189 ) ) ;
#10902=ADVANCED_FACE ( 'NONE', ( #30071 ), #25978, .F. ) ;
#10904=VERTEX_POINT ( 'NONE', #16227 ) ;
#10905=CARTESIAN_POINT ( 'NONE',  ( 9.999999999999998224, 0.000000000000000000, -122.3750000040967905 ) ) ;
#10908=ORIENTED_EDGE ( 'NONE', *, *, #17752, .T. ) ;
#10914=CARTESIAN_POINT ( 'NONE',  ( -10.00000000000000000, -5.773502691896251982, -41.62499999999996447 ) ) ;
#10916=CARTESIAN_POINT ( 'NONE',  ( 5.405949406249999534, 9.363379034771803333, -163.0937500020484094 ) ) ;
#10919=CARTESIAN_POINT ( 'NONE',  ( -4.999999999999996447, 8.660254037844387298, -147.0000000000000000 ) ) ;
#10926=CARTESIAN_POINT ( 'NONE',  ( 10.81189881249999729, 0.000000000000000000, -67.34375000204836681 ) ) ;
#10927=CARTESIAN_POINT ( 'NONE',  ( -10.81189881249999729, 1.324075727343319199E-15, -77.28125000204838102 ) ) ;
#10929=CARTESIAN_POINT ( 'NONE',  ( -9.999999999999998224, 1.224646799147353059E-15, -131.7499999999999716 ) ) ;
#10930=CARTESIAN_POINT ( 'NONE',  ( 10.81189881249999729, 0.000000000000000000, -160.5312500020484094 ) ) ;
#10931=CARTESIAN_POINT ( 'NONE',  ( -10.81189881249999729, 1.324075727343319199E-15, -173.2812500020484094 ) ) ;
#10932=CARTESIAN_POINT ( 'NONE',  ( -9.999999999999998224, 1.224646799147353059E-15, -145.6250000040967905 ) ) ;
#10934=CARTESIAN_POINT ( 'NONE',  ( 5.405949406249992428, -9.363379034771808662, -108.0937500020483810 ) ) ;
#10937=CARTESIAN_POINT ( 'NONE',  ( -10.81189881249999729, 1.324075727343319199E-15, -2.281250002048373915 ) ) ;
#10940=CARTESIAN_POINT ( 'NONE',  ( 10.81189881249999729, 0.000000000000000000, -97.53125000204839523 ) ) ;
#10942=CARTESIAN_POINT ( 'NONE',  ( -5.000000000000003553, -8.660254037844383745, -76.37500000409677625 ) ) ;
#10944=CARTESIAN_POINT ( 'NONE',  ( -10.81189881249999729, 6.242252689847871849, -33.71875000204835260 ) ) ;
#10947=CARTESIAN_POINT ( 'NONE',  ( -10.81189881249999907, -6.242252689847864744, -29.15625000204835970 ) ) ;
#10949=CARTESIAN_POINT ( 'NONE',  ( -10.00000000000025580, 5.773502691896109873, -160.3750000000000000 ) ) ;
#10951=CARTESIAN_POINT ( 'NONE',  ( 7.070501591499377789E-16, 11.54700538379251284, -0.5000000040967511605 ) ) ;
#10958=ORIENTED_EDGE ( 'NONE', *, *, #38837, .F. ) ;
#10961=EDGE_CURVE ( 'NONE', #25900, #6469, #32464, .T. ) ;
#10963=CARTESIAN_POINT ( 'NONE',  ( 9.999999999999998224, 0.000000000000000000, -143.3750000040967905 ) ) ;
#10964=FACE_OUTER_BOUND ( 'NONE', #9685, .T. ) ;
#10966=CARTESIAN_POINT ( 'NONE',  ( 10.81189881249999907, 6.242252689847868297, -169.4062500020484094 ) ) ;
#10969=CARTESIAN_POINT ( 'NONE',  ( 10.81189881249999907, 6.242252689847868297, -91.21875000204838102 ) ) ;
#10971=CARTESIAN_POINT ( 'NONE',  ( -9.999999999999998224, 1.224646799147353059E-15, -154.2500000000000000 ) ) ;
#10972=CARTESIAN_POINT ( 'NONE',  ( 10.81189881249999907, 6.242252689847868297, -98.90625000204839523 ) ) ;
#10974=CARTESIAN_POINT ( 'NONE',  ( 10.81189881249999551, -6.242252689847874514, -106.4687500020483810 ) ) ;
#10976=CARTESIAN_POINT ( 'NONE',  ( 7.070501591499376803E-16, 11.54700538379251284, -108.1249999999999858 ) ) ;
#10978=CARTESIAN_POINT ( 'NONE',  ( -10.81189881249999729, 1.324075727343319199E-15, -197.2812500020484094 ) ) ;
#10982=CARTESIAN_POINT ( 'NONE',  ( -10.00000000000000000, -5.773502691896251982, -175.5000000040967905 ) ) ;
#10984=CARTESIAN_POINT ( 'NONE',  ( -5.405949406250003975, -9.363379034771801557, -24.34375000204835970 ) ) ;
#10986=CARTESIAN_POINT ( 'NONE',  ( -5.405949406249996869, 9.363379034771805109, -131.3437500020484094 ) ) ;
#10988=CARTESIAN_POINT ( 'NONE',  ( -5.405949406249996869, 9.363379034771805109, -26.53125000204836681 ) ) ;
#10991=CARTESIAN_POINT ( 'NONE',  ( -4.999999999999996447, 8.660254037844387298, -61.49999999999997158 ) ) ;
#10992=CARTESIAN_POINT ( 'NONE',  ( -10.81189881249999907, -6.242252689847864744, -128.1562500020483810 ) ) ;
#10994=EDGE_LOOP ( 'NONE', ( #25069, #1890, #26001, #15680 ) ) ;
#10997=CARTESIAN_POINT ( 'NONE',  ( -9.999999999999998224, 1.224646799147353059E-15, -100.6250000040967905 ) ) ;
#10998=CARTESIAN_POINT ( 'NONE',  ( -5.000000000000003553, -8.660254037844383745, -151.3750000040967905 ) ) ;
#11000=CARTESIAN_POINT ( 'NONE',  ( -5.405949406249996869, 9.363379034771805109, -57.84375000204835970 ) ) ;
#11005=CARTESIAN_POINT ( 'NONE',  ( 0.000000000000000000, 0.000000000000000000, -99.99999999999998579 ) ) ;
#11006=CARTESIAN_POINT ( 'NONE',  ( -4.999999999999996447, 8.660254037844387298, -30.37500000409676204 ) ) ;
#11018=FACE_OUTER_BOUND ( 'NONE', #15503, .T. ) ;
#11023=CARTESIAN_POINT ( 'NONE',  ( -10.81189881249999729, 6.242252689847871849, -116.2187500020483810 ) ) ;
#11024=CARTESIAN_POINT ( 'NONE',  ( -5.405949406249996869, 9.363379034771805109, 0.6562499979516356330 ) ) ;
#11025=CARTESIAN_POINT ( 'NONE',  ( 7.644554776091147741E-16, 12.48450537969573659, -125.6562500020483810 ) ) ;
#11027=CARTESIAN_POINT ( 'NONE',  ( -10.81189881249999729, -6.242252689847864744, -129.4687500020483810 ) ) ;
#11031=CARTESIAN_POINT ( 'NONE',  ( -9.999999999999998224, 5.773502691896259087, -154.3749999999999716 ) ) ;
#11032=CARTESIAN_POINT ( 'NONE',  ( 4.999999999999992006, -8.660254037844389075, -17.24999999999996092 ) ) ;
#11035=FACE_OUTER_BOUND ( 'NONE', #40829, .T. ) ;
#11037=CARTESIAN_POINT ( 'NONE',  ( 10.81189881249999551, -6.242252689847874514, -49.46875000204836681 ) ) ;
#11039=CARTESIAN_POINT ( 'NONE',  ( 10.81189881249999551, -6.242252689847874514, -151.4687500020483810 ) ) ;
#11043=CARTESIAN_POINT ( 'NONE',  ( 7.070501591499377789E-16, 11.54700538379251284, -85.62499999999997158 ) ) ;
#11046=CARTESIAN_POINT ( 'NONE',  ( 10.81189881249999551, -6.242252689847874514, -102.1562500020483952 ) ) ;
#11047=CARTESIAN_POINT ( 'NONE',  ( -4.999999999999996447, 8.660254037844387298, -121.8750000040967905 ) ) ;
#11051=CARTESIAN_POINT ( 'NONE',  ( 10.81189881249999729, 0.000000000000000000, -40.53125000204838102 ) ) ;
#11058=ORIENTED_EDGE ( 'NONE', *, *, #23349, .F. ) ;
#11060=VERTEX_POINT ( 'NONE', #12991 ) ;
#11065=DIRECTION ( 'NONE',  ( -1.000000000000000000, 0.000000000000000000, 0.000000000000000000 ) ) ;
#11070=CARTESIAN_POINT ( 'NONE',  ( -5.405949406250003975, -9.363379034771801557, -144.3437500020483810 ) ) ;
#11071=CARTESIAN_POINT ( 'NONE',  ( -5.405949406249996869, 9.363379034771805109, -153.8437500020483810 ) ) ;
#11072=CYLINDRICAL_SURFACE ( 'NONE', #29511, 9.999999999999998224 ) ;
#11073=CARTESIAN_POINT ( 'NONE',  ( 4.999999999999992006, -8.660254037844389075, -182.2500000000000000 ) ) ;
#11078=EDGE_CURVE ( 'NONE', #23210, #37997, #16019, .T. ) ;
#11079=CARTESIAN_POINT ( 'NONE',  ( 10.81189881249999551, -6.242252689847874514, -176.9687500020483810 ) ) ;
#11083=CYLINDRICAL_SURFACE ( 'NONE', #19959, 9.999999999999998224 ) ;
#11084=CARTESIAN_POINT ( 'NONE',  ( -10.81189881249999729, 6.242252689847871849, -44.40625000204836681 ) ) ;
#11086=CARTESIAN_POINT ( 'NONE',  ( -5.000000000000003553, -8.660254037844383745, -107.4999999999999858 ) ) ;
#11088=CARTESIAN_POINT ( 'NONE',  ( -5.405949406250003975, -9.363379034771801557, -125.0312500020483952 ) ) ;
#11089=CARTESIAN_POINT ( 'NONE',  ( 9.999999999999998224, 0.000000000000000000, -146.3750000040967905 ) ) ;
#11093=CARTESIAN_POINT ( 'NONE',  ( -10.81189881249999729, 6.242252689847871849, -177.7187500020483810 ) ) ;
#11096=CARTESIAN_POINT ( 'NONE',  ( -9.999999999999998224, 0.000000000000000000, -99.99999999999998579 ) ) ;
#11097=CARTESIAN_POINT ( 'NONE',  ( 5.405949406249992428, -9.363379034771808662, -73.78125000204838102 ) ) ;
#11099=CARTESIAN_POINT ( 'NONE',  ( -2.121150477449813534E-15, -11.54700538379251284, -49.25000000409676915 ) ) ;
#11100=CARTESIAN_POINT ( 'NONE',  ( 10.81189881249999729, 0.000000000000000000, -10.34375000204834549 ) ) ;
#11104=CARTESIAN_POINT ( 'NONE',  ( -2.293366432827344421E-15, -12.48450537969573659, -1.906250002048359704 ) ) ;
#11105=CARTESIAN_POINT ( 'NONE',  ( -4.999999999999996447, 8.660254037844387298, -148.5000000000000000 ) ) ;
#11106=DIRECTION ( 'NONE',  ( -0.000000000000000000, -0.000000000000000000, -1.000000000000000000 ) ) ;
#11112=DIRECTION ( 'NONE',  ( 0.000000000000000000, 0.000000000000000000, 1.000000000000000000 ) ) ;
#11113=CARTESIAN_POINT ( 'NONE',  ( -2.121150477449813534E-15, -11.54700538379251284, -122.7500000040967905 ) ) ;
#11115=EDGE_LOOP ( 'NONE', ( #30612, #22075, #23671, #29032 ) ) ;
#11121=CARTESIAN_POINT ( 'NONE',  ( -5.000000000000003553, -8.660254037844383745, -45.99999999999998579 ) ) ;
#11123=CARTESIAN_POINT ( 'NONE',  ( 5.405949406249992428, -9.363379034771808662, -168.0937500020484094 ) ) ;
#11125=( BOUNDED_CURVE ( )  B_SPLINE_CURVE ( 2, ( #30841, #8609, #37521, #21763, #7964, #17865, #21328 ),
 .UNSPECIFIED., .F., .F. ) 
 B_SPLINE_CURVE_WITH_KNOTS ( ( 3, 2, 2, 3 ),
 ( 0.4626865671641792743, 0.4639303482587066596, 0.4651741293532339339, 0.4664179104477613191 ),
 .UNSPECIFIED. ) 
 CURVE ( )  GEOMETRIC_REPRESENTATION_ITEM ( )  RATIONAL_B_SPLINE_CURVE ( ( 0.9999999999999820144, 0.8660254037844566932, 1.000000000000000000, 0.8660254037844387076, 1.000000000000000000, 0.8660254037844267172, 1.000000000000011990 ) ) 
 REPRESENTATION_ITEM ( '' )  );
#11126=CARTESIAN_POINT ( 'NONE',  ( -2.293366432827344421E-15, -12.48450537969573659, -177.2187500020484094 ) ) ;
#11135=ADVANCED_FACE ( 'NONE', ( #39130 ), #26187, .F. ) ;
#11137=CARTESIAN_POINT ( 'NONE',  ( 7.644554776091147741E-16, 12.48450537969573659, -65.46875000204838102 ) ) ;
#11139=CARTESIAN_POINT ( 'NONE',  ( -10.81189881249999729, 1.324075727343319199E-15, -80.28125000204838102 ) ) ;
#11141=CARTESIAN_POINT ( 'NONE',  ( 5.000000000000000000, 8.660254037844385522, -127.7499999999999716 ) ) ;
#11143=CARTESIAN_POINT ( 'NONE',  ( 5.405949406249992428, -9.363379034771808662, -154.7812500020484094 ) ) ;
#11144=CARTESIAN_POINT ( 'NONE',  ( 10.81189881249999551, -6.242252689847874514, -169.6562500020484094 ) ) ;
#11146=DIRECTION ( 'NONE',  ( -0.000000000000000000, -0.000000000000000000, -1.000000000000000000 ) ) ;
#11147=CARTESIAN_POINT ( 'NONE',  ( 7.644554776091147741E-16, 12.48450537969573659, -104.4687500020483668 ) ) ;
#11150=CARTESIAN_POINT ( 'NONE',  ( -5.405949406249996869, 9.363379034771805109, -1.031250002048372805 ) ) ;
#11152=CARTESIAN_POINT ( 'NONE',  ( -9.999999999999998224, 1.224646799147353059E-15, -141.1250000040967905 ) ) ;
#11153=CARTESIAN_POINT ( 'NONE',  ( -2.293366432827344421E-15, -12.48450537969573659, -100.9062500020483952 ) ) ;
#11155=CARTESIAN_POINT ( 'NONE',  ( 7.070501591499377789E-16, 11.54700538379251284, -77.00000000409677625 ) ) ;
#11157=CARTESIAN_POINT ( 'NONE',  ( -10.81189881249999729, 1.324075727343319199E-15, -36.59375000204836681 ) ) ;
#11160=CARTESIAN_POINT ( 'NONE',  ( -5.405949406249996869, 9.363379034771805109, -28.03125000204837036 ) ) ;
#11163=ADVANCED_FACE ( 'NONE', ( #19696 ), #32879, .F. ) ;
#11164=CARTESIAN_POINT ( 'NONE',  ( -5.000000000000003553, -8.660254037844383745, -5.875000004096770034 ) ) ;
#11166=VECTOR ( 'NONE', #34156, 1000.000000000000000 ) ;
#11172=CARTESIAN_POINT ( 'NONE',  ( 0.000000000000000000, 0.000000000000000000, -99.99999999999998579 ) ) ;
#11174=EDGE_LOOP ( 'NONE', ( #9019, #26158, #30473, #8061 ) ) ;
#11178=AXIS2_PLACEMENT_3D ( 'NONE', #29644, #88, #29862 ) ;
#11181=EDGE_CURVE ( 'NONE', #33599, #36083, #27119, .T. ) ;
#11182=CARTESIAN_POINT ( 'NONE',  ( 3.425473324849547030, 10.17518912463928338, -99.99999999999998579 ) ) ;
#11184=CARTESIAN_POINT ( 'NONE',  ( 5.405949406249999534, 9.363379034771803333, -161.7812500020484094 ) ) ;
#11187=CARTESIAN_POINT ( 'NONE',  ( -10.81189881249999729, 6.242252689847871849, -90.71875000204838102 ) ) ;
#11189=CARTESIAN_POINT ( 'NONE',  ( 5.000000000000000000, 8.660254037844385522, -106.7499999999999858 ) ) ;
#11190=CARTESIAN_POINT ( 'NONE',  ( -5.405949406249996869, 9.363379034771805109, -97.03125000204839523 ) ) ;
#11192=CARTESIAN_POINT ( 'NONE',  ( -2.293366432827344421E-15, -12.48450537969573659, -105.2187500020483952 ) ) ;
#11196=CARTESIAN_POINT ( 'NONE',  ( -10.81189881249999729, 1.324075727343319199E-15, -194.2812500020484094 ) ) ;
#11198=CARTESIAN_POINT ( 'NONE',  ( 4.999999999999992006, -8.660254037844389075, -169.1250000040967905 ) ) ;
#11200=CARTESIAN_POINT ( 'NONE',  ( 10.81189881249999907, 6.242252689847868297, -20.71875000204837036 ) ) ;
#11202=CARTESIAN_POINT ( 'NONE',  ( -10.81189881249999907, -6.242252689847864744, -132.4687500020483810 ) ) ;
#11204=CARTESIAN_POINT ( 'NONE',  ( -5.405949406250003975, -9.363379034771801557, -32.03125000204837391 ) ) ;
#11206=CARTESIAN_POINT ( 'NONE',  ( 7.070501591499376803E-16, 11.54700538379251284, -102.1250000000000000 ) ) ;
#11207=CARTESIAN_POINT ( 'NONE',  ( -9.999999999999998224, 5.773502691896259087, -53.87499999999997868 ) ) ;
#11208=CARTESIAN_POINT ( 'NONE',  ( 10.81189881249999551, -6.242252689847874514, -121.6562500020483952 ) ) ;
#11211=CARTESIAN_POINT ( 'NONE',  ( -9.999999999999998224, 5.773502691896259087, -100.7500000040967905 ) ) ;
#11213=CARTESIAN_POINT ( 'NONE',  ( 5.405949406249992428, -9.363379034771808662, -58.59375000204835970 ) ) ;
#11219=CYLINDRICAL_SURFACE ( 'NONE', #18688, 9.999999999999998224 ) ;
#11220=CARTESIAN_POINT ( 'NONE',  ( -9.999999999999998224, 5.773502691896259087, -30.25000000409675138 ) ) ;
#11232=DIRECTION ( 'NONE',  ( -0.000000000000000000, -0.000000000000000000, -1.000000000000000000 ) ) ;
#11234=CARTESIAN_POINT ( 'NONE',  ( 9.999999999999998224, 0.000000000000000000, -129.5000000000000000 ) ) ;
#11238=CARTESIAN_POINT ( 'NONE',  ( 5.405949406249992428, -9.363379034771808662, -118.5937500020483810 ) ) ;
#11239=CARTESIAN_POINT ( 'NONE',  ( -4.999999999999996447, 8.660254037844387298, -198.3750000040967905 ) ) ;
#11240=CARTESIAN_POINT ( 'NONE',  ( 10.81189881249999551, -6.242252689847874514, -121.6562500020483952 ) ) ;
#11242=CARTESIAN_POINT ( 'NONE',  ( 7.644554776091147741E-16, 12.48450537969573659, -129.9687500020483810 ) ) ;
#11245=CARTESIAN_POINT ( 'NONE',  ( 4.999999999999992006, -8.660254037844389075, -150.7500000000000000 ) ) ;
#11246=CARTESIAN_POINT ( 'NONE',  ( 5.000000000000000000, 8.660254037844385522, -21.24999999999996447 ) ) ;
#11251=CARTESIAN_POINT ( 'NONE',  ( 5.405949406249999534, 9.363379034771803333, -49.09375000204838102 ) ) ;
#11253=CARTESIAN_POINT ( 'NONE',  ( -2.293366432827344421E-15, -12.48450537969573659, -157.7187500020484094 ) ) ;
#11257=CARTESIAN_POINT ( 'NONE',  ( 5.000000000000000000, 8.660254037844385522, -79.74999999999998579 ) ) ;
#11259=ORIENTED_EDGE ( 'NONE', *, *, #27279, .T. ) ;
#11260=CARTESIAN_POINT ( 'NONE',  ( 5.405949406249999534, 9.363379034771803333, -106.2812500020483810 ) ) ;
#11261=CARTESIAN_POINT ( 'NONE',  ( 9.999999999999996447, -5.773502691896262640, -125.5000000040967763 ) ) ;
#11266=CARTESIAN_POINT ( 'NONE',  ( 10.81189881249999551, -6.242252689847874514, -43.65625000204836681 ) ) ;
#11267=LINE ( 'NONE', #24463, #4183 ) ;
#11273=ORIENTED_EDGE ( 'NONE', *, *, #26456, .T. ) ;
#11285=CARTESIAN_POINT ( 'NONE',  ( 5.405949406249992428, -9.363379034771808662, -145.5937500020483810 ) ) ;
#11286=CARTESIAN_POINT ( 'NONE',  ( -5.405949406250003975, -9.363379034771801557, -146.0312500020483810 ) ) ;
#11287=CARTESIAN_POINT ( 'NONE',  ( -2.293366432827344421E-15, -12.48450537969573659, -156.2187500020483810 ) ) ;
#11290=CARTESIAN_POINT ( 'NONE',  ( -9.999999999999998224, 1.224646799147353059E-15, -178.2500000000000284 ) ) ;
#11292=DIRECTION ( 'NONE',  ( -0.000000000000000000, -0.000000000000000000, -1.000000000000000000 ) ) ;
#11294=CARTESIAN_POINT ( 'NONE',  ( -9.999999999999998224, 1.224646799147353059E-15, -168.1250000040967905 ) ) ;
#11295=CARTESIAN_POINT ( 'NONE',  ( -5.405949406250003975, -9.363379034771801557, -178.8437500020483810 ) ) ;
#11298=CARTESIAN_POINT ( 'NONE',  ( 0.000000000000000000, 0.000000000000000000, -99.99999999999998579 ) ) ;
#11299=CARTESIAN_POINT ( 'NONE',  ( 7.644554776091147741E-16, 12.48450537969573659, -46.15625000204837391 ) ) ;
#11301=CARTESIAN_POINT ( 'NONE',  ( 7.070501591499377789E-16, 11.54700538379251284, -108.1249999999999716 ) ) ;
#11302=EDGE_CURVE ( 'NONE', #10534, #21693, #13345, .T. ) ;
#11304=CARTESIAN_POINT ( 'NONE',  ( -10.81189881249999729, 1.324075727343319199E-15, -125.2812500020483668 ) ) ;
#11305=CARTESIAN_POINT ( 'NONE',  ( 5.000000000000000000, 8.660254037844385522, -146.1250000040967905 ) ) ;
#11310=CARTESIAN_POINT ( 'NONE',  ( -2.293366432827344421E-15, -12.48450537969573659, -174.2187500020484094 ) ) ;
#11312=LINE ( 'NONE', #37657, #5853 ) ;
#11314=CARTESIAN_POINT ( 'NONE',  ( 10.81189881249999551, -6.242252689847874514, -64.65625000204839523 ) ) ;
#11316=CARTESIAN_POINT ( 'NONE',  ( 9.999999999999996447, -5.773502691896262640, -46.00000000409675494 ) ) ;
#11317=CARTESIAN_POINT ( 'NONE',  ( -10.81189881249999907, -6.242252689847864744, -4.968750002048355263 ) ) ;
#11322=ORIENTED_EDGE ( 'NONE', *, *, #35080, .T. ) ;
#11339=CARTESIAN_POINT ( 'NONE',  ( -9.999999999999998224, 5.773502691896259087, -37.37499999999995737 ) ) ;
#11341=( BOUNDED_SURFACE ( )  B_SPLINE_SURFACE ( 1, 2, ( 
 ( #1018, #24115, #27339, #37251, #20853, #28632, #12197, #37907, #38757, #15434, #12406, #41764, #28840, #21924, #5530, #41557, #31657, #8977, #1877, #11990, #8351, #27985, #41114, #28203, #18470, #25186, #31877, #15640, #28421, #22354, #41973, #41337, #31234, #38535, #25599, #38326, #18679, #8768, #18250, #18038, #34684, #11553, #25387, #15222, #35104, #22144, #24976, #2092, #24762, #2308, #38117, #5317, #21502, #35318, #8562, #9183, #5747, #35530, #18900, #32081, #2515, #1657, #15005, #14790, #5104, #11774, #31442, #21712, #34893, #6578, #22989, #2930, #5959, #9397, #26017, #26432, #42395, #36146, #29892, #42186, #10228, #39169, #39583, #32500, #6167, #19735, #3348, #32915, #29680, #22561, #124, #3138, #332, #16480, #36357, #16059, #35739, #13245, #19307, #9602, #13033, #16265, #10019, #2715, #29251, #19521, #23197, #6790, #12826, #22776, #19945, #25806, #35937, #6378, #32705, #15847, #33134, #29464, #42606, #26227, #23415, #39375, #9811, #13451, #3562, #19109, #26646, #16696, #39795, #32292, #29047, #12613, #38963, #20795, #30322, #40011, #546, #37195, #40216, #34202, #756, #4618, #11073, #3772, #33983, #24276, #4190, #14298, #965, #40851, #17763, #13877, #30107, #30745, #40632, #20367, #27498, #36992, #21012, #37421, #27713, #33556, #7864, #4404, #30958, #27073, #1389, #33767, #36564, #3980, #7010, #33352, #17543, #14520, #11290, #1176, #16906, #20162, #13663, #26856, #17121, #10649, #10441, #23633, #17335, #36778, #10863, #7215, #20578, #30538, #14083, #23842, #7427, #27282, #40419, #24054, #7644, #4831, #21874, #38063, #38273, #18414, #24705, #25127, #2036, #8719, #35267, #35052, #25339, #12147, #22092, #41282, #1823, #41923, #17977, #21657, #34838, #31177, #38486, #5479, #41059, #1606, #5262, #8930, #11503, #37851, #11935, #15380, #18629, #24918, #31824, #8294, #32032, #2260, #5051, #28579, #21440, #14736, #34624, #8504, #28148, #18197, #31603, #31388, #41709, #2460, #8076, #11720, #5701, #18852, #15166, #27929, #14949, #24485, #28364, #15591, #41502, #28792, #21227, #37637, #34412, #22945, #38915, #19897, #6533, #35688, #3301, #9346, #32240, #22515, #39120, #16010, #6117, #9554, #19262, #36099, #33081, #38703, #42345, #71, #19685, #29205, #5906, #32454, #29847, #28997, #32870, #19059, #3089, #9138, #22306, #12568, #39324, #2880, #15801, #2667, #12981, #12777, #9970, #25969, #23150, #29628, #35479, #9764, #13195, #22728, #16429, #19474, #16645, #36311, #35893, #42137, #26388, #39540, #6330, #6744, #32660, #3508, #12355, #25552, #16217, #25762, #29417, #42557, #26178, #24224, #40170, #285, #26811, #13406, #39749, #10815, #30695, #1127, #24008, #10183, #4570, #7818, #20966, #39963, #10392, #14250, #37150, #23788, #27453, #17286, #23369, #27024, #36943, #10601, #37375, #16858, #40589, #36519, #13830, #27230, #6957, #40373, #7385, #14034, #20532, #504, #919, #33721, #7596, #11031, #20750, #34152, #17712, #26599, #17075, #20320, #20114, #33303, #4144, #30491, #3728, #30061, #33937, #13619, #23582, #4361, #36730, #7168, #33514, #17500, #3937, #30273, #711, #18587, #28533, #5008, #8247, #5648, #11245, #28104, #41232, #24442, #31774, #28312, #4782, #37588, #11670, #2203, #17930, #1561, #18370, #21827, #1991, #31345, #41452, #14692, #38438, #25083, #11458, #35006, #27881, #8032, #41013, #14904, #34578, #24659, #24870, #37801, #11887, #8882, #14472, #18150, #15336, #38228, #1775, #21176, #21394, #30907, #31128, #8673, #34366, #21615, #27666, #40804, #38019, #15117, #8463, #34794, #5214, #31558, #5435, #41665, #12100, #25295, #22045, #35217, #1343, #6487, #29158, #39280, #25916, #23101, #21, #38863, #12308, #12930, #22895, #2621, #9713, #19216, #3249, #36051, #9922, #15753, #19635, #16167, #32818, #12521, #13144, #15962, #18796, #28951, #31985, #15543, #29363, #16376, #29576, #42502, #28745, #36263, #26339, #39491, #42088, #25713, #2411, #26125, #42297, #41871, #35846, #25506, #2828, #12719, #39068, #38654, #35427, #9089, #22257, #32406, #3040, #5855, #19009, #9507, #32615, #22676, #32194, #19425, #6279, #9291, #22462, #35639, #6067, #20861, #16594, #4466, #14147, #37262, #237, #27777, #40482, #27994, #37700, #24771, #31023, #27564, #11355, #24549, #33253, #19845, #11563, #1026, #33029, #17608, #29797, #7926, #24341, #4256, #6693, #10135, #27347, #40913, #10929, #37482, #31242, #13359, #3459, #24123, #8142, #17398, #6904, #21075, #4680, #34264, #1453, #23314, #14588, #30804, #1669, #17828, #21290, #30596, #36469, #34476, #20058, #7712, #14366, #1242, #4898, #26551, #34045, #40698, #18046, #14798, #11141, #41123, #39699, #15013, #5324, #38124, #18478, #5112, #28848, #38334, #31665, #15441, #12621, #8569, #15229, #2724, #35112, #8359, #32303, #2099, #41345, #38764, #11997, #28210, #21933, #5754, #32088, #11781, #15857, #35326, #29055, #18907, #5966, #41772, #25397, #18686, #8777, #41983, #21719, #31884, #24983, #18261, #31450, #28428, #5537, #2314, #8984, #35537, #28639, #42194, #19117, #41564, #21510, #15648, #37915, #12204, #38543, #22151, #34902, #34692, #25193, #1884, #2522, #12413, #25606, #9190, #22361, #30118, #33362, #3782, #9612, #22786, #39806, #19956, #6588, #10238, #132, #35748, #9819, #19744, #23000, #7020, #42404, #26656, #22569, #39386, #10028, #6176, #23209, #36155, #39594, #32924, #26026, #26442, #3358, #36367, #36574, #6802, #23425, #13463, #20173, #42615, #3147, #555, #19316, #16490, #29689, #32510, #16916, #33144, #12836, #2939, #13255, #25814, #39179, #35946, #3572, #16706, #29903, #26237, #341, #6389, #38970, #9406, #19530, #16068, #32714, #29261, #16274, #29473, #13042, #37002, #40430, #23853, #24287, #34424, #40021, #975, #1401, #21022, #30547, #7226, #7437, #31188, #30334, #34213, #20377, #4415, #10451, #23643, #13887, #40644, #20590, #17133, #33566, #14310, #17344, #11301, #33778, #24495, #30971, #36789, #11086, #14531, #24066, #4629, #20806, #17988, #37648, #4200, #3990, #7875, #17775, #40226, #27725, #14093, #40861, #8088, #4843, #10660, #21238, #37432, #13675, #27294, #26867, #10873, #764, #37208, #27083, #7655, #33994, #17554, #30755, #1188, #27510, #28804, #18641, #11514, #28375, #25138, #41515, #25565, #18209, #2473, #41069, #15178, #28590, #24716, #41721, #11947, #15393, #38284, #1833, #2271, #21885, #12158, #12367, #25351, #15602, #32044, #41936, #18425, #21668, #19070, #37862, #8731, #35063, #8307, #38717, #38497, #31399, #21452, #5491, #9150, #14961, #28159, #31835, #35279, #8941, #2048, #22105, #41293, #22318, #5712, #24931, #18863, #11732, #34635, #38075, #35491, #5273, #8515, #5919, #34850, #1618, #14747, #27940, #31615, #5062, #39550, #6342, #25772, #12789, #6970, #6127, #9981, #38925, #22956, #29008, #42148, #32466, #16441, #25980, #35699, #9356, #32881, #35905, #29858, #39132, #296, #6754, #12579, #29640, #19908, #42569, #23160, #39337, #36530, #13417, #9565, #22526, #26399, #36323, #16021, #33093, #32672, #16657, #3521, #23380, #29217, #26612, #83, #39760, #22739, #10195, #29428, #32251, #42356, #2678, #19271, #13206, #15812, #2891, #19485, #3100, #16229, #12993, #26189, #9776, #36110, #6544, #19698, #3312, #37601, #514, #17299, #30504, #13629, #20978, #17513, #36741, #26821, #931, #7831, #7179, #33525, #7608, #11043, #33951, #20545, #30709, #3948, #27679, #14262, #724, #24237, #17086, #39974, #30285, #4155, #23801, #13843, #14047, #27038, #1139, #40817, #3739, #7397, #34165, #27465, #36955, #10405, #40182, #20126, #20332, #40600, #23596, #10827, #16869, #30072, #10613, #4373, #33733, #27243, #40384, #20762, #24020, #17724, #37161, #30919, #37388, #4584, #1354, #14484, #11257, #24454, #33314, #12319, #31996, #28116, #1574, #2217, #12113, #34590, #28544, #8473, #35229, #41676, #41884, #5021, #8892, #5447, #25306, #1787, #2422, #5226, #8044, #18162, #21190, #4794, #18598, #38451, #22056, #31785, #17942, #25517, #15555, #28757, #31356, #14916, #5660, #15346, #31570, #18811, #25094, #31141, #34805, #2002, #18381, #34378, #24670, #14703, #27893, #21627, #35018, #41026, #11469, #15129, #21838, #28325, #8258, #8685, #41464, #37815, #21404, #41243, #11684, #24881, #38030, #11898, #38240, #9724, #39503, #26350, #36276, #12731, #15973, #13371, #19020, #35857, #6291, #32205, #9934, #36063, #12532, #2634, #19434, #23113, #25725, #9305, #26138, #29590, #22907, #39080, #6498, #22474, #3471, #32833, #19227, #34, #35650, #15764, #6081, #22689, #42309, #32417, #32626, #2839, #19647, #16606, #22269, #25931, #6707, #3262, #9519, #28961, #29169, #38665, #38874, #16391, #42098, #29375, #35440, #5866, #3052, #13156, #16178, #42517, #12943, #39290, #19859, #33044, #29809, #249, #9101, #36481, #23968, #14212, #36903, #4321, #33683, #30865, #7780, #3902, #20070, #20710, #30658, #10353, #17459, #26976, #10991, #1086, #17670, #23544, #27411, #37113, #40547, #20286, #20924, #23750, #26563, #36693, #39712, #23329, #7557, #24186, #37333, #33898, #6918, #1301, #34106, #4528, #7132, #33474, #10147, #33265, #7348, #3691, #879, #16819, #10564, #20496, #4108, #30018, #465, #13580, #26772, #40136, #10779, #39925, #17036, #17249, #40337, #30450, #30236, #27193, #13998, #675, #13794, #37761, #31733, #25046, #28494, #31519, #11627, #41411, #11845, #1519, #14432, #27626, #8205, #11207, #28060, #37547, #5175, #21575, #40974, #40765, #14653, #4962, #38188, #21353, #18329, #15297, #4742, #24405, #31305, #21788, #34538, #24612, #1948, #8632, #28275, #34968, #11418, #5392, #37978, #7986, #18544, #2163, #18110, #1737, #15074, #14863, #41186, #34755, #8423, #21138, #17888, #24833, #34324, #31086, #27842, #13712, #10488, #37245, #30155, #20418, #23677, #33606, #20209, #1225, #10698, #4025, #30581, #27760, #36824, #30371, #17812, #7476, #23464, #4662, #17170, #26901, #11121, #27120, #595, #37040, #20846, #4450, #40057, #31008, #7692, #1437, #34030, #21058, #14131, #40466, #33816, #23892, #14350, #7266, #4239, #801, #33398, #3822, #13925, #20627, #17381, #24106, #7911, #1011, #14570, #34249, #40261, #36611, #30791, #10277, #27332, #10914, #17592, #27549, #7059, #40682, #16958, #24324, #37467, #5310, #31869, #5098, #11767, #8123, #38110, #18244, #28196, #2300, #1652, #41106, #25177, #18030, #8343, #11546, #21494, #21275, #15426, #41329, #34675, #18462, #15631, #24753, #31435, #5740, #8553, #11339, #35310, #1871, #14782, #41754, #14998, #31226, #24968, #8761, #35096, #27978, #18893, #38320, #32073, #21917, #8970, #2084, #28413, #21704, #34886, #28624, #37900, #31649, #15214, #34461, #4883, #41551, #11982, #5522, #18672, #38528, #12190, #2508, #22136, #25381, #24534, #40897, #37683, #35929, #29457, #22768, #29040, #28834, #2708, #22347, #22983, #26010, #6370, #19727, #35730, #42387, #38747, #39162, #6159, #16052, #35523, #6571, #19300, #6783, #16473, #3554, #9804, #19514, #32908, #3341, #12605, #41965, #33127, #22554, #12399, #9594, #9176, #42600, #3129, #25799, #25592, #32283, #32494, #29672, #2922, #16258, #10011, #5952, #19102, #29243, #116, #38955, #42178, #13026, #26219, #39367, #36140, #15840, #13237, #32698, #23189, #26425, #39576, #9389, #12819, #36350, #19938, #30492, #30908, #41014, #3938, #7597, #8033, #27667, #27025, #20967, #24009, #17931, #27231, #31129, #37589, #30274, #17713, #21177, #30696, #40805, #27454, #24660, #1562, #40374, #13831, #14473, #24443, #4145, #11246, #20751, #4783, #34367, #11459, #17287, #14693, #1344, #27882, #14035, #37802, #17501, #20321, #920, #33515, #17076, #712, #40171, #10602, #23789, #36944, #7386, #20533, #33722, #10816, #37151, #33938, #4362, #1128, #14251, #37376, #40590, #11032, #24225, #7819, #34153, #4571, #9090, #5009, #21828, #35218, #31346, #5649, #35007, #22046, #2204, #8464, #8883, #28534, #18797, #19010, #31986, #22258, #38655, #5856, #25084, #28313, #25714, #1776, #5436, #18588, #18151, #12522, #2412, #25296, #32195, #14905, #8248, #41453, #41872, #34795, #21616, #38439, #15544, #28746, #12309, #24871, #25507, #31775, #2622, #35428, #15754, #5215, #38020, #11671, #31559, #28105, #28952, #15337, #42089, #41233, #18371, #41666, #21395, #34579, #1992, #15118, #11888, #38229, #8674, #12101, #19426, #6068, #29798, #39281, #32616, #16377, #13569, #453, #29364, #238, #22677, #39069, #13145, #36264, #9923, #19846, #12720, #33030, #36052, #20059, #23102, #26552, #35847, #25917, #42298, #3041, #2829, #26340, #6488, #13360, #35640, #9508, #9714, #39700, #10136, #6280, #16168, #6694, #15963, #42503, #12931, #26126, #19217, #23315, #22896, #19636, #29577, #38864, #32819, #3250, #3680, #22, #9292, #33254, #39492, #3460, #36470, #16595, #29159, #6905, #16808, #30007, #22463, #32407, #24174, #21125, #37321, #37535, #30643, #14199 ),
 ( #4308, #30853, #1291, #10553, #39912, #31075, #20485, #10343, #37101, #36681, #27399, #1074, #23739, #26760, #10768, #7121, #1508, #40535, #10978, #7975, #20276, #7768, #33464, #23957, #7544, #20698, #34314, #663, #27614, #23531, #40326, #20911, #3890, #34094, #33886, #4515, #17447, #26965, #17659, #14420, #40754, #4730, #11196, #24394, #17878, #17025, #869, #4096, #30224, #13782, #40123, #36892, #7336, #33671, #17238, #30438, #13985, #27182, #2363, #1725, #28049, #2151, #5591, #28483, #15063, #25245, #41175, #22204, #8831, #37967, #18744, #11614, #34528, #24822, #41400, #38599, #34744, #37749, #8412, #38390, #35379, #40963, #1937, #15490, #21988, #31507, #8193, #21563, #32144, #31294, #35165, #21340, #5380, #11406, #24600, #14852, #41615, #5165, #18099, #4952, #15286, #18317, #12259, #28262, #25454, #31936, #11834, #12049, #28695, #25035, #41822, #21777, #18957, #9039, #38177, #8621, #5804, #14642, #34956, #27831, #18531, #31721, #36209, #36423, #42248, #3411, #42670, #6645, #39024, #26501, #42459, #2574, #29112, #15703, #42037, #13094, #32982, #16547, #26295, #12466, #6858, #10087, #23264, #12673, #25869, #29745, #39444, #26081, #191, #9460, #23052, #2993, #13312, #19795, #20010, #22627, #39648, #9879, #28902, #35801, #25660, #12887, #38815, #6232, #9242, #22412, #35590, #6018, #19168, #32358, #2782, #15910, #19378, #32566, #16118, #29315, #39232, #9670, #22843, #36005, #19584, #6441, #32767, #3203, #16329, #29528, #7076, #34047, #29961, #4044, #17400, #13523, #30598, #17188, #4258, #27134, #33415, #33833, #10717, #1028, #1244, #14150, #4469, #20863, #30806, #7284, #10506, #7928, #26709, #30386, #10931, #23481, #40277, #39861, #20225, #10295, #13941, #17611, #3842, #16976, #20647, #24125, #27349, #33622, #40485, #30174, #40700, #37265, #13728, #7714, #612, #36629, #26917, #819, #14369, #23693, #40075, #36840, #27566, #11144, #16761, #20437, #24343, #37485, #23911, #37056, #7494, #33202, #3633, #401, #27780, #11784, #17830, #31026, #21292, #5326, #14800, #24552, #40915, #21721, #24773, #18691, #27996, #31887, #38337, #1456, #18481, #8779, #31452, #41567, #28214, #25400, #2317, #41126, #14590, #15233, #25196, #15444, #1886, #38546, #28643, #31244, #34266, #12001, #41774, #41347, #34904, #15015, #34479, #21078, #37702, #11357, #28431, #18263, #24985, #21936, #11566, #34694, #8144, #38128, #37917, #8361, #4901, #35116, #21513, #12207, #5540, #4682, #2103, #8571, #18048, #1672, #5114, #31669, #13258, #2728, #35330, #19319, #18910, #9616, #26030, #5969, #8987, #35752, #32092, #26445, #22789, #39182, #32928, #2526, #22155, #42197, #42618, #35540, #9194, #35950, #6392, #19533, #32717, #25609, #3150, #6180, #3361, #16279, #39389, #19121, #38767, #12416, #32306, #15651, #29476, #32513, #13046, #5757, #22364, #22572, #26240, #9822, #15860, #29059, #23004, #28851, #12624, #25818, #38973, #41987, #36158, #9409, #2942, #29264, #16071, #42408, #12839, #16494, #6591, #19748, #29692, #136, #345, #40434, #13679, #29906, #23646, #7441, #33782, #16709, #17559, #37006, #33998, #20594, #7659, #767, #27086, #20380, #10455, #30552, #23429, #33570, #13466, #6806, #19961, #7024, #40025, #3993, #10664, #4205, #4419, #17348, #20812, #13893, #40229, #17136, #36792, #979, #36577, #30338, #26659, #33147, #3576, #20176, #7229, #23857, #14097, #37212, #27299, #1192, #30759, #33365, #10031, #10878, #14314, #24070, #39597, #23213, #39809, #36370, #10241, #3786, #16920, #30121, #558, #26870, #35019, #41677, #38031, #25307, #5448, #15347, #21628, #5867, #18599, #6082, #15765, #2840, #9102, #5661, #32206, #2635, #11899, #41244, #32418, #21839, #11685, #38452, #8474, #28758, #2423, #25095, #27514, #12114, #34806, #24882, #41885, #15556, #9306, #5227, #18382, #31786, #19021, #38241, #28326, #12320, #25518, #38666, #22270, #2003, #35441, #8893, #22475, #28962, #42099, #8686, #15130, #31571, #2218, #41465, #12533, #22057, #25726, #28545, #35230, #18812, #38875, #35651, #31997, #19228, #250, #35858, #26139, #16179, #39291, #25932, #6919, #16392, #9725, #36277, #33475, #29376, #36064, #23545, #13157, #29170, #10354, #22908, #19435, #16820, #32834, #6292, #35, #26564, #10148, #32627, #36694, #42310, #7133, #6499, #3053, #30019, #3263, #42518, #26351, #39713, #23330, #12944, #20287, #13372, #15974, #36482, #26773, #19860, #3472, #39504, #29591, #20071, #19648, #9935, #23114, #39081, #9520, #6708, #33045, #16607, #29810, #13581, #33266, #12732, #39926, #3692, #22690, #466, #40975, #10992, #4529, #40548, #4109, #3903, #20497, #40137, #40766, #1087, #24187, #37548, #10780, #17460, #13795, #14213, #23969, #33899, #10565, #24406, #37114, #24613, #34325, #21354, #27627, #37334, #7987, #21139, #30451, #17037, #8206, #40338, #30237, #27412, #26977, #17671, #20925, #880, #676, #30659, #23751, #36904, #30866, #34107, #27843, #7349, #33684, #7558, #4743, #13999, #17250, #1302, #14433, #11208, #17889, #27194, #31087, #7781, #11419, #1520, #14654, #20711, #4322, #37762, #15075, #41187, #8843, #2164, #25467, #31306, #37979, #5393, #38612, #9049, #8424, #34756, #18756, #11628, #1949, #5176, #28276, #1738, #22215, #34969, #41412, #12060, #9254, #18330, #11846, #42050, #31734, #15298, #4963, #28913, #25047, #21576, #35391, #8633, #24834, #18545, #2374, #28706, #31520, #12478, #31946, #25671, #15501, #2585, #38401, #22001, #28495, #41626, #5815, #38189, #25256, #21789, #14864, #28061, #35177, #5602, #41833, #12270, #32155, #18968, #38825, #15714, #34539, #18111, #201, #16770, #29538, #23064, #16340, #22638, #22423, #39034, #15922, #16558, #19595, #42680, #13322, #29325, #36015, #32368, #32777, #42469, #9680, #29123, #26511, #12896, #412, #10096, #39870, #3421, #13106, #39660, #23273, #6243, #35601, #26718, #16128, #6029, #3213, #2792, #36220, #39454, #19387, #19179, #6454, #42258, #12683, #6655, #9889, #3643, #25880, #9470, #26091, #36432, #32578, #35811, #19805, #32993, #29756, #6868, #3004, #20019, #26305, #29970, #33212, #13532, #39242, #22853, #13737, #33631, #16985, #27359, #20656, #1254, #7085, #26927, #23920, #14378, #27575, #40085, #10515, #37276, #30184, #20445, #23702, #4054, #20235, #40711, #10728, #17196, #30607, #27790, #36851, #30397, #17839, #11153, #37064, #828, #1035, #10304, #7295, #13950, #31035, #7504, #23492, #4690, #27143, #40286, #24352, #33843, #621, #4268, #20871, #4478, #17409, #1466, #7724, #14600, #34057, #21087, #14160, #40494, #10940, #24134, #37493, #17621, #30815, #7937, #33424, #3851, #34275, #36639, #34914, #12010, #38556, #8582, #2536, #8997, #8372, #11366, #18702, #35339, #5336, #41578, #18491, #41134, #40923, #14809, #34489, #35126, #38138, #31679, #31898, #5124, #11794, #8153, #21732, #18272, #28224, #4911, #2326, #31461, #18920, #28653, #15661, #21946, #2113, #15455, #41784, #24781, #24562, #37711, #34704, #21301, #15243, #18059, #25206, #28442, #37926, #31254, #24997, #1681, #28006, #38348, #8788, #22165, #11575, #21522, #1895, #12218, #15024, #41357, #5550, #25410, #5767, #32103, #2741, #23014, #26041, #10041, #13057, #16505, #12634, #15868, #32316, #9419, #35550, #3161, #39193, #19757, #25621, #29070, #42418, #32940, #3370, #42208, #25828, #26250, #5980, #38982, #22585, #35762, #38778, #19131, #12849, #39400, #36168, #6190, #6816, #9835, #23223, #6601, #39607, #32727, #16289, #9627, #22799, #29702, #19332, #35963, #32524, #9204, #22373, #2953, #29275, #6402, #42627, #26457, #19543, #33157, #36383, #16080, #41997, #148, #19971, #29488, #13268, #3587, #28862, #12426, #33376, #10252, #10888, #13902, #23867, #7667, #23654, #30347, #26669, #27095, #36801, #4003, #23439, #37220, #7239, #37444, #4428, #34225, #40444, #37015, #20820, #34006, #568, #29916, #21035, #10464, #357, #40237, #39820, #17357, #33791, #13687, #16721, #776, #36587, #13478, #30559, #4214, #40657, #7034, #20186, #20389, #17567, #26879, #16932, #988, #14106, #27307, #24080, #3796, #30767, #10673, #11097, #1199, #14326, #40034, #30131, #33582, #17146, #7455, #27522, #20604, #24300, #7887, #8099, #18221, #8741, #38296, #21250, #4857, #31627, #24506, #14758, #17999, #27953, #14545, #21895, #5075, #41081, #24942, #22113, #31201, #24728, #12169, #1846, #17788, #41730, #11525, #34436, #5500, #21463, #1629, #37873, #18650, #41528, #28171, #31844, #21681, #27737, #31411, #41305, #14972, #28600, #8318, #2281, #1414, #11743, #2060, #40873, #15190, #38086, #18437, #8526, #34647, #5284, #34862, #28387, #15402, #11958, #25359, #35075, #38507, #25148, #8950, #4641, #11314, #30985, #37659, #25572, #29225, #41945, #9157, #15610, #16030, #22965, #22326, #5927, #22747, #26197, #6350, #35707, #3108, #19079, #92, #29438, #15821, #39344, #32259, #12377, #2688, #19281, #16452, #12587, #28814, #29018, #16237, #13214, #18872, #22534, #36119, #42579, #9365, #38725, #42156, #9989, #35501, #13002, #25780, #25991, #32053, #2482, #38933, #19494, #6137, #32475, #2899, #35914, #42364, #32889, #12797, #3319, #9785, #39142, #32680, #6552, #9573, #19706, #29650, #39558, #26409, #35287, #5720, #17309, #27251, #6980, #939, #23606, #7617, #14058, #14271, #20135, #24030, #20553, #40391, #16879, #4381, #20341, #23168, #33322, #36331, #19917, #33742, #10836, #37169, #4164, #33106, #27472, #30721, #1148, #40608, #6762, #3530, #3747, #30082, #20771, #30512, #3956, #33959, #40193, #16665, #7187, #17094, #33534, #17520, #39769, #29865, #305, #36751, #7406, #13423, #26620, #30294, #36963, #733, #23389, #23809, #13852, #10203, #36539, #522, #13637, #26829, #39983, #10413, #27047, #10622, #34174, #8267, #31580, #1362, #5031, #17733, #27687, #4593, #34600, #41477, #40824, #24462, #41253, #2012, #24892, #11478, #21636, #37609, #18608, #5238, #34386, #15140, #8052, #30927, #21200, #37826, #35029, #31151, #14494, #4803, #34815, #31799, #37397, #41035, #11909, #18392, #27902, #11266, #17951, #28555, #1582, #28339, #14712, #1799, #7840, #20987, #24679, #38041, #21415, #18171, #31365, #11696, #14926, #8697, #28125, #21850, #25104, #8483, #38250, #5458, #2231, #15357, #11051, #24246, #23500, #19034, #35242, #35871, #3067, #25530, #19449, #42112, #26152, #32640, #33432, #38679, #42532, #39094, #16193, #35455, #36649, #38888, #41687, #9113, #12126, #38463, #9533, #29391, #12957, #22703, #8904, #22068, #39303, #12546, #22282, #19241, #16995, #12331, #32217, #7093, #9318, #25317, #20243, #5879, #2433, #10313, #15776, #32008, #25738, #6304, #3859, #18824, #5673, #15568, #28769, #41897, #2645, #2854, #29183, #22488, #35663, #28972, #6094, #32430, #15987, #42323, #12746, #25945, #30614, #24144, #1261, #27798, #40502, #34497, #40930, #40293, #628, #7943, #24569, #37283, #30823, #7730, #30404, #30192, #4061, #23708, #24359, #27366, #20878, #21094, #37071, #1042, #40092, #10947, #7514, #17416, #36859, #34282, #20663, #8160, #17846, #4918, #11160, #34064, #4697, #31043, #13957, #13745, #26934, #23927, #10524, #4486, #7302, #14385, #17628, #27151, #20452, #14167, #33640, #17203, #27582, #40720, #11372, #835, #10735, #33851, #1474, #4275, #37501, #14609, #37718, #21308, #41791, #34711, #12226, #15250, #42004, #2334, #5774, #1902, #5133, #21529, #41365, #24789, #35134, #28451, #9005, #14817, #18279, #31686, #22173, #35346, #31469, #15031, #15462, #37934, #28230, #11802, #25004, #11581, #25418, #18928, #38146, #38563, #18498, #2543, #32111, #9210, #8589, #15669, #28661, #28870, #21742, #12432, #41585, #18066, #34921, #31263, #28014, #25628, #38785, #22381, #35559, #41142, #1688, #8379, #5343, #2120, #12017, #25213, #38357, #8795, #21953, #5558, #18711, #31904, #29494, #3169, #29922, #22591, #6822, #2748, #19549, #32946, #29077, #3376, #32733, #19763, #42634, #6196, #6609, #26258, #16512, #16727, #29710, #19976, #36389, #3596, #22806, #26048, #23445, #42214, #16296, #26464, #38989, #13063, #12641, #35768, #25834, #39407, #33165, #19341, #32531, #36173, #39613, #154, #6408, #13274, #2959, #13486, #10049, #29281, #23229, #16086, #9426, #42425, #9842, #364, #39199, #12855, #9634, #26675, #39826, #32322, #35971, #10259, #5986, #23020, #19137, #15875, #7894, #26885, #37226, #16940, #33797, #20193, #33382, #10471, #14113, #33588, #40040, #30137, #994, #784, #1207, #4009, #14332, #34013, #3801, #27315, #4434, #23873, #7675, #7461, #37450, #27528, #17152, #13908, #30353, #36594, #575, #37021, #20827, #13693, #20611, #23661, #36808, #7246, #4223, #17573, #20396, #27101, #40450, #30775, #10894, #40244, #24087, #10680, #24307, #40663, #17364, #11104, #30565, #7042, #42558, #16430, #13620, #9765, #12778, #12982, #286, #10393, #16011, #19686, #20115, #39750, #6534, #25970, #26179, #7169, #6331 ) ),
 .UNSPECIFIED., .F., .F., .F. ) 
 B_SPLINE_SURFACE_WITH_KNOTS ( ( 2, 2 ),
 ( 3, 2, 2, 2, 2, 2, 2, 2, 2, 2, 2, 2, 2, 2, 2, 2, 2, 2, 2, 2, 2, 2, 2, 2, 2, 2, 2, 2, 2, 2, 2, 2, 2, 2, 2, 2, 2, 2, 2, 2, 2, 2, 2, 2, 2, 2, 2, 2, 2, 2, 2, 2, 2, 2, 2, 2, 2, 2, 2, 2, 2, 2, 2, 2, 2, 2, 2, 2, 2, 2, 2, 2, 2, 2, 2, 2, 2, 2, 2, 2, 2, 2, 2, 2, 2, 2, 2, 2, 2, 2, 2, 2, 2, 2, 2, 2, 2, 2, 2, 2, 2, 2, 2, 2, 2, 2, 2, 2, 2, 2, 2, 2, 2, 2, 2, 2, 2, 2, 2, 2, 2, 2, 2, 2, 2, 2, 2, 2, 2, 2, 2, 2, 2, 2, 2, 2, 2, 2, 2, 2, 2, 2, 2, 2, 2, 2, 2, 2, 2, 2, 2, 2, 2, 2, 2, 2, 2, 2, 2, 2, 2, 2, 2, 2, 2, 2, 2, 2, 2, 2, 2, 2, 2, 2, 2, 2, 2, 2, 2, 2, 2, 2, 2, 2, 2, 2, 2, 2, 2, 2, 2, 2, 2, 2, 2, 2, 2, 2, 2, 2, 2, 2, 2, 2, 2, 2, 2, 2, 2, 2, 2, 2, 2, 2, 2, 2, 2, 2, 2, 2, 2, 2, 2, 2, 2, 2, 2, 2, 2, 2, 2, 2, 2, 2, 2, 2, 2, 2, 2, 2, 2, 2, 2, 2, 2, 2, 2, 2, 2, 2, 2, 2, 2, 2, 2, 2, 2, 2, 2, 2, 2, 2, 2, 2, 2, 2, 2, 2, 2, 2, 2, 2, 2, 2, 2, 2, 2, 2, 2, 2, 2, 2, 2, 2, 2, 2, 2, 2, 2, 2, 2, 2, 2, 2, 2, 2, 2, 2, 2, 2, 2, 2, 2, 2, 2, 2, 2, 2, 2, 2, 2, 2, 2, 2, 2, 2, 2, 2, 2, 2, 2, 2, 2, 2, 2, 2, 2, 2, 2, 2, 2, 2, 2, 2, 2, 2, 2, 2, 2, 2, 2, 2, 2, 2, 2, 2, 2, 2, 2, 2, 2, 2, 2, 2, 2, 2, 2, 2, 2, 2, 2, 2, 2, 2, 2, 2, 2, 2, 2, 2, 2, 2, 2, 2, 2, 2, 2, 2, 2, 2, 2, 2, 2, 2, 2, 2, 2, 2, 2, 2, 2, 2, 2, 2, 2, 2, 2, 2, 2, 2, 2, 2, 2, 2, 2, 2, 2, 2, 2, 2, 2, 2, 2, 2, 2, 2, 2, 2, 2, 2, 2, 2, 2, 2, 2, 2, 2, 2, 2, 2, 2, 2, 2, 2, 2, 2, 2, 2, 2, 2, 2, 2, 2, 2, 2, 2, 2, 2, 2, 2, 2, 2, 2, 2, 2, 2, 2, 2, 2, 2, 2, 2, 2, 2, 2, 2, 2, 2, 2, 2, 2, 2, 2, 2, 2, 2, 2, 2, 2, 2, 2, 2, 2, 2, 2, 2, 2, 2, 2, 2, 2, 2, 2, 2, 2, 2, 2, 2, 2, 2, 2, 2, 2, 2, 2, 2, 2, 2, 2, 2, 2, 2, 2, 2, 2, 2, 2, 2, 2, 2, 2, 2, 2, 2, 2, 2, 2, 2, 2, 2, 2, 2, 2, 2, 2, 2, 2, 2, 2, 2, 2, 2, 2, 2, 2, 2, 2, 2, 2, 2, 2, 2, 2, 2, 2, 2, 2, 2, 2, 2, 2, 2, 2, 2, 2, 2, 2, 2, 2, 2, 2, 2, 2, 2, 2, 2, 2, 2, 2, 2, 2, 2, 2, 2, 2, 2, 2, 2, 2, 2, 2, 2, 2, 2, 2, 2, 2, 2, 2, 2, 2, 2, 2, 2, 2, 2, 2, 2, 2, 2, 2, 2, 2, 2, 2, 2, 2, 2, 2, 2, 2, 2, 2, 2, 2, 2, 2, 2, 2, 2, 2, 2, 2, 2, 2, 2, 2, 2, 2, 2, 2, 2, 2, 2, 2, 2, 2, 2, 2, 2, 2, 2, 2, 2, 2, 2, 2, 2, 2, 2, 2, 2, 2, 2, 2, 2, 2, 2, 2, 2, 2, 2, 2, 2, 2, 2, 2, 2, 2, 2, 2, 2, 2, 2, 2, 2, 2, 2, 2, 2, 2, 2, 2, 2, 2, 2, 2, 2, 2, 2, 2, 2, 2, 2, 2, 2, 2, 2, 2, 2, 2, 2, 2, 2, 2, 2, 2, 2, 2, 2, 2, 2, 2, 2, 2, 2, 2, 2, 2, 2, 2, 2, 2, 2, 2, 2, 2, 2, 2, 2, 2, 2, 2, 2, 2, 2, 2, 2, 2, 2, 2, 2, 2, 2, 2, 2, 2, 2, 2, 2, 2, 2, 2, 2, 2, 2, 2, 2, 2, 2, 2, 2, 2, 2, 2, 2, 2, 2, 2, 2, 2, 2, 2, 2, 2, 2, 2, 2, 2, 2, 2, 2, 2, 2, 2, 2, 2, 2, 2, 2, 3 ),
 ( 0.000000000000000000, 1.000000000000000000 ),
 ( 0.000000000000000000, 0.001243781094527363160, 0.002487562189054726321, 0.003731343283582089481, 0.004975124378109452641, 0.006218905472636816235, 0.007462686567164178962, 0.008706467661691542556, 0.009950248756218905283, 0.01119402985074626801, 0.01243781094527363247, 0.01368159203980099520, 0.01492537313432835792, 0.01616915422885572065, 0.01741293532338308511, 0.01865671641791044610, 0.01990049751243781057, 0.02114427860696517503, 0.02238805970149253602, 0.02363184079601990048, 0.02487562189054726494, 0.02611940298507462593, 0.02736318407960199039, 0.02860696517412935486, 0.02985074626865671585, 0.03109452736318408031, 0.03233830845771144130, 0.03358208955223880576, 0.03482587064676617022, 0.03606965174129353469, 0.03731343283582089221, 0.03855721393034825667, 0.03980099502487562113, 0.04104477611940298559, 0.04228855721393035005, 0.04353233830845771452, 0.04477611940298507204, 0.04601990049751243650, 0.04726368159203980096, 0.04850746268656716542, 0.04975124378109452988, 0.05099502487562188741, 0.05223880597014925187, 0.05348258706467661633, 0.05472636815920398079, 0.05597014925373134525, 0.05721393034825870971, 0.05845771144278606724, 0.05970149253731343170, 0.06094527363184079616, 0.06218905472636816062, 0.06343283582089552508, 0.06467661691542288260, 0.06592039800995025400, 0.06716417910447761153, 0.06840796019900496905, 0.06965174129353234045, 0.07089552238805969797, 0.07213930348258706937, 0.07338308457711442689, 0.07462686567164178442, 0.07587064676616915582, 0.07711442786069651334, 0.07835820895522388474, 0.07960199004975124226, 0.08084577114427861366, 0.08208955223880597118, 0.08333333333333332871, 0.08457711442786070011, 0.08582089552238805763, 0.08706467661691542903, 0.08830845771144278655, 0.08955223880597014408, 0.09079601990049751548, 0.09203980099502487300, 0.09328358208955224440, 0.09452736318407960192, 0.09577114427860695944, 0.09701492537313433084, 0.09825870646766168837, 0.09950248756218905977, 0.1007462686567164173, 0.1019900497512437748, 0.1032338308457711462, 0.1044776119402985037, 0.1057213930348258751, 0.1069651741293532327, 0.1082089552238805902, 0.1094527363184079616, 0.1106965174129353191, 0.1119402985074626905, 0.1131840796019900480, 0.1144278606965174194, 0.1156716417910447769, 0.1169154228855721345, 0.1181592039800995059, 0.1194029850746268634, 0.1206467661691542348, 0.1218905472636815923, 0.1231343283582089498, 0.1243781094527363212, 0.1256218905472636926, 0.1268656716417910502, 0.1281094527363184077, 0.1293532338308457652, 0.1305970149253731227, 0.1318407960199005080, 0.1330845771144278655, 0.1343283582089552231, 0.1355721393034825806, 0.1368159203980099381, 0.1380597014925373234, 0.1393034825870646809, 0.1405472636815920384, 0.1417910447761193959, 0.1430348258706467535, 0.1442786069651741387, 0.1455223880597014963, 0.1467661691542288538, 0.1480099502487562113, 0.1492537313432835688, 0.1504975124378109541, 0.1517412935323383116, 0.1529850746268656692, 0.1542288557213930267, 0.1554726368159203842, 0.1567164179104477695, 0.1579601990049751270, 0.1592039800995024845, 0.1604477611940298420, 0.1616915422885572273, 0.1629353233830845848, 0.1641791044776119424, 0.1654228855721392999, 0.1666666666666666574, 0.1679104477611940427, 0.1691542288557214002, 0.1703980099502487577, 0.1716417910447761153, 0.1728855721393034728, 0.1741293532338308581, 0.1753731343283582156, 0.1766169154228855731, 0.1778606965174129306, 0.1791044776119402882, 0.1803482587064676734, 0.1815920398009950310, 0.1828358208955223885, 0.1840796019900497460, 0.1853233830845771035, 0.1865671641791044888, 0.1878109452736318463, 0.1890547263681592038, 0.1902985074626865614, 0.1915422885572139189, 0.1927860696517413042, 0.1940298507462686617, 0.1952736318407960192, 0.1965174129353233767, 0.1977611940298507343, 0.1990049751243781195, 0.2002487562189054771, 0.2014925373134328346, 0.2027363184079601921, 0.2039800995024875496, 0.2052238805970149349, 0.2064676616915422924, 0.2077114427860696499, 0.2089552238805970075, 0.2101990049751243650, 0.2114427860696517503, 0.2126865671641791078, 0.2139303482587064653, 0.2151741293532338228, 0.2164179104477611804, 0.2176616915422885656, 0.2189054726368159232, 0.2201492537313432807, 0.2213930348258706382, 0.2226368159203980235, 0.2238805970149253810, 0.2251243781094527385, 0.2263681592039800961, 0.2276119402985074536, 0.2288557213930348389, 0.2300995024875621964, 0.2313432835820895539, 0.2325870646766169114, 0.2338308457711442689, 0.2350746268656716542, 0.2363184079601990117, 0.2375621890547263693, 0.2388059701492537268, 0.2400497512437810843, 0.2412935323383084696, 0.2425373134328358271, 0.2437810945273631846, 0.2450248756218905422, 0.2462686567164178997, 0.2475124378109452850, 0.2487562189054726425, 0.2500000000000000000, 0.2512437810945273853, 0.2524875621890547150, 0.2537313432835821003, 0.2549751243781094301, 0.2562189054726368154, 0.2574626865671642006, 0.2587064676616915304, 0.2599502487562189157, 0.2611940298507462455, 0.2624378109452736307, 0.2636815920398010160, 0.2649253731343283458, 0.2661691542288557311, 0.2674129353233830608, 0.2686567164179104461, 0.2699004975124378314, 0.2711442786069651611, 0.2723880597014925464, 0.2736318407960198762, 0.2748756218905472615, 0.2761194029850746468, 0.2773631840796019765, 0.2786069651741293618, 0.2798507462686566916, 0.2810945273631840768, 0.2823383084577114621, 0.2835820895522387919, 0.2848258706467661772, 0.2860696517412935069, 0.2873134328358208922, 0.2885572139303482775, 0.2898009950248756073, 0.2910447761194029925, 0.2922885572139303223, 0.2935323383084577076, 0.2947761194029850929, 0.2960199004975124226, 0.2972636815920398079, 0.2985074626865671377, 0.2997512437810945229, 0.3009950248756219082, 0.3022388059701492380, 0.3034825870646766233, 0.3047263681592039530, 0.3059701492537313383, 0.3072139303482587236, 0.3084577114427860534, 0.3097014925373134386, 0.3109452736318407684, 0.3121890547263681537, 0.3134328358208955390, 0.3146766169154228687, 0.3159203980099502540, 0.3171641791044776393, 0.3184079601990049690, 0.3196517412935323543, 0.3208955223880596841, 0.3221393034825870694, 0.3233830845771144546, 0.3246268656716417844, 0.3258706467661691697, 0.3271144278606964995, 0.3283582089552238847, 0.3296019900497512700, 0.3308457711442785998, 0.3320895522388059851, 0.3333333333333333148, 0.3345771144278607001, 0.3358208955223880854, 0.3370646766169154152, 0.3383084577114428004, 0.3395522388059701302, 0.3407960199004975155, 0.3420398009950249008, 0.3432835820895522305, 0.3445273631840796158, 0.3457711442786069456, 0.3470149253731343308, 0.3482587064676617161, 0.3495024875621890459, 0.3507462686567164312, 0.3519900497512437609, 0.3532338308457711462, 0.3544776119402985315, 0.3557213930348258613, 0.3569651741293532465, 0.3582089552238805763, 0.3594527363184079616, 0.3606965174129353469, 0.3619402985074626766, 0.3631840796019900619, 0.3644278606965173917, 0.3656716417910447769, 0.3669154228855721622, 0.3681592039800994920, 0.3694029850746268773, 0.3706467661691542070, 0.3718905472636815923, 0.3731343283582089776, 0.3743781094527363074, 0.3756218905472636926, 0.3768656716417910224, 0.3781094527363184077, 0.3793532338308457930, 0.3805970149253731227, 0.3818407960199005080, 0.3830845771144278378, 0.3843283582089552231, 0.3855721393034826083, 0.3868159203980099381, 0.3880597014925373234, 0.3893034825870646531, 0.3905472636815920384, 0.3917910447761194237, 0.3930348258706467535, 0.3942786069651741387, 0.3955223880597014685, 0.3967661691542288538, 0.3980099502487562391, 0.3992537313432835688, 0.4004975124378109541, 0.4017412935323382839, 0.4029850746268656692, 0.4042288557213930544, 0.4054726368159203842, 0.4067164179104477695, 0.4079601990049750992, 0.4092039800995024845, 0.4104477611940298698, 0.4116915422885571996, 0.4129353233830845848, 0.4141791044776119146, 0.4154228855721392999, 0.4166666666666666852, 0.4179104477611940149, 0.4191542288557214002, 0.4203980099502487300, 0.4216417910447761153, 0.4228855721393035005, 0.4241293532338308303, 0.4253731343283582156, 0.4266169154228855454, 0.4278606965174129306, 0.4291044776119403159, 0.4303482587064676457, 0.4315920398009950310, 0.4328358208955223607, 0.4340796019900497460, 0.4353233830845771313, 0.4365671641791044610, 0.4378109452736318463, 0.4390547263681592316, 0.4402985074626865614, 0.4415422885572139466, 0.4427860696517412764, 0.4440298507462686617, 0.4452736318407960470, 0.4465174129353233767, 0.4477611940298507620, 0.4490049751243780918, 0.4502487562189054771, 0.4514925373134328623, 0.4527363184079601921, 0.4539800995024875774, 0.4552238805970149071, 0.4564676616915422924, 0.4577114427860696777, 0.4589552238805970075, 0.4601990049751243927, 0.4614427860696517225, 0.4626865671641791078, 0.4639303482587064931, 0.4651741293532338228, 0.4664179104477612081, 0.4676616915422885379, 0.4689054726368159232, 0.4701492537313433084, 0.4713930348258706382, 0.4726368159203980235, 0.4738805970149253532, 0.4751243781094527385, 0.4763681592039801238, 0.4776119402985074536, 0.4788557213930348389, 0.4800995024875621686, 0.4813432835820895539, 0.4825870646766169392, 0.4838308457711442689, 0.4850746268656716542, 0.4863184079601989840, 0.4875621890547263693, 0.4888059701492537545, 0.4900497512437810843, 0.4912935323383084696, 0.4925373134328357994, 0.4937810945273631846, 0.4950248756218905699, 0.4962686567164178997, 0.4975124378109452850, 0.4987562189054726147, 0.5000000000000000000, 0.5012437810945273853, 0.5024875621890547706, 0.5037313432835820448, 0.5049751243781094301, 0.5062189054726368154, 0.5074626865671642006, 0.5087064676616915859, 0.5099502487562188602, 0.5111940298507462455, 0.5124378109452736307, 0.5136815920398010160, 0.5149253731343284013, 0.5161691542288556755, 0.5174129353233830608, 0.5186567164179104461, 0.5199004975124378314, 0.5211442786069652167, 0.5223880597014924909, 0.5236318407960198762, 0.5248756218905472615, 0.5261194029850746468, 0.5273631840796020320, 0.5286069651741293063, 0.5298507462686566916, 0.5310945273631840768, 0.5323383084577114621, 0.5335820895522388474, 0.5348258706467661217, 0.5360696517412935069, 0.5373134328358208922, 0.5385572139303482775, 0.5398009950248756628, 0.5410447761194029370, 0.5422885572139303223, 0.5435323383084577076, 0.5447761194029850929, 0.5460199004975124781, 0.5472636815920397524, 0.5485074626865671377, 0.5497512437810945229, 0.5509950248756219082, 0.5522388059701492935, 0.5534825870646765678, 0.5547263681592039530, 0.5559701492537313383, 0.5572139303482587236, 0.5584577114427861089, 0.5597014925373133831, 0.5609452736318407684, 0.5621890547263681537, 0.5634328358208955390, 0.5646766169154229242, 0.5659203980099501985, 0.5671641791044775838, 0.5684079601990049690, 0.5696517412935323543, 0.5708955223880597396, 0.5721393034825870139, 0.5733830845771143991, 0.5746268656716417844, 0.5758706467661691697, 0.5771144278606965550, 0.5783582089552238292, 0.5796019900497512145, 0.5808457711442785998, 0.5820895522388059851, 0.5833333333333333703, 0.5845771144278606446, 0.5858208955223880299, 0.5870646766169154152, 0.5883084577114428004, 0.5895522388059701857, 0.5907960199004974600, 0.5920398009950248452, 0.5932835820895522305, 0.5945273631840796158, 0.5957711442786070011, 0.5970149253731342753, 0.5982587064676616606, 0.5995024875621890459, 0.6007462686567164312, 0.6019900497512438164, 0.6032338308457710907, 0.6044776119402984760, 0.6057213930348258613, 0.6069651741293532465, 0.6082089552238806318, 0.6094527363184079061, 0.6106965174129352913, 0.6119402985074626766, 0.6131840796019900619, 0.6144278606965174472, 0.6156716417910447214, 0.6169154228855721067, 0.6181592039800994920, 0.6194029850746268773, 0.6206467661691542625, 0.6218905472636815368, 0.6231343283582089221, 0.6243781094527363074, 0.6256218905472636926, 0.6268656716417910779, 0.6281094527363184632, 0.6293532338308457375, 0.6305970149253731227, 0.6318407960199005080, 0.6330845771144278933, 0.6343283582089552786, 0.6355721393034825528, 0.6368159203980099381, 0.6380597014925373234, 0.6393034825870647087, 0.6405472636815920939, 0.6417910447761193682, 0.6430348258706467535, 0.6442786069651741387, 0.6455223880597015240, 0.6467661691542289093, 0.6480099502487561836, 0.6492537313432835688, 0.6504975124378109541, 0.6517412935323383394, 0.6529850746268657247, 0.6542288557213929989, 0.6554726368159203842, 0.6567164179104477695, 0.6579601990049751548, 0.6592039800995025400, 0.6604477611940298143, 0.6616915422885571996, 0.6629353233830845848, 0.6641791044776119701, 0.6654228855721393554, 0.6666666666666666297, 0.6679104477611940149, 0.6691542288557214002, 0.6703980099502487855, 0.6716417910447761708, 0.6728855721393034450, 0.6741293532338308303, 0.6753731343283582156, 0.6766169154228856009, 0.6778606965174129861, 0.6791044776119402604, 0.6803482587064676457, 0.6815920398009950310, 0.6828358208955224162, 0.6840796019900498015, 0.6853233830845770758, 0.6865671641791044610, 0.6878109452736318463, 0.6890547263681592316, 0.6902985074626866169, 0.6915422885572138911, 0.6927860696517412764, 0.6940298507462686617, 0.6952736318407960470, 0.6965174129353234322, 0.6977611940298507065, 0.6990049751243780918, 0.7002487562189054771, 0.7014925373134328623, 0.7027363184079602476, 0.7039800995024875219, 0.7052238805970149071, 0.7064676616915422924, 0.7077114427860696777, 0.7089552238805970630, 0.7101990049751243372, 0.7114427860696517225, 0.7126865671641791078, 0.7139303482587064931, 0.7151741293532338783, 0.7164179104477611526, 0.7176616915422885379, 0.7189054726368159232, 0.7201492537313433084, 0.7213930348258706937, 0.7226368159203979680, 0.7238805970149253532, 0.7251243781094527385, 0.7263681592039801238, 0.7276119402985075091, 0.7288557213930347833, 0.7300995024875621686, 0.7313432835820895539, 0.7325870646766169392, 0.7338308457711443245, 0.7350746268656715987, 0.7363184079601989840, 0.7375621890547263693, 0.7388059701492537545, 0.7400497512437811398, 0.7412935323383084141, 0.7425373134328357994, 0.7437810945273631846, 0.7450248756218905699, 0.7462686567164179552, 0.7475124378109452294, 0.7487562189054726147, 0.7500000000000000000, 0.7512437810945273853, 0.7524875621890547706, 0.7537313432835820448, 0.7549751243781094301, 0.7562189054726368154, 0.7574626865671642006, 0.7587064676616915859, 0.7599502487562188602, 0.7611940298507462455, 0.7624378109452736307, 0.7636815920398010160, 0.7649253731343284013, 0.7661691542288556755, 0.7674129353233830608, 0.7686567164179104461, 0.7699004975124378314, 0.7711442786069652167, 0.7723880597014924909, 0.7736318407960198762, 0.7748756218905472615, 0.7761194029850746468, 0.7773631840796020320, 0.7786069651741293063, 0.7798507462686566916, 0.7810945273631840768, 0.7823383084577114621, 0.7835820895522388474, 0.7848258706467661217, 0.7860696517412935069, 0.7873134328358208922, 0.7885572139303482775, 0.7898009950248756628, 0.7910447761194029370, 0.7922885572139303223, 0.7935323383084577076, 0.7947761194029850929, 0.7960199004975124781, 0.7972636815920397524, 0.7985074626865671377, 0.7997512437810945229, 0.8009950248756219082, 0.8022388059701492935, 0.8034825870646765678, 0.8047263681592039530, 0.8059701492537313383, 0.8072139303482587236, 0.8084577114427861089, 0.8097014925373133831, 0.8109452736318407684, 0.8121890547263681537, 0.8134328358208955390, 0.8146766169154229242, 0.8159203980099501985, 0.8171641791044775838, 0.8184079601990049690, 0.8196517412935323543, 0.8208955223880597396, 0.8221393034825870139, 0.8233830845771143991, 0.8246268656716417844, 0.8258706467661691697, 0.8271144278606965550, 0.8283582089552238292, 0.8296019900497512145, 0.8308457711442785998, 0.8320895522388059851, 0.8333333333333333703, 0.8345771144278606446, 0.8358208955223880299, 0.8370646766169154152, 0.8383084577114428004, 0.8395522388059701857, 0.8407960199004974600, 0.8420398009950248452, 0.8432835820895522305, 0.8445273631840796158, 0.8457711442786070011, 0.8470149253731342753, 0.8482587064676616606, 0.8495024875621890459, 0.8507462686567164312, 0.8519900497512438164, 0.8532338308457710907, 0.8544776119402984760, 0.8557213930348258613, 0.8569651741293532465, 0.8582089552238806318, 0.8594527363184079061, 0.8606965174129352913, 0.8619402985074626766, 0.8631840796019900619, 0.8644278606965174472, 0.8656716417910447214, 0.8669154228855721067, 0.8681592039800994920, 0.8694029850746268773, 0.8706467661691542625, 0.8718905472636815368, 0.8731343283582089221, 0.8743781094527363074, 0.8756218905472636926, 0.8768656716417910779, 0.8781094527363184632, 0.8793532338308457375, 0.8805970149253731227, 0.8818407960199005080, 0.8830845771144278933, 0.8843283582089552786, 0.8855721393034825528, 0.8868159203980099381, 0.8880597014925373234, 0.8893034825870647087, 0.8905472636815920939, 0.8917910447761193682, 0.8930348258706467535, 0.8942786069651741387, 0.8955223880597015240, 0.8967661691542289093, 0.8980099502487561836, 0.8992537313432835688, 0.9004975124378109541, 0.9017412935323383394, 0.9029850746268657247, 0.9042288557213929989, 0.9054726368159203842, 0.9067164179104477695, 0.9079601990049751548, 0.9092039800995025400, 0.9104477611940298143, 0.9116915422885571996, 0.9129353233830845848, 0.9141791044776119701, 0.9154228855721393554, 0.9166666666666666297, 0.9179104477611940149, 0.9191542288557214002, 0.9203980099502487855, 0.9216417910447761708, 0.9228855721393034450, 0.9241293532338308303, 0.9253731343283582156, 0.9266169154228856009, 0.9278606965174129861, 0.9291044776119402604, 0.9303482587064676457, 0.9315920398009950310, 0.9328358208955224162, 0.9340796019900498015, 0.9353233830845770758, 0.9365671641791044610, 0.9378109452736318463, 0.9390547263681592316, 0.9402985074626866169, 0.9415422885572138911, 0.9427860696517412764, 0.9440298507462686617, 0.9452736318407960470, 0.9465174129353234322, 0.9477611940298507065, 0.9490049751243780918, 0.9502487562189054771, 0.9514925373134328623, 0.9527363184079602476, 0.9539800995024875219, 0.9552238805970149071, 0.9564676616915422924, 0.9577114427860696777, 0.9589552238805970630, 0.9601990049751243372, 0.9614427860696517225, 0.9626865671641791078, 0.9639303482587064931, 0.9651741293532338783, 0.9664179104477611526, 0.9676616915422885379, 0.9689054726368159232, 0.9701492537313433084, 0.9713930348258706937, 0.9726368159203979680, 0.9738805970149253532, 0.9751243781094527385, 0.9763681592039801238, 0.9776119402985075091, 0.9788557213930347833, 0.9800995024875621686, 0.9813432835820895539, 0.9825870646766169392, 0.9838308457711443245, 0.9850746268656715987, 0.9863184079601989840, 0.9875621890547263693, 0.9888059701492537545, 0.9900497512437811398, 0.9912935323383084141, 0.9925373134328357994, 0.9937810945273631846, 0.9950248756218905699 ),
 .UNSPECIFIED. ) 
 GEOMETRIC_REPRESENTATION_ITEM ( )  RATIONAL_B_SPLINE_SURFACE ( (
 ( 1.000000000000000000, 0.8660254037844387076, 1.000000000000000000, 0.8660254037844387076, 1.000000000000000000, 0.8660254037844387076, 1.000000000000000000, 0.8660254037844387076, 1.000000000000000000, 0.8660254037844387076, 1.000000000000000000, 0.8660254037844387076, 1.000000000000000000, 0.8660254037844387076, 1.000000000000000000, 0.8660254037844387076, 1.000000000000000000, 0.8660254037844387076, 1.000000000000000000, 0.8660254037844387076, 1.000000000000000000, 0.8660254037844387076, 1.000000000000000000, 0.8660254037844387076, 1.000000000000000000, 0.8660254037844387076, 1.000000000000000000, 0.8660254037844387076, 1.000000000000000000, 0.8660254037844387076, 1.000000000000000000, 0.8660254037844387076, 1.000000000000000000, 0.8660254037844387076, 1.000000000000000000, 0.8660254037844387076, 1.000000000000000000, 0.8660254037844387076, 1.000000000000000000, 0.8660254037844387076, 1.000000000000000000, 0.8660254037844387076, 1.000000000000000000, 0.8660254037844387076, 1.000000000000000000, 0.8660254037844387076, 1.000000000000000000, 0.8660254037844387076, 1.000000000000000000, 0.8660254037844387076, 1.000000000000000000, 0.8660254037844387076, 1.000000000000000000, 0.8660254037844387076, 1.000000000000000000, 0.8660254037844387076, 1.000000000000000000, 0.8660254037844387076, 1.000000000000000000, 0.8660254037844387076, 1.000000000000000000, 0.8660254037844387076, 1.000000000000000000, 0.8660254037844387076, 1.000000000000000000, 0.8660254037844387076, 1.000000000000000000, 0.8660254037844387076, 1.000000000000000000, 0.8660254037844387076, 1.000000000000000000, 0.8660254037844387076, 1.000000000000000000, 0.8660254037844387076, 1.000000000000000000, 0.8660254037844387076, 1.000000000000000000, 0.8660254037844387076, 1.000000000000000000, 0.8660254037844387076, 1.000000000000000000, 0.8660254037844387076, 1.000000000000000000, 0.8660254037844387076, 1.000000000000000000, 0.8660254037844387076, 1.000000000000000000, 0.8660254037844387076, 1.000000000000000000, 0.8660254037844387076, 1.000000000000000000, 0.8660254037844387076, 1.000000000000000000, 0.8660254037844387076, 1.000000000000000000, 0.8660254037844387076, 1.000000000000000000, 0.8660254037844387076, 1.000000000000000000, 0.8660254037844387076, 1.000000000000000000, 0.8660254037844387076, 1.000000000000000000, 0.8660254037844387076, 1.000000000000000000, 0.8660254037844387076, 1.000000000000000000, 0.8660254037844387076, 1.000000000000000000, 0.8660254037844387076, 1.000000000000000000, 0.8660254037844387076, 1.000000000000000000, 0.8660254037844387076, 1.000000000000000000, 0.8660254037844387076, 1.000000000000000000, 0.8660254037844387076, 1.000000000000000000, 0.8660254037844387076, 1.000000000000000000, 0.8660254037844387076, 1.000000000000000000, 0.8660254037844387076, 1.000000000000000000, 0.8660254037844387076, 1.000000000000000000, 0.8660254037844387076, 1.000000000000000000, 0.8660254037844387076, 1.000000000000000000, 0.8660254037844387076, 1.000000000000000000, 0.8660254037844387076, 1.000000000000000000, 0.8660254037844387076, 1.000000000000000000, 0.8660254037844387076, 1.000000000000000000, 0.8660254037844387076, 1.000000000000000000, 0.8660254037844387076, 1.000000000000000000, 0.8660254037844387076, 1.000000000000000000, 0.8660254037844387076, 1.000000000000000000, 0.8660254037844387076, 1.000000000000000000, 0.8660254037844387076, 1.000000000000000000, 0.8660254037844387076, 1.000000000000000000, 0.8660254037844387076, 1.000000000000000000, 0.8660254037844387076, 1.000000000000000000, 0.8660254037844387076, 1.000000000000000000, 0.8660254037844387076, 1.000000000000000000, 0.8660254037844387076, 1.000000000000000000, 0.8660254037844387076, 1.000000000000000000, 0.8660254037844387076, 1.000000000000000000, 0.8660254037844387076, 1.000000000000000000, 0.8660254037844387076, 1.000000000000000000, 0.8660254037844387076, 1.000000000000000000, 0.8660254037844387076, 1.000000000000000000, 0.8660254037844387076, 1.000000000000000000, 0.8660254037844387076, 1.000000000000000000, 0.8660254037844387076, 1.000000000000000000, 0.8660254037844387076, 1.000000000000000000, 0.8660254037844387076, 1.000000000000000000, 0.8660254037844387076, 1.000000000000000000, 0.8660254037844387076, 1.000000000000000000, 0.8660254037844387076, 1.000000000000000000, 0.8660254037844387076, 1.000000000000000000, 0.8660254037844387076, 1.000000000000000000, 0.8660254037844387076, 1.000000000000000000, 0.8660254037844387076, 1.000000000000000000, 0.8660254037844387076, 1.000000000000000000, 0.8660254037844387076, 1.000000000000000000, 0.8660254037844387076, 1.000000000000000000, 0.8660254037844387076, 1.000000000000000000, 0.8660254037844387076, 1.000000000000000000, 0.8660254037844387076, 1.000000000000000000, 0.8660254037844387076, 1.000000000000000000, 0.8660254037844387076, 1.000000000000000000, 0.8660254037844387076, 1.000000000000000000, 0.8660254037844387076, 1.000000000000000000, 0.8660254037844387076, 1.000000000000000000, 0.8660254037844387076, 1.000000000000000000, 0.8660254037844387076, 1.000000000000000000, 0.8660254037844387076, 1.000000000000000000, 0.8660254037844387076, 1.000000000000000000, 0.8660254037844387076, 1.000000000000000000, 0.8660254037844387076, 1.000000000000000000, 0.8660254037844387076, 1.000000000000000000, 0.8660254037844387076, 1.000000000000000000, 0.8660254037844387076, 1.000000000000000000, 0.8660254037844387076, 1.000000000000000000, 0.8660254037844387076, 1.000000000000000000, 0.8660254037844387076, 1.000000000000000000, 0.8660254037844387076, 1.000000000000000000, 0.8660254037844387076, 1.000000000000000000, 0.8660254037844387076, 1.000000000000000000, 0.8660254037844387076, 1.000000000000000000, 0.8660254037844387076, 1.000000000000000000, 0.8660254037844387076, 1.000000000000000000, 0.8660254037844387076, 1.000000000000000000, 0.8660254037844387076, 1.000000000000000000, 0.8660254037844387076, 1.000000000000000000, 0.8660254037844387076, 1.000000000000000000, 0.8660254037844387076, 1.000000000000000000, 0.8660254037844387076, 1.000000000000000000, 0.8660254037844387076, 1.000000000000000000, 0.8660254037844387076, 1.000000000000000000, 0.8660254037844387076, 1.000000000000000000, 0.8660254037844387076, 1.000000000000000000, 0.8660254037844387076, 1.000000000000000000, 0.8660254037844387076, 1.000000000000000000, 0.8660254037844387076, 1.000000000000000000, 0.8660254037844387076, 1.000000000000000000, 0.8660254037844387076, 1.000000000000000000, 0.8660254037844387076, 1.000000000000000000, 0.8660254037844387076, 1.000000000000000000, 0.8660254037844387076, 1.000000000000000000, 0.8660254037844387076, 1.000000000000000000, 0.8660254037844387076, 1.000000000000000000, 0.8660254037844387076, 1.000000000000000000, 0.8660254037844387076, 1.000000000000000000, 0.8660254037844387076, 1.000000000000000000, 0.8660254037844387076, 1.000000000000000000, 0.8660254037844387076, 1.000000000000000000, 0.8660254037844387076, 1.000000000000000000, 0.8660254037844387076, 1.000000000000000000, 0.8660254037844387076, 1.000000000000000000, 0.8660254037844387076, 1.000000000000000000, 0.8660254037844387076, 1.000000000000000000, 0.8660254037844387076, 1.000000000000000000, 0.8660254037844387076, 1.000000000000000000, 0.8660254037844387076, 1.000000000000000000, 0.8660254037844387076, 1.000000000000000000, 0.8660254037844387076, 1.000000000000000000, 0.8660254037844387076, 1.000000000000000000, 0.8660254037844387076, 1.000000000000000000, 0.8660254037844387076, 1.000000000000000000, 0.8660254037844387076, 1.000000000000000000, 0.8660254037844387076, 1.000000000000000000, 0.8660254037844387076, 1.000000000000000000, 0.8660254037844387076, 1.000000000000000000, 0.8660254037844387076, 1.000000000000000000, 0.8660254037844387076, 1.000000000000000000, 0.8660254037844387076, 1.000000000000000000, 0.8660254037844387076, 1.000000000000000000, 0.8660254037844387076, 1.000000000000000000, 0.8660254037844387076, 1.000000000000000000, 0.8660254037844387076, 1.000000000000000000, 0.8660254037844387076, 1.000000000000000000, 0.8660254037844387076, 1.000000000000000000, 0.8660254037844387076, 1.000000000000000000, 0.8660254037844387076, 1.000000000000000000, 0.8660254037844387076, 1.000000000000000000, 0.8660254037844387076, 1.000000000000000000, 0.8660254037844387076, 1.000000000000000000, 0.8660254037844387076, 1.000000000000000000, 0.8660254037844387076, 1.000000000000000000, 0.8660254037844387076, 1.000000000000000000, 0.8660254037844387076, 1.000000000000000000, 0.8660254037844387076, 1.000000000000000000, 0.8660254037844387076, 1.000000000000000000, 0.8660254037844387076, 1.000000000000000000, 0.8660254037844387076, 1.000000000000000000, 0.8660254037844387076, 1.000000000000000000, 0.8660254037844387076, 1.000000000000000000, 0.8660254037844387076, 1.000000000000000000, 0.8660254037844387076, 1.000000000000000000, 0.8660254037844387076, 1.000000000000000000, 0.8660254037844387076, 1.000000000000000000, 0.8660254037844387076, 1.000000000000000000, 0.8660254037844387076, 1.000000000000000000, 0.8660254037844387076, 1.000000000000000000, 0.8660254037844387076, 1.000000000000000000, 0.8660254037844387076, 1.000000000000000000, 0.8660254037844387076, 1.000000000000000000, 0.8660254037844387076, 1.000000000000000000, 0.8660254037844387076, 1.000000000000000000, 0.8660254037844387076, 1.000000000000000000, 0.8660254037844387076, 1.000000000000000000, 0.8660254037844387076, 1.000000000000000000, 0.8660254037844387076, 1.000000000000000000, 0.8660254037844387076, 1.000000000000000000, 0.8660254037844387076, 1.000000000000000000, 0.8660254037844387076, 1.000000000000000000, 0.8660254037844387076, 1.000000000000000000, 0.8660254037844387076, 1.000000000000000000, 0.8660254037844387076, 1.000000000000000000, 0.8660254037844387076, 1.000000000000000000, 0.8660254037844387076, 1.000000000000000000, 0.8660254037844387076, 1.000000000000000000, 0.8660254037844387076, 1.000000000000000000, 0.8660254037844387076, 1.000000000000000000, 0.8660254037844387076, 1.000000000000000000, 0.8660254037844387076, 1.000000000000000000, 0.8660254037844387076, 1.000000000000000000, 0.8660254037844387076, 1.000000000000000000, 0.8660254037844387076, 1.000000000000000000, 0.8660254037844387076, 1.000000000000000000, 0.8660254037844387076, 1.000000000000000000, 0.8660254037844387076, 1.000000000000000000, 0.8660254037844387076, 1.000000000000000000, 0.8660254037844387076, 1.000000000000000000, 0.8660254037844387076, 1.000000000000000000, 0.8660254037844387076, 1.000000000000000000, 0.8660254037844387076, 1.000000000000000000, 0.8660254037844387076, 1.000000000000000000, 0.8660254037844387076, 1.000000000000000000, 0.8660254037844387076, 1.000000000000000000, 0.8660254037844387076, 1.000000000000000000, 0.8660254037844387076, 1.000000000000000000, 0.8660254037844387076, 1.000000000000000000, 0.8660254037844387076, 1.000000000000000000, 0.8660254037844387076, 1.000000000000000000, 0.8660254037844387076, 1.000000000000000000, 0.8660254037844387076, 1.000000000000000000, 0.8660254037844387076, 1.000000000000000000, 0.8660254037844387076, 1.000000000000000000, 0.8660254037844387076, 1.000000000000000000, 0.8660254037844387076, 1.000000000000000000, 0.8660254037844387076, 1.000000000000000000, 0.8660254037844387076, 1.000000000000000000, 0.8660254037844387076, 1.000000000000000000, 0.8660254037844387076, 1.000000000000000000, 0.8660254037844387076, 1.000000000000000000, 0.8660254037844387076, 1.000000000000000000, 0.8660254037844387076, 1.000000000000000000, 0.8660254037844387076, 1.000000000000000000, 0.8660254037844387076, 1.000000000000000000, 0.8660254037844387076, 1.000000000000000000, 0.8660254037844387076, 1.000000000000000000, 0.8660254037844387076, 1.000000000000000000, 0.8660254037844387076, 1.000000000000000000, 0.8660254037844387076, 1.000000000000000000, 0.8660254037844387076, 1.000000000000000000, 0.8660254037844387076, 1.000000000000000000, 0.8660254037844387076, 1.000000000000000000, 0.8660254037844387076, 1.000000000000000000, 0.8660254037844387076, 1.000000000000000000, 0.8660254037844387076, 1.000000000000000000, 0.8660254037844387076, 1.000000000000000000, 0.8660254037844387076, 1.000000000000000000, 0.8660254037844387076, 1.000000000000000000, 0.8660254037844387076, 1.000000000000000000, 0.8660254037844387076, 1.000000000000000000, 0.8660254037844387076, 1.000000000000000000, 0.8660254037844387076, 1.000000000000000000, 0.8660254037844387076, 1.000000000000000000, 0.8660254037844387076, 1.000000000000000000, 0.8660254037844387076, 1.000000000000000000, 0.8660254037844387076, 1.000000000000000000, 0.8660254037844387076, 1.000000000000000000, 0.8660254037844387076, 1.000000000000000000, 0.8660254037844387076, 1.000000000000000000, 0.8660254037844387076, 1.000000000000000000, 0.8660254037844387076, 1.000000000000000000, 0.8660254037844387076, 1.000000000000000000, 0.8660254037844387076, 1.000000000000000000, 0.8660254037844387076, 1.000000000000000000, 0.8660254037844387076, 1.000000000000000000, 0.8660254037844387076, 1.000000000000000000, 0.8660254037844387076, 1.000000000000000000, 0.8660254037844387076, 1.000000000000000000, 0.8660254037844387076, 1.000000000000000000, 0.8660254037844387076, 1.000000000000000000, 0.8660254037844387076, 1.000000000000000000, 0.8660254037844387076, 1.000000000000000000, 0.8660254037844387076, 1.000000000000000000, 0.8660254037844387076, 1.000000000000000000, 0.8660254037844387076, 1.000000000000000000, 0.8660254037844387076, 1.000000000000000000, 0.8660254037844387076, 1.000000000000000000, 0.8660254037844387076, 1.000000000000000000, 0.8660254037844387076, 1.000000000000000000, 0.8660254037844387076, 1.000000000000000000, 0.8660254037844387076, 1.000000000000000000, 0.8660254037844387076, 1.000000000000000000, 0.8660254037844387076, 1.000000000000000000, 0.8660254037844387076, 1.000000000000000000, 0.8660254037844387076, 1.000000000000000000, 0.8660254037844387076, 1.000000000000000000, 0.8660254037844387076, 1.000000000000000000, 0.8660254037844387076, 1.000000000000000000, 0.8660254037844387076, 1.000000000000000000, 0.8660254037844387076, 1.000000000000000000, 0.8660254037844387076, 1.000000000000000000, 0.8660254037844387076, 1.000000000000000000, 0.8660254037844387076, 1.000000000000000000, 0.8660254037844387076, 1.000000000000000000, 0.8660254037844387076, 1.000000000000000000, 0.8660254037844387076, 1.000000000000000000, 0.8660254037844387076, 1.000000000000000000, 0.8660254037844387076, 1.000000000000000000, 0.8660254037844387076, 1.000000000000000000, 0.8660254037844387076, 1.000000000000000000, 0.8660254037844387076, 1.000000000000000000, 0.8660254037844387076, 1.000000000000000000, 0.8660254037844387076, 1.000000000000000000, 0.8660254037844387076, 1.000000000000000000, 0.8660254037844387076, 1.000000000000000000, 0.8660254037844387076, 1.000000000000000000, 0.8660254037844387076, 1.000000000000000000, 0.8660254037844387076, 1.000000000000000000, 0.8660254037844387076, 1.000000000000000000, 0.8660254037844387076, 1.000000000000000000, 0.8660254037844387076, 1.000000000000000000, 0.8660254037844387076, 1.000000000000000000, 0.8660254037844387076, 1.000000000000000000, 0.8660254037844387076, 1.000000000000000000, 0.8660254037844387076, 1.000000000000000000, 0.8660254037844387076, 1.000000000000000000, 0.8660254037844387076, 1.000000000000000000, 0.8660254037844387076, 1.000000000000000000, 0.8660254037844387076, 1.000000000000000000, 0.8660254037844387076, 1.000000000000000000, 0.8660254037844387076, 1.000000000000000000, 0.8660254037844387076, 1.000000000000000000, 0.8660254037844387076, 1.000000000000000000, 0.8660254037844387076, 1.000000000000000000, 0.8660254037844387076, 1.000000000000000000, 0.8660254037844387076, 1.000000000000000000, 0.8660254037844387076, 1.000000000000000000, 0.8660254037844387076, 1.000000000000000000, 0.8660254037844387076, 1.000000000000000000, 0.8660254037844387076, 1.000000000000000000, 0.8660254037844387076, 1.000000000000000000, 0.8660254037844387076, 1.000000000000000000, 0.8660254037844387076, 1.000000000000000000, 0.8660254037844387076, 1.000000000000000000, 0.8660254037844387076, 1.000000000000000000, 0.8660254037844387076, 1.000000000000000000, 0.8660254037844387076, 1.000000000000000000, 0.8660254037844387076, 1.000000000000000000, 0.8660254037844387076, 1.000000000000000000, 0.8660254037844387076, 1.000000000000000000, 0.8660254037844387076, 1.000000000000000000, 0.8660254037844387076, 1.000000000000000000, 0.8660254037844387076, 1.000000000000000000, 0.8660254037844387076, 1.000000000000000000, 0.8660254037844387076, 1.000000000000000000, 0.8660254037844387076, 1.000000000000000000, 0.8660254037844387076, 1.000000000000000000, 0.8660254037844387076, 1.000000000000000000, 0.8660254037844387076, 1.000000000000000000, 0.8660254037844387076, 1.000000000000000000, 0.8660254037844387076, 1.000000000000000000, 0.8660254037844387076, 1.000000000000000000, 0.8660254037844387076, 1.000000000000000000, 0.8660254037844387076, 1.000000000000000000, 0.8660254037844387076, 1.000000000000000000, 0.8660254037844387076, 1.000000000000000000, 0.8660254037844387076, 1.000000000000000000, 0.8660254037844387076, 1.000000000000000000, 0.8660254037844387076, 1.000000000000000000, 0.8660254037844387076, 1.000000000000000000, 0.8660254037844387076, 1.000000000000000000, 0.8660254037844387076, 1.000000000000000000, 0.8660254037844387076, 1.000000000000000000, 0.8660254037844387076, 1.000000000000000000, 0.8660254037844387076, 1.000000000000000000, 0.8660254037844387076, 1.000000000000000000, 0.8660254037844387076, 1.000000000000000000, 0.8660254037844387076, 1.000000000000000000, 0.8660254037844387076, 1.000000000000000000, 0.8660254037844387076, 1.000000000000000000, 0.8660254037844387076, 1.000000000000000000, 0.8660254037844387076, 1.000000000000000000, 0.8660254037844387076, 1.000000000000000000, 0.8660254037844387076, 1.000000000000000000, 0.8660254037844387076, 1.000000000000000000, 0.8660254037844387076, 1.000000000000000000, 0.8660254037844387076, 1.000000000000000000, 0.8660254037844387076, 1.000000000000000000, 0.8660254037844387076, 1.000000000000000000, 0.8660254037844387076, 1.000000000000000000, 0.8660254037844387076, 1.000000000000000000, 0.8660254037844387076, 1.000000000000000000, 0.8660254037844387076, 1.000000000000000000, 0.8660254037844387076, 1.000000000000000000, 0.8660254037844387076, 1.000000000000000000, 0.8660254037844387076, 1.000000000000000000, 0.8660254037844387076, 1.000000000000000000, 0.8660254037844387076, 1.000000000000000000, 0.8660254037844387076, 1.000000000000000000, 0.8660254037844387076, 1.000000000000000000, 0.8660254037844387076, 1.000000000000000000, 0.8660254037844387076, 1.000000000000000000, 0.8660254037844387076, 1.000000000000000000, 0.8660254037844387076, 1.000000000000000000, 0.8660254037844387076, 1.000000000000000000, 0.8660254037844387076, 1.000000000000000000, 0.8660254037844387076, 1.000000000000000000, 0.8660254037844387076, 1.000000000000000000, 0.8660254037844387076, 1.000000000000000000, 0.8660254037844387076, 1.000000000000000000, 0.8660254037844387076, 1.000000000000000000, 0.8660254037844387076, 1.000000000000000000, 0.8660254037844387076, 1.000000000000000000, 0.8660254037844387076, 1.000000000000000000, 0.8660254037844387076, 1.000000000000000000, 0.8660254037844387076, 1.000000000000000000, 0.8660254037844387076, 1.000000000000000000, 0.8660254037844387076, 1.000000000000000000, 0.8660254037844387076, 1.000000000000000000, 0.8660254037844387076, 1.000000000000000000, 0.8660254037844387076, 1.000000000000000000, 0.8660254037844387076, 1.000000000000000000, 0.8660254037844387076, 1.000000000000000000, 0.8660254037844387076, 1.000000000000000000, 0.8660254037844387076, 1.000000000000000000, 0.8660254037844387076, 1.000000000000000000, 0.8660254037844387076, 1.000000000000000000, 0.8660254037844387076, 1.000000000000000000, 0.8660254037844387076, 1.000000000000000000, 0.8660254037844387076, 1.000000000000000000, 0.8660254037844387076, 1.000000000000000000, 0.8660254037844387076, 1.000000000000000000, 0.8660254037844387076, 1.000000000000000000, 0.8660254037844387076, 1.000000000000000000, 0.8660254037844387076, 1.000000000000000000, 0.8660254037844387076, 1.000000000000000000, 0.8660254037844387076, 1.000000000000000000, 0.8660254037844387076, 1.000000000000000000, 0.8660254037844387076, 1.000000000000000000, 0.8660254037844387076, 1.000000000000000000, 0.8660254037844387076, 1.000000000000000000, 0.8660254037844387076, 1.000000000000000000, 0.8660254037844387076, 1.000000000000000000, 0.8660254037844387076, 1.000000000000000000, 0.8660254037844387076, 1.000000000000000000, 0.8660254037844387076, 1.000000000000000000, 0.8660254037844387076, 1.000000000000000000, 0.8660254037844387076, 1.000000000000000000, 0.8660254037844387076, 1.000000000000000000, 0.8660254037844387076, 1.000000000000000000, 0.8660254037844387076, 1.000000000000000000, 0.8660254037844387076, 1.000000000000000000, 0.8660254037844387076, 1.000000000000000000, 0.8660254037844387076, 1.000000000000000000, 0.8660254037844387076, 1.000000000000000000, 0.8660254037844387076, 1.000000000000000000, 0.8660254037844387076, 1.000000000000000000, 0.8660254037844387076, 1.000000000000000000, 0.8660254037844387076, 1.000000000000000000, 0.8660254037844387076, 1.000000000000000000, 0.8660254037844387076, 1.000000000000000000, 0.8660254037844387076, 1.000000000000000000, 0.8660254037844387076, 1.000000000000000000, 0.8660254037844387076, 1.000000000000000000, 0.8660254037844387076, 1.000000000000000000, 0.8660254037844387076, 1.000000000000000000, 0.8660254037844387076, 1.000000000000000000, 0.8660254037844387076, 1.000000000000000000, 0.8660254037844387076, 1.000000000000000000, 0.8660254037844387076, 1.000000000000000000, 0.8660254037844387076, 1.000000000000000000, 0.8660254037844387076, 1.000000000000000000, 0.8660254037844387076, 1.000000000000000000, 0.8660254037844387076, 1.000000000000000000, 0.8660254037844387076, 1.000000000000000000, 0.8660254037844387076, 1.000000000000000000, 0.8660254037844387076, 1.000000000000000000, 0.8660254037844387076, 1.000000000000000000, 0.8660254037844387076, 1.000000000000000000, 0.8660254037844387076, 1.000000000000000000, 0.8660254037844387076, 1.000000000000000000, 0.8660254037844387076, 1.000000000000000000, 0.8660254037844387076, 1.000000000000000000, 0.8660254037844387076, 1.000000000000000000, 0.8660254037844387076, 1.000000000000000000, 0.8660254037844387076, 1.000000000000000000, 0.8660254037844387076, 1.000000000000000000, 0.8660254037844387076, 1.000000000000000000, 0.8660254037844387076, 1.000000000000000000, 0.8660254037844387076, 1.000000000000000000, 0.8660254037844387076, 1.000000000000000000, 0.8660254037844387076, 1.000000000000000000, 0.8660254037844387076, 1.000000000000000000, 0.8660254037844387076, 1.000000000000000000, 0.8660254037844387076, 1.000000000000000000, 0.8660254037844387076, 1.000000000000000000, 0.8660254037844387076, 1.000000000000000000, 0.8660254037844387076, 1.000000000000000000, 0.8660254037844387076, 1.000000000000000000, 0.8660254037844387076, 1.000000000000000000, 0.8660254037844387076, 1.000000000000000000, 0.8660254037844387076, 1.000000000000000000, 0.8660254037844387076, 1.000000000000000000, 0.8660254037844387076, 1.000000000000000000, 0.8660254037844387076, 1.000000000000000000, 0.8660254037844387076, 1.000000000000000000, 0.8660254037844387076, 1.000000000000000000, 0.8660254037844387076, 1.000000000000000000, 0.8660254037844387076, 1.000000000000000000, 0.8660254037844387076, 1.000000000000000000, 0.8660254037844387076, 1.000000000000000000, 0.8660254037844387076, 1.000000000000000000, 0.8660254037844387076, 1.000000000000000000, 0.8660254037844387076, 1.000000000000000000, 0.8660254037844387076, 1.000000000000000000, 0.8660254037844387076, 1.000000000000000000, 0.8660254037844387076, 1.000000000000000000, 0.8660254037844387076, 1.000000000000000000, 0.8660254037844387076, 1.000000000000000000, 0.8660254037844387076, 1.000000000000000000, 0.8660254037844387076, 1.000000000000000000, 0.8660254037844387076, 1.000000000000000000, 0.8660254037844387076, 1.000000000000000000, 0.8660254037844387076, 1.000000000000000000, 0.8660254037844387076, 1.000000000000000000, 0.8660254037844387076, 1.000000000000000000, 0.8660254037844387076, 1.000000000000000000, 0.8660254037844387076, 1.000000000000000000, 0.8660254037844387076, 1.000000000000000000, 0.8660254037844387076, 1.000000000000000000, 0.8660254037844387076, 1.000000000000000000, 0.8660254037844387076, 1.000000000000000000, 0.8660254037844387076, 1.000000000000000000, 0.8660254037844387076, 1.000000000000000000, 0.8660254037844387076, 1.000000000000000000, 0.8660254037844387076, 1.000000000000000000, 0.8660254037844387076, 1.000000000000000000, 0.8660254037844387076, 1.000000000000000000, 0.8660254037844387076, 1.000000000000000000, 0.8660254037844387076, 1.000000000000000000, 0.8660254037844387076, 1.000000000000000000, 0.8660254037844387076, 1.000000000000000000, 0.8660254037844387076, 1.000000000000000000, 0.8660254037844387076, 1.000000000000000000, 0.8660254037844387076, 1.000000000000000000, 0.8660254037844387076, 1.000000000000000000, 0.8660254037844387076, 1.000000000000000000, 0.8660254037844387076, 1.000000000000000000, 0.8660254037844387076, 1.000000000000000000, 0.8660254037844387076, 1.000000000000000000, 0.8660254037844387076, 1.000000000000000000, 0.8660254037844387076, 1.000000000000000000, 0.8660254037844387076, 1.000000000000000000, 0.8660254037844387076, 1.000000000000000000, 0.8660254037844387076, 1.000000000000000000, 0.8660254037844387076, 1.000000000000000000, 0.8660254037844387076, 1.000000000000000000, 0.8660254037844387076, 1.000000000000000000, 0.8660254037844387076, 1.000000000000000000, 0.8660254037844387076, 1.000000000000000000, 0.8660254037844387076, 1.000000000000000000, 0.8660254037844387076, 1.000000000000000000, 0.8660254037844387076, 1.000000000000000000, 0.8660254037844387076, 1.000000000000000000, 0.8660254037844387076, 1.000000000000000000, 0.8660254037844387076, 1.000000000000000000, 0.8660254037844387076, 1.000000000000000000, 0.8660254037844387076, 1.000000000000000000, 0.8660254037844387076, 1.000000000000000000, 0.8660254037844387076, 1.000000000000000000, 0.8660254037844387076, 1.000000000000000000, 0.8660254037844387076, 1.000000000000000000, 0.8660254037844387076, 1.000000000000000000, 0.8660254037844387076, 1.000000000000000000, 0.8660254037844387076, 1.000000000000000000, 0.8660254037844387076, 1.000000000000000000, 0.8660254037844387076, 1.000000000000000000, 0.8660254037844387076, 1.000000000000000000, 0.8660254037844387076, 1.000000000000000000, 0.8660254037844387076, 1.000000000000000000, 0.8660254037844387076, 1.000000000000000000, 0.8660254037844387076, 1.000000000000000000, 0.8660254037844387076, 1.000000000000000000, 0.8660254037844387076, 1.000000000000000000, 0.8660254037844387076, 1.000000000000000000, 0.8660254037844387076, 1.000000000000000000, 0.8660254037844387076, 1.000000000000000000, 0.8660254037844387076, 1.000000000000000000, 0.8660254037844387076, 1.000000000000000000, 0.8660254037844387076, 1.000000000000000000, 0.8660254037844387076, 1.000000000000000000, 0.8660254037844387076, 1.000000000000000000, 0.8660254037844387076, 1.000000000000000000, 0.8660254037844387076, 1.000000000000000000, 0.8660254037844387076, 1.000000000000000000, 0.8660254037844387076, 1.000000000000000000, 0.8660254037844387076, 1.000000000000000000, 0.8660254037844387076, 1.000000000000000000, 0.8660254037844387076, 1.000000000000000000, 0.8660254037844387076, 1.000000000000000000, 0.8660254037844387076, 1.000000000000000000, 0.8660254037844387076, 1.000000000000000000, 0.8660254037844387076, 1.000000000000000000, 0.8660254037844387076, 1.000000000000000000, 0.8660254037844387076, 1.000000000000000000, 0.8660254037844387076, 1.000000000000000000, 0.8660254037844387076, 1.000000000000000000, 0.8660254037844387076, 1.000000000000000000, 0.8660254037844387076, 1.000000000000000000, 0.8660254037844387076, 1.000000000000000000, 0.8660254037844387076, 1.000000000000000000, 0.8660254037844387076, 1.000000000000000000, 0.8660254037844387076, 1.000000000000000000, 0.8660254037844387076, 1.000000000000000000, 0.8660254037844387076, 1.000000000000000000, 0.8660254037844387076, 1.000000000000000000, 0.8660254037844387076, 1.000000000000000000, 0.8660254037844387076, 1.000000000000000000, 0.8660254037844387076, 1.000000000000000000, 0.8660254037844387076, 1.000000000000000000, 0.8660254037844387076, 1.000000000000000000, 0.8660254037844387076, 1.000000000000000000, 0.8660254037844387076, 1.000000000000000000, 0.8660254037844387076, 1.000000000000000000, 0.8660254037844387076, 1.000000000000000000, 0.8660254037844387076, 1.000000000000000000, 0.8660254037844387076, 1.000000000000000000, 0.8660254037844387076, 1.000000000000000000, 0.8660254037844387076, 1.000000000000000000, 0.8660254037844387076, 1.000000000000000000, 0.8660254037844387076, 1.000000000000000000, 0.8660254037844387076, 1.000000000000000000, 0.8660254037844387076, 1.000000000000000000, 0.8660254037844387076, 1.000000000000000000, 0.8660254037844387076, 1.000000000000000000, 0.8660254037844387076, 1.000000000000000000, 0.8660254037844387076, 1.000000000000000000, 0.8660254037844387076, 1.000000000000000000, 0.8660254037844387076, 1.000000000000000000, 0.8660254037844387076, 1.000000000000000000, 0.8660254037844387076, 1.000000000000000000, 0.8660254037844387076, 1.000000000000000000, 0.8660254037844387076, 1.000000000000000000, 0.8660254037844387076, 1.000000000000000000, 0.8660254037844387076, 1.000000000000000000, 0.8660254037844387076, 1.000000000000000000, 0.8660254037844387076, 1.000000000000000000, 0.8660254037844387076, 1.000000000000000000, 0.8660254037844387076, 1.000000000000000000, 0.8660254037844387076, 1.000000000000000000, 0.8660254037844387076, 1.000000000000000000, 0.8660254037844387076, 1.000000000000000000, 0.8660254037844387076, 1.000000000000000000, 0.8660254037844387076, 1.000000000000000000, 0.8660254037844387076, 1.000000000000000000, 0.8660254037844387076, 1.000000000000000000, 0.8660254037844387076, 1.000000000000000000, 0.8660254037844387076, 1.000000000000000000, 0.8660254037844387076, 1.000000000000000000, 0.8660254037844387076, 1.000000000000000000, 0.8660254037844387076, 1.000000000000000000, 0.8660254037844387076, 1.000000000000000000, 0.8660254037844387076, 1.000000000000000000, 0.8660254037844387076, 1.000000000000000000, 0.8660254037844387076, 1.000000000000000000, 0.8660254037844387076, 1.000000000000000000, 0.8660254037844387076, 1.000000000000000000, 0.8660254037844387076, 1.000000000000000000, 0.8660254037844387076, 1.000000000000000000, 0.8660254037844387076, 1.000000000000000000, 0.8660254037844387076, 1.000000000000000000, 0.8660254037844387076, 1.000000000000000000, 0.8660254037844387076, 1.000000000000000000, 0.8660254037844387076, 1.000000000000000000, 0.8660254037844387076, 1.000000000000000000, 0.8660254037844387076, 1.000000000000000000, 0.8660254037844387076, 1.000000000000000000, 0.8660254037844387076, 1.000000000000000000, 0.8660254037844387076, 1.000000000000000000, 0.8660254037844387076, 1.000000000000000000, 0.8660254037844387076, 1.000000000000000000, 0.8660254037844387076, 1.000000000000000000, 0.8660254037844387076, 1.000000000000000000, 0.8660254037844387076, 1.000000000000000000, 0.8660254037844387076, 1.000000000000000000, 0.8660254037844387076, 1.000000000000000000, 0.8660254037844387076, 1.000000000000000000, 0.8660254037844387076, 1.000000000000000000, 0.8660254037844387076, 1.000000000000000000, 0.8660254037844387076, 1.000000000000000000, 0.8660254037844387076, 1.000000000000000000, 0.8660254037844387076, 1.000000000000000000, 0.8660254037844387076, 1.000000000000000000, 0.8660254037844387076, 1.000000000000000000, 0.8660254037844387076, 1.000000000000000000, 0.8660254037844387076, 1.000000000000000000, 0.8660254037844387076, 1.000000000000000000, 0.8660254037844387076, 1.000000000000000000, 0.8660254037844387076, 1.000000000000000000, 0.8660254037844387076, 1.000000000000000000, 0.8660254037844387076, 1.000000000000000000, 0.8660254037844387076, 1.000000000000000000, 0.8660254037844387076, 1.000000000000000000, 0.8660254037844387076, 1.000000000000000000, 0.8660254037844387076, 1.000000000000000000, 0.8660254037844387076, 1.000000000000000000, 0.8660254037844387076, 1.000000000000000000, 0.8660254037844387076, 1.000000000000000000, 0.8660254037844387076, 1.000000000000000000, 0.8660254037844387076, 1.000000000000000000, 0.8660254037844387076, 1.000000000000000000, 0.8660254037844387076, 1.000000000000000000, 0.8660254037844387076, 1.000000000000000000, 0.8660254037844387076, 1.000000000000000000, 0.8660254037844387076, 1.000000000000000000, 0.8660254037844387076, 1.000000000000000000, 0.8660254037844387076, 1.000000000000000000, 0.8660254037844387076, 1.000000000000000000, 0.8660254037844387076, 1.000000000000000000, 0.8660254037844387076, 1.000000000000000000, 0.8660254037844387076, 1.000000000000000000, 0.8660254037844387076, 1.000000000000000000, 0.8660254037844387076, 1.000000000000000000, 0.8660254037844387076, 1.000000000000000000, 0.8660254037844387076, 1.000000000000000000, 0.8660254037844387076, 1.000000000000000000, 0.8660254037844387076, 1.000000000000000000, 0.8660254037844387076, 1.000000000000000000, 0.8660254037844387076, 1.000000000000000000, 0.8660254037844387076, 1.000000000000000000, 0.8660254037844387076, 1.000000000000000000, 0.8660254037844387076, 1.000000000000000000, 0.8660254037844387076, 1.000000000000000000, 0.8660254037844387076, 1.000000000000000000, 0.8660254037844387076, 1.000000000000000000, 0.8660254037844387076, 1.000000000000000000, 0.8660254037844387076, 1.000000000000000000, 0.8660254037844387076, 1.000000000000000000, 0.8660254037844387076, 1.000000000000000000, 0.8660254037844387076, 1.000000000000000000, 0.8660254037844387076, 1.000000000000000000, 0.8660254037844387076, 1.000000000000000000, 0.8660254037844387076, 1.000000000000000000, 0.8660254037844387076, 1.000000000000000000, 0.8660254037844387076, 1.000000000000000000, 0.8660254037844387076, 1.000000000000000000, 0.8660254037844387076, 1.000000000000000000, 0.8660254037844387076, 1.000000000000000000, 0.8660254037844387076, 1.000000000000000000, 0.8660254037844387076, 1.000000000000000000, 0.8660254037844387076, 1.000000000000000000, 0.8660254037844387076, 1.000000000000000000, 0.8660254037844387076, 1.000000000000000000, 0.8660254037844387076, 1.000000000000000000, 0.8660254037844387076, 1.000000000000000000, 0.8660254037844387076, 1.000000000000000000, 0.8660254037844387076, 1.000000000000000000, 0.8660254037844387076, 1.000000000000000000, 0.8660254037844387076, 1.000000000000000000, 0.8660254037844387076, 1.000000000000000000, 0.8660254037844387076, 1.000000000000000000, 0.8660254037844387076, 1.000000000000000000, 0.8660254037844387076, 1.000000000000000000, 0.8660254037844387076, 1.000000000000000000, 0.8660254037844387076, 1.000000000000000000, 0.8660254037844387076, 1.000000000000000000, 0.8660254037844387076, 1.000000000000000000, 0.8660254037844387076, 1.000000000000000000, 0.8660254037844387076, 1.000000000000000000, 0.8660254037844387076, 1.000000000000000000, 0.8660254037844387076, 1.000000000000000000, 0.8660254037844387076, 1.000000000000000000, 0.8660254037844387076, 1.000000000000000000, 0.8660254037844387076, 1.000000000000000000, 0.8660254037844387076, 1.000000000000000000, 0.8660254037844387076, 1.000000000000000000, 0.8660254037844387076, 1.000000000000000000, 0.8660254037844387076, 1.000000000000000000, 0.8660254037844387076, 1.000000000000000000, 0.8660254037844387076, 1.000000000000000000, 0.8660254037844387076, 1.000000000000000000, 0.8660254037844387076, 1.000000000000000000, 0.8660254037844387076, 1.000000000000000000, 0.8660254037844387076, 1.000000000000000000, 0.8660254037844387076, 1.000000000000000000, 0.8660254037844387076, 1.000000000000000000, 0.8660254037844387076, 1.000000000000000000),
 ( 1.000000000000000000, 0.8660254037844387076, 1.000000000000000000, 0.8660254037844387076, 1.000000000000000000, 0.8660254037844387076, 1.000000000000000000, 0.8660254037844387076, 1.000000000000000000, 0.8660254037844387076, 1.000000000000000000, 0.8660254037844387076, 1.000000000000000000, 0.8660254037844387076, 1.000000000000000000, 0.8660254037844387076, 1.000000000000000000, 0.8660254037844387076, 1.000000000000000000, 0.8660254037844387076, 1.000000000000000000, 0.8660254037844387076, 1.000000000000000000, 0.8660254037844387076, 1.000000000000000000, 0.8660254037844387076, 1.000000000000000000, 0.8660254037844387076, 1.000000000000000000, 0.8660254037844387076, 1.000000000000000000, 0.8660254037844387076, 1.000000000000000000, 0.8660254037844387076, 1.000000000000000000, 0.8660254037844387076, 1.000000000000000000, 0.8660254037844387076, 1.000000000000000000, 0.8660254037844387076, 1.000000000000000000, 0.8660254037844387076, 1.000000000000000000, 0.8660254037844387076, 1.000000000000000000, 0.8660254037844387076, 1.000000000000000000, 0.8660254037844387076, 1.000000000000000000, 0.8660254037844387076, 1.000000000000000000, 0.8660254037844387076, 1.000000000000000000, 0.8660254037844387076, 1.000000000000000000, 0.8660254037844387076, 1.000000000000000000, 0.8660254037844387076, 1.000000000000000000, 0.8660254037844387076, 1.000000000000000000, 0.8660254037844387076, 1.000000000000000000, 0.8660254037844387076, 1.000000000000000000, 0.8660254037844387076, 1.000000000000000000, 0.8660254037844387076, 1.000000000000000000, 0.8660254037844387076, 1.000000000000000000, 0.8660254037844387076, 1.000000000000000000, 0.8660254037844387076, 1.000000000000000000, 0.8660254037844387076, 1.000000000000000000, 0.8660254037844387076, 1.000000000000000000, 0.8660254037844387076, 1.000000000000000000, 0.8660254037844387076, 1.000000000000000000, 0.8660254037844387076, 1.000000000000000000, 0.8660254037844387076, 1.000000000000000000, 0.8660254037844387076, 1.000000000000000000, 0.8660254037844387076, 1.000000000000000000, 0.8660254037844387076, 1.000000000000000000, 0.8660254037844387076, 1.000000000000000000, 0.8660254037844387076, 1.000000000000000000, 0.8660254037844387076, 1.000000000000000000, 0.8660254037844387076, 1.000000000000000000, 0.8660254037844387076, 1.000000000000000000, 0.8660254037844387076, 1.000000000000000000, 0.8660254037844387076, 1.000000000000000000, 0.8660254037844387076, 1.000000000000000000, 0.8660254037844387076, 1.000000000000000000, 0.8660254037844387076, 1.000000000000000000, 0.8660254037844387076, 1.000000000000000000, 0.8660254037844387076, 1.000000000000000000, 0.8660254037844387076, 1.000000000000000000, 0.8660254037844387076, 1.000000000000000000, 0.8660254037844387076, 1.000000000000000000, 0.8660254037844387076, 1.000000000000000000, 0.8660254037844387076, 1.000000000000000000, 0.8660254037844387076, 1.000000000000000000, 0.8660254037844387076, 1.000000000000000000, 0.8660254037844387076, 1.000000000000000000, 0.8660254037844387076, 1.000000000000000000, 0.8660254037844387076, 1.000000000000000000, 0.8660254037844387076, 1.000000000000000000, 0.8660254037844387076, 1.000000000000000000, 0.8660254037844387076, 1.000000000000000000, 0.8660254037844387076, 1.000000000000000000, 0.8660254037844387076, 1.000000000000000000, 0.8660254037844387076, 1.000000000000000000, 0.8660254037844387076, 1.000000000000000000, 0.8660254037844387076, 1.000000000000000000, 0.8660254037844387076, 1.000000000000000000, 0.8660254037844387076, 1.000000000000000000, 0.8660254037844387076, 1.000000000000000000, 0.8660254037844387076, 1.000000000000000000, 0.8660254037844387076, 1.000000000000000000, 0.8660254037844387076, 1.000000000000000000, 0.8660254037844387076, 1.000000000000000000, 0.8660254037844387076, 1.000000000000000000, 0.8660254037844387076, 1.000000000000000000, 0.8660254037844387076, 1.000000000000000000, 0.8660254037844387076, 1.000000000000000000, 0.8660254037844387076, 1.000000000000000000, 0.8660254037844387076, 1.000000000000000000, 0.8660254037844387076, 1.000000000000000000, 0.8660254037844387076, 1.000000000000000000, 0.8660254037844387076, 1.000000000000000000, 0.8660254037844387076, 1.000000000000000000, 0.8660254037844387076, 1.000000000000000000, 0.8660254037844387076, 1.000000000000000000, 0.8660254037844387076, 1.000000000000000000, 0.8660254037844387076, 1.000000000000000000, 0.8660254037844387076, 1.000000000000000000, 0.8660254037844387076, 1.000000000000000000, 0.8660254037844387076, 1.000000000000000000, 0.8660254037844387076, 1.000000000000000000, 0.8660254037844387076, 1.000000000000000000, 0.8660254037844387076, 1.000000000000000000, 0.8660254037844387076, 1.000000000000000000, 0.8660254037844387076, 1.000000000000000000, 0.8660254037844387076, 1.000000000000000000, 0.8660254037844387076, 1.000000000000000000, 0.8660254037844387076, 1.000000000000000000, 0.8660254037844387076, 1.000000000000000000, 0.8660254037844387076, 1.000000000000000000, 0.8660254037844387076, 1.000000000000000000, 0.8660254037844387076, 1.000000000000000000, 0.8660254037844387076, 1.000000000000000000, 0.8660254037844387076, 1.000000000000000000, 0.8660254037844387076, 1.000000000000000000, 0.8660254037844387076, 1.000000000000000000, 0.8660254037844387076, 1.000000000000000000, 0.8660254037844387076, 1.000000000000000000, 0.8660254037844387076, 1.000000000000000000, 0.8660254037844387076, 1.000000000000000000, 0.8660254037844387076, 1.000000000000000000, 0.8660254037844387076, 1.000000000000000000, 0.8660254037844387076, 1.000000000000000000, 0.8660254037844387076, 1.000000000000000000, 0.8660254037844387076, 1.000000000000000000, 0.8660254037844387076, 1.000000000000000000, 0.8660254037844387076, 1.000000000000000000, 0.8660254037844387076, 1.000000000000000000, 0.8660254037844387076, 1.000000000000000000, 0.8660254037844387076, 1.000000000000000000, 0.8660254037844387076, 1.000000000000000000, 0.8660254037844387076, 1.000000000000000000, 0.8660254037844387076, 1.000000000000000000, 0.8660254037844387076, 1.000000000000000000, 0.8660254037844387076, 1.000000000000000000, 0.8660254037844387076, 1.000000000000000000, 0.8660254037844387076, 1.000000000000000000, 0.8660254037844387076, 1.000000000000000000, 0.8660254037844387076, 1.000000000000000000, 0.8660254037844387076, 1.000000000000000000, 0.8660254037844387076, 1.000000000000000000, 0.8660254037844387076, 1.000000000000000000, 0.8660254037844387076, 1.000000000000000000, 0.8660254037844387076, 1.000000000000000000, 0.8660254037844387076, 1.000000000000000000, 0.8660254037844387076, 1.000000000000000000, 0.8660254037844387076, 1.000000000000000000, 0.8660254037844387076, 1.000000000000000000, 0.8660254037844387076, 1.000000000000000000, 0.8660254037844387076, 1.000000000000000000, 0.8660254037844387076, 1.000000000000000000, 0.8660254037844387076, 1.000000000000000000, 0.8660254037844387076, 1.000000000000000000, 0.8660254037844387076, 1.000000000000000000, 0.8660254037844387076, 1.000000000000000000, 0.8660254037844387076, 1.000000000000000000, 0.8660254037844387076, 1.000000000000000000, 0.8660254037844387076, 1.000000000000000000, 0.8660254037844387076, 1.000000000000000000, 0.8660254037844387076, 1.000000000000000000, 0.8660254037844387076, 1.000000000000000000, 0.8660254037844387076, 1.000000000000000000, 0.8660254037844387076, 1.000000000000000000, 0.8660254037844387076, 1.000000000000000000, 0.8660254037844387076, 1.000000000000000000, 0.8660254037844387076, 1.000000000000000000, 0.8660254037844387076, 1.000000000000000000, 0.8660254037844387076, 1.000000000000000000, 0.8660254037844387076, 1.000000000000000000, 0.8660254037844387076, 1.000000000000000000, 0.8660254037844387076, 1.000000000000000000, 0.8660254037844387076, 1.000000000000000000, 0.8660254037844387076, 1.000000000000000000, 0.8660254037844387076, 1.000000000000000000, 0.8660254037844387076, 1.000000000000000000, 0.8660254037844387076, 1.000000000000000000, 0.8660254037844387076, 1.000000000000000000, 0.8660254037844387076, 1.000000000000000000, 0.8660254037844387076, 1.000000000000000000, 0.8660254037844387076, 1.000000000000000000, 0.8660254037844387076, 1.000000000000000000, 0.8660254037844387076, 1.000000000000000000, 0.8660254037844387076, 1.000000000000000000, 0.8660254037844387076, 1.000000000000000000, 0.8660254037844387076, 1.000000000000000000, 0.8660254037844387076, 1.000000000000000000, 0.8660254037844387076, 1.000000000000000000, 0.8660254037844387076, 1.000000000000000000, 0.8660254037844387076, 1.000000000000000000, 0.8660254037844387076, 1.000000000000000000, 0.8660254037844387076, 1.000000000000000000, 0.8660254037844387076, 1.000000000000000000, 0.8660254037844387076, 1.000000000000000000, 0.8660254037844387076, 1.000000000000000000, 0.8660254037844387076, 1.000000000000000000, 0.8660254037844387076, 1.000000000000000000, 0.8660254037844387076, 1.000000000000000000, 0.8660254037844387076, 1.000000000000000000, 0.8660254037844387076, 1.000000000000000000, 0.8660254037844387076, 1.000000000000000000, 0.8660254037844387076, 1.000000000000000000, 0.8660254037844387076, 1.000000000000000000, 0.8660254037844387076, 1.000000000000000000, 0.8660254037844387076, 1.000000000000000000, 0.8660254037844387076, 1.000000000000000000, 0.8660254037844387076, 1.000000000000000000, 0.8660254037844387076, 1.000000000000000000, 0.8660254037844387076, 1.000000000000000000, 0.8660254037844387076, 1.000000000000000000, 0.8660254037844387076, 1.000000000000000000, 0.8660254037844387076, 1.000000000000000000, 0.8660254037844387076, 1.000000000000000000, 0.8660254037844387076, 1.000000000000000000, 0.8660254037844387076, 1.000000000000000000, 0.8660254037844387076, 1.000000000000000000, 0.8660254037844387076, 1.000000000000000000, 0.8660254037844387076, 1.000000000000000000, 0.8660254037844387076, 1.000000000000000000, 0.8660254037844387076, 1.000000000000000000, 0.8660254037844387076, 1.000000000000000000, 0.8660254037844387076, 1.000000000000000000, 0.8660254037844387076, 1.000000000000000000, 0.8660254037844387076, 1.000000000000000000, 0.8660254037844387076, 1.000000000000000000, 0.8660254037844387076, 1.000000000000000000, 0.8660254037844387076, 1.000000000000000000, 0.8660254037844387076, 1.000000000000000000, 0.8660254037844387076, 1.000000000000000000, 0.8660254037844387076, 1.000000000000000000, 0.8660254037844387076, 1.000000000000000000, 0.8660254037844387076, 1.000000000000000000, 0.8660254037844387076, 1.000000000000000000, 0.8660254037844387076, 1.000000000000000000, 0.8660254037844387076, 1.000000000000000000, 0.8660254037844387076, 1.000000000000000000, 0.8660254037844387076, 1.000000000000000000, 0.8660254037844387076, 1.000000000000000000, 0.8660254037844387076, 1.000000000000000000, 0.8660254037844387076, 1.000000000000000000, 0.8660254037844387076, 1.000000000000000000, 0.8660254037844387076, 1.000000000000000000, 0.8660254037844387076, 1.000000000000000000, 0.8660254037844387076, 1.000000000000000000, 0.8660254037844387076, 1.000000000000000000, 0.8660254037844387076, 1.000000000000000000, 0.8660254037844387076, 1.000000000000000000, 0.8660254037844387076, 1.000000000000000000, 0.8660254037844387076, 1.000000000000000000, 0.8660254037844387076, 1.000000000000000000, 0.8660254037844387076, 1.000000000000000000, 0.8660254037844387076, 1.000000000000000000, 0.8660254037844387076, 1.000000000000000000, 0.8660254037844387076, 1.000000000000000000, 0.8660254037844387076, 1.000000000000000000, 0.8660254037844387076, 1.000000000000000000, 0.8660254037844387076, 1.000000000000000000, 0.8660254037844387076, 1.000000000000000000, 0.8660254037844387076, 1.000000000000000000, 0.8660254037844387076, 1.000000000000000000, 0.8660254037844387076, 1.000000000000000000, 0.8660254037844387076, 1.000000000000000000, 0.8660254037844387076, 1.000000000000000000, 0.8660254037844387076, 1.000000000000000000, 0.8660254037844387076, 1.000000000000000000, 0.8660254037844387076, 1.000000000000000000, 0.8660254037844387076, 1.000000000000000000, 0.8660254037844387076, 1.000000000000000000, 0.8660254037844387076, 1.000000000000000000, 0.8660254037844387076, 1.000000000000000000, 0.8660254037844387076, 1.000000000000000000, 0.8660254037844387076, 1.000000000000000000, 0.8660254037844387076, 1.000000000000000000, 0.8660254037844387076, 1.000000000000000000, 0.8660254037844387076, 1.000000000000000000, 0.8660254037844387076, 1.000000000000000000, 0.8660254037844387076, 1.000000000000000000, 0.8660254037844387076, 1.000000000000000000, 0.8660254037844387076, 1.000000000000000000, 0.8660254037844387076, 1.000000000000000000, 0.8660254037844387076, 1.000000000000000000, 0.8660254037844387076, 1.000000000000000000, 0.8660254037844387076, 1.000000000000000000, 0.8660254037844387076, 1.000000000000000000, 0.8660254037844387076, 1.000000000000000000, 0.8660254037844387076, 1.000000000000000000, 0.8660254037844387076, 1.000000000000000000, 0.8660254037844387076, 1.000000000000000000, 0.8660254037844387076, 1.000000000000000000, 0.8660254037844387076, 1.000000000000000000, 0.8660254037844387076, 1.000000000000000000, 0.8660254037844387076, 1.000000000000000000, 0.8660254037844387076, 1.000000000000000000, 0.8660254037844387076, 1.000000000000000000, 0.8660254037844387076, 1.000000000000000000, 0.8660254037844387076, 1.000000000000000000, 0.8660254037844387076, 1.000000000000000000, 0.8660254037844387076, 1.000000000000000000, 0.8660254037844387076, 1.000000000000000000, 0.8660254037844387076, 1.000000000000000000, 0.8660254037844387076, 1.000000000000000000, 0.8660254037844387076, 1.000000000000000000, 0.8660254037844387076, 1.000000000000000000, 0.8660254037844387076, 1.000000000000000000, 0.8660254037844387076, 1.000000000000000000, 0.8660254037844387076, 1.000000000000000000, 0.8660254037844387076, 1.000000000000000000, 0.8660254037844387076, 1.000000000000000000, 0.8660254037844387076, 1.000000000000000000, 0.8660254037844387076, 1.000000000000000000, 0.8660254037844387076, 1.000000000000000000, 0.8660254037844387076, 1.000000000000000000, 0.8660254037844387076, 1.000000000000000000, 0.8660254037844387076, 1.000000000000000000, 0.8660254037844387076, 1.000000000000000000, 0.8660254037844387076, 1.000000000000000000, 0.8660254037844387076, 1.000000000000000000, 0.8660254037844387076, 1.000000000000000000, 0.8660254037844387076, 1.000000000000000000, 0.8660254037844387076, 1.000000000000000000, 0.8660254037844387076, 1.000000000000000000, 0.8660254037844387076, 1.000000000000000000, 0.8660254037844387076, 1.000000000000000000, 0.8660254037844387076, 1.000000000000000000, 0.8660254037844387076, 1.000000000000000000, 0.8660254037844387076, 1.000000000000000000, 0.8660254037844387076, 1.000000000000000000, 0.8660254037844387076, 1.000000000000000000, 0.8660254037844387076, 1.000000000000000000, 0.8660254037844387076, 1.000000000000000000, 0.8660254037844387076, 1.000000000000000000, 0.8660254037844387076, 1.000000000000000000, 0.8660254037844387076, 1.000000000000000000, 0.8660254037844387076, 1.000000000000000000, 0.8660254037844387076, 1.000000000000000000, 0.8660254037844387076, 1.000000000000000000, 0.8660254037844387076, 1.000000000000000000, 0.8660254037844387076, 1.000000000000000000, 0.8660254037844387076, 1.000000000000000000, 0.8660254037844387076, 1.000000000000000000, 0.8660254037844387076, 1.000000000000000000, 0.8660254037844387076, 1.000000000000000000, 0.8660254037844387076, 1.000000000000000000, 0.8660254037844387076, 1.000000000000000000, 0.8660254037844387076, 1.000000000000000000, 0.8660254037844387076, 1.000000000000000000, 0.8660254037844387076, 1.000000000000000000, 0.8660254037844387076, 1.000000000000000000, 0.8660254037844387076, 1.000000000000000000, 0.8660254037844387076, 1.000000000000000000, 0.8660254037844387076, 1.000000000000000000, 0.8660254037844387076, 1.000000000000000000, 0.8660254037844387076, 1.000000000000000000, 0.8660254037844387076, 1.000000000000000000, 0.8660254037844387076, 1.000000000000000000, 0.8660254037844387076, 1.000000000000000000, 0.8660254037844387076, 1.000000000000000000, 0.8660254037844387076, 1.000000000000000000, 0.8660254037844387076, 1.000000000000000000, 0.8660254037844387076, 1.000000000000000000, 0.8660254037844387076, 1.000000000000000000, 0.8660254037844387076, 1.000000000000000000, 0.8660254037844387076, 1.000000000000000000, 0.8660254037844387076, 1.000000000000000000, 0.8660254037844387076, 1.000000000000000000, 0.8660254037844387076, 1.000000000000000000, 0.8660254037844387076, 1.000000000000000000, 0.8660254037844387076, 1.000000000000000000, 0.8660254037844387076, 1.000000000000000000, 0.8660254037844387076, 1.000000000000000000, 0.8660254037844387076, 1.000000000000000000, 0.8660254037844387076, 1.000000000000000000, 0.8660254037844387076, 1.000000000000000000, 0.8660254037844387076, 1.000000000000000000, 0.8660254037844387076, 1.000000000000000000, 0.8660254037844387076, 1.000000000000000000, 0.8660254037844387076, 1.000000000000000000, 0.8660254037844387076, 1.000000000000000000, 0.8660254037844387076, 1.000000000000000000, 0.8660254037844387076, 1.000000000000000000, 0.8660254037844387076, 1.000000000000000000, 0.8660254037844387076, 1.000000000000000000, 0.8660254037844387076, 1.000000000000000000, 0.8660254037844387076, 1.000000000000000000, 0.8660254037844387076, 1.000000000000000000, 0.8660254037844387076, 1.000000000000000000, 0.8660254037844387076, 1.000000000000000000, 0.8660254037844387076, 1.000000000000000000, 0.8660254037844387076, 1.000000000000000000, 0.8660254037844387076, 1.000000000000000000, 0.8660254037844387076, 1.000000000000000000, 0.8660254037844387076, 1.000000000000000000, 0.8660254037844387076, 1.000000000000000000, 0.8660254037844387076, 1.000000000000000000, 0.8660254037844387076, 1.000000000000000000, 0.8660254037844387076, 1.000000000000000000, 0.8660254037844387076, 1.000000000000000000, 0.8660254037844387076, 1.000000000000000000, 0.8660254037844387076, 1.000000000000000000, 0.8660254037844387076, 1.000000000000000000, 0.8660254037844387076, 1.000000000000000000, 0.8660254037844387076, 1.000000000000000000, 0.8660254037844387076, 1.000000000000000000, 0.8660254037844387076, 1.000000000000000000, 0.8660254037844387076, 1.000000000000000000, 0.8660254037844387076, 1.000000000000000000, 0.8660254037844387076, 1.000000000000000000, 0.8660254037844387076, 1.000000000000000000, 0.8660254037844387076, 1.000000000000000000, 0.8660254037844387076, 1.000000000000000000, 0.8660254037844387076, 1.000000000000000000, 0.8660254037844387076, 1.000000000000000000, 0.8660254037844387076, 1.000000000000000000, 0.8660254037844387076, 1.000000000000000000, 0.8660254037844387076, 1.000000000000000000, 0.8660254037844387076, 1.000000000000000000, 0.8660254037844387076, 1.000000000000000000, 0.8660254037844387076, 1.000000000000000000, 0.8660254037844387076, 1.000000000000000000, 0.8660254037844387076, 1.000000000000000000, 0.8660254037844387076, 1.000000000000000000, 0.8660254037844387076, 1.000000000000000000, 0.8660254037844387076, 1.000000000000000000, 0.8660254037844387076, 1.000000000000000000, 0.8660254037844387076, 1.000000000000000000, 0.8660254037844387076, 1.000000000000000000, 0.8660254037844387076, 1.000000000000000000, 0.8660254037844387076, 1.000000000000000000, 0.8660254037844387076, 1.000000000000000000, 0.8660254037844387076, 1.000000000000000000, 0.8660254037844387076, 1.000000000000000000, 0.8660254037844387076, 1.000000000000000000, 0.8660254037844387076, 1.000000000000000000, 0.8660254037844387076, 1.000000000000000000, 0.8660254037844387076, 1.000000000000000000, 0.8660254037844387076, 1.000000000000000000, 0.8660254037844387076, 1.000000000000000000, 0.8660254037844387076, 1.000000000000000000, 0.8660254037844387076, 1.000000000000000000, 0.8660254037844387076, 1.000000000000000000, 0.8660254037844387076, 1.000000000000000000, 0.8660254037844387076, 1.000000000000000000, 0.8660254037844387076, 1.000000000000000000, 0.8660254037844387076, 1.000000000000000000, 0.8660254037844387076, 1.000000000000000000, 0.8660254037844387076, 1.000000000000000000, 0.8660254037844387076, 1.000000000000000000, 0.8660254037844387076, 1.000000000000000000, 0.8660254037844387076, 1.000000000000000000, 0.8660254037844387076, 1.000000000000000000, 0.8660254037844387076, 1.000000000000000000, 0.8660254037844387076, 1.000000000000000000, 0.8660254037844387076, 1.000000000000000000, 0.8660254037844387076, 1.000000000000000000, 0.8660254037844387076, 1.000000000000000000, 0.8660254037844387076, 1.000000000000000000, 0.8660254037844387076, 1.000000000000000000, 0.8660254037844387076, 1.000000000000000000, 0.8660254037844387076, 1.000000000000000000, 0.8660254037844387076, 1.000000000000000000, 0.8660254037844387076, 1.000000000000000000, 0.8660254037844387076, 1.000000000000000000, 0.8660254037844387076, 1.000000000000000000, 0.8660254037844387076, 1.000000000000000000, 0.8660254037844387076, 1.000000000000000000, 0.8660254037844387076, 1.000000000000000000, 0.8660254037844387076, 1.000000000000000000, 0.8660254037844387076, 1.000000000000000000, 0.8660254037844387076, 1.000000000000000000, 0.8660254037844387076, 1.000000000000000000, 0.8660254037844387076, 1.000000000000000000, 0.8660254037844387076, 1.000000000000000000, 0.8660254037844387076, 1.000000000000000000, 0.8660254037844387076, 1.000000000000000000, 0.8660254037844387076, 1.000000000000000000, 0.8660254037844387076, 1.000000000000000000, 0.8660254037844387076, 1.000000000000000000, 0.8660254037844387076, 1.000000000000000000, 0.8660254037844387076, 1.000000000000000000, 0.8660254037844387076, 1.000000000000000000, 0.8660254037844387076, 1.000000000000000000, 0.8660254037844387076, 1.000000000000000000, 0.8660254037844387076, 1.000000000000000000, 0.8660254037844387076, 1.000000000000000000, 0.8660254037844387076, 1.000000000000000000, 0.8660254037844387076, 1.000000000000000000, 0.8660254037844387076, 1.000000000000000000, 0.8660254037844387076, 1.000000000000000000, 0.8660254037844387076, 1.000000000000000000, 0.8660254037844387076, 1.000000000000000000, 0.8660254037844387076, 1.000000000000000000, 0.8660254037844387076, 1.000000000000000000, 0.8660254037844387076, 1.000000000000000000, 0.8660254037844387076, 1.000000000000000000, 0.8660254037844387076, 1.000000000000000000, 0.8660254037844387076, 1.000000000000000000, 0.8660254037844387076, 1.000000000000000000, 0.8660254037844387076, 1.000000000000000000, 0.8660254037844387076, 1.000000000000000000, 0.8660254037844387076, 1.000000000000000000, 0.8660254037844387076, 1.000000000000000000, 0.8660254037844387076, 1.000000000000000000, 0.8660254037844387076, 1.000000000000000000, 0.8660254037844387076, 1.000000000000000000, 0.8660254037844387076, 1.000000000000000000, 0.8660254037844387076, 1.000000000000000000, 0.8660254037844387076, 1.000000000000000000, 0.8660254037844387076, 1.000000000000000000, 0.8660254037844387076, 1.000000000000000000, 0.8660254037844387076, 1.000000000000000000, 0.8660254037844387076, 1.000000000000000000, 0.8660254037844387076, 1.000000000000000000, 0.8660254037844387076, 1.000000000000000000, 0.8660254037844387076, 1.000000000000000000, 0.8660254037844387076, 1.000000000000000000, 0.8660254037844387076, 1.000000000000000000, 0.8660254037844387076, 1.000000000000000000, 0.8660254037844387076, 1.000000000000000000, 0.8660254037844387076, 1.000000000000000000, 0.8660254037844387076, 1.000000000000000000, 0.8660254037844387076, 1.000000000000000000, 0.8660254037844387076, 1.000000000000000000, 0.8660254037844387076, 1.000000000000000000, 0.8660254037844387076, 1.000000000000000000, 0.8660254037844387076, 1.000000000000000000, 0.8660254037844387076, 1.000000000000000000, 0.8660254037844387076, 1.000000000000000000, 0.8660254037844387076, 1.000000000000000000, 0.8660254037844387076, 1.000000000000000000, 0.8660254037844387076, 1.000000000000000000, 0.8660254037844387076, 1.000000000000000000, 0.8660254037844387076, 1.000000000000000000, 0.8660254037844387076, 1.000000000000000000, 0.8660254037844387076, 1.000000000000000000, 0.8660254037844387076, 1.000000000000000000, 0.8660254037844387076, 1.000000000000000000, 0.8660254037844387076, 1.000000000000000000, 0.8660254037844387076, 1.000000000000000000, 0.8660254037844387076, 1.000000000000000000, 0.8660254037844387076, 1.000000000000000000, 0.8660254037844387076, 1.000000000000000000, 0.8660254037844387076, 1.000000000000000000, 0.8660254037844387076, 1.000000000000000000, 0.8660254037844387076, 1.000000000000000000, 0.8660254037844387076, 1.000000000000000000, 0.8660254037844387076, 1.000000000000000000, 0.8660254037844387076, 1.000000000000000000, 0.8660254037844387076, 1.000000000000000000, 0.8660254037844387076, 1.000000000000000000, 0.8660254037844387076, 1.000000000000000000, 0.8660254037844387076, 1.000000000000000000, 0.8660254037844387076, 1.000000000000000000, 0.8660254037844387076, 1.000000000000000000, 0.8660254037844387076, 1.000000000000000000, 0.8660254037844387076, 1.000000000000000000, 0.8660254037844387076, 1.000000000000000000, 0.8660254037844387076, 1.000000000000000000, 0.8660254037844387076, 1.000000000000000000, 0.8660254037844387076, 1.000000000000000000, 0.8660254037844387076, 1.000000000000000000, 0.8660254037844387076, 1.000000000000000000, 0.8660254037844387076, 1.000000000000000000, 0.8660254037844387076, 1.000000000000000000, 0.8660254037844387076, 1.000000000000000000, 0.8660254037844387076, 1.000000000000000000, 0.8660254037844387076, 1.000000000000000000, 0.8660254037844387076, 1.000000000000000000, 0.8660254037844387076, 1.000000000000000000, 0.8660254037844387076, 1.000000000000000000, 0.8660254037844387076, 1.000000000000000000, 0.8660254037844387076, 1.000000000000000000, 0.8660254037844387076, 1.000000000000000000, 0.8660254037844387076, 1.000000000000000000, 0.8660254037844387076, 1.000000000000000000, 0.8660254037844387076, 1.000000000000000000, 0.8660254037844387076, 1.000000000000000000, 0.8660254037844387076, 1.000000000000000000, 0.8660254037844387076, 1.000000000000000000, 0.8660254037844387076, 1.000000000000000000, 0.8660254037844387076, 1.000000000000000000, 0.8660254037844387076, 1.000000000000000000, 0.8660254037844387076, 1.000000000000000000, 0.8660254037844387076, 1.000000000000000000, 0.8660254037844387076, 1.000000000000000000, 0.8660254037844387076, 1.000000000000000000, 0.8660254037844387076, 1.000000000000000000, 0.8660254037844387076, 1.000000000000000000, 0.8660254037844387076, 1.000000000000000000, 0.8660254037844387076, 1.000000000000000000, 0.8660254037844387076, 1.000000000000000000, 0.8660254037844387076, 1.000000000000000000, 0.8660254037844387076, 1.000000000000000000, 0.8660254037844387076, 1.000000000000000000, 0.8660254037844387076, 1.000000000000000000, 0.8660254037844387076, 1.000000000000000000, 0.8660254037844387076, 1.000000000000000000, 0.8660254037844387076, 1.000000000000000000, 0.8660254037844387076, 1.000000000000000000, 0.8660254037844387076, 1.000000000000000000, 0.8660254037844387076, 1.000000000000000000, 0.8660254037844387076, 1.000000000000000000, 0.8660254037844387076, 1.000000000000000000, 0.8660254037844387076, 1.000000000000000000, 0.8660254037844387076, 1.000000000000000000, 0.8660254037844387076, 1.000000000000000000, 0.8660254037844387076, 1.000000000000000000, 0.8660254037844387076, 1.000000000000000000, 0.8660254037844387076, 1.000000000000000000, 0.8660254037844387076, 1.000000000000000000, 0.8660254037844387076, 1.000000000000000000, 0.8660254037844387076, 1.000000000000000000, 0.8660254037844387076, 1.000000000000000000, 0.8660254037844387076, 1.000000000000000000, 0.8660254037844387076, 1.000000000000000000, 0.8660254037844387076, 1.000000000000000000, 0.8660254037844387076, 1.000000000000000000, 0.8660254037844387076, 1.000000000000000000, 0.8660254037844387076, 1.000000000000000000, 0.8660254037844387076, 1.000000000000000000, 0.8660254037844387076, 1.000000000000000000, 0.8660254037844387076, 1.000000000000000000, 0.8660254037844387076, 1.000000000000000000, 0.8660254037844387076, 1.000000000000000000, 0.8660254037844387076, 1.000000000000000000, 0.8660254037844387076, 1.000000000000000000, 0.8660254037844387076, 1.000000000000000000, 0.8660254037844387076, 1.000000000000000000, 0.8660254037844387076, 1.000000000000000000, 0.8660254037844387076, 1.000000000000000000, 0.8660254037844387076, 1.000000000000000000, 0.8660254037844387076, 1.000000000000000000, 0.8660254037844387076, 1.000000000000000000, 0.8660254037844387076, 1.000000000000000000, 0.8660254037844387076, 1.000000000000000000, 0.8660254037844387076, 1.000000000000000000, 0.8660254037844387076, 1.000000000000000000, 0.8660254037844387076, 1.000000000000000000, 0.8660254037844387076, 1.000000000000000000, 0.8660254037844387076, 1.000000000000000000, 0.8660254037844387076, 1.000000000000000000, 0.8660254037844387076, 1.000000000000000000, 0.8660254037844387076, 1.000000000000000000, 0.8660254037844387076, 1.000000000000000000, 0.8660254037844387076, 1.000000000000000000, 0.8660254037844387076, 1.000000000000000000, 0.8660254037844387076, 1.000000000000000000, 0.8660254037844387076, 1.000000000000000000, 0.8660254037844387076, 1.000000000000000000, 0.8660254037844387076, 1.000000000000000000, 0.8660254037844387076, 1.000000000000000000, 0.8660254037844387076, 1.000000000000000000, 0.8660254037844387076, 1.000000000000000000, 0.8660254037844387076, 1.000000000000000000, 0.8660254037844387076, 1.000000000000000000, 0.8660254037844387076, 1.000000000000000000, 0.8660254037844387076, 1.000000000000000000, 0.8660254037844387076, 1.000000000000000000, 0.8660254037844387076, 1.000000000000000000, 0.8660254037844387076, 1.000000000000000000, 0.8660254037844387076, 1.000000000000000000, 0.8660254037844387076, 1.000000000000000000, 0.8660254037844387076, 1.000000000000000000, 0.8660254037844387076, 1.000000000000000000, 0.8660254037844387076, 1.000000000000000000, 0.8660254037844387076, 1.000000000000000000, 0.8660254037844387076, 1.000000000000000000, 0.8660254037844387076, 1.000000000000000000, 0.8660254037844387076, 1.000000000000000000, 0.8660254037844387076, 1.000000000000000000, 0.8660254037844387076, 1.000000000000000000, 0.8660254037844387076, 1.000000000000000000, 0.8660254037844387076, 1.000000000000000000, 0.8660254037844387076, 1.000000000000000000, 0.8660254037844387076, 1.000000000000000000, 0.8660254037844387076, 1.000000000000000000, 0.8660254037844387076, 1.000000000000000000, 0.8660254037844387076, 1.000000000000000000, 0.8660254037844387076, 1.000000000000000000, 0.8660254037844387076, 1.000000000000000000, 0.8660254037844387076, 1.000000000000000000, 0.8660254037844387076, 1.000000000000000000, 0.8660254037844387076, 1.000000000000000000, 0.8660254037844387076, 1.000000000000000000, 0.8660254037844387076, 1.000000000000000000, 0.8660254037844387076, 1.000000000000000000, 0.8660254037844387076, 1.000000000000000000, 0.8660254037844387076, 1.000000000000000000, 0.8660254037844387076, 1.000000000000000000, 0.8660254037844387076, 1.000000000000000000, 0.8660254037844387076, 1.000000000000000000, 0.8660254037844387076, 1.000000000000000000, 0.8660254037844387076, 1.000000000000000000, 0.8660254037844387076, 1.000000000000000000, 0.8660254037844387076, 1.000000000000000000, 0.8660254037844387076, 1.000000000000000000, 0.8660254037844387076, 1.000000000000000000, 0.8660254037844387076, 1.000000000000000000, 0.8660254037844387076, 1.000000000000000000, 0.8660254037844387076, 1.000000000000000000, 0.8660254037844387076, 1.000000000000000000, 0.8660254037844387076, 1.000000000000000000, 0.8660254037844387076, 1.000000000000000000, 0.8660254037844387076, 1.000000000000000000, 0.8660254037844387076, 1.000000000000000000, 0.8660254037844387076, 1.000000000000000000, 0.8660254037844387076, 1.000000000000000000, 0.8660254037844387076, 1.000000000000000000, 0.8660254037844387076, 1.000000000000000000, 0.8660254037844387076, 1.000000000000000000, 0.8660254037844387076, 1.000000000000000000, 0.8660254037844387076, 1.000000000000000000, 0.8660254037844387076, 1.000000000000000000, 0.8660254037844387076, 1.000000000000000000, 0.8660254037844387076, 1.000000000000000000, 0.8660254037844387076, 1.000000000000000000, 0.8660254037844387076, 1.000000000000000000, 0.8660254037844387076, 1.000000000000000000, 0.8660254037844387076, 1.000000000000000000, 0.8660254037844387076, 1.000000000000000000, 0.8660254037844387076, 1.000000000000000000, 0.8660254037844387076, 1.000000000000000000, 0.8660254037844387076, 1.000000000000000000, 0.8660254037844387076, 1.000000000000000000, 0.8660254037844387076, 1.000000000000000000, 0.8660254037844387076, 1.000000000000000000, 0.8660254037844387076, 1.000000000000000000, 0.8660254037844387076, 1.000000000000000000, 0.8660254037844387076, 1.000000000000000000, 0.8660254037844387076, 1.000000000000000000, 0.8660254037844387076, 1.000000000000000000, 0.8660254037844387076, 1.000000000000000000, 0.8660254037844387076, 1.000000000000000000, 0.8660254037844387076, 1.000000000000000000, 0.8660254037844387076, 1.000000000000000000, 0.8660254037844387076, 1.000000000000000000, 0.8660254037844387076, 1.000000000000000000, 0.8660254037844387076, 1.000000000000000000, 0.8660254037844387076, 1.000000000000000000, 0.8660254037844387076, 1.000000000000000000, 0.8660254037844387076, 1.000000000000000000, 0.8660254037844387076, 1.000000000000000000, 0.8660254037844387076, 1.000000000000000000, 0.8660254037844387076, 1.000000000000000000, 0.8660254037844387076, 1.000000000000000000, 0.8660254037844387076, 1.000000000000000000, 0.8660254037844387076, 1.000000000000000000, 0.8660254037844387076, 1.000000000000000000, 0.8660254037844387076, 1.000000000000000000, 0.8660254037844387076, 1.000000000000000000, 0.8660254037844387076, 1.000000000000000000, 0.8660254037844387076, 1.000000000000000000, 0.8660254037844387076, 1.000000000000000000, 0.8660254037844387076, 1.000000000000000000, 0.8660254037844387076, 1.000000000000000000, 0.8660254037844387076, 1.000000000000000000, 0.8660254037844387076, 1.000000000000000000, 0.8660254037844387076, 1.000000000000000000, 0.8660254037844387076, 1.000000000000000000, 0.8660254037844387076, 1.000000000000000000, 0.8660254037844387076, 1.000000000000000000, 0.8660254037844387076, 1.000000000000000000, 0.8660254037844387076, 1.000000000000000000, 0.8660254037844387076, 1.000000000000000000, 0.8660254037844387076, 1.000000000000000000, 0.8660254037844387076, 1.000000000000000000, 0.8660254037844387076, 1.000000000000000000, 0.8660254037844387076, 1.000000000000000000, 0.8660254037844387076, 1.000000000000000000, 0.8660254037844387076, 1.000000000000000000, 0.8660254037844387076, 1.000000000000000000, 0.8660254037844387076, 1.000000000000000000, 0.8660254037844387076, 1.000000000000000000, 0.8660254037844387076, 1.000000000000000000, 0.8660254037844387076, 1.000000000000000000, 0.8660254037844387076, 1.000000000000000000, 0.8660254037844387076, 1.000000000000000000, 0.8660254037844387076, 1.000000000000000000, 0.8660254037844387076, 1.000000000000000000, 0.8660254037844387076, 1.000000000000000000, 0.8660254037844387076, 1.000000000000000000, 0.8660254037844387076, 1.000000000000000000, 0.8660254037844387076, 1.000000000000000000, 0.8660254037844387076, 1.000000000000000000, 0.8660254037844387076, 1.000000000000000000, 0.8660254037844387076, 1.000000000000000000, 0.8660254037844387076, 1.000000000000000000, 0.8660254037844387076, 1.000000000000000000, 0.8660254037844387076, 1.000000000000000000, 0.8660254037844387076, 1.000000000000000000, 0.8660254037844387076, 1.000000000000000000, 0.8660254037844387076, 1.000000000000000000, 0.8660254037844387076, 1.000000000000000000, 0.8660254037844387076, 1.000000000000000000, 0.8660254037844387076, 1.000000000000000000, 0.8660254037844387076, 1.000000000000000000, 0.8660254037844387076, 1.000000000000000000, 0.8660254037844387076, 1.000000000000000000, 0.8660254037844387076, 1.000000000000000000, 0.8660254037844387076, 1.000000000000000000, 0.8660254037844387076, 1.000000000000000000, 0.8660254037844387076, 1.000000000000000000) ) ) 
 REPRESENTATION_ITEM ( '' )  SURFACE ( )  );
#11342=CARTESIAN_POINT ( 'NONE',  ( 10.81189881249999729, 0.000000000000000000, -161.8437500020484094 ) ) ;
#11343=CARTESIAN_POINT ( 'NONE',  ( 10.81189881249999551, -6.242252689847874514, -176.9687500020484094 ) ) ;
#11352=CARTESIAN_POINT ( 'NONE',  ( -10.81189881249999729, 1.324075727343319199E-15, -59.09375000204835970 ) ) ;
#11353=CARTESIAN_POINT ( 'NONE',  ( 5.405949406249999534, 9.363379034771803333, -70.28125000204838102 ) ) ;
#11355=CARTESIAN_POINT ( 'NONE',  ( 5.000000000000000000, 8.660254037844385522, -133.7499999999999716 ) ) ;
#11356=CARTESIAN_POINT ( 'NONE',  ( 5.405949406249999534, 9.363379034771803333, -151.2812500020484094 ) ) ;
#11357=CARTESIAN_POINT ( 'NONE',  ( 7.644554776091147741E-16, 12.48450537969573659, -163.1562500020484094 ) ) ;
#11358=DIRECTION ( 'NONE',  ( -0.000000000000000000, -0.000000000000000000, -1.000000000000000000 ) ) ;
#11360=CARTESIAN_POINT ( 'NONE',  ( -10.81189881249999729, 1.324075727343319199E-15, -98.09375000204838102 ) ) ;
#11363=CARTESIAN_POINT ( 'NONE',  ( -10.81189881249999729, 6.242252689847871849, -192.7187500020483810 ) ) ;
#11366=CARTESIAN_POINT ( 'NONE',  ( -10.81189881249999729, 6.242252689847871849, -95.40625000204838102 ) ) ;
#11368=CARTESIAN_POINT ( 'NONE',  ( 5.000000000000000000, 8.660254037844385522, -80.12500000409677625 ) ) ;
#11369=CARTESIAN_POINT ( 'NONE',  ( 10.81189881249999907, 6.242252689847868297, -28.21875000204838102 ) ) ;
#11372=CARTESIAN_POINT ( 'NONE',  ( 10.81189881249999729, 0.000000000000000000, -25.53125000204836681 ) ) ;
#11375=CARTESIAN_POINT ( 'NONE',  ( -2.121150477449813534E-15, -11.54700538379251284, -5.750000004096755823 ) ) ;
#11379=CARTESIAN_POINT ( 'NONE',  ( 9.999999999999479527, 5.773502691896553074, -120.3749999999999716 ) ) ;
#11384=VERTEX_POINT ( 'NONE', #34804 ) ;
#11385=EDGE_CURVE ( 'NONE', #3574, #33493, #11972, .T. ) ;
#11391=LINE ( 'NONE', #7530, #18759 ) ;
#11392=CARTESIAN_POINT ( 'NONE',  ( -9.999999999999998224, 1.224646799147353059E-15, -113.7499999999999858 ) ) ;
#11394=CARTESIAN_POINT ( 'NONE',  ( -10.00000000000025580, 5.773502691896109873, -156.2500000040968189 ) ) ;
#11395=CARTESIAN_POINT ( 'NONE',  ( -10.81189881249999729, 6.242252689847871849, -164.4062500020484094 ) ) ;
#11398=CARTESIAN_POINT ( 'NONE',  ( 10.81189881249999551, -6.242252689847874514, -85.46875000204836681 ) ) ;
#11400=CARTESIAN_POINT ( 'NONE',  ( -10.81189881249999907, -6.242252689847864744, -195.4687500020484094 ) ) ;
#11401=CARTESIAN_POINT ( 'NONE',  ( -10.81189881249999729, 6.242252689847871849, -90.90625000204838102 ) ) ;
#11405=CARTESIAN_POINT ( 'NONE',  ( 7.644554776091147741E-16, 12.48450537969573659, -170.6562500020484094 ) ) ;
#11406=CARTESIAN_POINT ( 'NONE',  ( -2.293366432827344421E-15, -12.48450537969573659, -187.9062500020484094 ) ) ;
#11408=CARTESIAN_POINT ( 'NONE',  ( 9.999999999999998224, 0.000000000000000000, -174.8750000040967905 ) ) ;
#11410=CARTESIAN_POINT ( 'NONE',  ( 5.405949406249992428, -9.363379034771808662, -21.09375000204835615 ) ) ;
#11412=CARTESIAN_POINT ( 'NONE',  ( -10.81189881249999907, -6.242252689847864744, -124.9687500020483810 ) ) ;
#11414=CARTESIAN_POINT ( 'NONE',  ( -5.405949406249996869, 9.363379034771805109, -32.53125000204837391 ) ) ;
#11416=EDGE_CURVE ( 'NONE', #4599, #28346, #42594, .T. ) ;
#11418=CARTESIAN_POINT ( 'NONE',  ( -4.999999999999996447, 8.660254037844387298, -50.99999999999996447 ) ) ;
#11419=CARTESIAN_POINT ( 'NONE',  ( -5.405949406249996869, 9.363379034771805109, -121.0312500020483952 ) ) ;
#11422=CARTESIAN_POINT ( 'NONE',  ( -9.999999999999998224, 5.773502691896259087, -103.7500000040967620 ) ) ;
#11425=CARTESIAN_POINT ( 'NONE',  ( -5.405949406250003975, -9.363379034771801557, -57.34375000204835970 ) ) ;
#11430=DIRECTION ( 'NONE',  ( -0.000000000000000000, -0.000000000000000000, -1.000000000000000000 ) ) ;
#11431=CARTESIAN_POINT ( 'NONE',  ( 9.999999999999996447, -5.773502691896262640, -28.00000000409677625 ) ) ;
#11435=EDGE_CURVE ( 'NONE', #16951, #15509, #31569, .T. ) ;
#11436=CARTESIAN_POINT ( 'NONE',  ( -10.00000000000051337, 5.773502691895962435, -142.7500000040967905 ) ) ;
#11437=ORIENTED_EDGE ( 'NONE', *, *, #3272, .F. ) ;
#11438=ADVANCED_FACE ( 'NONE', ( #2001 ), #41675, .F. ) ;
#11441=ORIENTED_EDGE ( 'NONE', *, *, #18832, .T. ) ;
#11445=CARTESIAN_POINT ( 'NONE',  ( 10.81189881249999729, 0.000000000000000000, -186.0312500020484094 ) ) ;
#11451=CARTESIAN_POINT ( 'NONE',  ( 10.81189881249999729, 0.000000000000000000, -106.3437500020483810 ) ) ;
#11453=CARTESIAN_POINT ( 'NONE',  ( -5.405949406249996869, 9.363379034771805109, -115.0312500020483952 ) ) ;
#11455=CARTESIAN_POINT ( 'NONE',  ( -2.293366432827344421E-15, -12.48450537969573659, -129.2187500020483810 ) ) ;
#11457=CARTESIAN_POINT ( 'NONE',  ( -9.999999999999804601, 5.773502691896371886, -178.7500000040967905 ) ) ;
#11458=CARTESIAN_POINT ( 'NONE',  ( -9.999999999999998224, 1.224646799147353059E-15, -148.2500000000000000 ) ) ;
#11459=CARTESIAN_POINT ( 'NONE',  ( -9.999999999999998224, 1.224646799147353059E-15, -20.74999999999996447 ) ) ;
#11464=CARTESIAN_POINT ( 'NONE',  ( 10.81189881249999551, -6.242252689847874514, -47.96875000204836681 ) ) ;
#11466=CARTESIAN_POINT ( 'NONE',  ( 10.81189881249999907, 6.242252689847868297, -155.7187500020483810 ) ) ;
#11469=CARTESIAN_POINT ( 'NONE',  ( -9.999999999999998224, 1.224646799147353059E-15, -73.24999999999998579 ) ) ;
#11472=CARTESIAN_POINT ( 'NONE',  ( 10.81189881249999729, 6.242252689847867408, -103.4062500020483952 ) ) ;
#11473=CARTESIAN_POINT ( 'NONE',  ( -5.000000000000003553, -8.660254037844383745, -124.3750000040967763 ) ) ;
#11474=CARTESIAN_POINT ( 'NONE',  ( -9.999999999999612754, -5.773502691896474914, -154.5000000040967905 ) ) ;
#11475=CARTESIAN_POINT ( 'NONE',  ( -10.81189881249999729, 1.324075727343319199E-15, -81.59375000204838102 ) ) ;
#11478=CARTESIAN_POINT ( 'NONE',  ( 10.81189881249999907, 6.242252689847868297, -46.40625000204836681 ) ) ;
#11479=CARTESIAN_POINT ( 'NONE',  ( -5.000000000000003553, -8.660254037844383745, -137.5000000000000000 ) ) ;
#11487=ORIENTED_EDGE ( 'NONE', *, *, #13010, .F. ) ;
#11488=CARTESIAN_POINT ( 'NONE',  ( 7.070501591499376803E-16, 11.54700538379251284, -103.6249999999999858 ) ) ;
#11491=EDGE_CURVE ( 'NONE', #29774, #17140, #41207, .T. ) ;
#11493=CARTESIAN_POINT ( 'NONE',  ( 4.999999999999992006, -8.660254037844389075, -132.7499999999999716 ) ) ;
#11497=CARTESIAN_POINT ( 'NONE',  ( 5.405949406249999534, 9.363379034771803333, -143.5937500020483810 ) ) ;
#11498=CARTESIAN_POINT ( 'NONE',  ( 7.644554776091147741E-16, 12.48450537969573659, -148.1562500020484094 ) ) ;
#11499=( BOUNDED_CURVE ( )  B_SPLINE_CURVE ( 2, ( #39349, #39563, #23611, #9994, #29443, #23173, #36336 ),
 .UNSPECIFIED., .F., .F. ) 
 B_SPLINE_CURVE_WITH_KNOTS ( ( 3, 2, 2, 3 ),
 ( 0.1343283582089551953, 0.1355721393034825528, 0.1368159203980099381, 0.1380597014925373234 ),
 .UNSPECIFIED. ) 
 CURVE ( )  GEOMETRIC_REPRESENTATION_ITEM ( )  RATIONAL_B_SPLINE_CURVE ( ( 1.000000000000003109, 0.8660254037844358210, 1.000000000000000000, 0.8660254037844387076, 1.000000000000000000, 0.8660254037844387076, 1.000000000000000000 ) ) 
 REPRESENTATION_ITEM ( '' )  );
#11500=CARTESIAN_POINT ( 'NONE',  ( 7.644554776091147741E-16, 12.48450537969573659, -156.9687500020484094 ) ) ;
#11503=CARTESIAN_POINT ( 'NONE',  ( -5.000000000000003553, -8.660254037844383745, -172.0000000000000000 ) ) ;
#11507=CARTESIAN_POINT ( 'NONE',  ( -6.774270544292668284, -7.481437397228863695, -100.0000000000000142 ) ) ;
#11508=CARTESIAN_POINT ( 'NONE',  ( -10.81189881249999907, -6.242252689847864744, -181.9687500020484094 ) ) ;
#11512=CARTESIAN_POINT ( 'NONE',  ( -5.405949406249996869, 9.363379034771805109, -47.53125000204838813 ) ) ;
#11514=CARTESIAN_POINT ( 'NONE',  ( -10.00000000000000000, -5.773502691896251982, -103.1249999999999858 ) ) ;
#11515=ORIENTED_EDGE ( 'NONE', *, *, #37809, .F. ) ;
#11516=CARTESIAN_POINT ( 'NONE',  ( -10.81189881249999729, 1.324075727343319199E-15, -123.7812500020483952 ) ) ;
#11517=CARTESIAN_POINT ( 'NONE',  ( -4.999999999999996447, 8.660254037844387298, -148.8750000040967905 ) ) ;
#11521=CARTESIAN_POINT ( 'NONE',  ( 7.644554776091147741E-16, 12.48450537969573659, -176.4687500020483810 ) ) ;
#11525=CARTESIAN_POINT ( 'NONE',  ( -2.293366432827344421E-15, -12.48450537969573659, -69.40625000204838102 ) ) ;
#11527=CARTESIAN_POINT ( 'NONE',  ( -9.999999999999998224, 5.773502691896259087, -43.75000000409676204 ) ) ;
#11528=CARTESIAN_POINT ( 'NONE',  ( -5.405949406250003975, -9.363379034771801557, -1.843750002048366587 ) ) ;
#11536=ORIENTED_EDGE ( 'NONE', *, *, #4340, .F. ) ;
#11546=CARTESIAN_POINT ( 'NONE',  ( -9.999999999999998224, 5.773502691896259087, -38.87499999999997158 ) ) ;
#11548=CARTESIAN_POINT ( 'NONE',  ( -10.81189881249999729, 6.242252689847871849, -168.7187500020483810 ) ) ;
#11549=CARTESIAN_POINT ( 'NONE',  ( 10.81189881249999551, -6.242252689847874514, -178.4687500020484094 ) ) ;
#11551=CARTESIAN_POINT ( 'NONE',  ( -9.999999999999998224, 1.224646799147353059E-15, -168.1250000040967905 ) ) ;
#11552=CARTESIAN_POINT ( 'NONE',  ( -10.00000000000076916, 5.773502691895813221, -125.8749999999999858 ) ) ;
#11553=CARTESIAN_POINT ( 'NONE',  ( -9.999999999999998224, 5.773502691896259087, -194.8750000000000000 ) ) ;
#11560=CARTESIAN_POINT ( 'NONE',  ( -10.81189881249999907, -6.242252689847864744, -60.46875000204838102 ) ) ;
#11561=CARTESIAN_POINT ( 'NONE',  ( 10.81189881249999907, 6.242252689847868297, -70.40625000204839523 ) ) ;
#11563=CARTESIAN_POINT ( 'NONE',  ( -9.999999999999998224, 1.224646799147353059E-15, -133.2499999999999716 ) ) ;
#11565=CARTESIAN_POINT ( 'NONE',  ( 10.81189881249999551, -6.242252689847874514, -148.6562500020484094 ) ) ;
#11566=CARTESIAN_POINT ( 'NONE',  ( -5.405949406250003975, -9.363379034771801557, -162.5312500020484094 ) ) ;
#11569=CARTESIAN_POINT ( 'NONE',  ( -5.405949406250003975, -9.363379034771801557, -97.84375000204838102 ) ) ;
#11572=CARTESIAN_POINT ( 'NONE',  ( -2.293366432827344421E-15, -12.48450537969573659, -198.2187500020484379 ) ) ;
#11574=CARTESIAN_POINT ( 'NONE',  ( 4.999999999999992006, -8.660254037844389075, -133.1250000040967620 ) ) ;
#11575=CARTESIAN_POINT ( 'NONE',  ( -5.405949406249996869, 9.363379034771805109, -89.53125000204838102 ) ) ;
#11577=CARTESIAN_POINT ( 'NONE',  ( -9.999999999999998224, 1.224646799147353059E-15, -70.62500000409677625 ) ) ;
#11578=CARTESIAN_POINT ( 'NONE',  ( 5.405949406249999534, 9.363379034771803333, -29.59375000204836326 ) ) ;
#11581=CARTESIAN_POINT ( 'NONE',  ( 10.81189881249999907, 6.242252689847868297, -20.90625000204837747 ) ) ;
#11585=CARTESIAN_POINT ( 'NONE',  ( 9.999999999999996447, -5.773502691896262640, 0.4999999959032497276 ) ) ;
#11586=CARTESIAN_POINT ( 'NONE',  ( 0.000000000000000000, 0.000000000000000000, -99.99999999999998579 ) ) ;
#11591=ORIENTED_EDGE ( 'NONE', *, *, #13019, .T. ) ;
#11601=CARTESIAN_POINT ( 'NONE',  ( 5.000000000000000000, 8.660254037844385522, -114.2499999999999858 ) ) ;
#11603=CARTESIAN_POINT ( 'NONE',  ( -10.81189881249999907, -6.242252689847864744, -165.6562500020483810 ) ) ;
#11606=CARTESIAN_POINT ( 'NONE',  ( 10.81189881249999729, 0.000000000000000000, -82.34375000204836681 ) ) ;
#11608=CARTESIAN_POINT ( 'NONE',  ( -5.405949406249996869, 9.363379034771805109, -191.3437500020484094 ) ) ;
#11609=CARTESIAN_POINT ( 'NONE',  ( 5.405949406249999534, 9.363379034771803333, -94.28125000204838102 ) ) ;
#11613=CARTESIAN_POINT ( 'NONE',  ( -5.405949406250003975, -9.363379034771801557, -176.0312500020483810 ) ) ;
#11614=CARTESIAN_POINT ( 'NONE',  ( 10.81189881249999551, -6.242252689847874514, -190.6562500020484094 ) ) ;
#11616=CARTESIAN_POINT ( 'NONE',  ( -10.00000000000000000, -5.773502691896251982, -163.5000000040967620 ) ) ;
#11618=CARTESIAN_POINT ( 'NONE',  ( 10.81189881249999907, 6.242252689847868297, -10.21875000204835970 ) ) ;
#11620=CARTESIAN_POINT ( 'NONE',  ( -10.81189881249999729, 1.324075727343319199E-15, -125.0937500020483668 ) ) ;
#11623=CARTESIAN_POINT ( 'NONE',  ( -5.405949406250003975, -9.363379034771801557, -21.53125000204836326 ) ) ;
#11626=EDGE_CURVE ( 'NONE', #31885, #25488, #39502, .T. ) ;
#11627=CARTESIAN_POINT ( 'NONE',  ( 4.999999999999992006, -8.660254037844389075, -54.74999999999996447 ) ) ;
#11628=CARTESIAN_POINT ( 'NONE',  ( 10.81189881249999551, -6.242252689847874514, -118.6562500020483952 ) ) ;
#11631=CARTESIAN_POINT ( 'NONE',  ( 7.070501591499377789E-16, 11.54700538379251284, -90.50000000409677625 ) ) ;
#11634=CARTESIAN_POINT ( 'NONE',  ( 5.405949406249992428, -9.363379034771808662, -46.59375000204838102 ) ) ;
#11641=CARTESIAN_POINT ( 'NONE',  ( 5.000000000000000000, 8.660254037844385522, -26.12500000409675849 ) ) ;
#11642=( BOUNDED_CURVE ( )  B_SPLINE_CURVE ( 2, ( #13562, #14413, #17231, #4509, #656, #27391, #10971 ),
 .UNSPECIFIED., .F., .F. ) 
 B_SPLINE_CURVE_WITH_KNOTS ( ( 3, 2, 2, 3 ),
 ( 0.2238805970149254365, 0.2251243781094527940, 0.2263681592039801793, 0.2276119402985075368 ),
 .UNSPECIFIED. ) 
 CURVE ( )  GEOMETRIC_REPRESENTATION_ITEM ( )  RATIONAL_B_SPLINE_CURVE ( ( 0.9999999999999940048, 0.8660254037844447028, 1.000000000000000000, 0.8660254037844387076, 1.000000000000000000, 0.8660254037844297148, 1.000000000000008882 ) ) 
 REPRESENTATION_ITEM ( '' )  );
#11644=DIRECTION ( 'NONE',  ( -1.000000000000000000, 0.000000000000000000, 0.000000000000000000 ) ) ;
#11648=ORIENTED_EDGE ( 'NONE', *, *, #19041, .T. ) ;
#11655=DIRECTION ( 'NONE',  ( -1.000000000000000000, 0.000000000000000000, 0.000000000000000000 ) ) ;
#11657=CARTESIAN_POINT ( 'NONE',  ( 10.81189881249999729, 0.000000000000000000, -190.5312500020484094 ) ) ;
#11659=VECTOR ( 'NONE', #2912, 1000.000000000000000 ) ;
#11662=CARTESIAN_POINT ( 'NONE',  ( -2.293366432827344421E-15, -12.48450537969573659, -112.7187500020483952 ) ) ;
#11664=CARTESIAN_POINT ( 'NONE',  ( -10.81189881249999907, -6.242252689847864744, -113.1562500020483952 ) ) ;
#11666=CARTESIAN_POINT ( 'NONE',  ( -5.405949406250003975, -9.363379034771801557, -127.8437500020483952 ) ) ;
#11668=AXIS2_PLACEMENT_3D ( 'NONE', #27937, #34421, #14744 ) ;
#11669=DIRECTION ( 'NONE',  ( -0.000000000000000000, -0.000000000000000000, -1.000000000000000000 ) ) ;
#11670=CARTESIAN_POINT ( 'NONE',  ( -9.999999999999998224, 1.224646799147353059E-15, -149.7500000000000000 ) ) ;
#11671=CARTESIAN_POINT ( 'NONE',  ( 5.000000000000000000, 8.660254037844385522, -10.74999999999995381 ) ) ;
#11674=CARTESIAN_POINT ( 'NONE',  ( 7.070501591499377789E-16, 11.54700538379251284, -188.0000000040967905 ) ) ;
#11676=CARTESIAN_POINT ( 'NONE',  ( 7.644554776091147741E-16, 12.48450537969573659, -38.46875000204835260 ) ) ;
#11678=CARTESIAN_POINT ( 'NONE',  ( -5.405949406250003975, -9.363379034771801557, -145.8437500020483810 ) ) ;
#11684=CARTESIAN_POINT ( 'NONE',  ( -4.999999999999996447, 8.660254037844387298, -71.99999999999998579 ) ) ;
#11685=CARTESIAN_POINT ( 'NONE',  ( -10.81189881249999729, 1.324075727343319199E-15, -141.7812500020483810 ) ) ;
#11687=EDGE_CURVE ( 'NONE', #22477, #23032, #14990, .T. ) ;
#11689=CARTESIAN_POINT ( 'NONE',  ( -5.000000000000003553, -8.660254037844383745, -164.5000000000000000 ) ) ;
#11690=CARTESIAN_POINT ( 'NONE',  ( 9.999999999999998224, 0.000000000000000000, -122.3750000040967905 ) ) ;
#11692=CARTESIAN_POINT ( 'NONE',  ( -10.81189881249999729, 1.324075727343319199E-15, -75.59375000204838102 ) ) ;
#11696=CARTESIAN_POINT ( 'NONE',  ( 10.81189881249999907, 6.242252689847868297, -41.90625000204836681 ) ) ;
#11701=ADVANCED_FACE ( 'NONE', ( #16389 ), #36274, .F. ) ;
#11703=ORIENTED_EDGE ( 'NONE', *, *, #16335, .F. ) ;
#11706=ORIENTED_EDGE ( 'NONE', *, *, #26481, .F. ) ;
#11715=CARTESIAN_POINT ( 'NONE',  ( -10.81189881249999729, 6.242252689847871849, -132.7187500020483810 ) ) ;
#11716=CARTESIAN_POINT ( 'NONE',  ( -10.81189881249999729, 1.324075727343319199E-15, -143.2812500020483810 ) ) ;
#11717=CARTESIAN_POINT ( 'NONE',  ( -2.293366432827344421E-15, -12.48450537969573659, -157.7187500020483810 ) ) ;
#11720=CARTESIAN_POINT ( 'NONE',  ( -10.00000000000000000, -5.773502691896251982, -169.1249999999999716 ) ) ;
#11725=CARTESIAN_POINT ( 'NONE',  ( 4.999999999999992006, -8.660254037844389075, -149.2500000000000000 ) ) ;
#11726=CARTESIAN_POINT ( 'NONE',  ( -10.81189881249999907, -6.242252689847864744, -171.4687500020484094 ) ) ;
#11730=CARTESIAN_POINT ( 'NONE',  ( -2.293366432827344421E-15, -12.48450537969573659, -43.90625000204837391 ) ) ;
#11732=CARTESIAN_POINT ( 'NONE',  ( -5.000000000000003553, -8.660254037844383745, -96.99999999999998579 ) ) ;
#11734=CARTESIAN_POINT ( 'NONE',  ( -5.405949406250003975, -9.363379034771801557, -128.0312500020484094 ) ) ;
#11735=CARTESIAN_POINT ( 'NONE',  ( 9.999999999999996447, -5.773502691896262640, -149.5000000040968189 ) ) ;
#11738=EDGE_LOOP ( 'NONE', ( #26943, #20253, #18571, #13600 ) ) ;
#11739=CARTESIAN_POINT ( 'NONE',  ( 5.405949406249992428, -9.363379034771808662, -171.0937500020484094 ) ) ;
#11742=CARTESIAN_POINT ( 'NONE',  ( -9.999999999999998224, 1.224646799147353059E-15, -134.7499999999999716 ) ) ;
#11743=CARTESIAN_POINT ( 'NONE',  ( -5.405949406249996869, 9.363379034771805109, -67.03125000204838102 ) ) ;
#11744=CARTESIAN_POINT ( 'NONE',  ( 9.999999999999998224, 0.000000000000000000, -41.37500000409677625 ) ) ;
#11745=CARTESIAN_POINT ( 'NONE',  ( 7.644554776091147741E-16, 12.48450537969573659, -5.468750002048355263 ) ) ;
#11748=EDGE_CURVE ( 'NONE', #33393, #28805, #32427, .T. ) ;
#11758=VERTEX_POINT ( 'NONE', #20709 ) ;
#11766=DIRECTION ( 'NONE',  ( -0.000000000000000000, -0.000000000000000000, -1.000000000000000000 ) ) ;
#11767=CARTESIAN_POINT ( 'NONE',  ( -9.999999999999998224, 1.224646799147353059E-15, -40.24999999999997868 ) ) ;
#11770=CARTESIAN_POINT ( 'NONE',  ( -10.81189881249999729, 1.324075727343319199E-15, -155.0937500020483810 ) ) ;
#11771=CARTESIAN_POINT ( 'NONE',  ( 7.644554776091147741E-16, 12.48450537969573659, -177.9687500020484094 ) ) ;
#11773=DIRECTION ( 'NONE',  ( -0.000000000000000000, -0.000000000000000000, -1.000000000000000000 ) ) ;
#11774=CARTESIAN_POINT ( 'NONE',  ( -9.999999999999998224, 5.773502691896259087, -191.8750000000000000 ) ) ;
#11776=CARTESIAN_POINT ( 'NONE',  ( -9.999999999999998224, 1.224646799147353059E-15, -100.6250000040967905 ) ) ;
#11779=CARTESIAN_POINT ( 'NONE',  ( 7.644554776091147741E-16, 12.48450537969573659, -67.15625000204838102 ) ) ;
#11781=CARTESIAN_POINT ( 'NONE',  ( -9.999999999999998224, 5.773502691896259087, -124.3750000000000000 ) ) ;
#11782=AXIS2_PLACEMENT_3D ( 'NONE', #21034, #10251, #16720 ) ;
#11783=CARTESIAN_POINT ( 'NONE',  ( 5.405949406249999534, 9.363379034771803333, -146.7812500020483810 ) ) ;
#11784=CARTESIAN_POINT ( 'NONE',  ( 10.81189881249999551, -6.242252689847874514, -168.1562500020484094 ) ) ;
#11787=CARTESIAN_POINT ( 'NONE',  ( 5.405949406249992428, -9.363379034771808662, -97.59375000204838102 ) ) ;
#11790=CARTESIAN_POINT ( 'NONE',  ( -2.293366432827344421E-15, -12.48450537969573659, -195.2187500020484094 ) ) ;
#11792=CARTESIAN_POINT ( 'NONE',  ( 7.099235607825172600, -8.054141481624315091, -180.0000000000000000 ) ) ;
#11793=CARTESIAN_POINT ( 'NONE',  ( 9.999999999999998224, 0.000000000000000000, -137.3750000040967905 ) ) ;
#11794=CARTESIAN_POINT ( 'NONE',  ( -5.405949406250003975, -9.363379034771801557, -93.53125000204838102 ) ) ;
#11796=CARTESIAN_POINT ( 'NONE',  ( -4.999999999999996447, 8.660254037844387298, -66.37500000409676204 ) ) ;
#11798=CARTESIAN_POINT ( 'NONE',  ( -10.81189881249999729, 1.324075727343319199E-15, -24.59375000204835970 ) ) ;
#11799=ORIENTED_EDGE ( 'NONE', *, *, #34413, .T. ) ;
#11802=CARTESIAN_POINT ( 'NONE',  ( 10.81189881249999551, -6.242252689847874514, -21.15625000204837391 ) ) ;
#11812=ORIENTED_EDGE ( 'NONE', *, *, #29149, .F. ) ;
#11819=CARTESIAN_POINT ( 'NONE',  ( -9.999999999999998224, 0.000000000000000000, -99.99999999999998579 ) ) ;
#11822=CARTESIAN_POINT ( 'NONE',  ( 5.405949406249992428, -9.363379034771808662, -162.2812500020484094 ) ) ;
#11823=AXIS2_PLACEMENT_3D ( 'NONE', #41216, #8660, #11655 ) ;
#11826=CARTESIAN_POINT ( 'NONE',  ( 10.81189881249999729, 0.000000000000000000, -83.84375000204836681 ) ) ;
#11828=CARTESIAN_POINT ( 'NONE',  ( 10.81189881249999907, 6.242252689847868297, -190.2187500020484094 ) ) ;
#11829=CARTESIAN_POINT ( 'NONE',  ( 10.81189881249999729, 0.000000000000000000, -93.03125000204838102 ) ) ;
#11833=CARTESIAN_POINT ( 'NONE',  ( 10.81189881249999729, 0.000000000000000000, -174.0312500020484094 ) ) ;
#11834=CARTESIAN_POINT ( 'NONE',  ( 5.405949406249992428, -9.363379034771808662, -186.2812500020484094 ) ) ;
#11836=CARTESIAN_POINT ( 'NONE',  ( -4.999999999999996447, 8.660254037844387298, -160.8750000040967905 ) ) ;
#11838=CARTESIAN_POINT ( 'NONE',  ( 5.405949406249992428, -9.363379034771808662, -15.09375000204835082 ) ) ;
#11840=CARTESIAN_POINT ( 'NONE',  ( 10.81189881249999729, 0.000000000000000000, -119.8437500020483810 ) ) ;
#11842=CARTESIAN_POINT ( 'NONE',  ( 5.405949406249992428, -9.363379034771808662, -21.28125000204836326 ) ) ;
#11845=CARTESIAN_POINT ( 'NONE',  ( 9.999999999999998224, 0.000000000000000000, -54.49999999999996447 ) ) ;
#11846=CARTESIAN_POINT ( 'NONE',  ( 5.405949406249992428, -9.363379034771808662, -117.2812500020483952 ) ) ;
#11851=CARTESIAN_POINT ( 'NONE',  ( -5.000000000000003553, -8.660254037844383745, -94.37500000409677625 ) ) ;
#11854=CARTESIAN_POINT ( 'NONE',  ( 7.644554776091147741E-16, 12.48450537969573659, -48.96875000204836681 ) ) ;
#11861=CARTESIAN_POINT ( 'NONE',  ( 9.999999999999996447, -5.773502691896262640, -23.50000000409677270 ) ) ;
#11862=CARTESIAN_POINT ( 'NONE',  ( -10.00000000000012434, 5.773502691896184480, -167.8749999999999716 ) ) ;
#11865=LINE ( 'NONE', #18563, #18308 ) ;
#11876=CARTESIAN_POINT ( 'NONE',  ( 7.644554776091147741E-16, 12.48450537969573659, -185.6562500020484094 ) ) ;
#11880=CARTESIAN_POINT ( 'NONE',  ( -10.81189881249999729, 1.324075727343319199E-15, -111.5937500020483810 ) ) ;
#11881=CARTESIAN_POINT ( 'NONE',  ( -9.999999999999479527, -5.773502691896549521, -150.0000000040967905 ) ) ;
#11882=CARTESIAN_POINT ( 'NONE',  ( 10.81189881249999551, -6.242252689847874514, -117.1562500020483810 ) ) ;
#11884=CARTESIAN_POINT ( 'NONE',  ( 10.81189881249999551, -6.242252689847874514, -125.9687500020483810 ) ) ;
#11887=CARTESIAN_POINT ( 'NONE',  ( -4.999999999999996447, 8.660254037844387298, -147.0000000000000000 ) ) ;
#11888=CARTESIAN_POINT ( 'NONE',  ( 7.070501591499377789E-16, 11.54700538379251284, -9.124999999999966249 ) ) ;
#11889=AXIS2_PLACEMENT_3D ( 'NONE', #20130, #33318, #24459 ) ;
#11892=CARTESIAN_POINT ( 'NONE',  ( -2.121150477449813534E-15, -11.54700538379251284, -185.7500000040967905 ) ) ;
#11894=CARTESIAN_POINT ( 'NONE',  ( 5.405949406249999534, 9.363379034771803333, -40.09375000204837391 ) ) ;
#11895=CARTESIAN_POINT ( 'NONE',  ( -5.000000000000003553, -8.660254037844383745, -163.3750000040967905 ) ) ;
#11896=CARTESIAN_POINT ( 'NONE',  ( -10.81189881249999729, 6.242252689847871849, -143.2187500020484094 ) ) ;
#11898=CARTESIAN_POINT ( 'NONE',  ( -10.00000000000000000, -5.773502691896251982, -71.62500000000000000 ) ) ;
#11899=CARTESIAN_POINT ( 'NONE',  ( 5.405949406249999534, 9.363379034771803333, -142.2812500020483810 ) ) ;
#11903=CARTESIAN_POINT ( 'NONE',  ( -10.81189881249999729, 1.324075727343319199E-15, -105.7812500020483810 ) ) ;
#11904=CARTESIAN_POINT ( 'NONE',  ( 5.000000000000000000, 8.660254037844385522, -113.1250000040967763 ) ) ;
#11905=CARTESIAN_POINT ( 'NONE',  ( 4.999999999999992006, -8.660254037844389075, -140.2500000000000000 ) ) ;
#11906=CARTESIAN_POINT ( 'NONE',  ( 5.405949406249992428, -9.363379034771808662, -73.59375000204838102 ) ) ;
#11909=CARTESIAN_POINT ( 'NONE',  ( -5.405949406250003975, -9.363379034771801557, -44.03125000204838102 ) ) ;
#11910=( BOUNDED_CURVE ( )  B_SPLINE_CURVE ( 2, ( #26779, #40142, #29815, #256, #13377, #19654, #26569 ),
 .UNSPECIFIED., .F., .F. ) 
 B_SPLINE_CURVE_WITH_KNOTS ( ( 3, 2, 2, 3 ),
 ( 0.2649253731343284568, 0.2661691542288558421, 0.2674129353233831718, 0.2686567164179105571 ),
 .UNSPECIFIED. ) 
 CURVE ( )  GEOMETRIC_REPRESENTATION_ITEM ( )  RATIONAL_B_SPLINE_CURVE ( ( 0.9999999999999880096, 0.8660254037844506980, 1.000000000000000000, 0.8660254037844387076, 1.000000000000000000, 0.8660254037844267172, 1.000000000000011990 ) ) 
 REPRESENTATION_ITEM ( '' )  );
#11930=CARTESIAN_POINT ( 'NONE',  ( -10.81189881249999907, -6.242252689847864744, -133.9687500020483810 ) ) ;
#11931=CARTESIAN_POINT ( 'NONE',  ( 7.644554776091147741E-16, 12.48450537969573659, -140.6562500020484094 ) ) ;
#11932=CARTESIAN_POINT ( 'NONE',  ( 5.405949406249992428, -9.363379034771808662, -144.0937500020483810 ) ) ;
#11935=CARTESIAN_POINT ( 'NONE',  ( 4.999999999999992006, -8.660254037844389075, -171.7500000000000000 ) ) ;
#11937=CARTESIAN_POINT ( 'NONE',  ( 9.999999999999998224, 0.000000000000000000, -128.3750000040967905 ) ) ;
#11939=CARTESIAN_POINT ( 'NONE',  ( -8.268648510919758721, -5.984980119022559109, -100.0000000000000142 ) ) ;
#11940=CARTESIAN_POINT ( 'NONE',  ( -2.293366432827344421E-15, -12.48450537969573659, -166.7187500020484094 ) ) ;
#11945=CARTESIAN_POINT ( 'NONE',  ( 10.81189881249999907, 6.242252689847868297, -46.40625000204836681 ) ) ;
#11947=CARTESIAN_POINT ( 'NONE',  ( -10.00000000000000000, -5.773502691896251982, -101.6249999999999858 ) ) ;
#11949=CARTESIAN_POINT ( 'NONE',  ( -10.81189881249999729, -6.242252689847864744, -123.6562500020484094 ) ) ;
#11950=CARTESIAN_POINT ( 'NONE',  ( 7.070501591499377789E-16, 11.54700538379251284, -138.5000000040967905 ) ) ;
#11954=CARTESIAN_POINT ( 'NONE',  ( 5.405949406249992428, -9.363379034771808662, -172.5937500020484094 ) ) ;
#11956=EDGE_CURVE ( 'NONE', #19459, #36911, #24994, .T. ) ;
#11957=CARTESIAN_POINT ( 'NONE',  ( -9.999999999999998224, 1.224646799147353059E-15, -155.7500000000000000 ) ) ;
#11958=CARTESIAN_POINT ( 'NONE',  ( -5.405949406249996869, 9.363379034771805109, -65.53125000204838102 ) ) ;
#11959=CARTESIAN_POINT ( 'NONE',  ( -2.121150477449813534E-15, -11.54700538379251284, -46.25000000409676204 ) ) ;
#11972=( BOUNDED_CURVE ( )  B_SPLINE_CURVE ( 2, ( #28756, #41883, #19019, #35228, #1785, #21626, #5659 ),
 .UNSPECIFIED., .F., .F. ) 
 B_SPLINE_CURVE_WITH_KNOTS ( ( 3, 2, 2, 3 ),
 ( 0.4813432835820896649, 0.4825870646766170502, 0.4838308457711443800, 0.4850746268656717652 ),
 .UNSPECIFIED. ) 
 CURVE ( )  GEOMETRIC_REPRESENTATION_ITEM ( )  RATIONAL_B_SPLINE_CURVE ( ( 0.9999999999999880096, 0.8660254037844506980, 1.000000000000000000, 0.8660254037844387076, 1.000000000000000000, 0.8660254037844267172, 1.000000000000011990 ) ) 
 REPRESENTATION_ITEM ( '' )  );
#11974=EDGE_CURVE ( 'NONE', #17462, #21319, #22214, .T. ) ;
#11976=CARTESIAN_POINT ( 'NONE',  ( 9.999999999999998224, 1.224646799147353059E-15, -99.99999999999998579 ) ) ;
#11981=CARTESIAN_POINT ( 'NONE',  ( 9.999999999999998224, 0.000000000000000000, -112.9999999999999858 ) ) ;
#11982=CARTESIAN_POINT ( 'NONE',  ( -5.000000000000003553, -8.660254037844383745, -33.99999999999997158 ) ) ;
#11986=CARTESIAN_POINT ( 'NONE',  ( -5.405949406250003975, -9.363379034771801557, -154.8437500020483810 ) ) ;
#11987=CARTESIAN_POINT ( 'NONE',  ( -10.81189881249999729, -6.242252689847864744, -177.4687500020484094 ) ) ;
#11990=CARTESIAN_POINT ( 'NONE',  ( -10.00000000000000000, -5.773502691896251982, -197.6250000000000284 ) ) ;
#11995=CARTESIAN_POINT ( 'NONE',  ( 7.644554776091147741E-16, 12.48450537969573659, -65.65625000204838102 ) ) ;
#11997=CARTESIAN_POINT ( 'NONE',  ( 9.999999999999998224, 0.000000000000000000, -125.0000000000000000 ) ) ;
#11998=EDGE_CURVE ( 'NONE', #17213, #37997, #16361, .T. ) ;
#12000=CARTESIAN_POINT ( 'NONE',  ( -5.405949406250003975, -9.363379034771801557, -153.5312500020484094 ) ) ;
#12001=CARTESIAN_POINT ( 'NONE',  ( -10.81189881249999907, -6.242252689847864744, -164.1562500020484094 ) ) ;
#12004=CARTESIAN_POINT ( 'NONE',  ( -5.405949406249996869, 9.363379034771805109, -101.3437500020483810 ) ) ;
#12007=CARTESIAN_POINT ( 'NONE',  ( 5.405949406249992428, -9.363379034771808662, -0.2812500020483721386 ) ) ;
#12010=CARTESIAN_POINT ( 'NONE',  ( 10.81189881249999551, -6.242252689847874514, -96.15625000204838102 ) ) ;
#12012=CARTESIAN_POINT ( 'NONE',  ( 9.999999999999996447, -5.773502691896262640, -70.00000000409679046 ) ) ;
#12013=LINE ( 'NONE', #22168, #35576 ) ;
#12014=CARTESIAN_POINT ( 'NONE',  ( 7.644554776091147741E-16, 12.48450537969573659, -24.96875000204837391 ) ) ;
#12017=CARTESIAN_POINT ( 'NONE',  ( -10.81189881249999729, 1.324075727343319199E-15, -17.28125000204835970 ) ) ;
#12019=CARTESIAN_POINT ( 'NONE',  ( 7.070501591499376803E-16, 11.54700538379251284, -137.0000000040967905 ) ) ;
#12021=CARTESIAN_POINT ( 'NONE',  ( 10.00000000000000000, 5.773502691896255534, 0.7499999959032500607 ) ) ;
#12037=CARTESIAN_POINT ( 'NONE',  ( -5.405949406249996869, 9.363379034771805109, -166.0312500020484094 ) ) ;
#12042=CARTESIAN_POINT ( 'NONE',  ( -5.405949406250003975, -9.363379034771801557, -88.84375000204838102 ) ) ;
#12043=CARTESIAN_POINT ( 'NONE',  ( 5.405949406249999534, 9.363379034771803333, -196.0937500020484094 ) ) ;
#12044=CARTESIAN_POINT ( 'NONE',  ( -5.405949406250003975, -9.363379034771801557, -90.53125000204838102 ) ) ;
#12047=CARTESIAN_POINT ( 'NONE',  ( -9.999999999999479527, -5.773502691896549521, -151.1250000000000000 ) ) ;
#12048=CARTESIAN_POINT ( 'NONE',  ( 7.644554776091147741E-16, 12.48450537969573659, -172.1562500020484094 ) ) ;
#12049=CARTESIAN_POINT ( 'NONE',  ( 10.81189881249999551, -6.242252689847874514, -186.1562500020484379 ) ) ;
#12051=CARTESIAN_POINT ( 'NONE',  ( 5.000000000000000000, 8.660254037844385522, -167.1250000040967905 ) ) ;
#12053=CARTESIAN_POINT ( 'NONE',  ( -2.293366432827344421E-15, -12.48450537969573659, -12.21875000204836148 ) ) ;
#12055=CARTESIAN_POINT ( 'NONE',  ( -10.81189881249999907, -6.242252689847864744, -123.4687500020483810 ) ) ;
#12057=CARTESIAN_POINT ( 'NONE',  ( -5.405949406250003975, -9.363379034771801557, -24.53125000204836681 ) ) ;
#12059=DIRECTION ( 'NONE',  ( -0.000000000000000000, -0.000000000000000000, -1.000000000000000000 ) ) ;
#12060=CARTESIAN_POINT ( 'NONE',  ( -10.81189881249999907, -6.242252689847864744, -117.6562500020483952 ) ) ;
#12063=ORIENTED_EDGE ( 'NONE', *, *, #7526, .F. ) ;
#12065=CARTESIAN_POINT ( 'NONE',  ( -4.999999999999996447, 8.660254037844387298, -88.87500000409677625 ) ) ;
#12068=CARTESIAN_POINT ( 'NONE',  ( -10.81189881249999907, -6.242252689847864744, -49.96875000204837391 ) ) ;
#12073=CARTESIAN_POINT ( 'NONE',  ( -9.999999999999998224, 1.224646799147353059E-15, -18.12500000409675138 ) ) ;
#12078=CARTESIAN_POINT ( 'NONE',  ( 9.999999999999998224, 1.224646799147353059E-15, -99.99999999999998579 ) ) ;
#12080=ORIENTED_EDGE ( 'NONE', *, *, #34162, .T. ) ;
#12084=ORIENTED_EDGE ( 'NONE', *, *, #8000, .T. ) ;
#12087=DIRECTION ( 'NONE',  ( -0.000000000000000000, -0.000000000000000000, -1.000000000000000000 ) ) ;
#12091=CARTESIAN_POINT ( 'NONE',  ( 10.81189881249999729, 0.000000000000000000, -192.0312500020484094 ) ) ;
#12094=CARTESIAN_POINT ( 'NONE',  ( 10.81189881249999551, -6.242252689847874514, -110.9687500020483810 ) ) ;
#12096=CARTESIAN_POINT ( 'NONE',  ( -10.81189881249999907, -6.242252689847864744, -114.6562500020483952 ) ) ;
#12098=CARTESIAN_POINT ( 'NONE',  ( -2.293366432827344421E-15, -12.48450537969573659, -126.2187500020483952 ) ) ;
#12100=CARTESIAN_POINT ( 'NONE',  ( -4.999999999999996447, 8.660254037844387298, -144.0000000000000000 ) ) ;
#12101=CARTESIAN_POINT ( 'NONE',  ( -9.999999999999998224, 1.224646799147353059E-15, -8.749999999999952038 ) ) ;
#12104=CARTESIAN_POINT ( 'NONE',  ( -4.999999999999996447, 8.660254037844387298, -190.8750000040967905 ) ) ;
#12106=CARTESIAN_POINT ( 'NONE',  ( 5.405949406249992428, -9.363379034771808662, -40.59375000204837391 ) ) ;
#12108=CARTESIAN_POINT ( 'NONE',  ( 10.81189881249999907, 6.242252689847868297, -142.2187500020484094 ) ) ;
#12110=ADVANCED_FACE ( 'NONE', ( #8631 ), #28493, .F. ) ;
#12113=CARTESIAN_POINT ( 'NONE',  ( 4.999999999999992006, -8.660254037844389075, -78.74999999999998579 ) ) ;
#12114=CARTESIAN_POINT ( 'NONE',  ( 10.81189881249999907, 6.242252689847868297, -140.9062500020484094 ) ) ;
#12119=CARTESIAN_POINT ( 'NONE',  ( 7.070501591499377789E-16, 11.54700538379251284, -116.0000000040967763 ) ) ;
#12121=CARTESIAN_POINT ( 'NONE',  ( 5.405949406249992428, -9.363379034771808662, -76.59375000204838102 ) ) ;
#12124=VECTOR ( 'NONE', #20301, 1000.000000000000000 ) ;
#12126=CARTESIAN_POINT ( 'NONE',  ( 5.405949406249992428, -9.363379034771808662, -37.78125000204838102 ) ) ;
#12142=CARTESIAN_POINT ( 'NONE',  ( 10.81189881249999551, -6.242252689847874514, -130.4687500020483810 ) ) ;
#12143=CARTESIAN_POINT ( 'NONE',  ( -5.405949406250003975, -9.363379034771801557, -137.0312500020484094 ) ) ;
#12144=CARTESIAN_POINT ( 'NONE',  ( 5.405949406249999534, 9.363379034771803333, -146.5937500020483810 ) ) ;
#12147=CARTESIAN_POINT ( 'NONE',  ( -9.999999999999998224, 5.773502691896259087, -173.8749999999999716 ) ) ;
#12149=CARTESIAN_POINT ( 'NONE',  ( -0.06394991864857380026, 10.83468475260746544, -100.0000000000000142 ) ) ;
#12151=CARTESIAN_POINT ( 'NONE',  ( -2.121150477449813534E-15, -11.54700538379251284, -149.3750000000000000 ) ) ;
#12152=CARTESIAN_POINT ( 'NONE',  ( 10.81189881249999729, 0.000000000000000000, -166.3437500020484094 ) ) ;
#12156=CARTESIAN_POINT ( 'NONE',  ( -10.81189881249999729, 1.324075727343319199E-15, -39.78125000204838102 ) ) ;
#12158=CARTESIAN_POINT ( 'NONE',  ( 10.00000000000000000, 5.773502691896255534, -100.8750000000000000 ) ) ;
#12160=( BOUNDED_CURVE ( )  B_SPLINE_CURVE ( 2, ( #18875, #2691, #31850, #35505, #25363, #18226, #35078 ),
 .UNSPECIFIED., .F., .F. ) 
 B_SPLINE_CURVE_WITH_KNOTS ( ( 3, 2, 2, 3 ),
 ( 0.1828358208955224162, 0.1840796019900497738, 0.1853233830845771313, 0.1865671641791045166 ),
 .UNSPECIFIED. ) 
 CURVE ( )  GEOMETRIC_REPRESENTATION_ITEM ( )  RATIONAL_B_SPLINE_CURVE ( ( 0.9999999999999970024, 0.8660254037844417052, 1.000000000000000000, 0.8660254037844387076, 1.000000000000000000, 0.8660254037844357100, 1.000000000000002887 ) ) 
 REPRESENTATION_ITEM ( '' )  );
#12161=CARTESIAN_POINT ( 'NONE',  ( -5.405949406249996869, 9.363379034771805109, -116.5312500020483952 ) ) ;
#12162=CARTESIAN_POINT ( 'NONE',  ( 9.999999999999998224, 0.000000000000000000, -140.3750000040967905 ) ) ;
#12163=CARTESIAN_POINT ( 'NONE',  ( 7.070501591499376803E-16, 11.54700538379251284, -159.1250000000000284 ) ) ;
#12167=CARTESIAN_POINT ( 'NONE',  ( 9.999999999999998224, 0.000000000000000000, -174.8750000040967905 ) ) ;
#12169=CARTESIAN_POINT ( 'NONE',  ( -10.81189881249999729, 6.242252689847871849, -69.90625000204839523 ) ) ;
#12190=CARTESIAN_POINT ( 'NONE',  ( 9.999999999999998224, 0.000000000000000000, -33.49999999999997158 ) ) ;
#12193=CARTESIAN_POINT ( 'NONE',  ( 10.81189881249999907, 6.242252689847868297, -158.7187500020483810 ) ) ;
#12194=CARTESIAN_POINT ( 'NONE',  ( -10.81189881249999729, 1.324075727343319199E-15, -170.0937500020484094 ) ) ;
#12197=CARTESIAN_POINT ( 'NONE',  ( -9.999999999999998224, 1.224646799147353059E-15, -199.2500000000000000 ) ) ;
#12202=CARTESIAN_POINT ( 'NONE',  ( -10.81189881249999907, -6.242252689847864744, -63.65625000204838102 ) ) ;
#12204=CARTESIAN_POINT ( 'NONE',  ( -2.121150477449813534E-15, -11.54700538379251284, -120.8749999999999858 ) ) ;
#12206=CARTESIAN_POINT ( 'NONE',  ( -10.81189881249999729, 1.324075727343319199E-15, -149.2812500020483810 ) ) ;
#12207=CARTESIAN_POINT ( 'NONE',  ( -10.81189881249999729, 6.242252689847871849, -161.4062500020483810 ) ) ;
#12210=CARTESIAN_POINT ( 'NONE',  ( -5.405949406250003975, -9.363379034771801557, -99.34375000204838102 ) ) ;
#12213=CARTESIAN_POINT ( 'NONE',  ( -5.405949406250003975, -9.363379034771801557, -195.3437500020484094 ) ) ;
#12217=CARTESIAN_POINT ( 'NONE',  ( 10.00000000000051159, -5.773502691895965988, -144.6250000000000000 ) ) ;
#12218=CARTESIAN_POINT ( 'NONE',  ( -10.81189881249999907, -6.242252689847864744, -89.15625000204839523 ) ) ;
#12221=CARTESIAN_POINT ( 'NONE',  ( -5.000000000000003553, -8.660254037844383745, -68.87500000409677625 ) ) ;
#12223=CARTESIAN_POINT ( 'NONE',  ( -10.81189881249999729, 6.242252689847871849, -24.71875000204837391 ) ) ;
#12226=CARTESIAN_POINT ( 'NONE',  ( 10.81189881249999729, 0.000000000000000000, -24.03125000204836681 ) ) ;
#12236=CARTESIAN_POINT ( 'NONE',  ( -9.999999999999998224, 1.224646799147353059E-15, -155.7500000000000000 ) ) ;
#12237=ORIENTED_EDGE ( 'NONE', *, *, #9328, .T. ) ;
#12247=CARTESIAN_POINT ( 'NONE',  ( 10.00000000000051159, -5.773502691895965988, -127.0000000040967763 ) ) ;
#12249=CARTESIAN_POINT ( 'NONE',  ( 10.81189881249999907, 6.242252689847868297, -152.9062500020483810 ) ) ;
#12254=CARTESIAN_POINT ( 'NONE',  ( -5.405949406250003975, -9.363379034771801557, -82.84375000204836681 ) ) ;
#12255=CARTESIAN_POINT ( 'NONE',  ( -10.81189881249999729, 6.242252689847871849, -89.40625000204838102 ) ) ;
#12258=CARTESIAN_POINT ( 'NONE',  ( 10.81189881249999729, 6.242252689847867408, -178.4062500020484094 ) ) ;
#12259=CARTESIAN_POINT ( 'NONE',  ( -10.81189881249999729, 1.324075727343319199E-15, -186.7812500020484094 ) ) ;
#12261=CARTESIAN_POINT ( 'NONE',  ( 4.999999999999992006, -8.660254037844389075, -167.6250000040967905 ) ) ;
#12263=CARTESIAN_POINT ( 'NONE',  ( -10.81189881249999729, 1.324075727343319199E-15, -14.09375000204834905 ) ) ;
#12264=CARTESIAN_POINT ( 'NONE',  ( 5.000000000000000000, 8.660254037844385522, -162.6250000040967905 ) ) ;
#12265=CARTESIAN_POINT ( 'NONE',  ( -10.81189881249999729, 6.242252689847871849, -119.2187500020483810 ) ) ;
#12267=CARTESIAN_POINT ( 'NONE',  ( -2.293366432827344421E-15, -12.48450537969573659, -16.90625000204837391 ) ) ;
#12269=CARTESIAN_POINT ( 'NONE',  ( 9.999999999999998224, 1.224646799147353059E-15, -99.99999999999998579 ) ) ;
#12270=CARTESIAN_POINT ( 'NONE',  ( -10.81189881249999907, -6.242252689847864744, -113.1562500020483952 ) ) ;
#12274=CARTESIAN_POINT ( 'NONE',  ( 4.999999999999992006, -8.660254037844389075, -91.12500000409677625 ) ) ;
#12277=CARTESIAN_POINT ( 'NONE',  ( 10.81189881249999551, -6.242252689847874514, -47.96875000204836681 ) ) ;
#12282=VECTOR ( 'NONE', #39322, 1000.000000000000000 ) ;
#12283=CARTESIAN_POINT ( 'NONE',  ( 7.070501591499377789E-16, 11.54700538379251284, -17.00000000409676559 ) ) ;
#12285=EDGE_CURVE ( 'NONE', #35398, #6419, #12477, .T. ) ;
#12292=ORIENTED_EDGE ( 'NONE', *, *, #42320, .T. ) ;
#12294=CARTESIAN_POINT ( 'NONE',  ( 9.999999999999998224, 0.000000000000000000, -170.3750000040968189 ) ) ;
#12297=CARTESIAN_POINT ( 'NONE',  ( 5.405949406249999534, 9.363379034771803333, -188.7812500020484094 ) ) ;
#12299=CARTESIAN_POINT ( 'NONE',  ( 0.000000000000000000, 0.000000000000000000, -99.99999999999998579 ) ) ;
#12302=CARTESIAN_POINT ( 'NONE',  ( 10.81189881249999729, 0.000000000000000000, -110.8437500020483810 ) ) ;
#12303=CARTESIAN_POINT ( 'NONE',  ( 10.81189881249999551, -6.242252689847874514, -118.6562500020483952 ) ) ;
#12305=CARTESIAN_POINT ( 'NONE',  ( -10.81189881249999729, -6.242252689847864744, -120.4687500020483952 ) ) ;
#12307=CARTESIAN_POINT ( 'NONE',  ( 7.070501591499376803E-16, 11.54700538379251284, -179.0000000040967905 ) ) ;
#12308=CARTESIAN_POINT ( 'NONE',  ( -4.999999999999996447, 8.660254037844387298, -142.5000000000000000 ) ) ;
#12309=CARTESIAN_POINT ( 'NONE',  ( -9.999999999999998224, 5.773502691896259087, -11.87499999999996803 ) ) ;
#12312=CARTESIAN_POINT ( 'NONE',  ( -9.999999999999998224, 5.773502691896259087, -184.7500000040968189 ) ) ;
#12314=CARTESIAN_POINT ( 'NONE',  ( -10.81189881249999729, 1.324075727343319199E-15, -38.09375000204837391 ) ) ;
#12315=CARTESIAN_POINT ( 'NONE',  ( -10.00000000000051337, 5.773502691895962435, -148.7500000040967620 ) ) ;
#12316=CARTESIAN_POINT ( 'NONE',  ( -5.405949406249996869, 9.363379034771805109, -144.8437500020483810 ) ) ;
#12318=CARTESIAN_POINT ( 'NONE',  ( -4.999999999999996447, 8.660254037844387298, -145.5000000000000000 ) ) ;
#12319=CARTESIAN_POINT ( 'NONE',  ( -9.999999999999998224, 5.773502691896259087, -79.37500000000000000 ) ) ;
#12320=CARTESIAN_POINT ( 'NONE',  ( 10.81189881249999907, 6.242252689847868297, -139.4062500020484094 ) ) ;
#12322=ORIENTED_EDGE ( 'NONE', *, *, #13590, .F. ) ;
#12324=CARTESIAN_POINT ( 'NONE',  ( -2.121150477449813534E-15, -11.54700538379251284, -112.2500000040967763 ) ) ;
#12326=CARTESIAN_POINT ( 'NONE',  ( -2.293366432827344421E-15, -12.48450537969573659, -76.71875000204838102 ) ) ;
#12331=CARTESIAN_POINT ( 'NONE',  ( 10.81189881249999551, -6.242252689847874514, -36.15625000204835970 ) ) ;
#12335=CIRCLE ( 'NONE', #1324, 31.99999999999997158 ) ;
#12336=CARTESIAN_POINT ( 'NONE',  ( -9.999999999999998224, 1.224646799147353059E-15, -174.1250000040968189 ) ) ;
#12348=CARTESIAN_POINT ( 'NONE',  ( 9.999999999999998224, 0.000000000000000000, -176.0000000000000000 ) ) ;
#12349=CARTESIAN_POINT ( 'NONE',  ( -10.81189881249999907, -6.242252689847864744, -135.4687500020483810 ) ) ;
#12350=CARTESIAN_POINT ( 'NONE',  ( -2.293366432827344421E-15, -12.48450537969573659, -139.9062500020484094 ) ) ;
#12352=CARTESIAN_POINT ( 'NONE',  ( -10.81189881249999729, 1.324075727343319199E-15, -149.0937500020483810 ) ) ;
#12355=CARTESIAN_POINT ( 'NONE',  ( -9.999999999999998224, 1.224646799147353059E-15, -160.2500000000000000 ) ) ;
#12359=CARTESIAN_POINT ( 'NONE',  ( -2.293366432827344421E-15, -12.48450537969573659, -60.21875000204837391 ) ) ;
#12361=CARTESIAN_POINT ( 'NONE',  ( -5.405949406249996869, 9.363379034771805109, -171.8437500020484094 ) ) ;
#12365=CARTESIAN_POINT ( 'NONE',  ( 5.405949406249992428, -9.363379034771808662, -36.28125000204837391 ) ) ;
#12367=CARTESIAN_POINT ( 'NONE',  ( 5.000000000000000000, 8.660254037844385522, -100.7499999999999858 ) ) ;
#12368=EDGE_LOOP ( 'NONE', ( #28282, #26238, #35608, #32518 ) ) ;
#12369=CARTESIAN_POINT ( 'NONE',  ( -10.81189881249999729, 1.324075727343319199E-15, -116.2812500020483952 ) ) ;
#12370=CARTESIAN_POINT ( 'NONE',  ( -2.121150477449813534E-15, -11.54700538379251284, -142.2500000040967905 ) ) ;
#12371=CARTESIAN_POINT ( 'NONE',  ( -9.999999999999998224, 1.224646799147353059E-15, -158.7500000000000000 ) ) ;
#12373=EDGE_CURVE ( 'NONE', #34380, #21209, #17755, .T. ) ;
#12377=CARTESIAN_POINT ( 'NONE',  ( 5.405949406249992428, -9.363379034771808662, -61.78125000204837391 ) ) ;
#12378=CARTESIAN_POINT ( 'NONE',  ( 9.999999999999998224, 0.000000000000000000, -147.8750000040967905 ) ) ;
#12382=ORIENTED_EDGE ( 'NONE', *, *, #32988, .F. ) ;
#12389=ORIENTED_EDGE ( 'NONE', *, *, #10314, .F. ) ;
#12390=ORIENTED_EDGE ( 'NONE', *, *, #7748, .F. ) ;
#12397=CARTESIAN_POINT ( 'NONE',  ( 4.999999999999992006, -8.660254037844389075, -109.1250000040967763 ) ) ;
#12399=CARTESIAN_POINT ( 'NONE',  ( 5.000000000000000000, 8.660254037844385522, -28.74999999999997158 ) ) ;
#12402=CARTESIAN_POINT ( 'NONE',  ( 5.405949406249992428, -9.363379034771808662, -156.0937500020483810 ) ) ;
#12403=CARTESIAN_POINT ( 'NONE',  ( -5.405949406249996869, 9.363379034771805109, -167.3437500020484094 ) ) ;
#12405=( BOUNDED_CURVE ( )  B_SPLINE_CURVE ( 2, ( #24935, #41297, #14535, #1839, #4848, #34640, #21027 ),
 .UNSPECIFIED., .F., .F. ) 
 B_SPLINE_CURVE_WITH_KNOTS ( ( 3, 2, 2, 3 ),
 ( 0.1604477611940298698, 0.1616915422885572551, 0.1629353233830845848, 0.1641791044776119424 ),
 .UNSPECIFIED. ) 
 CURVE ( )  GEOMETRIC_REPRESENTATION_ITEM ( )  RATIONAL_B_SPLINE_CURVE ( ( 0.9999999999999970024, 0.8660254037844417052, 1.000000000000000000, 0.8660254037844387076, 1.000000000000000000, 0.8660254037844387076, 1.000000000000000000 ) ) 
 REPRESENTATION_ITEM ( '' )  );
#12406=CARTESIAN_POINT ( 'NONE',  ( 4.999999999999992006, -8.660254037844389075, -198.7500000000000000 ) ) ;
#12411=CARTESIAN_POINT ( 'NONE',  ( 10.81189881249999907, 6.242252689847868297, -56.90625000204837391 ) ) ;
#12413=CARTESIAN_POINT ( 'NONE',  ( -9.999999999999998224, 5.773502691896259087, -119.8750000000000000 ) ) ;
#12415=CARTESIAN_POINT ( 'NONE',  ( 10.81189881249999729, 0.000000000000000000, -145.5312500020483810 ) ) ;
#12416=CARTESIAN_POINT ( 'NONE',  ( 10.81189881249999551, -6.242252689847874514, -156.1562500020484094 ) ) ;
#12419=CARTESIAN_POINT ( 'NONE',  ( 10.81189881249999729, 0.000000000000000000, -86.84375000204836681 ) ) ;
#12422=CARTESIAN_POINT ( 'NONE',  ( 10.81189881249999551, -6.242252689847874514, -190.4687500020484094 ) ) ;
#12424=CARTESIAN_POINT ( 'NONE',  ( -2.121150477449813534E-15, -11.54700538379251284, -116.7500000040967905 ) ) ;
#12425=CARTESIAN_POINT ( 'NONE',  ( 9.999999999999998224, 0.000000000000000000, -140.3750000040967905 ) ) ;
#12426=CARTESIAN_POINT ( 'NONE',  ( -10.81189881249999729, 6.242252689847871849, -80.40625000204839523 ) ) ;
#12428=CARTESIAN_POINT ( 'NONE',  ( 9.999999999999998224, 0.000000000000000000, -66.87500000409676204 ) ) ;
#12429=CARTESIAN_POINT ( 'NONE',  ( 10.81189881249999907, 6.242252689847868297, -17.71875000204836681 ) ) ;
#12432=CARTESIAN_POINT ( 'NONE',  ( 7.644554776091147741E-16, 12.48450537969573659, -19.15625000204837391 ) ) ;
#12441=ORIENTED_EDGE ( 'NONE', *, *, #37394, .F. ) ;
#12442=CARTESIAN_POINT ( 'NONE',  ( 5.000000000000000000, 8.660254037844385522, -116.1250000040967905 ) ) ;
#12444=ORIENTED_EDGE ( 'NONE', *, *, #23289, .T. ) ;
#12446=ADVANCED_FACE ( 'NONE', ( #26510 ), #22852, .F. ) ;
#12448=DIRECTION ( 'NONE',  ( 1.000000000000000000, 0.000000000000000000, 0.000000000000000000 ) ) ;
#12450=CARTESIAN_POINT ( 'NONE',  ( 10.18637341149928410, -0.5909213003623300375, -100.0000000000000000 ) ) ;
#12453=CARTESIAN_POINT ( 'NONE',  ( 9.999999999999998224, 0.000000000000000000, -108.4999999999999858 ) ) ;
#12455=CARTESIAN_POINT ( 'NONE',  ( -10.81189881249999729, 6.242252689847871849, -156.9062500020483810 ) ) ;
#12457=DIRECTION ( 'NONE',  ( 1.000000000000000000, 0.000000000000000000, 0.000000000000000000 ) ) ;
#12461=CARTESIAN_POINT ( 'NONE',  ( 10.81189881249999551, -6.242252689847874514, -80.96875000204838102 ) ) ;
#12462=CARTESIAN_POINT ( 'NONE',  ( -2.293366432827344421E-15, -12.48450537969573659, -84.40625000204838102 ) ) ;
#12465=CARTESIAN_POINT ( 'NONE',  ( -2.293366432827344421E-15, -12.48450537969573659, -165.4062500020483526 ) ) ;
#12466=CARTESIAN_POINT ( 'NONE',  ( -10.81189881249999907, -6.242252689847864744, -182.1562500020483810 ) ) ;
#12468=CARTESIAN_POINT ( 'NONE',  ( 9.999999999999998224, 0.000000000000000000, -156.8750000040967905 ) ) ;
#12470=CARTESIAN_POINT ( 'NONE',  ( -2.293366432827344421E-15, -12.48450537969573659, -7.718750002048357040 ) ) ;
#12471=CARTESIAN_POINT ( 'NONE',  ( -10.81189881249999729, 1.324075727343319199E-15, -111.5937500020483810 ) ) ;
#12473=CARTESIAN_POINT ( 'NONE',  ( -10.81189881249999907, -6.242252689847864744, -20.15625000204837747 ) ) ;
#12477=LINE ( 'NONE', #16557, #16844 ) ;
#12478=CARTESIAN_POINT ( 'NONE',  ( 10.81189881249999907, 6.242252689847868297, -115.4062500020484094 ) ) ;
#12480=EDGE_LOOP ( 'NONE', ( #19404, #38003, #6343, #27634 ) ) ;
#12481=CARTESIAN_POINT ( 'NONE',  ( 9.999999999999996447, -5.773502691896262640, -91.00000000409677625 ) ) ;
#12483=CARTESIAN_POINT ( 'NONE',  ( 10.81189881249999551, -6.242252689847874514, -50.96875000204836681 ) ) ;
#12490=CARTESIAN_POINT ( 'NONE',  ( 5.000000000000000000, 8.660254037844385522, -20.12500000409675494 ) ) ;
#12491=VECTOR ( 'NONE', #732, 1000.000000000000000 ) ;
#12504=CARTESIAN_POINT ( 'NONE',  ( -9.999999999999998224, 1.224646799147353059E-15, -175.2500000000000284 ) ) ;
#12508=CARTESIAN_POINT ( 'NONE',  ( 10.81189881249999551, -6.242252689847874514, -180.1562500020484379 ) ) ;
#12513=CARTESIAN_POINT ( 'NONE',  ( 10.81189881249999907, 6.242252689847868297, -100.2187500020483810 ) ) ;
#12514=CARTESIAN_POINT ( 'NONE',  ( -9.999999999999998224, 1.224646799147353059E-15, -143.7500000000000000 ) ) ;
#12515=CARTESIAN_POINT ( 'NONE',  ( 7.644554776091147741E-16, 12.48450537969573659, -104.6562500020483810 ) ) ;
#12517=CARTESIAN_POINT ( 'NONE',  ( 10.81189881249999729, 0.000000000000000000, -119.8437500020483810 ) ) ;
#12521=CARTESIAN_POINT ( 'NONE',  ( -9.999999999999998224, 5.773502691896259087, -140.8750000000000000 ) ) ;
#12522=CARTESIAN_POINT ( 'NONE',  ( -4.999999999999996447, 8.660254037844387298, -13.49999999999995737 ) ) ;
#12525=CARTESIAN_POINT ( 'NONE',  ( -9.999999999999998224, 5.773502691896259087, -189.2500000040967905 ) ) ;
#12527=CARTESIAN_POINT ( 'NONE',  ( -10.81189881249999729, 1.324075727343319199E-15, -35.09375000204836681 ) ) ;
#12528=CARTESIAN_POINT ( 'NONE',  ( -2.121150477449813534E-15, -11.54700538379251284, -105.8749999999999858 ) ) ;
#12529=CARTESIAN_POINT ( 'NONE',  ( -2.293366432827344421E-15, -12.48450537969573659, -147.2187500020484094 ) ) ;
#12532=CARTESIAN_POINT ( 'NONE',  ( 4.999999999999992006, -8.660254037844389075, -69.74999999999997158 ) ) ;
#12533=CARTESIAN_POINT ( 'NONE',  ( -5.405949406249996869, 9.363379034771805109, -137.5312500020484094 ) ) ;
#12535=EDGE_CURVE ( 'NONE', #36340, #7903, #410, .T. ) ;
#12538=CARTESIAN_POINT ( 'NONE',  ( 4.999999999999992006, -8.660254037844389075, -118.1250000040967905 ) ) ;
#12540=CARTESIAN_POINT ( 'NONE',  ( 10.81189881249999729, 0.000000000000000000, -70.34375000204836681 ) ) ;
#12546=CARTESIAN_POINT ( 'NONE',  ( -10.81189881249999907, -6.242252689847864744, -36.65625000204835970 ) ) ;
#12547=LINE ( 'NONE', #3277, #16215 ) ;
#12550=CARTESIAN_POINT ( 'NONE',  ( -10.00000000000012790, -5.773502691896178263, -174.0000000040968473 ) ) ;
#12558=DIRECTION ( 'NONE',  ( -0.000000000000000000, -0.000000000000000000, -1.000000000000000000 ) ) ;
#12562=CARTESIAN_POINT ( 'NONE',  ( 10.81189881249999907, 6.242252689847868297, -133.2187500020483810 ) ) ;
#12563=CARTESIAN_POINT ( 'NONE',  ( 10.81189881249999729, 0.000000000000000000, -139.5312500020484094 ) ) ;
#12565=CARTESIAN_POINT ( 'NONE',  ( -10.81189881249999729, -6.242252689847864744, -142.9687500020483810 ) ) ;
#12566=DIRECTION ( 'NONE',  ( -0.000000000000000000, -0.000000000000000000, -1.000000000000000000 ) ) ;
#12567=CARTESIAN_POINT ( 'NONE',  ( 9.999999999999479527, 5.773502691896553074, -141.7500000040967620 ) ) ;
#12568=CARTESIAN_POINT ( 'NONE',  ( 7.070501591499377789E-16, 11.54700538379251284, -163.6250000000000000 ) ) ;
#12572=CARTESIAN_POINT ( 'NONE',  ( -5.405949406249996869, 9.363379034771805109, -59.34375000204835970 ) ) ;
#12573=FACE_OUTER_BOUND ( 'NONE', #17482, .T. ) ;
#12574=CARTESIAN_POINT ( 'NONE',  ( -2.293366432827344421E-15, -12.48450537969573659, -168.2187500020483810 ) ) ;
#12579=CARTESIAN_POINT ( 'NONE',  ( -10.00000000000000000, -5.773502691896251982, -92.62499999999998579 ) ) ;
#12580=ORIENTED_EDGE ( 'NONE', *, *, #30657, .T. ) ;
#12581=CARTESIAN_POINT ( 'NONE',  ( 5.405949406249999534, 9.363379034771803333, -116.7812500020483952 ) ) ;
#12582=CARTESIAN_POINT ( 'NONE',  ( -10.00000000000000000, -5.773502691896251982, -138.0000000040967905 ) ) ;
#12587=CARTESIAN_POINT ( 'NONE',  ( 5.405949406249999534, 9.363379034771803333, -61.28125000204837391 ) ) ;
#12593=ORIENTED_EDGE ( 'NONE', *, *, #41196, .F. ) ;
#12594=DIRECTION ( 'NONE',  ( -0.000000000000000000, -0.000000000000000000, -1.000000000000000000 ) ) ;
#12596=ORIENTED_EDGE ( 'NONE', *, *, #16447, .F. ) ;
#12597=ORIENTED_EDGE ( 'NONE', *, *, #23293, .T. ) ;
#12598=VERTEX_POINT ( 'NONE', #36638 ) ;
#12603=ORIENTED_EDGE ( 'NONE', *, *, #19230, .T. ) ;
#12605=CARTESIAN_POINT ( 'NONE',  ( 4.999999999999992006, -8.660254037844389075, -29.24999999999997158 ) ) ;
#12608=CARTESIAN_POINT ( 'NONE',  ( -10.81189881249999729, 1.324075727343319199E-15, -158.0937500020483810 ) ) ;
#12609=CARTESIAN_POINT ( 'NONE',  ( -10.81189881249999729, 6.242252689847871849, -173.2187500020483810 ) ) ;
#12613=CARTESIAN_POINT ( 'NONE',  ( 9.999999999999996447, -5.773502691896262640, -183.6250000000000000 ) ) ;
#12617=CARTESIAN_POINT ( 'NONE',  ( 0.000000000000000000, 0.000000000000000000, -99.99999999999998579 ) ) ;
#12619=CARTESIAN_POINT ( 'NONE',  ( -2.293366432827344421E-15, -12.48450537969573659, -58.90625000204838102 ) ) ;
#12621=CARTESIAN_POINT ( 'NONE',  ( 5.000000000000000000, 8.660254037844385522, -126.2499999999999716 ) ) ;
#12623=CARTESIAN_POINT ( 'NONE',  ( 10.81189881249999551, -6.242252689847874514, -145.6562500020484094 ) ) ;
#12624=CARTESIAN_POINT ( 'NONE',  ( 5.405949406249999534, 9.363379034771803333, -154.2812500020484094 ) ) ;
#12627=CARTESIAN_POINT ( 'NONE',  ( -10.81189881249999907, -6.242252689847864744, -90.46875000204836681 ) ) ;
#12630=CARTESIAN_POINT ( 'NONE',  ( 10.81189881249999729, 0.000000000000000000, -190.3437500020484094 ) ) ;
#12634=CARTESIAN_POINT ( 'NONE',  ( -5.405949406250003975, -9.363379034771801557, -87.53125000204838102 ) ) ;
#12637=CARTESIAN_POINT ( 'NONE',  ( 9.999999999999998224, 0.000000000000000000, -59.37500000409676204 ) ) ;
#12638=CARTESIAN_POINT ( 'NONE',  ( -5.405949406250003975, -9.363379034771801557, -19.84375000204835615 ) ) ;
#12639=VERTEX_POINT ( 'NONE', #11152 ) ;
#12641=CARTESIAN_POINT ( 'NONE',  ( -5.405949406250003975, -9.363379034771801557, -12.53125000204835615 ) ) ;
#12654=ORIENTED_EDGE ( 'NONE', *, *, #22021, .F. ) ;
#12660=CARTESIAN_POINT ( 'NONE',  ( -4.999999999999996447, 8.660254037844387298, -124.5000000000000000 ) ) ;
#12662=CARTESIAN_POINT ( 'NONE',  ( 7.644554776091147741E-16, 12.48450537969573659, -157.1562500020484094 ) ) ;
#12668=CARTESIAN_POINT ( 'NONE',  ( -2.293366432827344421E-15, -12.48450537969573659, -75.21875000204839523 ) ) ;
#12669=CARTESIAN_POINT ( 'NONE',  ( -10.81189881249999729, 6.242252689847871849, -81.90625000204838102 ) ) ;
#12672=CARTESIAN_POINT ( 'NONE',  ( -10.81189881249999729, -6.242252689847864744, -170.1562500020484094 ) ) ;
#12673=CARTESIAN_POINT ( 'NONE',  ( 10.81189881249999551, -6.242252689847874514, -181.6562500020484379 ) ) ;
#12674=CARTESIAN_POINT ( 'NONE',  ( 9.999999999999998224, 0.000000000000000000, -152.3750000040967905 ) ) ;
#12676=CARTESIAN_POINT ( 'NONE',  ( -10.81189881249999907, -6.242252689847864744, -6.468750002048357040 ) ) ;
#12678=CARTESIAN_POINT ( 'NONE',  ( -5.405949406249996869, 9.363379034771805109, -110.3437500020483810 ) ) ;
#12680=CARTESIAN_POINT ( 'NONE',  ( 5.405949406249999534, 9.363379034771803333, -8.781250002048352599 ) ) ;
#12683=CARTESIAN_POINT ( 'NONE',  ( -5.405949406250003975, -9.363379034771801557, -107.0312500020483810 ) ) ;
#12686=CARTESIAN_POINT ( 'NONE',  ( -4.999999999999996447, 8.660254037844387298, -85.87500000409677625 ) ) ;
#12687=CARTESIAN_POINT ( 'NONE',  ( -9.999999999999998224, 0.000000000000000000, -99.99999999999998579 ) ) ;
#12688=CARTESIAN_POINT ( 'NONE',  ( -10.81189881249999907, -6.242252689847864744, -45.46875000204835970 ) ) ;
#12691=EDGE_CURVE ( 'NONE', #270, #7415, #1797, .T. ) ;
#12693=CARTESIAN_POINT ( 'NONE',  ( -9.999999999999998224, 5.773502691896259087, -21.25000000409676915 ) ) ;
#12695=CARTESIAN_POINT ( 'NONE',  ( -9.999999999999998224, 0.000000000000000000, -99.99999999999998579 ) ) ;
#12697=ORIENTED_EDGE ( 'NONE', *, *, #30302, .F. ) ;
#12703=ORIENTED_EDGE ( 'NONE', *, *, #36279, .T. ) ;
#12707=CARTESIAN_POINT ( 'NONE',  ( -10.81189881249999907, -6.242252689847864744, -183.6562500020483810 ) ) ;
#12708=CARTESIAN_POINT ( 'NONE',  ( -9.999999999999998224, 1.224646799147353059E-15, -174.1250000040968189 ) ) ;
#12712=CARTESIAN_POINT ( 'NONE',  ( -10.81189881249999729, 6.242252689847871849, -104.2187500020483810 ) ) ;
#12714=CARTESIAN_POINT ( 'NONE',  ( -10.81189881249999729, 1.324075727343319199E-15, -111.7812500020483810 ) ) ;
#12716=CARTESIAN_POINT ( 'NONE',  ( 10.81189881249999729, 6.242252689847867408, -124.2187500020483952 ) ) ;
#12719=CARTESIAN_POINT ( 'NONE',  ( -9.999999999999998224, 5.773502691896259087, -137.8750000000000000 ) ) ;
#12720=CARTESIAN_POINT ( 'NONE',  ( 9.999999999999996447, -5.773502691896262640, -6.624999999999964473 ) ) ;
#12724=CARTESIAN_POINT ( 'NONE',  ( -10.00000000000000000, -5.773502691896251982, -177.0000000040967620 ) ) ;
#12726=CARTESIAN_POINT ( 'NONE',  ( -10.81189881249999729, 6.242252689847871849, -27.71875000204837391 ) ) ;
#12728=CARTESIAN_POINT ( 'NONE',  ( -2.293366432827344421E-15, -12.48450537969573659, -138.2187500020483810 ) ) ;
#12731=CARTESIAN_POINT ( 'NONE',  ( 10.00000000000000000, 5.773502691896255534, -70.87499999999998579 ) ) ;
#12732=CARTESIAN_POINT ( 'NONE',  ( 10.81189881249999907, 6.242252689847868297, -128.9062500020483810 ) ) ;
#12736=CARTESIAN_POINT ( 'NONE',  ( -5.000000000000003553, -8.660254037844383745, -119.8750000040967905 ) ) ;
#12737=CARTESIAN_POINT ( 'NONE',  ( -9.999999999999998224, 1.224646799147353059E-15, -169.2500000000000000 ) ) ;
#12738=CARTESIAN_POINT ( 'NONE',  ( 7.644554776091147741E-16, 12.48450537969573659, -66.96875000204838102 ) ) ;
#12745=CARTESIAN_POINT ( 'NONE',  ( 10.00000000000000000, 5.773502691896255534, -44.25000000409676204 ) ) ;
#12746=CARTESIAN_POINT ( 'NONE',  ( -5.405949406249996869, 9.363379034771805109, -32.53125000204837391 ) ) ;
#12749=DIRECTION ( 'NONE',  ( -0.000000000000000000, -0.000000000000000000, -1.000000000000000000 ) ) ;
#12751=ADVANCED_FACE ( 'NONE', ( #31677 ), #21300, .F. ) ;
#12762=( BOUNDED_CURVE ( )  B_SPLINE_CURVE ( 2, ( #20099, #13185, #16635, #29195, #33292, #3718, #29837 ),
 .UNSPECIFIED., .F., .F. ) 
 B_SPLINE_CURVE_WITH_KNOTS ( ( 3, 2, 2, 3 ),
 ( 0.2686567164179105571, 0.2699004975124379424, 0.2711442786069652722, 0.2723880597014926574 ),
 .UNSPECIFIED. ) 
 CURVE ( )  GEOMETRIC_REPRESENTATION_ITEM ( )  RATIONAL_B_SPLINE_CURVE ( ( 0.9999999999999880096, 0.8660254037844506980, 1.000000000000000000, 0.8660254037844387076, 1.000000000000000000, 0.8660254037844267172, 1.000000000000011990 ) ) 
 REPRESENTATION_ITEM ( '' )  );
#12768=DIRECTION ( 'NONE',  ( 0.000000000000000000, 0.000000000000000000, -1.000000000000000000 ) ) ;
#12769=CARTESIAN_POINT ( 'NONE',  ( -10.81189881249999907, -6.242252689847864744, -124.9687500020483810 ) ) ;
#12770=VECTOR ( 'NONE', #23771, 1000.000000000000000 ) ;
#12771=CARTESIAN_POINT ( 'NONE',  ( 10.81189881249999551, -6.242252689847874514, -130.6562500020484094 ) ) ;
#12773=CARTESIAN_POINT ( 'NONE',  ( -5.405949406250003975, -9.363379034771801557, -145.8437500020483810 ) ) ;
#12774=CARTESIAN_POINT ( 'NONE',  ( 9.415087197078790382, -5.361960122183175415, -179.9999999999999432 ) ) ;
#12777=CARTESIAN_POINT ( 'NONE',  ( -2.121150477449813534E-15, -11.54700538379251284, -162.8750000000000000 ) ) ;
#12778=CARTESIAN_POINT ( 'NONE',  ( -5.405949406249996869, 9.363379034771805109, -1.031250002048372805 ) ) ;
#12781=CARTESIAN_POINT ( 'NONE',  ( -2.293366432827344421E-15, -12.48450537969573659, -52.71875000204837391 ) ) ;
#12783=CARTESIAN_POINT ( 'NONE',  ( -10.81189881249999729, 1.324075727343319199E-15, -165.5937500020484094 ) ) ;
#12787=CARTESIAN_POINT ( 'NONE',  ( 9.999999999999998224, 1.224646799147353059E-15, -99.99999999999998579 ) ) ;
#12789=CARTESIAN_POINT ( 'NONE',  ( 9.999999999999998224, 0.000000000000000000, -94.99999999999998579 ) ) ;
#12790=ORIENTED_EDGE ( 'NONE', *, *, #14180, .F. ) ;
#12791=CARTESIAN_POINT ( 'NONE',  ( -10.81189881249999729, 6.242252689847871849, -117.9062500020483952 ) ) ;
#12792=CARTESIAN_POINT ( 'NONE',  ( 5.000000000000000000, 8.660254037844385522, -138.6250000040967905 ) ) ;
#12797=CARTESIAN_POINT ( 'NONE',  ( -10.81189881249999729, 6.242252689847871849, -57.90625000204838813 ) ) ;
#12806=EDGE_CURVE ( 'NONE', #35300, #41736, #22603, .T. ) ;
#12808=EDGE_LOOP ( 'NONE', ( #13955, #20092, #12580, #29190 ) ) ;
#12811=ORIENTED_EDGE ( 'NONE', *, *, #4462, .T. ) ;
#12819=CARTESIAN_POINT ( 'NONE',  ( -5.000000000000003553, -8.660254037844383745, -24.99999999999996803 ) ) ;
#12822=CARTESIAN_POINT ( 'NONE',  ( 7.644554776091147741E-16, 12.48450537969573659, -146.4687500020484094 ) ) ;
#12823=CARTESIAN_POINT ( 'NONE',  ( 10.81189881249999729, 6.242252689847867408, -173.7187500020483810 ) ) ;
#12825=CARTESIAN_POINT ( 'NONE',  ( 4.999999999999992006, -8.660254037844389075, -161.6250000040967905 ) ) ;
#12826=CARTESIAN_POINT ( 'NONE',  ( 9.999999999999998224, 0.000000000000000000, -186.5000000000000000 ) ) ;
#12831=CARTESIAN_POINT ( 'NONE',  ( -10.81189881249999729, 1.324075727343319199E-15, -188.0937500020483810 ) ) ;
#12833=VECTOR ( 'NONE', #2094, 1000.000000000000000 ) ;
#12834=CARTESIAN_POINT ( 'NONE',  ( 10.81189881249999551, -6.242252689847874514, -57.15625000204837391 ) ) ;
#12836=CARTESIAN_POINT ( 'NONE',  ( -4.999999999999996447, 8.660254037844387298, -113.9999999999999858 ) ) ;
#12837=ORIENTED_EDGE ( 'NONE', *, *, #13221, .T. ) ;
#12838=CARTESIAN_POINT ( 'NONE',  ( -5.405949406249996869, 9.363379034771805109, -140.5312500020484094 ) ) ;
#12839=CARTESIAN_POINT ( 'NONE',  ( 10.81189881249999729, 0.000000000000000000, -153.0312500020484094 ) ) ;
#12842=CARTESIAN_POINT ( 'NONE',  ( 5.405949406249999534, 9.363379034771803333, -94.09375000204838102 ) ) ;
#12845=CARTESIAN_POINT ( 'NONE',  ( 5.405949406249992428, -9.363379034771808662, -190.5937500020484094 ) ) ;
#12847=DIRECTION ( 'NONE',  ( -0.000000000000000000, -0.000000000000000000, -1.000000000000000000 ) ) ;
#12849=CARTESIAN_POINT ( 'NONE',  ( -10.81189881249999729, 1.324075727343319199E-15, -84.78125000204838102 ) ) ;
#12851=CARTESIAN_POINT ( 'NONE',  ( 4.999999999999992006, -8.660254037844389075, -58.12500000409676204 ) ) ;
#12852=CARTESIAN_POINT ( 'NONE',  ( -10.81189881249999729, 6.242252689847871849, -21.71875000204837036 ) ) ;
#12853=DIRECTION ( 'NONE',  ( -0.000000000000000000, -0.000000000000000000, -1.000000000000000000 ) ) ;
#12855=CARTESIAN_POINT ( 'NONE',  ( -10.81189881249999907, -6.242252689847864744, -9.656250002048366810 ) ) ;
#12875=CARTESIAN_POINT ( 'NONE',  ( 5.405949406249999534, 9.363379034771803333, -154.2812500020484094 ) ) ;
#12877=CARTESIAN_POINT ( 'NONE',  ( 5.000000000000000000, 8.660254037844385522, -121.7500000000000000 ) ) ;
#12881=CARTESIAN_POINT ( 'NONE',  ( 5.405949406249992428, -9.363379034771808662, -81.09375000204838102 ) ) ;
#12882=CARTESIAN_POINT ( 'NONE',  ( 10.81189881249999729, 0.000000000000000000, -82.53125000204838102 ) ) ;
#12884=( BOUNDED_CURVE ( )  B_SPLINE_CURVE ( 2, ( #24035, #1803, #28129, #20992, #33964, #4385, #30725 ),
 .UNSPECIFIED., .F., .F. ) 
 B_SPLINE_CURVE_WITH_KNOTS ( ( 3, 2, 2, 3 ),
 ( 0.1641791044776119424, 0.1654228855721392999, 0.1666666666666666574, 0.1679104477611940427 ),
 .UNSPECIFIED. ) 
 CURVE ( )  GEOMETRIC_REPRESENTATION_ITEM ( )  RATIONAL_B_SPLINE_CURVE ( ( 1.000000000000000000, 0.8660254037844387076, 1.000000000000000000, 0.8660254037844387076, 1.000000000000000000, 0.8660254037844387076, 1.000000000000000000 ) ) 
 REPRESENTATION_ITEM ( '' )  );
#12886=CARTESIAN_POINT ( 'NONE',  ( -10.81189881249999729, 1.324075727343319199E-15, -164.2812500020484094 ) ) ;
#12887=CARTESIAN_POINT ( 'NONE',  ( -10.81189881249999729, 6.242252689847871849, -179.4062500020484094 ) ) ;
#12888=CARTESIAN_POINT ( 'NONE',  ( 9.999999999999996447, -5.773502691896262640, -157.0000000040968189 ) ) ;
#12889=CARTESIAN_POINT ( 'NONE',  ( -9.999999999999998224, 1.224646799147353059E-15, -178.2500000000000284 ) ) ;
#12890=CARTESIAN_POINT ( 'NONE',  ( -10.81189881249999729, 1.324075727343319199E-15, -9.593750002048345493 ) ) ;
#12892=CARTESIAN_POINT ( 'NONE',  ( -5.405949406250003975, -9.363379034771801557, -114.3437500020483810 ) ) ;
#12894=CARTESIAN_POINT ( 'NONE',  ( -5.405949406250003975, -9.363379034771801557, -12.53125000204835615 ) ) ;
#12896=CARTESIAN_POINT ( 'NONE',  ( 10.81189881249999551, -6.242252689847874514, -109.6562500020483810 ) ) ;
#12899=CARTESIAN_POINT ( 'NONE',  ( -9.999999999999998224, 5.773502691896259087, -85.75000000409676204 ) ) ;
#12900=CARTESIAN_POINT ( 'NONE',  ( 5.000000000000000000, 8.660254037844385522, -146.1250000040967905 ) ) ;
#12901=CARTESIAN_POINT ( 'NONE',  ( 7.644554776091147741E-16, 12.48450537969573659, -38.46875000204835260 ) ) ;
#12905=CARTESIAN_POINT ( 'NONE',  ( -4.999999999999996447, 8.660254037844387298, -9.375000004096744277 ) ) ;
#12908=ORIENTED_EDGE ( 'NONE', *, *, #13545, .T. ) ;
#12911=ORIENTED_EDGE ( 'NONE', *, *, #28516, .T. ) ;
#12915=ORIENTED_EDGE ( 'NONE', *, *, #1201, .T. ) ;
#12918=CARTESIAN_POINT ( 'NONE',  ( 7.644554776091147741E-16, 12.48450537969573659, -176.6562500020484094 ) ) ;
#12920=CARTESIAN_POINT ( 'NONE',  ( -5.000000000000003553, -8.660254037844383745, -146.8750000040967905 ) ) ;
#12923=CARTESIAN_POINT ( 'NONE',  ( -10.81189881249999729, 6.242252689847871849, -105.7187500020483668 ) ) ;
#12925=CARTESIAN_POINT ( 'NONE',  ( 7.644554776091147741E-16, 12.48450537969573659, -110.6562500020483952 ) ) ;
#12927=CARTESIAN_POINT ( 'NONE',  ( -10.81189881249999729, 1.324075727343319199E-15, -116.0937500020483810 ) ) ;
#12930=CARTESIAN_POINT ( 'NONE',  ( -9.999999999999998224, 5.773502691896259087, -142.3750000000000000 ) ) ;
#12931=CARTESIAN_POINT ( 'NONE',  ( 9.999999999999996447, -5.773502691896262640, -3.624999999999961364 ) ) ;
#12934=CARTESIAN_POINT ( 'NONE',  ( -2.121150477449813534E-15, -11.54700538379251284, -182.7500000040967905 ) ) ;
#12937=CARTESIAN_POINT ( 'NONE',  ( -10.81189881249999729, 6.242252689847871849, -26.21875000204837391 ) ) ;
#12939=CARTESIAN_POINT ( 'NONE',  ( 10.81189881249999729, 0.000000000000000000, -134.8437500020484094 ) ) ;
#12942=CARTESIAN_POINT ( 'NONE',  ( 5.000000000000000000, 8.660254037844385522, -111.2499999999999858 ) ) ;
#12943=CARTESIAN_POINT ( 'NONE',  ( -9.999999999999998224, 1.224646799147353059E-15, -64.24999999999997158 ) ) ;
#12944=CARTESIAN_POINT ( 'NONE',  ( 7.644554776091147741E-16, 12.48450537969573659, -131.6562500020483810 ) ) ;
#12948=CARTESIAN_POINT ( 'NONE',  ( 4.999999999999992006, -8.660254037844389075, -106.1250000040967763 ) ) ;
#12950=CARTESIAN_POINT ( 'NONE',  ( -2.293366432827344421E-15, -12.48450537969573659, -67.71875000204838102 ) ) ;
#12956=CARTESIAN_POINT ( 'NONE',  ( -5.000000000000003553, -8.660254037844383745, -34.37500000409676915 ) ) ;
#12957=CARTESIAN_POINT ( 'NONE',  ( 5.405949406249999534, 9.363379034771803333, -37.28125000204837391 ) ) ;
#12958=CARTESIAN_POINT ( 'NONE',  ( 9.999999999999479527, 5.773502691896553074, -117.7500000040968189 ) ) ;
#12966=( BOUNDED_CURVE ( )  B_SPLINE_CURVE ( 2, ( #6636, #33191, #19574, #13085, #9451, #39223, #32757 ),
 .UNSPECIFIED., .F., .F. ) 
 B_SPLINE_CURVE_WITH_KNOTS ( ( 3, 2, 2, 3 ),
 ( 0.1044776119402986148, 0.1057213930348259306, 0.1069651741293532465, 0.1082089552238805485 ),
 .UNSPECIFIED. ) 
 CURVE ( )  GEOMETRIC_REPRESENTATION_ITEM ( )  RATIONAL_B_SPLINE_CURVE ( ( 0.9999999999999880096, 0.8660254037844506980, 1.000000000000000000, 0.8660254037844387076, 1.000000000000000000, 0.8660254037844431485, 0.9999999999999955591 ) ) 
 REPRESENTATION_ITEM ( '' )  );
#12967=CARTESIAN_POINT ( 'NONE',  ( -5.000000000000003553, -8.660254037844383745, -104.4999999999999858 ) ) ;
#12970=CARTESIAN_POINT ( 'NONE',  ( 9.999999999999998224, 1.224646799147353059E-15, -99.99999999999998579 ) ) ;
#12971=EDGE_CURVE ( 'NONE', #41419, #40786, #3173, .T. ) ;
#12974=EDGE_CURVE ( 'NONE', #40153, #33328, #20789, .T. ) ;
#12975=CARTESIAN_POINT ( 'NONE',  ( -2.293366432827344421E-15, -12.48450537969573659, -126.2187500020483952 ) ) ;
#12976=CARTESIAN_POINT ( 'NONE',  ( 5.405949406249999534, 9.363379034771803333, -133.2812500020483810 ) ) ;
#12978=CARTESIAN_POINT ( 'NONE',  ( 10.81189881249999729, 0.000000000000000000, -134.8437500020484094 ) ) ;
#12981=CARTESIAN_POINT ( 'NONE',  ( -5.000000000000003553, -8.660254037844383745, -163.0000000000000000 ) ) ;
#12982=CARTESIAN_POINT ( 'NONE',  ( -10.81189881249999729, 6.242252689847871849, -0.9062500020483588159 ) ) ;
#12985=CARTESIAN_POINT ( 'NONE',  ( -10.81189881249999729, 6.242252689847871849, -54.71875000204837391 ) ) ;
#12987=CARTESIAN_POINT ( 'NONE',  ( 7.644554776091147741E-16, 12.48450537969573659, -158.4687500020483810 ) ) ;
#12991=CARTESIAN_POINT ( 'NONE',  ( -9.999999999999998224, 1.224646799147353059E-15, -179.7500000000000284 ) ) ;
#12993=CARTESIAN_POINT ( 'NONE',  ( -9.999999999999998224, 1.224646799147353059E-15, -88.24999999999998579 ) ) ;
#12994=VERTEX_POINT ( 'NONE', #9832 ) ;
#12995=CARTESIAN_POINT ( 'NONE',  ( -5.405949406250003975, -9.363379034771801557, -114.5312500020483952 ) ) ;
#12996=CARTESIAN_POINT ( 'NONE',  ( 4.999999999999992006, -8.660254037844389075, -131.6250000040967620 ) ) ;
#13002=CARTESIAN_POINT ( 'NONE',  ( -5.405949406249996869, 9.363379034771805109, -59.53125000204836681 ) ) ;
#13005=EDGE_CURVE ( 'NONE', #28518, #19199, #1537, .T. ) ;
#13008=CARTESIAN_POINT ( 'NONE',  ( -9.999999999999998224, 1.224646799147353059E-15, -166.6250000040967905 ) ) ;
#13010=EDGE_CURVE ( 'NONE', #7903, #19199, #32314, .T. ) ;
#13012=CARTESIAN_POINT ( 'NONE',  ( -9.999999999999998224, 1.224646799147353059E-15, -130.6250000040967620 ) ) ;
#13014=AXIS2_PLACEMENT_3D ( 'NONE', #8246, #11669, #41664 ) ;
#13018=ORIENTED_EDGE ( 'NONE', *, *, #21969, .T. ) ;
#13019=EDGE_CURVE ( 'NONE', #10539, #23457, #2739, .T. ) ;
#13025=CARTESIAN_POINT ( 'NONE',  ( 0.000000000000000000, 0.000000000000000000, -99.99999999999998579 ) ) ;
#13026=CARTESIAN_POINT ( 'NONE',  ( -2.121150477449813534E-15, -11.54700538379251284, -26.37499999999997868 ) ) ;
#13029=CARTESIAN_POINT ( 'NONE',  ( 10.81189881249999729, 0.000000000000000000, -152.8437500020483810 ) ) ;
#13030=CARTESIAN_POINT ( 'NONE',  ( -5.405949406249996869, 9.363379034771805109, -164.3437500020484094 ) ) ;
#13033=CARTESIAN_POINT ( 'NONE',  ( -4.999999999999996447, 8.660254037844387298, -187.5000000000000000 ) ) ;
#13038=CARTESIAN_POINT ( 'NONE',  ( 5.405949406249999534, 9.363379034771803333, -190.0937500020483810 ) ) ;
#13040=CARTESIAN_POINT ( 'NONE',  ( -10.81189881249999907, -6.242252689847864744, -60.65625000204838813 ) ) ;
#13042=CARTESIAN_POINT ( 'NONE',  ( 9.999999999999998224, 0.000000000000000000, -111.4999999999999858 ) ) ;
#13044=AXIS2_PLACEMENT_3D ( 'NONE', #11298, #24492, #8085 ) ;
#13045=CARTESIAN_POINT ( 'NONE',  ( -10.81189881249999729, -6.242252689847864744, -138.6562500020484094 ) ) ;
#13046=CARTESIAN_POINT ( 'NONE',  ( -5.405949406249996869, 9.363379034771805109, -155.5312500020484094 ) ) ;
#13050=CARTESIAN_POINT ( 'NONE',  ( 10.81189881249999907, 6.242252689847868297, -86.71875000204836681 ) ) ;
#13053=CARTESIAN_POINT ( 'NONE',  ( 10.81189881249999907, 6.242252689847868297, -187.2187500020484094 ) ) ;
#13055=CARTESIAN_POINT ( 'NONE',  ( -9.999999999999742428, -5.773502691896402084, -117.0000000040967763 ) ) ;
#13057=CARTESIAN_POINT ( 'NONE',  ( -10.81189881249999729, 1.324075727343319199E-15, -87.78125000204838102 ) ) ;
#13059=CARTESIAN_POINT ( 'NONE',  ( 10.00000000000000000, 5.773502691896255534, -57.75000000409677625 ) ) ;
#13060=CARTESIAN_POINT ( 'NONE',  ( 5.405949406249999534, 9.363379034771803333, -19.09375000204835260 ) ) ;
#13063=CARTESIAN_POINT ( 'NONE',  ( -10.81189881249999907, -6.242252689847864744, -12.65625000204837036 ) ) ;
#13066=CYLINDRICAL_SURFACE ( 'NONE', #17609, 9.999999999999998224 ) ;
#13073=CARTESIAN_POINT ( 'NONE',  ( 4.999999999999992006, -8.660254037844389075, -153.7500000000000000 ) ) ;
#13083=CARTESIAN_POINT ( 'NONE',  ( 10.81189881249999729, 0.000000000000000000, -157.5312500020484094 ) ) ;
#13085=CARTESIAN_POINT ( 'NONE',  ( 7.070501591499376803E-16, 11.54700538379251284, -178.6250000000000000 ) ) ;
#13089=CARTESIAN_POINT ( 'NONE',  ( 10.81189881249999729, 0.000000000000000000, -76.34375000204838102 ) ) ;
#13090=CARTESIAN_POINT ( 'NONE',  ( -10.81189881249999729, 1.324075727343319199E-15, -87.78125000204838102 ) ) ;
#13093=CARTESIAN_POINT ( 'NONE',  ( 10.81189881249999729, 0.000000000000000000, -166.5312500020484094 ) ) ;
#13094=CARTESIAN_POINT ( 'NONE',  ( 7.644554776091147741E-16, 12.48450537969573659, -182.6562500020484094 ) ) ;
#13095=CONICAL_SURFACE ( 'NONE', #40669, 31.99999999999997158, 0.7853981633974447263 ) ;
#13097=CARTESIAN_POINT ( 'NONE',  ( -10.00000000000000000, -5.773502691896251982, -159.0000000040967905 ) ) ;
#13099=CARTESIAN_POINT ( 'NONE',  ( -10.81189881249999729, 6.242252689847871849, -5.218750002048355263 ) ) ;
#13101=CARTESIAN_POINT ( 'NONE',  ( -10.81189881249999729, 6.242252689847871849, -113.2187500020483952 ) ) ;
#13103=CARTESIAN_POINT ( 'NONE',  ( -2.293366432827344421E-15, -12.48450537969573659, -13.90625000204836859 ) ) ;
#13106=CARTESIAN_POINT ( 'NONE',  ( -5.405949406249996869, 9.363379034771805109, -109.0312500020483810 ) ) ;
#13109=CARTESIAN_POINT ( 'NONE',  ( 9.999999999999996447, -5.773502691896262640, -80.50000000409676204 ) ) ;
#13110=CARTESIAN_POINT ( 'NONE',  ( -10.00000000000051337, 5.773502691895962435, -145.7500000040967905 ) ) ;
#13111=CARTESIAN_POINT ( 'NONE',  ( -5.405949406250003975, -9.363379034771801557, -40.84375000204837391 ) ) ;
#13115=CARTESIAN_POINT ( 'NONE',  ( -2.121150477449813534E-15, -11.54700538379251284, -13.25000000409676204 ) ) ;
#13131=( BOUNDED_CURVE ( )  B_SPLINE_CURVE ( 2, ( #4665, #27981, #18034, #17596, #14355, #41109, #15219, #17816, #1655, #40901, #28418, #18248, #27763, #11549, #40686, #37904, #34464, #11771, #5103, #27552, #18466, #11987, #31011, #11126, #14575, #11343, #1440, #37686, #4886, #31439, #24329, #37248, #14785, #24758, #24973, #37470, #8348, #38114, #5315, #20849, #21499, #31654, #7914, #7697, #2089, #34033, #32498, #18676, #2927, #25596, #32077, #12823, #5744, #22140, #35315, #12609, #32288, #16056, #42391, #42604, #15844, #29247, #26014, #6164, #5526, #35101, #39166, #41760, #18897, #42183, #35736, #9599, #8765, #22351, #38753, #2712, #19106, #25182, #9393, #8974, #12194, #29044, #3133, #2512, #5956, #28838, #16262, #19304, #15636, #25803, #28628, #38960, #9180, #22773, #35934, #31874, #6374, #21921, #19518, #25385, #35527, #41970, #12403, #22558, #32703, #29461, #38324, #2305, #15430, #38532, #7424, #29889, #13448, #29677, #27070, #16903, #26224, #33553, #26429, #16477, #10016, #39792, #10225, #16693, #22987, #543, #13030, #30535, #20158, #33349, #32913, #36144, #753, #39580, #33764, #26644, #328, #3769, #121, #19942, #13875, #3345, #39372, #19731, #36354, #33131, #23412, #23839, #13242, #17332, #9809, #30104, #23194, #6787, #6575, #3558, #36561, #26853, #7007, #13661, #20364, #23630, #3978, #40007, #10438, #36774, #7212, #17118, #30318, #40213, #10645, #36988, #20575, #4187, #40416, #18193, #21437, #31385, #24702, #11717, #41279, #4401, #1603, #27710, #8290, #11500, #37192, #24914, #10860, #38060, #30742, #11287, #41056, #37848, #17759, #8502, #24051, #17541, #1172, #30954, #14296, #21654, #1386, #14517, #27495, #14946, #4828, #14080, #34621, #40629, #11071, #24272, #40848, #14733, #5048, #24482, #7641, #37419, #37634, #27925, #28146, #20792, #33979, #1820, #7861, #34836, #8073, #21223, #34408, #21010, #34199, #5259, #4616, #17974, #31174, #18411, #962, #27278, #28789, #19260, #35685, #22089, #25337, #15376, #8927, #28994, #8716, #9551, #12352, #5902, #9343, #41498, #28576, #38912, #2877, #15162, #41706, #35890, #6113, #16007, #35476, #25966, #22511, #25124, #32451, #32028, #38483, #29202, #12144, #35264, #5698, #19056, #38700, #42342, #12773, #39116, #25550, #18848, #2457, #22725, #15588, #6327, #9134, #18626, #31600, #2033, #2664, #28361, #11932, #32238, #41920, #22304, #15798, #38270, #42134, #21870, #35049, #12565, #25759, #5477, #31822, #2257, #40167, #33078, #36309, #10180, #36096, #26385, #20317, #9967, #26175, #13192, #29624, #6740, #23146, #16642, #7165, #23579, #26595, #6530, #30057, #39537, #16855, #39321, #10599, #282, #36517, #39959, #29414, #16426, #26808, #33511, #3085, #67, #23785, #36726, #3934, #23365, #27021, #19894, #32867, #10390, #3504, #29844, #17072, #13403, #39745, #6954, #20110, #33300, #30269, #708, #36940, #3725, #3299, #501, #16213, #19472, #13616, #13827, #42554, #32657, #12978, #9761, #22942, #19681, #4567, #20963, #14470, #1339, #7382, #34363, #33934, #24005, #27878, #27660, #4141, #24655, #41010, #37798, #31124, #40586, #40801, #10812, #8029, #34149, #14689, #17927, #916, #31342, #17282, #18146, #37145, #17709, #4779, #1557, #24221, #1772, #30487, #4357, #7593, #11242, #28101, #30691, #30904, #11027, #41229, #11455, #37372, #24441, #20747, #21173, #37584, #8243, #21391, #14031, #14902, #27227, #11666, #17498, #34574, #7815, #1124, #5005, #24867, #27450, #20528, #33716, #40371, #14247, #32402, #12098, #38436, #11884, #9287, #41867, #8460, #15749, #8669, #41448, #35003, #22042, #35214, #41662, #5211, #25502, #38015, #12716, #2408, #15539, #15114, #18367, #25710, #21823, #15958, #8879, #25291, #28741, #25080, #2199, #38860, #28309, #21611, #1988, #18583, #15333, #5644, #6063, #38225, #42294, #28530, #31771, #5432, #18793, #35424, #31982, #29155, #12305, #38651, #28948, #31555, #5851, #12517, #42085, #9086, #22254, #19006, #32191, #34790, #2618, #2825, #22459, #35636, #19213, #26335, #32815, #13565, #6484, #22889, #36048, #13355, #35843, #42499, #30220, #9503, #6901, #33248, #26756, #20054, #6275, #19421, #448, #12927, #19631, #233, #36465, #16803, #22672, #23096, #39487, #33025, #3246, #16590, #6689, #9920, #3675, #30002, #32612, #7117, #3037, #36676, #26122, #36259, #23310, #39908, #17, #20271, #16164, #39276, #29360, #13140, #16372, #33459, #19840, #3454, #9710, #10339, #29792, #39065, #23527, #29572, #26546, #39695, #10131, #3886, #17021, #659, #25913, #27178, #4304, #7763, #40531, #7332, #23735, #24390, #865, #1504, #17443, #20694, #24170, #4092, #23953, #37531, #37097, #20481, #10762, #40321, #33882, #30639, #1071, #7972, #14638, #7540, #14195, #13981, #27394, #4512, #33668, #31070, #10974, #37317, #27610, #10550, #20907, #14416, #21121, #26961, #34089, #27826, #11192, #34310, #13777, #17655, #30850, #40117, #36886, #17874, #1287, #40750, #4725, #17234, #30435, #13288, #19558, #26268, #13915, #35981, #33391, #16949, #40048, #3814, #10061, #23456, #32744, #39420, #30146, #23239, #165, #3181, #7258, #9854, #36604, #23670, #19773, #376, #33175, #16307, #29503, #13497, #30363, #32956, #585, #26893 ),
 .UNSPECIFIED., .F., .F. ) 
 B_SPLINE_CURVE_WITH_KNOTS ( ( 3, 2, 2, 2, 2, 2, 2, 2, 2, 2, 2, 2, 2, 2, 2, 2, 2, 2, 2, 2, 2, 2, 2, 2, 2, 2, 2, 2, 2, 2, 2, 2, 2, 2, 2, 2, 2, 2, 2, 2, 2, 2, 2, 2, 2, 2, 2, 2, 2, 2, 2, 2, 2, 2, 2, 2, 2, 2, 2, 2, 2, 2, 2, 2, 2, 2, 2, 2, 2, 2, 2, 2, 2, 2, 2, 2, 2, 2, 2, 2, 2, 2, 2, 2, 2, 2, 2, 2, 2, 2, 2, 2, 2, 2, 2, 2, 2, 2, 2, 2, 2, 2, 2, 2, 2, 2, 2, 2, 2, 2, 2, 2, 2, 2, 2, 2, 2, 2, 2, 2, 2, 2, 2, 2, 2, 2, 2, 2, 2, 2, 2, 2, 2, 2, 2, 2, 2, 2, 2, 2, 2, 2, 2, 2, 2, 2, 2, 2, 2, 2, 2, 2, 2, 2, 2, 2, 2, 2, 2, 2, 2, 2, 2, 2, 2, 2, 2, 2, 2, 2, 2, 2, 2, 2, 2, 2, 2, 2, 2, 2, 2, 2, 2, 2, 2, 2, 2, 2, 2, 2, 2, 2, 2, 2, 2, 2, 2, 2, 2, 2, 2, 2, 2, 2, 2, 2, 2, 2, 2, 2, 2, 2, 2, 2, 2, 2, 2, 2, 2, 2, 2, 2, 2, 2, 2, 2, 2, 2, 2, 2, 2, 2, 2, 2, 2, 2, 2, 2, 2, 2, 2, 2, 2, 2, 2, 2, 2, 2, 2, 2, 2, 2, 2, 2, 2, 2, 2, 2, 2, 2, 2, 2, 2, 2, 2, 2, 2, 2, 2, 2, 2, 2, 2, 2, 2, 2, 2, 2, 2, 2, 2, 2, 2, 2, 2, 2, 2, 2, 2, 2, 2, 2, 2, 2, 2, 2, 2, 2, 2, 2, 2, 2, 2, 2, 2, 2, 2, 2, 2, 2, 2, 2, 2, 2, 2, 2, 2, 2, 2, 2, 2, 3 ),
 ( 0.09624740578742232988, 0.09701492537313433084, 0.09825870646766168837, 0.09950248756218905977, 0.1007462686567164173, 0.1019900497512437748, 0.1032338308457711462, 0.1044776119402985037, 0.1057213930348258751, 0.1069651741293532327, 0.1082089552238805902, 0.1094527363184079616, 0.1106965174129353191, 0.1119402985074626905, 0.1131840796019900480, 0.1144278606965174194, 0.1156716417910447769, 0.1169154228855721345, 0.1181592039800995059, 0.1194029850746268634, 0.1206467661691542348, 0.1218905472636815923, 0.1231343283582089498, 0.1243781094527363212, 0.1256218905472636926, 0.1268656716417910502, 0.1281094527363184077, 0.1293532338308457652, 0.1305970149253731227, 0.1318407960199005080, 0.1330845771144278655, 0.1343283582089552231, 0.1355721393034825806, 0.1368159203980099381, 0.1380597014925373234, 0.1393034825870646809, 0.1405472636815920384, 0.1417910447761193959, 0.1430348258706467535, 0.1442786069651741387, 0.1455223880597014963, 0.1467661691542288538, 0.1480099502487562113, 0.1492537313432835688, 0.1504975124378109541, 0.1517412935323383116, 0.1529850746268656692, 0.1542288557213930267, 0.1554726368159203842, 0.1567164179104477695, 0.1579601990049751270, 0.1592039800995024845, 0.1604477611940298420, 0.1616915422885572273, 0.1629353233830845848, 0.1641791044776119424, 0.1654228855721392999, 0.1666666666666666574, 0.1679104477611940427, 0.1691542288557214002, 0.1703980099502487577, 0.1716417910447761153, 0.1728855721393034728, 0.1741293532338308581, 0.1753731343283582156, 0.1766169154228855731, 0.1778606965174129306, 0.1791044776119402882, 0.1803482587064676734, 0.1815920398009950310, 0.1828358208955223885, 0.1840796019900497460, 0.1853233830845771035, 0.1865671641791044888, 0.1878109452736318463, 0.1890547263681592038, 0.1902985074626865614, 0.1915422885572139189, 0.1927860696517413042, 0.1940298507462686617, 0.1952736318407960192, 0.1965174129353233767, 0.1977611940298507343, 0.1990049751243781195, 0.2002487562189054771, 0.2014925373134328346, 0.2027363184079601921, 0.2039800995024875496, 0.2052238805970149349, 0.2064676616915422924, 0.2077114427860696499, 0.2089552238805970075, 0.2101990049751243927, 0.2114427860696517503, 0.2126865671641791078, 0.2139303482587064653, 0.2151741293532338228, 0.2164179104477612081, 0.2176616915422885656, 0.2189054726368159232, 0.2201492537313432807, 0.2213930348258706382, 0.2226368159203980235, 0.2238805970149253810, 0.2251243781094527385, 0.2263681592039800961, 0.2276119402985074536, 0.2288557213930348389, 0.2300995024875621964, 0.2313432835820895539, 0.2325870646766169114, 0.2338308457711442689, 0.2350746268656716542, 0.2363184079601990117, 0.2375621890547263693, 0.2388059701492537268, 0.2400497512437810843, 0.2412935323383084696, 0.2425373134328358271, 0.2437810945273631846, 0.2450248756218905422, 0.2462686567164178997, 0.2475124378109452850, 0.2487562189054726425, 0.2500000000000000000, 0.2512437810945273853, 0.2524875621890547150, 0.2537313432835821003, 0.2549751243781094301, 0.2562189054726368154, 0.2574626865671642006, 0.2587064676616915304, 0.2599502487562189157, 0.2611940298507462455, 0.2624378109452736307, 0.2636815920398010160, 0.2649253731343283458, 0.2661691542288557311, 0.2674129353233830608, 0.2686567164179104461, 0.2699004975124378314, 0.2711442786069651611, 0.2723880597014925464, 0.2736318407960198762, 0.2748756218905472615, 0.2761194029850746468, 0.2773631840796019765, 0.2786069651741293618, 0.2798507462686566916, 0.2810945273631840768, 0.2823383084577114621, 0.2835820895522387919, 0.2848258706467661772, 0.2860696517412935069, 0.2873134328358208922, 0.2885572139303482775, 0.2898009950248756073, 0.2910447761194029925, 0.2922885572139303223, 0.2935323383084577076, 0.2947761194029850929, 0.2960199004975124226, 0.2972636815920398079, 0.2985074626865671377, 0.2997512437810945229, 0.3009950248756219082, 0.3022388059701492380, 0.3034825870646766233, 0.3047263681592039530, 0.3059701492537313383, 0.3072139303482587236, 0.3084577114427860534, 0.3097014925373134386, 0.3109452736318407684, 0.3121890547263681537, 0.3134328358208955390, 0.3146766169154228687, 0.3159203980099502540, 0.3171641791044776393, 0.3184079601990049690, 0.3196517412935323543, 0.3208955223880596841, 0.3221393034825870694, 0.3233830845771144546, 0.3246268656716417844, 0.3258706467661691697, 0.3271144278606964995, 0.3283582089552238847, 0.3296019900497512700, 0.3308457711442785998, 0.3320895522388059851, 0.3333333333333333148, 0.3345771144278607001, 0.3358208955223880854, 0.3370646766169154152, 0.3383084577114428004, 0.3395522388059701302, 0.3407960199004975155, 0.3420398009950249008, 0.3432835820895522305, 0.3445273631840796158, 0.3457711442786069456, 0.3470149253731342753, 0.3482587064676616606, 0.3495024875621890459, 0.3507462686567164312, 0.3519900497512437054, 0.3532338308457710907, 0.3544776119402984760, 0.3557213930348258613, 0.3569651741293532465, 0.3582089552238805208, 0.3594527363184079061, 0.3606965174129352913, 0.3619402985074626766, 0.3631840796019900619, 0.3644278606965173362, 0.3656716417910447214, 0.3669154228855721067, 0.3681592039800994920, 0.3694029850746268773, 0.3706467661691541515, 0.3718905472636815368, 0.3731343283582089221, 0.3743781094527363074, 0.3756218905472636926, 0.3768656716417909669, 0.3781094527363183522, 0.3793532338308457375, 0.3805970149253731227, 0.3818407960199005080, 0.3830845771144277823, 0.3843283582089551675, 0.3855721393034825528, 0.3868159203980099381, 0.3880597014925373234, 0.3893034825870645976, 0.3905472636815919829, 0.3917910447761193682, 0.3930348258706467535, 0.3942786069651741387, 0.3955223880597014130, 0.3967661691542287983, 0.3980099502487561836, 0.3992537313432835688, 0.4004975124378109541, 0.4017412935323382284, 0.4029850746268656136, 0.4042288557213929989, 0.4054726368159203842, 0.4067164179104477695, 0.4079601990049750437, 0.4092039800995024290, 0.4104477611940299253, 0.4116915422885571996, 0.4129353233830845848, 0.4141791044776118591, 0.4154228855721392444, 0.4166666666666666297, 0.4179104477611940149, 0.4191542288557214002, 0.4203980099502486745, 0.4216417910447760597, 0.4228855721393034450, 0.4241293532338308303, 0.4253731343283582156, 0.4266169154228854898, 0.4278606965174128751, 0.4291044776119402604, 0.4303482587064677567, 0.4315920398009950310, 0.4328358208955223052, 0.4340796019900496905, 0.4353233830845770758, 0.4365671641791044610, 0.4378109452736318463, 0.4390547263681592316, 0.4402985074626865059, 0.4415422885572138911, 0.4427860696517413874, 0.4440298507462686617, 0.4452736318407960470, 0.4465174129353233212, 0.4477611940298507065, 0.4490049751243780918, 0.4502487562189054771, 0.4514925373134328623, 0.4527363184079601366, 0.4539800995024875219, 0.4552238805970150182, 0.4564676616915422924, 0.4577114427860696777, 0.4589552238805969520, 0.4601990049751243372, 0.4614427860696517225, 0.4626865671641791078, 0.4639303482587064931, 0.4651741293532337673, 0.4664179104477611526, 0.4676616915422885379, 0.4689054726368159232, 0.4701492537313433084, 0.4713930348258705827, 0.4726368159203979680, 0.4738805970149253532, 0.4751243781094528496, 0.4763681592039801238, 0.4776119402985073981, 0.4788557213930347833, 0.4800995024875621686, 0.4813432835820895539, 0.4825870646766169392, 0.4838308457711442134, 0.4850746268656715987, 0.4863184079601989840, 0.4875621890547264803, 0.4888059701492537545, 0.4900497512437810288, 0.4912935323383084141, 0.4925373134328357994, 0.4937810945273631846, 0.4942573560361783747 ),
 .UNSPECIFIED. ) 
 CURVE ( )  GEOMETRIC_REPRESENTATION_ITEM ( )  RATIONAL_B_SPLINE_CURVE ( ( 0.9366860366984448572, 0.9173261862270272182, 1.000000000000000000, 0.8660254037844387076, 1.000000000000000000, 0.8660254037844387076, 1.000000000000000000, 0.8660254037844387076, 1.000000000000000000, 0.8660254037844387076, 1.000000000000000000, 0.8660254037844387076, 1.000000000000000000, 0.8660254037844387076, 1.000000000000000000, 0.8660254037844387076, 1.000000000000000000, 0.8660254037844387076, 1.000000000000000000, 0.8660254037844387076, 1.000000000000000000, 0.8660254037844387076, 1.000000000000000000, 0.8660254037844387076, 1.000000000000000000, 0.8660254037844387076, 1.000000000000000000, 0.8660254037844387076, 1.000000000000000000, 0.8660254037844387076, 1.000000000000000000, 0.8660254037844387076, 1.000000000000000000, 0.8660254037844387076, 1.000000000000000000, 0.8660254037844387076, 1.000000000000000000, 0.8660254037844387076, 1.000000000000000000, 0.8660254037844387076, 1.000000000000000000, 0.8660254037844387076, 1.000000000000000000, 0.8660254037844387076, 1.000000000000000000, 0.8660254037844387076, 1.000000000000000000, 0.8660254037844387076, 1.000000000000000000, 0.8660254037844387076, 1.000000000000000000, 0.8660254037844387076, 1.000000000000000000, 0.8660254037844387076, 1.000000000000000000, 0.8660254037844387076, 1.000000000000000000, 0.8660254037844387076, 1.000000000000000000, 0.8660254037844387076, 1.000000000000000000, 0.8660254037844387076, 1.000000000000000000, 0.8660254037844387076, 1.000000000000000000, 0.8660254037844387076, 1.000000000000000000, 0.8660254037844387076, 1.000000000000000000, 0.8660254037844387076, 1.000000000000000000, 0.8660254037844387076, 1.000000000000000000, 0.8660254037844387076, 1.000000000000000000, 0.8660254037844387076, 1.000000000000000000, 0.8660254037844387076, 1.000000000000000000, 0.8660254037844387076, 1.000000000000000000, 0.8660254037844387076, 1.000000000000000000, 0.8660254037844387076, 1.000000000000000000, 0.8660254037844387076, 1.000000000000000000, 0.8660254037844387076, 1.000000000000000000, 0.8660254037844387076, 1.000000000000000000, 0.8660254037844387076, 1.000000000000000000, 0.8660254037844387076, 1.000000000000000000, 0.8660254037844387076, 1.000000000000000000, 0.8660254037844387076, 1.000000000000000000, 0.8660254037844387076, 1.000000000000000000, 0.8660254037844387076, 1.000000000000000000, 0.8660254037844387076, 1.000000000000000000, 0.8660254037844387076, 1.000000000000000000, 0.8660254037844387076, 1.000000000000000000, 0.8660254037844387076, 1.000000000000000000, 0.8660254037844387076, 1.000000000000000000, 0.8660254037844387076, 1.000000000000000000, 0.8660254037844387076, 1.000000000000000000, 0.8660254037844387076, 1.000000000000000000, 0.8660254037844387076, 1.000000000000000000, 0.8660254037844387076, 1.000000000000000000, 0.8660254037844387076, 1.000000000000000000, 0.8660254037844387076, 1.000000000000000000, 0.8660254037844387076, 1.000000000000000000, 0.8660254037844387076, 1.000000000000000000, 0.8660254037844387076, 1.000000000000000000, 0.8660254037844387076, 1.000000000000000000, 0.8660254037844387076, 1.000000000000000000, 0.8660254037844387076, 1.000000000000000000, 0.8660254037844387076, 1.000000000000000000, 0.8660254037844387076, 1.000000000000000000, 0.8660254037844387076, 1.000000000000000000, 0.8660254037844387076, 1.000000000000000000, 0.8660254037844387076, 1.000000000000000000, 0.8660254037844387076, 1.000000000000000000, 0.8660254037844387076, 1.000000000000000000, 0.8660254037844387076, 1.000000000000000000, 0.8660254037844387076, 1.000000000000000000, 0.8660254037844387076, 1.000000000000000000, 0.8660254037844387076, 1.000000000000000000, 0.8660254037844387076, 1.000000000000000000, 0.8660254037844387076, 1.000000000000000000, 0.8660254037844387076, 1.000000000000000000, 0.8660254037844387076, 1.000000000000000000, 0.8660254037844387076, 1.000000000000000000, 0.8660254037844387076, 1.000000000000000000, 0.8660254037844387076, 1.000000000000000000, 0.8660254037844387076, 1.000000000000000000, 0.8660254037844387076, 1.000000000000000000, 0.8660254037844387076, 1.000000000000000000, 0.8660254037844387076, 1.000000000000000000, 0.8660254037844387076, 1.000000000000000000, 0.8660254037844387076, 1.000000000000000000, 0.8660254037844387076, 1.000000000000000000, 0.8660254037844387076, 1.000000000000000000, 0.8660254037844387076, 1.000000000000000000, 0.8660254037844387076, 1.000000000000000000, 0.8660254037844387076, 1.000000000000000000, 0.8660254037844387076, 1.000000000000000000, 0.8660254037844387076, 1.000000000000000000, 0.8660254037844387076, 1.000000000000000000, 0.8660254037844387076, 1.000000000000000000, 0.8660254037844387076, 1.000000000000000000, 0.8660254037844387076, 1.000000000000000000, 0.8660254037844387076, 1.000000000000000000, 0.8660254037844387076, 1.000000000000000000, 0.8660254037844387076, 1.000000000000000000, 0.8660254037844387076, 1.000000000000000000, 0.8660254037844387076, 1.000000000000000000, 0.8660254037844387076, 1.000000000000000000, 0.8660254037844387076, 1.000000000000000000, 0.8660254037844387076, 1.000000000000000000, 0.8660254037844387076, 1.000000000000000000, 0.8660254037844387076, 1.000000000000000000, 0.8660254037844387076, 1.000000000000000000, 0.8660254037844387076, 1.000000000000000000, 0.8660254037844387076, 1.000000000000000000, 0.8660254037844387076, 1.000000000000000000, 0.8660254037844387076, 1.000000000000000000, 0.8660254037844387076, 1.000000000000000000, 0.8660254037844387076, 1.000000000000000000, 0.8660254037844387076, 1.000000000000000000, 0.8660254037844387076, 1.000000000000000000, 0.8660254037844387076, 1.000000000000000000, 0.8660254037844387076, 1.000000000000000000, 0.8660254037844387076, 1.000000000000000000, 0.8660254037844387076, 1.000000000000000000, 0.8660254037844387076, 1.000000000000000000, 0.8660254037844387076, 1.000000000000000000, 0.8660254037844387076, 1.000000000000000000, 0.8660254037844387076, 1.000000000000000000, 0.8660254037844387076, 1.000000000000000000, 0.8660254037844387076, 1.000000000000000000, 0.8660254037844387076, 1.000000000000000000, 0.8660254037844387076, 1.000000000000000000, 0.8660254037844387076, 1.000000000000000000, 0.8660254037844387076, 1.000000000000000000, 0.8660254037844387076, 1.000000000000000000, 0.8660254037844387076, 1.000000000000000000, 0.8660254037844387076, 1.000000000000000000, 0.8660254037844387076, 1.000000000000000000, 0.8660254037844387076, 1.000000000000000000, 0.8660254037844387076, 1.000000000000000000, 0.8660254037844387076, 1.000000000000000000, 0.8660254037844387076, 1.000000000000000000, 0.8660254037844387076, 1.000000000000000000, 0.8660254037844387076, 1.000000000000000000, 0.8660254037844387076, 1.000000000000000000, 0.8660254037844387076, 1.000000000000000000, 0.8660254037844387076, 1.000000000000000000, 0.8660254037844387076, 1.000000000000000000, 0.8660254037844387076, 1.000000000000000000, 0.8660254037844387076, 1.000000000000000000, 0.8660254037844387076, 1.000000000000000000, 0.8660254037844387076, 1.000000000000000000, 0.8660254037844387076, 1.000000000000000000, 0.8660254037844387076, 1.000000000000000000, 0.8660254037844387076, 1.000000000000000000, 0.8660254037844387076, 1.000000000000000000, 0.8660254037844387076, 1.000000000000000000, 0.8660254037844387076, 1.000000000000000000, 0.8660254037844387076, 1.000000000000000000, 0.8660254037844387076, 1.000000000000000000, 0.8660254037844387076, 1.000000000000000000, 0.8660254037844387076, 1.000000000000000000, 0.8660254037844387076, 1.000000000000000000, 0.8660254037844387076, 1.000000000000000000, 0.8660254037844387076, 1.000000000000000000, 0.8660254037844387076, 1.000000000000000000, 0.8660254037844387076, 1.000000000000000000, 0.8660254037844387076, 1.000000000000000000, 0.8660254037844387076, 1.000000000000000000, 0.8660254037844387076, 1.000000000000000000, 0.8660254037844387076, 1.000000000000000000, 0.8660254037844387076, 1.000000000000000000, 0.8660254037844387076, 1.000000000000000000, 0.8660254037844387076, 1.000000000000000000, 0.8660254037844387076, 1.000000000000000000, 0.8660254037844387076, 1.000000000000000000, 0.8660254037844387076, 1.000000000000000000, 0.8660254037844387076, 1.000000000000000000, 0.8660254037844387076, 1.000000000000000000, 0.8660254037844387076, 1.000000000000000000, 0.8660254037844387076, 1.000000000000000000, 0.8660254037844387076, 1.000000000000000000, 0.8660254037844387076, 1.000000000000000000, 0.8660254037844387076, 1.000000000000000000, 0.8660254037844387076, 1.000000000000000000, 0.8660254037844387076, 1.000000000000000000, 0.8660254037844387076, 1.000000000000000000, 0.8660254037844387076, 1.000000000000000000, 0.8660254037844387076, 1.000000000000000000, 0.8660254037844387076, 1.000000000000000000, 0.8660254037844387076, 1.000000000000000000, 0.8660254037844387076, 1.000000000000000000, 0.8660254037844387076, 1.000000000000000000, 0.8660254037844387076, 1.000000000000000000, 0.8660254037844387076, 1.000000000000000000, 0.8660254037844387076, 1.000000000000000000, 0.8660254037844387076, 1.000000000000000000, 0.8660254037844387076, 1.000000000000000000, 0.8660254037844387076, 1.000000000000000000, 0.8660254037844387076, 1.000000000000000000, 0.8660254037844387076, 1.000000000000000000, 0.8660254037844387076, 1.000000000000000000, 0.8660254037844387076, 1.000000000000000000, 0.8660254037844387076, 1.000000000000000000, 0.8660254037844387076, 1.000000000000000000, 0.8660254037844387076, 1.000000000000000000, 0.8660254037844387076, 1.000000000000000000, 0.8660254037844387076, 1.000000000000000000, 0.8660254037844387076, 1.000000000000000000, 0.8660254037844387076, 1.000000000000000000, 0.8660254037844387076, 1.000000000000000000, 0.8660254037844387076, 1.000000000000000000, 0.8660254037844387076, 1.000000000000000000, 0.8660254037844387076, 1.000000000000000000, 0.8660254037844387076, 1.000000000000000000, 0.8660254037844387076, 1.000000000000000000, 0.8660254037844387076, 1.000000000000000000, 0.8660254037844387076, 1.000000000000000000, 0.8660254037844387076, 1.000000000000000000, 0.8660254037844387076, 1.000000000000000000, 0.8660254037844387076, 1.000000000000000000, 0.8660254037844387076, 1.000000000000000000, 0.8660254037844387076, 1.000000000000000000, 0.8660254037844387076, 1.000000000000000000, 0.8660254037844387076, 1.000000000000000000, 0.8660254037844387076, 1.000000000000000000, 0.8660254037844387076, 1.000000000000000000, 0.8660254037844387076, 1.000000000000000000, 0.8660254037844387076, 1.000000000000000000, 0.8660254037844387076, 1.000000000000000000, 0.8660254037844387076, 1.000000000000000000, 0.8660254037844387076, 1.000000000000000000, 0.8660254037844387076, 1.000000000000000000, 0.8660254037844387076, 1.000000000000000000, 0.8660254037844387076, 1.000000000000000000, 0.8660254037844387076, 1.000000000000000000, 0.8660254037844387076, 1.000000000000000000, 0.8660254037844387076, 1.000000000000000000, 0.8660254037844387076, 1.000000000000000000, 0.8660254037844387076, 1.000000000000000000, 0.8660254037844387076, 1.000000000000000000, 0.8660254037844387076, 1.000000000000000000, 0.8660254037844387076, 1.000000000000000000, 0.8660254037844387076, 1.000000000000000000, 0.8660254037844387076, 1.000000000000000000, 0.8660254037844387076, 1.000000000000000000, 0.8660254037844387076, 1.000000000000000000, 0.8660254037844387076, 1.000000000000000000, 0.8660254037844387076, 1.000000000000000000, 0.8660254037844387076, 1.000000000000000000, 0.8660254037844387076, 1.000000000000000000, 0.8660254037844387076, 1.000000000000000000, 0.8660254037844387076, 1.000000000000000000, 0.8660254037844387076, 1.000000000000000000, 0.8660254037844387076, 1.000000000000000000, 0.8660254037844387076, 1.000000000000000000, 0.8660254037844387076, 1.000000000000000000, 0.8660254037844387076, 1.000000000000000000, 0.8660254037844387076, 1.000000000000000000, 0.8660254037844387076, 1.000000000000000000, 0.8660254037844387076, 1.000000000000000000, 0.8660254037844387076, 1.000000000000000000, 0.8660254037844387076, 1.000000000000000000, 0.8660254037844387076, 1.000000000000000000, 0.8660254037844387076, 1.000000000000000000, 0.8660254037844387076, 1.000000000000000000, 0.8660254037844387076, 1.000000000000000000, 0.8660254037844387076, 1.000000000000000000, 0.8660254037844387076, 1.000000000000000000, 0.8660254037844387076, 1.000000000000000000, 0.8660254037844387076, 1.000000000000000000, 0.8660254037844387076, 1.000000000000000000, 0.8660254037844387076, 1.000000000000000000, 0.8660254037844387076, 1.000000000000000000, 0.8660254037844387076, 1.000000000000000000, 0.8660254037844387076, 1.000000000000000000, 0.8660254037844387076, 1.000000000000000000, 0.8660254037844387076, 1.000000000000000000, 0.8660254037844387076, 1.000000000000000000, 0.8660254037844387076, 1.000000000000000000, 0.8660254037844387076, 1.000000000000000000, 0.8660254037844387076, 1.000000000000000000, 0.8660254037844387076, 1.000000000000000000, 0.8660254037844387076, 1.000000000000000000, 0.8660254037844387076, 1.000000000000000000, 0.8660254037844387076, 1.000000000000000000, 0.8660254037844387076, 1.000000000000000000, 0.8660254037844387076, 1.000000000000000000, 0.8660254037844387076, 1.000000000000000000, 0.8660254037844387076, 1.000000000000000000, 0.8660254037844387076, 1.000000000000000000, 0.8660254037844387076, 1.000000000000000000, 0.8660254037844387076, 1.000000000000000000, 0.8660254037844387076, 1.000000000000000000, 0.8660254037844387076, 1.000000000000000000, 0.8660254037844387076, 1.000000000000000000, 0.8660254037844387076, 1.000000000000000000, 0.8660254037844387076, 1.000000000000000000, 0.8660254037844387076, 1.000000000000000000, 0.8660254037844387076, 1.000000000000000000, 0.8660254037844387076, 1.000000000000000000, 0.8660254037844387076, 1.000000000000000000, 0.8660254037844387076, 1.000000000000000000, 0.8660254037844387076, 1.000000000000000000, 0.8660254037844387076, 1.000000000000000000, 0.8660254037844387076, 1.000000000000000000, 0.8660254037844387076, 1.000000000000000000, 0.8660254037844387076, 1.000000000000000000, 0.8660254037844387076, 1.000000000000000000, 0.8660254037844387076, 1.000000000000000000, 0.8660254037844387076, 1.000000000000000000, 0.8660254037844387076, 1.000000000000000000, 0.8660254037844387076, 1.000000000000000000, 0.8660254037844387076, 1.000000000000000000, 0.8660254037844387076, 1.000000000000000000, 0.8660254037844387076, 1.000000000000000000, 0.8660254037844387076, 1.000000000000000000, 0.9486992175574255892, 0.9366860366984515185 ) ) 
 REPRESENTATION_ITEM ( '' )  );
#13132=CARTESIAN_POINT ( 'NONE',  ( -10.81189881249999729, 6.242252689847871849, -180.9062500020484094 ) ) ;
#13134=CARTESIAN_POINT ( 'NONE',  ( -2.121150477449813534E-15, -11.54700538379251284, -146.7500000040967905 ) ) ;
#13136=CARTESIAN_POINT ( 'NONE',  ( -5.405949406249996869, 9.363379034771805109, -99.84375000204838102 ) ) ;
#13138=CARTESIAN_POINT ( 'NONE',  ( -5.405949406250003975, -9.363379034771801557, -110.0312500020483810 ) ) ;
#13140=CARTESIAN_POINT ( 'NONE',  ( 5.405949406249992428, -9.363379034771808662, -112.5937500020483810 ) ) ;
#13143=CARTESIAN_POINT ( 'NONE',  ( 9.999999999999998224, 0.000000000000000000, -114.4999999999999858 ) ) ;
#13144=CARTESIAN_POINT ( 'NONE',  ( -9.999999999999998224, 1.224646799147353059E-15, -140.7500000000000000 ) ) ;
#13145=CARTESIAN_POINT ( 'NONE',  ( -10.00000000000000000, -5.773502691896251982, -7.124999999999964473 ) ) ;
#13148=CARTESIAN_POINT ( 'NONE',  ( 4.999999999999992006, -8.660254037844389075, -179.6250000040968189 ) ) ;
#13150=CARTESIAN_POINT ( 'NONE',  ( 5.405949406249992428, -9.363379034771808662, -30.09375000204836326 ) ) ;
#13151=CARTESIAN_POINT ( 'NONE',  ( 4.999999999999992006, -8.660254037844389075, -105.7499999999999858 ) ) ;
#13152=CARTESIAN_POINT ( 'NONE',  ( -5.405949406250003975, -9.363379034771801557, -141.3437500020483810 ) ) ;
#13154=CARTESIAN_POINT ( 'NONE',  ( 10.81189881249999729, 0.000000000000000000, -34.53125000204837391 ) ) ;
#13156=CARTESIAN_POINT ( 'NONE',  ( 7.070501591499377789E-16, 11.54700538379251284, -64.62499999999998579 ) ) ;
#13157=CARTESIAN_POINT ( 'NONE',  ( -5.405949406249996869, 9.363379034771805109, -134.5312500020484094 ) ) ;
#13159=ORIENTED_EDGE ( 'NONE', *, *, #5686, .F. ) ;
#13161=CARTESIAN_POINT ( 'NONE',  ( 4.999999999999992006, -8.660254037844389075, -128.2499999999999716 ) ) ;
#13162=CARTESIAN_POINT ( 'NONE',  ( 9.999999999999996447, -5.773502691896262640, -112.0000000040967763 ) ) ;
#13163=CARTESIAN_POINT ( 'NONE',  ( 10.00000000000076916, -5.773502691895816774, -107.1249999999999574 ) ) ;
#13164=CARTESIAN_POINT ( 'NONE',  ( 7.644554776091147741E-16, 12.48450537969573659, -63.96875000204837391 ) ) ;
#13171=CARTESIAN_POINT ( 'NONE',  ( -4.999999999999996447, 8.660254037844387298, -34.87500000409676915 ) ) ;
#13172=LINE ( 'NONE', #6932, #24550 ) ;
#13179=ORIENTED_EDGE ( 'NONE', *, *, #11626, .F. ) ;
#13185=CARTESIAN_POINT ( 'NONE',  ( 9.999999999999479527, 5.773502691896553074, -144.7500000040967620 ) ) ;
#13188=CARTESIAN_POINT ( 'NONE',  ( -5.000000000000003553, -8.660254037844383745, -116.4999999999999858 ) ) ;
#13189=CARTESIAN_POINT ( 'NONE',  ( -10.81189881249999729, 6.242252689847871849, -129.7187500020483810 ) ) ;
#13190=CARTESIAN_POINT ( 'NONE',  ( -2.293366432827344421E-15, -12.48450537969573659, -129.4062500020483810 ) ) ;
#13192=CARTESIAN_POINT ( 'NONE',  ( -2.293366432827344421E-15, -12.48450537969573659, -141.2187500020483810 ) ) ;
#13194=CARTESIAN_POINT ( 'NONE',  ( 9.999999999999998224, 0.000000000000000000, -102.5000000000000000 ) ) ;
#13195=CARTESIAN_POINT ( 'NONE',  ( -4.999999999999996447, 8.660254037844387298, -162.0000000000000000 ) ) ;
#13199=CARTESIAN_POINT ( 'NONE',  ( 10.81189881249999729, 0.000000000000000000, -53.84375000204835970 ) ) ;
#13201=CARTESIAN_POINT ( 'NONE',  ( 7.644554776091147741E-16, 12.48450537969573659, -161.4687500020484094 ) ) ;
#13206=CARTESIAN_POINT ( 'NONE',  ( 9.999999999999998224, 0.000000000000000000, -88.99999999999998579 ) ) ;
#13208=CARTESIAN_POINT ( 'NONE',  ( 10.81189881249999729, 6.242252689847867408, -107.9062500020483952 ) ) ;
#13209=CARTESIAN_POINT ( 'NONE',  ( 5.000000000000000000, 8.660254037844385522, -129.6250000040967620 ) ) ;
#13213=CYLINDRICAL_SURFACE ( 'NONE', #7669, 9.999999999999998224 ) ;
#13214=CARTESIAN_POINT ( 'NONE',  ( -10.81189881249999729, 1.324075727343319199E-15, -60.78125000204836681 ) ) ;
#13219=CARTESIAN_POINT ( 'NONE',  ( 9.999999999999998224, 0.000000000000000000, -105.8750000040967763 ) ) ;
#13221=EDGE_CURVE ( 'NONE', #33014, #3489, #9213, .T. ) ;
#13225=CARTESIAN_POINT ( 'NONE',  ( -9.999999999999998224, 0.000000000000000000, -99.99999999999998579 ) ) ;
#13237=CARTESIAN_POINT ( 'NONE',  ( 5.000000000000000000, 8.660254037844385522, -25.74999999999996803 ) ) ;
#13241=CARTESIAN_POINT ( 'NONE',  ( 10.81189881249999551, -6.242252689847874514, -152.9687500020484094 ) ) ;
#13242=CARTESIAN_POINT ( 'NONE',  ( 5.405949406249999534, 9.363379034771803333, -161.5937500020484094 ) ) ;
#13245=CARTESIAN_POINT ( 'NONE',  ( 10.00000000000000000, 5.773502691896255534, -187.8750000000000568 ) ) ;
#13247=CARTESIAN_POINT ( 'NONE',  ( -9.999999999999998224, 1.224646799147353059E-15, -137.7499999999999716 ) ) ;
#13250=CARTESIAN_POINT ( 'NONE',  ( 7.644554776091147741E-16, 12.48450537969573659, -186.9687500020483810 ) ) ;
#13251=EDGE_CURVE ( 'NONE', #23032, #34857, #19411, .T. ) ;
#13253=CARTESIAN_POINT ( 'NONE',  ( -5.405949406250003975, -9.363379034771801557, -50.03125000204838813 ) ) ;
#13255=CARTESIAN_POINT ( 'NONE',  ( -9.999999999999998224, 1.224646799147353059E-15, -113.7499999999999858 ) ) ;
#13257=CARTESIAN_POINT ( 'NONE',  ( -5.405949406250003975, -9.363379034771801557, -146.0312500020483810 ) ) ;
#13258=CARTESIAN_POINT ( 'NONE',  ( 5.405949406249999534, 9.363379034771803333, -160.2812500020484094 ) ) ;
#13262=CARTESIAN_POINT ( 'NONE',  ( 7.644554776091147741E-16, 12.48450537969573659, -92.46875000204838102 ) ) ;
#13265=CARTESIAN_POINT ( 'NONE',  ( 5.405949406249999534, 9.363379034771803333, -185.5937500020483810 ) ) ;
#13268=CARTESIAN_POINT ( 'NONE',  ( 5.405949406249999534, 9.363379034771803333, -80.78125000204838102 ) ) ;
#13271=CARTESIAN_POINT ( 'NONE',  ( -9.999999999999998224, 1.224646799147353059E-15, -58.62500000409676204 ) ) ;
#13272=CARTESIAN_POINT ( 'NONE',  ( 5.405949406249992428, -9.363379034771808662, -18.09375000204835260 ) ) ;
#13274=CARTESIAN_POINT ( 'NONE',  ( -10.81189881249999907, -6.242252689847864744, -11.15625000204836859 ) ) ;
#13288=CARTESIAN_POINT ( 'NONE',  ( 5.405949406249992428, -9.363379034771808662, -103.5937500020483668 ) ) ;
#13299=DIRECTION ( 'NONE',  ( -0.000000000000000000, -0.000000000000000000, -1.000000000000000000 ) ) ;
#13300=CARTESIAN_POINT ( 'NONE',  ( -5.405949406250003975, -9.363379034771801557, -149.0312500020483810 ) ) ;
#13307=CARTESIAN_POINT ( 'NONE',  ( 7.644554776091147741E-16, 12.48450537969573659, -80.46875000204838102 ) ) ;
#13308=CARTESIAN_POINT ( 'NONE',  ( -10.81189881249999729, 1.324075727343319199E-15, -81.78125000204839523 ) ) ;
#13311=CARTESIAN_POINT ( 'NONE',  ( -10.81189881249999729, 6.242252689847871849, -165.9062500020483810 ) ) ;
#13312=CARTESIAN_POINT ( 'NONE',  ( -5.405949406250003975, -9.363379034771801557, -180.5312500020483810 ) ) ;
#13313=CARTESIAN_POINT ( 'NONE',  ( 9.999999999999998224, 0.000000000000000000, -158.3750000040967905 ) ) ;
#13315=CARTESIAN_POINT ( 'NONE',  ( 7.644554776091147741E-16, 12.48450537969573659, -5.468750002048355263 ) ) ;
#13317=CARTESIAN_POINT ( 'NONE',  ( 10.81189881249999907, 6.242252689847868297, -112.2187500020483810 ) ) ;
#13319=CARTESIAN_POINT ( 'NONE',  ( -10.81189881249999729, 6.242252689847871849, -14.40625000204837036 ) ) ;
#13322=CARTESIAN_POINT ( 'NONE',  ( 5.405949406249999534, 9.363379034771803333, -110.7812500020483810 ) ) ;
#13325=CARTESIAN_POINT ( 'NONE',  ( -4.999999999999996447, 8.660254037844387298, -84.37500000409677625 ) ) ;
#13327=CARTESIAN_POINT ( 'NONE',  ( -2.293366432827344421E-15, -12.48450537969573659, -42.21875000204835970 ) ) ;
#13328=ORIENTED_EDGE ( 'NONE', *, *, #28926, .F. ) ;
#13332=CARTESIAN_POINT ( 'NONE',  ( 9.999999999999996447, -5.773502691896262640, -8.500000004096758488 ) ) ;
#13334=CARTESIAN_POINT ( 'NONE',  ( -2.121150477449813534E-15, -11.54700538379251284, -155.7500000040968189 ) ) ;
#13338=ORIENTED_EDGE ( 'NONE', *, *, #13221, .F. ) ;
#13345=( BOUNDED_CURVE ( )  B_SPLINE_CURVE ( 2, ( #15128, #2421, #15345, #5865, #38450, #31355, #18597 ),
 .UNSPECIFIED., .F., .F. ) 
 B_SPLINE_CURVE_WITH_KNOTS ( ( 3, 2, 2, 3 ),
 ( 0.3134328358208955390, 0.3146766169154229242, 0.3159203980099503650, 0.3171641791044778058 ),
 .UNSPECIFIED. ) 
 CURVE ( )  GEOMETRIC_REPRESENTATION_ITEM ( )  RATIONAL_B_SPLINE_CURVE ( ( 1.000000000000000000, 0.8660254037844387076, 1.000000000000000000, 0.8660254037844387076, 1.000000000000000000, 0.8660254037844207220, 1.000000000000017986 ) ) 
 REPRESENTATION_ITEM ( '' )  );
#13348=CARTESIAN_POINT ( 'NONE',  ( -10.81189881249999729, 6.242252689847871849, -177.9062500020484094 ) ) ;
#13351=CARTESIAN_POINT ( 'NONE',  ( -5.405949406249996869, 9.363379034771805109, -101.3437500020483810 ) ) ;
#13353=CARTESIAN_POINT ( 'NONE',  ( -2.293366432827344421E-15, -12.48450537969573659, -109.9062500020483952 ) ) ;
#13355=CARTESIAN_POINT ( 'NONE',  ( -10.81189881249999729, 1.324075727343319199E-15, -117.5937500020483810 ) ) ;
#13358=CARTESIAN_POINT ( 'NONE',  ( 9.999999999999998224, 0.000000000000000000, -134.3750000040967905 ) ) ;
#13359=CARTESIAN_POINT ( 'NONE',  ( -2.121150477449813534E-15, -11.54700538379251284, -131.3750000000000000 ) ) ;
#13360=CARTESIAN_POINT ( 'NONE',  ( 9.999999999999998224, 0.000000000000000000, -4.999999999999976907 ) ) ;
#13363=CARTESIAN_POINT ( 'NONE',  ( 10.00000000000000000, 5.773502691896255534, -179.2500000040967905 ) ) ;
#13365=CARTESIAN_POINT ( 'NONE',  ( -10.81189881249999729, 6.242252689847871849, -32.21875000204835260 ) ) ;
#13367=CARTESIAN_POINT ( 'NONE',  ( -5.405949406249996869, 9.363379034771805109, -138.8437500020484094 ) ) ;
#13369=CARTESIAN_POINT ( 'NONE',  ( 10.81189881249999907, 6.242252689847868297, -32.90625000204835970 ) ) ;
#13370=CARTESIAN_POINT ( 'NONE',  ( -4.999999999999996447, 8.660254037844387298, -110.9999999999999858 ) ) ;
#13371=CARTESIAN_POINT ( 'NONE',  ( 7.070501591499377789E-16, 11.54700538379251284, -70.62500000000000000 ) ) ;
#13372=CARTESIAN_POINT ( 'NONE',  ( -10.81189881249999729, 6.242252689847871849, -131.4062500020484094 ) ) ;
#13375=CARTESIAN_POINT ( 'NONE',  ( -9.999999999999998224, 1.224646799147353059E-15, -142.2500000000000000 ) ) ;
#13376=CARTESIAN_POINT ( 'NONE',  ( -10.00000000000000000, -5.773502691896251982, -105.0000000040967763 ) ) ;
#13377=CARTESIAN_POINT ( 'NONE',  ( 4.999999999999992006, -8.660254037844389075, -146.2500000000000000 ) ) ;
#13378=CARTESIAN_POINT ( 'NONE',  ( 7.644554776091147741E-16, 12.48450537969573659, -65.46875000204838102 ) ) ;
#13379=ORIENTED_EDGE ( 'NONE', *, *, #11416, .F. ) ;
#13384=CARTESIAN_POINT ( 'NONE',  ( -2.121150477449813534E-15, -11.54700538379251284, -34.25000000409675494 ) ) ;
#13387=CARTESIAN_POINT ( 'NONE',  ( 7.070501591499376803E-16, 11.54700538379251284, -122.0000000040967905 ) ) ;
#13389=( BOUNDED_CURVE ( )  B_SPLINE_CURVE ( 2, ( #28319, #24877, #42305, #41879, #6287, #9299, #9929 ),
 .UNSPECIFIED., .F., .F. ) 
 B_SPLINE_CURVE_WITH_KNOTS ( ( 3, 2, 2, 3 ),
 ( 0.4514925373134329734, 0.4527363184079603031, 0.4539800995024877439, 0.4552238805970150737 ),
 .UNSPECIFIED. ) 
 CURVE ( )  GEOMETRIC_REPRESENTATION_ITEM ( )  RATIONAL_B_SPLINE_CURVE ( ( 0.9999999999999880096, 0.8660254037844506980, 1.000000000000000000, 0.8660254037844387076, 1.000000000000000000, 0.8660254037844207220, 1.000000000000017986 ) ) 
 REPRESENTATION_ITEM ( '' )  );
#13400=CARTESIAN_POINT ( 'NONE',  ( 5.405949406249999534, 9.363379034771803333, -122.5937500020483952 ) ) ;
#13401=CARTESIAN_POINT ( 'NONE',  ( 5.405949406249999534, 9.363379034771803333, -134.7812500020483810 ) ) ;
#13403=CARTESIAN_POINT ( 'NONE',  ( -10.81189881249999729, -6.242252689847864744, -136.9687500020483810 ) ) ;
#13406=CARTESIAN_POINT ( 'NONE',  ( -9.999999999999998224, 5.773502691896259087, -158.8749999999999716 ) ) ;
#13410=CARTESIAN_POINT ( 'NONE',  ( -10.81189881249999729, 6.242252689847871849, -51.71875000204836681 ) ) ;
#13412=CARTESIAN_POINT ( 'NONE',  ( 7.644554776091147741E-16, 12.48450537969573659, -165.9687500020483810 ) ) ;
#13417=CARTESIAN_POINT ( 'NONE',  ( 5.000000000000000000, 8.660254037844385522, -91.74999999999998579 ) ) ;
#13418=VERTEX_POINT ( 'NONE', #27735 ) ;
#13419=CARTESIAN_POINT ( 'NONE',  ( 5.405949406249999534, 9.363379034771803333, -110.7812500020483810 ) ) ;
#13420=CARTESIAN_POINT ( 'NONE',  ( 9.999999999999996447, -5.773502691896262640, -134.5000000040967905 ) ) ;
#13423=CARTESIAN_POINT ( 'NONE',  ( -10.81189881249999729, 6.242252689847871849, -50.40625000204837391 ) ) ;
#13424=VECTOR ( 'NONE', #15867, 1000.000000000000000 ) ;
#13429=CARTESIAN_POINT ( 'NONE',  ( -9.999999999999996447, 5.773502691896259975, -173.8750000000000000 ) ) ;
#13433=ORIENTED_EDGE ( 'NONE', *, *, #29248, .T. ) ;
#13436=ORIENTED_EDGE ( 'NONE', *, *, #34791, .T. ) ;
#13443=CYLINDRICAL_SURFACE ( 'NONE', #4548, 9.999999999999998224 ) ;
#13447=CARTESIAN_POINT ( 'NONE',  ( -2.293366432827344421E-15, -12.48450537969573659, -150.2187500020483810 ) ) ;
#13448=CARTESIAN_POINT ( 'NONE',  ( 5.405949406249999534, 9.363379034771803333, -166.0937500020484094 ) ) ;
#13450=CARTESIAN_POINT ( 'NONE',  ( 9.999999999999998224, 0.000000000000000000, -161.3750000040967905 ) ) ;
#13451=CARTESIAN_POINT ( 'NONE',  ( 7.070501591499377789E-16, 11.54700538379251284, -184.6250000000000000 ) ) ;
#13455=DIRECTION ( 'NONE',  ( -0.000000000000000000, -0.000000000000000000, -1.000000000000000000 ) ) ;
#13457=CARTESIAN_POINT ( 'NONE',  ( -10.81189881249999729, 1.324075727343319199E-15, -189.5937500020483810 ) ) ;
#13460=EDGE_CURVE ( 'NONE', #15306, #24289, #11312, .T. ) ;
#13461=CARTESIAN_POINT ( 'NONE',  ( -5.405949406249996869, 9.363379034771805109, -50.53125000204835970 ) ) ;
#13463=CARTESIAN_POINT ( 'NONE',  ( -9.999999999999998224, 5.773502691896259087, -115.3749999999999858 ) ) ;
#13465=CARTESIAN_POINT ( 'NONE',  ( -10.81189881249999729, 1.324075727343319199E-15, -135.7812500020483810 ) ) ;
#13466=CARTESIAN_POINT ( 'NONE',  ( 5.405949406249999534, 9.363379034771803333, -149.7812500020483810 ) ) ;
#13469=CARTESIAN_POINT ( 'NONE',  ( -9.999999999999227285, -5.773502691896698735, -125.6249999999999574 ) ) ;
#13470=CARTESIAN_POINT ( 'NONE',  ( 5.405949406249992428, -9.363379034771808662, -84.09375000204836681 ) ) ;
#13473=CARTESIAN_POINT ( 'NONE',  ( 10.81189881249999907, 6.242252689847868297, -182.7187500020484094 ) ) ;
#13475=CARTESIAN_POINT ( 'NONE',  ( 9.999999999999998224, 0.000000000000000000, -171.5000000000000000 ) ) ;
#13477=CARTESIAN_POINT ( 'NONE',  ( -10.00000000000012790, -5.773502691896177375, -175.5000000040967905 ) ) ;
#13478=CARTESIAN_POINT ( 'NONE',  ( -10.81189881249999729, 6.242252689847871849, -75.90625000204838102 ) ) ;
#13481=AXIS2_PLACEMENT_3D ( 'NONE', #23665, #30141, #29497 ) ;
#13482=CARTESIAN_POINT ( 'NONE',  ( 4.999999999999992006, -8.660254037844389075, -56.62500000409676204 ) ) ;
#13483=CARTESIAN_POINT ( 'NONE',  ( 10.81189881249999907, 6.242252689847868297, -13.21875000204836148 ) ) ;
#13486=CARTESIAN_POINT ( 'NONE',  ( -2.293366432827344421E-15, -12.48450537969573659, -10.90625000204836681 ) ) ;
#13488=CARTESIAN_POINT ( 'NONE',  ( 4.999999999999992006, -8.660254037844389075, -161.2500000000000000 ) ) ;
#13489=AXIS2_PLACEMENT_3D ( 'NONE', #29354, #16366, #36251 ) ;
#13491=CARTESIAN_POINT ( 'NONE',  ( 0.000000000000000000, 0.000000000000000000, -99.99999999999998579 ) ) ;
#13497=CARTESIAN_POINT ( 'NONE',  ( 10.81189881249999729, 0.000000000000000000, -100.3437500020483810 ) ) ;
#13499=ORIENTED_EDGE ( 'NONE', *, *, #24915, .T. ) ;
#13507=CARTESIAN_POINT ( 'NONE',  ( 9.999999999999998224, 0.000000000000000000, -120.8750000040967905 ) ) ;
#13508=CARTESIAN_POINT ( 'NONE',  ( 5.405949406249999534, 9.363379034771803333, -145.2812500020483810 ) ) ;
#13512=CARTESIAN_POINT ( 'NONE',  ( 9.999999999999479527, 5.773502691896553074, -141.3750000000000000 ) ) ;
#13516=CARTESIAN_POINT ( 'NONE',  ( 7.644554776091147741E-16, 12.48450537969573659, -71.46875000204835260 ) ) ;
#13517=CARTESIAN_POINT ( 'NONE',  ( 7.644554776091147741E-16, 12.48450537969573659, -74.65625000204838102 ) ) ;
#13522=CARTESIAN_POINT ( 'NONE',  ( 7.644554776091147741E-16, 12.48450537969573659, -157.1562500020484094 ) ) ;
#13523=CARTESIAN_POINT ( 'NONE',  ( 10.81189881249999551, -6.242252689847874514, -175.6562500020484094 ) ) ;
#13525=CARTESIAN_POINT ( 'NONE',  ( -10.81189881249999729, 1.324075727343319199E-15, -0.5937500020483654772 ) ) ;
#13526=CARTESIAN_POINT ( 'NONE',  ( 10.81189881249999551, -6.242252689847874514, -103.4687500020483810 ) ) ;
#13528=CARTESIAN_POINT ( 'NONE',  ( 5.405949406249999534, 9.363379034771803333, -5.781250002048377468 ) ) ;
#13532=CARTESIAN_POINT ( 'NONE',  ( 7.644554776091147741E-16, 12.48450537969573659, -104.6562500020483810 ) ) ;
#13535=( BOUNDED_CURVE ( )  B_SPLINE_CURVE ( 2, ( #18782, #41858, #25492, #9076, #18356, #22242, #41651 ),
 .UNSPECIFIED., .F., .F. ) 
 B_SPLINE_CURVE_WITH_KNOTS ( ( 3, 2, 2, 3 ),
 ( 0.1417910447761193959, 0.1430348258706467535, 0.1442786069651741387, 0.1455223880597014963 ),
 .UNSPECIFIED. ) 
 CURVE ( )  GEOMETRIC_REPRESENTATION_ITEM ( )  RATIONAL_B_SPLINE_CURVE ( ( 1.000000000000000000, 0.8660254037844387076, 1.000000000000000000, 0.8660254037844387076, 1.000000000000000000, 0.8660254037844387076, 1.000000000000000000 ) ) 
 REPRESENTATION_ITEM ( '' )  );
#13536=CARTESIAN_POINT ( 'NONE',  ( -9.999999999999998224, 1.224646799147353059E-15, -85.62500000409677625 ) ) ;
#13538=CARTESIAN_POINT ( 'NONE',  ( -10.81189881249999729, 1.324075727343319199E-15, -41.09375000204837391 ) ) ;
#13539=VERTEX_POINT ( 'NONE', #4855 ) ;
#13543=CARTESIAN_POINT ( 'NONE',  ( 10.00000000000000000, 5.773502691896255534, -15.75000000409676559 ) ) ;
#13545=EDGE_CURVE ( 'NONE', #223, #18722, #37871, .T. ) ;
#13547=CARTESIAN_POINT ( 'NONE',  ( -9.999999999999998224, 1.224646799147353059E-15, -156.1250000040967905 ) ) ;
#13549=VERTEX_POINT ( 'NONE', #21462 ) ;
#13551=ORIENTED_EDGE ( 'NONE', *, *, #14202, .F. ) ;
#13558=CARTESIAN_POINT ( 'NONE',  ( 5.405949406249999534, 9.363379034771803333, -172.2812500020484094 ) ) ;
#13559=CARTESIAN_POINT ( 'NONE',  ( 9.999999999999612754, 5.773502691896477579, -155.2500000040967905 ) ) ;
#13561=CARTESIAN_POINT ( 'NONE',  ( 10.81189881249999907, 6.242252689847868297, -97.21875000204836681 ) ) ;
#13562=CARTESIAN_POINT ( 'NONE',  ( 9.999999999999998224, 0.000000000000000000, -155.0000000000000000 ) ) ;
#13563=CARTESIAN_POINT ( 'NONE',  ( 5.405949406249999534, 9.363379034771803333, -103.2812500020483952 ) ) ;
#13565=CARTESIAN_POINT ( 'NONE',  ( 5.405949406249999534, 9.363379034771803333, -118.0937500020483810 ) ) ;
#13569=CARTESIAN_POINT ( 'NONE',  ( 10.00000000000000000, 5.773502691896255534, -7.874999999999964473 ) ) ;
#13572=CARTESIAN_POINT ( 'NONE',  ( 9.999999999999996447, -5.773502691896262640, -179.5000000040968189 ) ) ;
#13574=CARTESIAN_POINT ( 'NONE',  ( 10.81189881249999907, 6.242252689847868297, -26.71875000204837391 ) ) ;
#13575=CYLINDRICAL_SURFACE ( 'NONE', #38506, 9.999999999999998224 ) ;
#13576=CARTESIAN_POINT ( 'NONE',  ( -5.405949406250003975, -9.363379034771801557, -127.8437500020483952 ) ) ;
#13578=CARTESIAN_POINT ( 'NONE',  ( 5.405949406249999534, 9.363379034771803333, -40.28125000204838102 ) ) ;
#13580=CARTESIAN_POINT ( 'NONE',  ( 7.070501591499377789E-16, 11.54700538379251284, -57.12499999999997868 ) ) ;
#13581=CARTESIAN_POINT ( 'NONE',  ( 10.81189881249999551, -6.242252689847874514, -129.1562500020483810 ) ) ;
#13585=CARTESIAN_POINT ( 'NONE',  ( 5.000000000000000000, 8.660254037844385522, -108.6250000040967763 ) ) ;
#13586=CARTESIAN_POINT ( 'NONE',  ( -10.00000000000025580, 5.773502691896109873, -161.8749999999999716 ) ) ;
#13587=CARTESIAN_POINT ( 'NONE',  ( -10.81189881249999729, 6.242252689847871849, -69.71875000204838102 ) ) ;
#13590=EDGE_CURVE ( 'NONE', #22548, #40153, #23836, .T. ) ;
#13594=CARTESIAN_POINT ( 'NONE',  ( 9.999999999999996447, -5.773502691896262640, -37.00000000409676204 ) ) ;
#13598=CARTESIAN_POINT ( 'NONE',  ( -9.999999999999998224, 1.224646799147353059E-15, -121.6250000040967905 ) ) ;
#13600=ORIENTED_EDGE ( 'NONE', *, *, #17595, .F. ) ;
#13603=CARTESIAN_POINT ( 'NONE',  ( -10.81189881249999907, -6.242252689847864744, -192.6562500020484094 ) ) ;
#13606=CARTESIAN_POINT ( 'NONE',  ( 5.000000000000000000, 8.660254037844385522, -150.2500000000000000 ) ) ;
#13609=VECTOR ( 'NONE', #24330, 1000.000000000000000 ) ;
#13611=CARTESIAN_POINT ( 'NONE',  ( 10.00000000000051159, -5.773502691895965988, -116.1249999999999716 ) ) ;
#13612=CARTESIAN_POINT ( 'NONE',  ( 7.644554776091147741E-16, 12.48450537969573659, -125.4687500020483952 ) ) ;
#13613=CARTESIAN_POINT ( 'NONE',  ( -5.000000000000003553, -8.660254037844383745, -193.3750000040967905 ) ) ;
#13614=CARTESIAN_POINT ( 'NONE',  ( -5.405949406250003975, -9.363379034771801557, -134.0312500020484094 ) ) ;
#13616=CARTESIAN_POINT ( 'NONE',  ( -5.405949406250003975, -9.363379034771801557, -135.3437500020484094 ) ) ;
#13617=CARTESIAN_POINT ( 'NONE',  ( 4.999999999999992006, -8.660254037844389075, -129.7499999999999716 ) ) ;
#13619=CARTESIAN_POINT ( 'NONE',  ( -10.00000000000000000, -5.773502691896251982, -152.6250000000000284 ) ) ;
#13620=CARTESIAN_POINT ( 'NONE',  ( 5.405949406249999534, 9.363379034771803333, -1.281250002048373027 ) ) ;
#13624=CARTESIAN_POINT ( 'NONE',  ( 10.81189881249999907, 6.242252689847868297, -53.71875000204837391 ) ) ;
#13625=CARTESIAN_POINT ( 'NONE',  ( 10.81189881249999551, -6.242252689847874514, -163.4687500020483810 ) ) ;
#13629=CARTESIAN_POINT ( 'NONE',  ( -9.999999999999998224, 5.773502691896259087, -86.87499999999998579 ) ) ;
#13631=ORIENTED_EDGE ( 'NONE', *, *, #7629, .T. ) ;
#13632=CARTESIAN_POINT ( 'NONE',  ( -10.81189881249999729, 1.324075727343319199E-15, -107.2812500020483810 ) ) ;
#13633=CARTESIAN_POINT ( 'NONE',  ( 7.070501591499377789E-16, 11.54700538379251284, -131.0000000040967905 ) ) ;
#13634=CARTESIAN_POINT ( 'NONE',  ( 9.999999999999998224, 0.000000000000000000, -177.5000000000000000 ) ) ;
#13637=CARTESIAN_POINT ( 'NONE',  ( -5.405949406249996869, 9.363379034771805109, -49.03125000204838813 ) ) ;
#13642=CARTESIAN_POINT ( 'NONE',  ( -9.999999999999998224, 1.224646799147353059E-15, -139.6250000040967905 ) ) ;
#13646=LINE ( 'NONE', #32896, #15526 ) ;
#13652=VERTEX_POINT ( 'NONE', #41045 ) ;
#13660=CARTESIAN_POINT ( 'NONE',  ( 7.644554776091147741E-16, 12.48450537969573659, -152.4687500020483810 ) ) ;
#13661=CARTESIAN_POINT ( 'NONE',  ( 10.81189881249999729, 6.242252689847867408, -160.2187500020483810 ) ) ;
#13663=CARTESIAN_POINT ( 'NONE',  ( 4.999999999999992006, -8.660254037844389075, -177.7500000000000284 ) ) ;
#13669=CARTESIAN_POINT ( 'NONE',  ( 5.405949406249992428, -9.363379034771808662, -183.0937500020483810 ) ) ;
#13671=VECTOR ( 'NONE', #9350, 1000.000000000000000 ) ;
#13673=CARTESIAN_POINT ( 'NONE',  ( 10.81189881249999729, 0.000000000000000000, -51.03125000204835970 ) ) ;
#13675=CARTESIAN_POINT ( 'NONE',  ( -4.999999999999996447, 8.660254037844387298, -104.9999999999999858 ) ) ;
#13676=EDGE_CURVE ( 'NONE', #23080, #30728, #22446, .T. ) ;
#13677=VERTEX_POINT ( 'NONE', #1162 ) ;
#13678=CARTESIAN_POINT ( 'NONE',  ( 5.405949406249999534, 9.363379034771803333, -136.2812500020483810 ) ) ;
#13679=CARTESIAN_POINT ( 'NONE',  ( -5.405949406250003975, -9.363379034771801557, -152.0312500020484094 ) ) ;
#13681=CARTESIAN_POINT ( 'NONE',  ( -10.81189881249999907, -6.242252689847864744, -79.96875000204836681 ) ) ;
#13684=CARTESIAN_POINT ( 'NONE',  ( -5.405949406250003975, -9.363379034771801557, -178.8437500020483810 ) ) ;
#13686=CARTESIAN_POINT ( 'NONE',  ( -2.121150477449813534E-15, -11.54700538379251284, -158.3750000000000000 ) ) ;
#13687=CARTESIAN_POINT ( 'NONE',  ( 10.81189881249999907, 6.242252689847868297, -76.40625000204839523 ) ) ;
#13689=CARTESIAN_POINT ( 'NONE',  ( 7.070501591499377789E-16, 11.54700538379251284, -48.50000000409676915 ) ) ;
#13690=CARTESIAN_POINT ( 'NONE',  ( 10.81189881249999907, 6.242252689847868297, -7.218750002048357040 ) ) ;
#13693=CARTESIAN_POINT ( 'NONE',  ( 7.644554776091147741E-16, 12.48450537969573659, -4.156250002048361480 ) ) ;
#13695=CARTESIAN_POINT ( 'NONE',  ( 5.000000000000000000, 8.660254037844385522, -176.1250000040968189 ) ) ;
#13700=ORIENTED_EDGE ( 'NONE', *, *, #39523, .T. ) ;
#13712=CARTESIAN_POINT ( 'NONE',  ( 9.999999999999996447, -5.773502691896262640, -48.62499999999997868 ) ) ;
#13716=CARTESIAN_POINT ( 'NONE',  ( 10.81189881249999551, -6.242252689847874514, -147.1562500020484094 ) ) ;
#13718=CARTESIAN_POINT ( 'NONE',  ( 9.999999999999998224, 1.224646799147353059E-15, -99.99999999999998579 ) ) ;
#13724=CARTESIAN_POINT ( 'NONE',  ( 5.405949406249992428, -9.363379034771808662, -72.09375000204836681 ) ) ;
#13725=CARTESIAN_POINT ( 'NONE',  ( -10.81189881249999907, -6.242252689847864744, -75.65625000204839523 ) ) ;
#13727=CARTESIAN_POINT ( 'NONE',  ( 10.81189881249999551, -6.242252689847874514, -156.1562500020483526 ) ) ;
#13728=CARTESIAN_POINT ( 'NONE',  ( 10.81189881249999729, 0.000000000000000000, -171.0312500020484094 ) ) ;
#13732=CARTESIAN_POINT ( 'NONE',  ( -10.81189881249999729, 6.242252689847871849, -107.2187500020483810 ) ) ;
#13734=CARTESIAN_POINT ( 'NONE',  ( -5.405949406249996869, 9.363379034771805109, -7.031250002048378356 ) ) ;
#13737=CARTESIAN_POINT ( 'NONE',  ( -10.81189881249999729, 1.324075727343319199E-15, -104.2812500020483810 ) ) ;
#13739=CARTESIAN_POINT ( 'NONE',  ( 9.999999999999998224, 0.000000000000000000, -78.87500000409677625 ) ) ;
#13740=CARTESIAN_POINT ( 'NONE',  ( -10.00000000000076916, 5.773502691895813221, -133.7500000040967905 ) ) ;
#13741=CARTESIAN_POINT ( 'NONE',  ( -10.81189881249999907, -6.242252689847864744, -30.46875000204835260 ) ) ;
#13745=CARTESIAN_POINT ( 'NONE',  ( -2.293366432827344421E-15, -12.48450537969573659, -27.40625000204838102 ) ) ;
#13748=CARTESIAN_POINT ( 'NONE',  ( -9.999999999999998224, 5.773502691896259087, -13.75000000409676382 ) ) ;
#13756=ORIENTED_EDGE ( 'NONE', *, *, #33653, .T. ) ;
#13765=FACE_OUTER_BOUND ( 'NONE', #37296, .T. ) ;
#13768=CARTESIAN_POINT ( 'NONE',  ( -5.405949406249996869, 9.363379034771805109, -175.0312500020484094 ) ) ;
#13773=CARTESIAN_POINT ( 'NONE',  ( 10.81189881249999729, 0.000000000000000000, -97.34375000204838102 ) ) ;
#13775=CARTESIAN_POINT ( 'NONE',  ( -5.405949406250003975, -9.363379034771801557, -102.5312500020483952 ) ) ;
#13777=CARTESIAN_POINT ( 'NONE',  ( 10.81189881249999551, -6.242252689847874514, -104.9687500020483810 ) ) ;
#13781=CARTESIAN_POINT ( 'NONE',  ( 5.405949406249992428, -9.363379034771808662, -178.7812500020484094 ) ) ;
#13782=CARTESIAN_POINT ( 'NONE',  ( 10.81189881249999907, 6.242252689847868297, -193.4062500020484094 ) ) ;
#13785=CARTESIAN_POINT ( 'NONE',  ( -9.999999999999998224, 5.773502691896259087, -169.7500000040967905 ) ) ;
#13787=CARTESIAN_POINT ( 'NONE',  ( -10.81189881249999729, 6.242252689847871849, -24.71875000204837391 ) ) ;
#13788=CARTESIAN_POINT ( 'NONE',  ( 9.999999999999998224, 0.000000000000000000, -108.8750000040967763 ) ) ;
#13789=CARTESIAN_POINT ( 'NONE',  ( -10.81189881249999907, -6.242252689847864744, -127.9687500020483810 ) ) ;
#13791=CARTESIAN_POINT ( 'NONE',  ( 10.81189881249999551, -6.242252689847874514, -30.15625000204835615 ) ) ;
#13794=CARTESIAN_POINT ( 'NONE',  ( -4.999999999999996447, 8.660254037844387298, -55.49999999999996447 ) ) ;
#13795=CARTESIAN_POINT ( 'NONE',  ( -5.405949406250003975, -9.363379034771801557, -126.5312500020483952 ) ) ;
#13798=CARTESIAN_POINT ( 'NONE',  ( 9.999999999999998224, 0.000000000000000000, -99.87500000409679046 ) ) ;
#13800=CARTESIAN_POINT ( 'NONE',  ( -10.81189881249999907, -6.242252689847864744, -55.96875000204836681 ) ) ;
#13805=CARTESIAN_POINT ( 'NONE',  ( -9.999999999999998224, 5.773502691896259087, -37.75000000409674783 ) ) ;
#13813=EDGE_LOOP ( 'NONE', ( #12596, #30413, #18179, #28086 ) ) ;
#13817=CARTESIAN_POINT ( 'NONE',  ( -10.81189881249999729, 6.242252689847871849, -197.4062500020484379 ) ) ;
#13822=CARTESIAN_POINT ( 'NONE',  ( 0.000000000000000000, 0.000000000000000000, -99.99999999999998579 ) ) ;
#13823=CARTESIAN_POINT ( 'NONE',  ( -5.405949406249996869, 9.363379034771805109, -114.8437500020483810 ) ) ;
#13824=CARTESIAN_POINT ( 'NONE',  ( -2.121150477449813534E-15, -11.54700538379251284, -196.2500000040967905 ) ) ;
#13825=CARTESIAN_POINT ( 'NONE',  ( -10.81189881249999729, 6.242252689847871849, -122.4062500020483952 ) ) ;
#13827=CARTESIAN_POINT ( 'NONE',  ( -2.293366432827344421E-15, -12.48450537969573659, -135.2187500020483810 ) ) ;
#13828=EDGE_CURVE ( 'NONE', #5087, #24099, #7573, .T. ) ;
#13830=CARTESIAN_POINT ( 'NONE',  ( -9.999999999999998224, 1.224646799147353059E-15, -155.7500000000000000 ) ) ;
#13831=CARTESIAN_POINT ( 'NONE',  ( 4.999999999999992006, -8.660254037844389075, -21.74999999999996447 ) ) ;
#13835=CARTESIAN_POINT ( 'NONE',  ( -2.121150477449813534E-15, -11.54700538379251284, -158.7500000040968189 ) ) ;
#13837=CARTESIAN_POINT ( 'NONE',  ( -10.81189881249999729, 1.324075727343319199E-15, -48.59375000204838102 ) ) ;
#13839=CARTESIAN_POINT ( 'NONE',  ( -2.293366432827344421E-15, -12.48450537969573659, -151.7187500020483810 ) ) ;
#13843=CARTESIAN_POINT ( 'NONE',  ( -9.999999999999998224, 5.773502691896259087, -83.87499999999998579 ) ) ;
#13846=CARTESIAN_POINT ( 'NONE',  ( -5.405949406249996869, 9.363379034771805109, -107.5312500020483810 ) ) ;
#13847=CARTESIAN_POINT ( 'NONE',  ( 9.999999999999998224, 0.000000000000000000, -132.8750000040967905 ) ) ;
#13852=CARTESIAN_POINT ( 'NONE',  ( 10.81189881249999729, 0.000000000000000000, -49.53125000204838813 ) ) ;
#13858=CARTESIAN_POINT ( 'NONE',  ( 5.000000000000000000, 8.660254037844385522, -177.2500000000000284 ) ) ;
#13871=CARTESIAN_POINT ( 'NONE',  ( -4.999999999999996447, 8.660254037844387298, -180.0000000000000000 ) ) ;
#13874=CARTESIAN_POINT ( 'NONE',  ( 5.405949406249992428, -9.363379034771808662, -139.5937500020483810 ) ) ;
#13875=CARTESIAN_POINT ( 'NONE',  ( -10.81189881249999729, 1.324075727343319199E-15, -162.5937500020484094 ) ) ;
#13877=CARTESIAN_POINT ( 'NONE',  ( -10.00000000000000000, -5.773502691896251982, -181.1249999999999716 ) ) ;
#13879=CARTESIAN_POINT ( 'NONE',  ( 5.000000000000000000, 8.660254037844385522, -138.2499999999999716 ) ) ;
#13882=CARTESIAN_POINT ( 'NONE',  ( -5.405949406250003975, -9.363379034771801557, -175.8437500020483810 ) ) ;
#13885=CARTESIAN_POINT ( 'NONE',  ( 7.644554776091147741E-16, 12.48450537969573659, -52.15625000204838102 ) ) ;
#13887=CARTESIAN_POINT ( 'NONE',  ( -5.000000000000003553, -8.660254037844383745, -108.9999999999999858 ) ) ;
#13889=VECTOR ( 'NONE', #36176, 1000.000000000000000 ) ;
#13892=CARTESIAN_POINT ( 'NONE',  ( -5.405949406250003975, -9.363379034771801557, -135.5312500020484094 ) ) ;
#13893=CARTESIAN_POINT ( 'NONE',  ( 10.81189881249999907, 6.242252689847868297, -148.4062500020484094 ) ) ;
#13895=CARTESIAN_POINT ( 'NONE',  ( 5.405949406249999534, 9.363379034771803333, -80.59375000204838102 ) ) ;
#13898=CARTESIAN_POINT ( 'NONE',  ( 5.405949406249999534, 9.363379034771803333, -181.0937500020483810 ) ) ;
#13902=CARTESIAN_POINT ( 'NONE',  ( -2.293366432827344421E-15, -12.48450537969573659, -79.90625000204839523 ) ) ;
#13904=CARTESIAN_POINT ( 'NONE',  ( 4.999999999999992006, -8.660254037844389075, -49.12500000409678336 ) ) ;
#13905=CARTESIAN_POINT ( 'NONE',  ( -5.405949406250003975, -9.363379034771801557, -10.84375000204834727 ) ) ;
#13908=CARTESIAN_POINT ( 'NONE',  ( -2.293366432827344421E-15, -12.48450537969573659, -4.906250002048362369 ) ) ;
#13910=CARTESIAN_POINT ( 'NONE',  ( -5.000000000000003553, -8.660254037844383745, -161.5000000000000000 ) ) ;
#13915=CARTESIAN_POINT ( 'NONE',  ( 10.81189881249999729, 6.242252689847867408, -103.2187500020483810 ) ) ;
#13916=ORIENTED_EDGE ( 'NONE', *, *, #30429, .F. ) ;
#13925=CARTESIAN_POINT ( 'NONE',  ( -9.999999999999998224, 1.224646799147353059E-15, -43.24999999999998579 ) ) ;
#13928=CARTESIAN_POINT ( 'NONE',  ( 9.999999999999998224, 0.000000000000000000, -147.5000000000000000 ) ) ;
#13929=CARTESIAN_POINT ( 'NONE',  ( 7.070501591499376803E-16, 11.54700538379251284, -144.1250000000000000 ) ) ;
#13933=CARTESIAN_POINT ( 'NONE',  ( 9.999999999999998224, 1.224646799147353059E-15, -99.99999999999998579 ) ) ;
#13937=CARTESIAN_POINT ( 'NONE',  ( 5.405949406249992428, -9.363379034771808662, -66.09375000204836681 ) ) ;
#13938=CARTESIAN_POINT ( 'NONE',  ( -10.81189881249999907, -6.242252689847864744, -72.65625000204836681 ) ) ;
#13940=CARTESIAN_POINT ( 'NONE',  ( 10.81189881249999551, -6.242252689847874514, -154.6562500020484094 ) ) ;
#13941=CARTESIAN_POINT ( 'NONE',  ( 10.81189881249999729, 0.000000000000000000, -172.5312500020484094 ) ) ;
#13942=DIRECTION ( 'NONE',  ( -0.000000000000000000, -0.000000000000000000, -1.000000000000000000 ) ) ;
#13943=DIRECTION ( 'NONE',  ( -0.000000000000000000, -0.000000000000000000, -1.000000000000000000 ) ) ;
#13944=CARTESIAN_POINT ( 'NONE',  ( 5.405949406249992428, -9.363379034771808662, -105.0937500020483810 ) ) ;
#13947=CARTESIAN_POINT ( 'NONE',  ( 7.644554776091147741E-16, 12.48450537969573659, -2.656250002048360592 ) ) ;
#13950=CARTESIAN_POINT ( 'NONE',  ( 7.644554776091147741E-16, 12.48450537969573659, -100.1562500020483952 ) ) ;
#13952=CARTESIAN_POINT ( 'NONE',  ( -9.999999999999998224, 1.224646799147353059E-15, -79.62500000409677625 ) ) ;
#13954=CARTESIAN_POINT ( 'NONE',  ( -2.293366432827344421E-15, -12.48450537969573659, -33.21875000204835260 ) ) ;
#13955=ORIENTED_EDGE ( 'NONE', *, *, #19077, .F. ) ;
#13957=CARTESIAN_POINT ( 'NONE',  ( -5.405949406250003975, -9.363379034771801557, -27.53125000204836681 ) ) ;
#13960=CARTESIAN_POINT ( 'NONE',  ( 4.999999999999992006, -8.660254037844389075, -2.625000004096766926 ) ) ;
#13967=ORIENTED_EDGE ( 'NONE', *, *, #35080, .F. ) ;
#13973=ORIENTED_EDGE ( 'NONE', *, *, #31492, .F. ) ;
#13975=CARTESIAN_POINT ( 'NONE',  ( 5.405949406249999534, 9.363379034771803333, -175.2812500020484094 ) ) ;
#13977=CARTESIAN_POINT ( 'NONE',  ( -10.81189881249999729, 1.324075727343319199E-15, -92.09375000204838102 ) ) ;
#13979=CARTESIAN_POINT ( 'NONE',  ( -5.405949406250003975, -9.363379034771801557, -104.0312500020483810 ) ) ;
#13981=CARTESIAN_POINT ( 'NONE',  ( -10.81189881249999729, 1.324075727343319199E-15, -107.0937500020483810 ) ) ;
#13984=CARTESIAN_POINT ( 'NONE',  ( -5.000000000000003553, -8.660254037844383745, -152.8750000040967905 ) ) ;
#13985=CARTESIAN_POINT ( 'NONE',  ( -5.405949406250003975, -9.363379034771801557, -192.5312500020484094 ) ) ;
#13988=CARTESIAN_POINT ( 'NONE',  ( 5.000000000000000000, 8.660254037844385522, -170.1250000040968189 ) ) ;
#13990=CARTESIAN_POINT ( 'NONE',  ( 7.644554776091147741E-16, 12.48450537969573659, -24.96875000204837391 ) ) ;
#13991=CARTESIAN_POINT ( 'NONE',  ( 0.000000000000000000, 0.000000000000000000, -99.99999999999998579 ) ) ;
#13992=CARTESIAN_POINT ( 'NONE',  ( 10.81189881249999551, -6.242252689847874514, -133.4687500020483810 ) ) ;
#13995=CARTESIAN_POINT ( 'NONE',  ( -5.405949406249996869, 9.363379034771805109, -31.03125000204837036 ) ) ;
#13997=EDGE_CURVE ( 'NONE', #37997, #24776, #38461, .T. ) ;
#13998=CARTESIAN_POINT ( 'NONE',  ( 5.000000000000000000, 8.660254037844385522, -55.74999999999996447 ) ) ;
#13999=CARTESIAN_POINT ( 'NONE',  ( -10.81189881249999907, -6.242252689847864744, -122.1562500020484094 ) ) ;
#14001=ORIENTED_EDGE ( 'NONE', *, *, #1047, .T. ) ;
#14003=CARTESIAN_POINT ( 'NONE',  ( 10.00000000000000000, 5.773502691896255534, -102.7500000040967905 ) ) ;
#14005=CARTESIAN_POINT ( 'NONE',  ( -5.405949406249996869, 9.363379034771805109, -56.34375000204835970 ) ) ;
#14010=CARTESIAN_POINT ( 'NONE',  ( 9.999999999999998224, 0.000000000000000000, -29.37500000409676204 ) ) ;
#14014=CARTESIAN_POINT ( 'NONE',  ( 7.070501591499376803E-16, 11.54700538379251284, -129.5000000040967905 ) ) ;
#14021=CARTESIAN_POINT ( 'NONE',  ( -5.405949406250003975, -9.363379034771801557, -195.5312500020484094 ) ) ;
#14023=CARTESIAN_POINT ( 'NONE',  ( -9.999999999999998224, 1.224646799147353059E-15, -138.1250000040967620 ) ) ;
#14027=CARTESIAN_POINT ( 'NONE',  ( -10.81189881249999729, 6.242252689847871849, -120.7187500020483952 ) ) ;
#14028=CARTESIAN_POINT ( 'NONE',  ( -10.00000000000000000, -5.773502691896251982, -196.5000000040967905 ) ) ;
#14029=CARTESIAN_POINT ( 'NONE',  ( -10.81189881249999729, 6.242252689847871849, -120.9062500020483952 ) ) ;
#14031=CARTESIAN_POINT ( 'NONE',  ( -10.81189881249999729, 6.242252689847871849, -128.2187500020483810 ) ) ;
#14034=CARTESIAN_POINT ( 'NONE',  ( 9.999999999999996447, -5.773502691896262640, -155.1250000000000000 ) ) ;
#14035=CARTESIAN_POINT ( 'NONE',  ( 9.999999999999996447, -5.773502691896262640, -20.12499999999997868 ) ) ;
#14038=CARTESIAN_POINT ( 'NONE',  ( -9.999999999999998224, 1.224646799147353059E-15, -169.6250000040967905 ) ) ;
#14040=CARTESIAN_POINT ( 'NONE',  ( -5.405949406250003975, -9.363379034771801557, -43.84375000204837391 ) ) ;
#14042=CARTESIAN_POINT ( 'NONE',  ( 7.644554776091147741E-16, 12.48450537969573659, -156.9687500020484094 ) ) ;
#14046=CARTESIAN_POINT ( 'NONE',  ( 10.53161979936726844, 2.338297538395752273, -180.0000000000000568 ) ) ;
#14047=CARTESIAN_POINT ( 'NONE',  ( -9.999999999999998224, 1.224646799147353059E-15, -83.74999999999997158 ) ) ;
#14050=ORIENTED_EDGE ( 'NONE', *, *, #16994, .T. ) ;
#14051=CARTESIAN_POINT ( 'NONE',  ( 10.81189881249999551, -6.242252689847874514, -111.1562500020483952 ) ) ;
#14052=CARTESIAN_POINT ( 'NONE',  ( -9.999999999999998224, 5.773502691896259087, -123.2500000040967763 ) ) ;
#14053=CARTESIAN_POINT ( 'NONE',  ( -9.999999999999227285, -5.773502691896698735, -112.1249999999999574 ) ) ;
#14054=ADVANCED_FACE ( 'NONE', ( #25328 ), #38473, .F. ) ;
#14057=PRODUCT_DEFINITION ( 'UNKNOWN', '', #26987, #29581 ) ;
#14058=CARTESIAN_POINT ( 'NONE',  ( 10.81189881249999729, 0.000000000000000000, -55.53125000204836681 ) ) ;
#14064=CARTESIAN_POINT ( 'NONE',  ( 9.999999999999872102, 5.773502691896329253, -164.2500000040968189 ) ) ;
#14074=CARTESIAN_POINT ( 'NONE',  ( 9.999999999999998224, 0.000000000000000000, -153.8750000040967905 ) ) ;
#14079=CARTESIAN_POINT ( 'NONE',  ( -2.293366432827344421E-15, -12.48450537969573659, -139.7187500020483810 ) ) ;
#14080=CARTESIAN_POINT ( 'NONE',  ( 10.81189881249999729, 6.242252689847867408, -154.2187500020483810 ) ) ;
#14082=CARTESIAN_POINT ( 'NONE',  ( 7.070501591499376803E-16, 11.54700538379251284, -102.5000000040967905 ) ) ;
#14083=CARTESIAN_POINT ( 'NONE',  ( 4.999999999999992006, -8.660254037844389075, -176.2500000000000284 ) ) ;
#14086=CARTESIAN_POINT ( 'NONE',  ( -9.999999999999996447, 5.773502691896259975, -168.2500000040968189 ) ) ;
#14087=CARTESIAN_POINT ( 'NONE',  ( 5.405949406249992428, -9.363379034771808662, -181.5937500020483810 ) ) ;
#14091=CARTESIAN_POINT ( 'NONE',  ( -5.405949406250003975, -9.363379034771801557, -56.03125000204836681 ) ) ;
#14093=CARTESIAN_POINT ( 'NONE',  ( -2.121150477449813534E-15, -11.54700538379251284, -105.8749999999999858 ) ) ;
#14095=CARTESIAN_POINT ( 'NONE',  ( -5.405949406250003975, -9.363379034771801557, -132.5312500020484094 ) ) ;
#14096=CARTESIAN_POINT ( 'NONE',  ( -2.121150477449813534E-15, -11.54700538379251284, -148.2500000040968189 ) ) ;
#14097=CARTESIAN_POINT ( 'NONE',  ( 5.405949406249999534, 9.363379034771803333, -146.7812500020483810 ) ) ;
#14101=CARTESIAN_POINT ( 'NONE',  ( 5.405949406249999534, 9.363379034771803333, -176.5937500020484094 ) ) ;
#14105=CARTESIAN_POINT ( 'NONE',  ( 10.00000000000025402, -5.773502691896113426, -158.1250000000000284 ) ) ;
#14106=CARTESIAN_POINT ( 'NONE',  ( -5.405949406249996869, 9.363379034771805109, -74.53125000204838102 ) ) ;
#14108=CARTESIAN_POINT ( 'NONE',  ( -9.999999999999998224, 1.224646799147353059E-15, -51.12500000409675494 ) ) ;
#14109=CARTESIAN_POINT ( 'NONE',  ( 10.81189881249999551, -6.242252689847874514, -10.46875000204835793 ) ) ;
#14113=CARTESIAN_POINT ( 'NONE',  ( 5.405949406249999534, 9.363379034771803333, -7.281250002048378356 ) ) ;
#14114=CARTESIAN_POINT ( 'NONE',  ( 0.000000000000000000, 0.000000000000000000, -99.99999999999998579 ) ) ;
#14122=CARTESIAN_POINT ( 'NONE',  ( 10.00000000000051159, -5.773502691895965988, -122.5000000040967763 ) ) ;
#14127=VECTOR ( 'NONE', #33042, 1000.000000000000000 ) ;
#14131=CARTESIAN_POINT ( 'NONE',  ( -5.000000000000003553, -8.660254037844383745, -44.49999999999998579 ) ) ;
#14133=CARTESIAN_POINT ( 'NONE',  ( -10.81189881249999729, 6.242252689847871849, -167.2187500020483810 ) ) ;
#14134=( BOUNDED_CURVE ( )  B_SPLINE_CURVE ( 2, ( #33350, #7213, #32914, #16478, #3135, #42392, #39581 ),
 .UNSPECIFIED., .F., .F. ) 
 B_SPLINE_CURVE_WITH_KNOTS ( ( 3, 2, 2, 3 ),
 ( 0.3731343283582090331, 0.3743781094527363629, 0.3756218905472638037, 0.3768656716417911334 ),
 .UNSPECIFIED. ) 
 CURVE ( )  GEOMETRIC_REPRESENTATION_ITEM ( )  RATIONAL_B_SPLINE_CURVE ( ( 0.9999999999999940048, 0.8660254037844447028, 1.000000000000000000, 0.8660254037844387076, 1.000000000000000000, 0.8660254037844267172, 1.000000000000011990 ) ) 
 REPRESENTATION_ITEM ( '' )  );
#14143=CARTESIAN_POINT ( 'NONE',  ( -5.405949406250003975, -9.363379034771801557, -69.34375000204836681 ) ) ;
#14144=VECTOR ( 'NONE', #694, 1000.000000000000000 ) ;
#14145=CARTESIAN_POINT ( 'NONE',  ( 10.81189881249999551, -6.242252689847874514, -79.65625000204838102 ) ) ;
#14147=CARTESIAN_POINT ( 'NONE',  ( -4.999999999999996447, 8.660254037844387298, -135.0000000000000000 ) ) ;
#14149=CARTESIAN_POINT ( 'NONE',  ( 10.81189881249999729, 6.242252689847867408, -155.9062500020483810 ) ) ;
#14150=CARTESIAN_POINT ( 'NONE',  ( -2.293366432827344421E-15, -12.48450537969573659, -174.4062500020483810 ) ) ;
#14151=CARTESIAN_POINT ( 'NONE',  ( -5.405949406249996869, 9.363379034771805109, -0.8437500020483656993 ) ) ;
#14152=CARTESIAN_POINT ( 'NONE',  ( 9.999999999999998224, 0.000000000000000000, -108.8750000040967763 ) ) ;
#14153=CARTESIAN_POINT ( 'NONE',  ( -2.293366432827344421E-15, -12.48450537969573659, -108.2187500020483668 ) ) ;
#14156=CARTESIAN_POINT ( 'NONE',  ( 10.81189881249999907, 6.242252689847868297, -4.406250002048361480 ) ) ;
#14160=CARTESIAN_POINT ( 'NONE',  ( 5.405949406249992428, -9.363379034771808662, -97.78125000204839523 ) ) ;
#14162=CARTESIAN_POINT ( 'NONE',  ( 5.000000000000000000, 8.660254037844385522, -72.62500000409677625 ) ) ;
#14164=CARTESIAN_POINT ( 'NONE',  ( 7.644554776091147741E-16, 12.48450537969573659, -30.96875000204835260 ) ) ;
#14167=CARTESIAN_POINT ( 'NONE',  ( -10.81189881249999907, -6.242252689847864744, -26.15625000204838102 ) ) ;
#14170=CARTESIAN_POINT ( 'NONE',  ( -9.999999999999998224, 1.224646799147353059E-15, -1.625000004096766038 ) ) ;
#14173=DIRECTION ( 'NONE',  ( -0.000000000000000000, -0.000000000000000000, -1.000000000000000000 ) ) ;
#14177=ORIENTED_EDGE ( 'NONE', *, *, #21602, .T. ) ;
#14180=EDGE_CURVE ( 'NONE', #40199, #19714, #6520, .T. ) ;
#14182=MECHANICAL_CONTEXT ( 'NONE', #25362, 'mechanical' ) ;
#14185=CARTESIAN_POINT ( 'NONE',  ( 0.000000000000000000, 0.000000000000000000, -99.99999999999998579 ) ) ;
#14187=CARTESIAN_POINT ( 'NONE',  ( -10.81189881249999729, 1.324075727343319199E-15, -176.2812500020484094 ) ) ;
#14190=CARTESIAN_POINT ( 'NONE',  ( 5.405949406249992428, -9.363379034771808662, -91.59375000204838102 ) ) ;
#14192=CARTESIAN_POINT ( 'NONE',  ( 5.000000000000000000, 8.660254037844385522, -113.1250000040967763 ) ) ;
#14193=CARTESIAN_POINT ( 'NONE',  ( -10.81189881249999907, -6.242252689847864744, -98.15625000204839523 ) ) ;
#14195=CARTESIAN_POINT ( 'NONE',  ( -10.81189881249999729, 6.242252689847871849, -107.2187500020483810 ) ) ;
#14198=CARTESIAN_POINT ( 'NONE',  ( -9.999999999999612754, -5.773502691896474914, -153.0000000040967620 ) ) ;
#14199=CARTESIAN_POINT ( 'NONE',  ( -4.999999999999996447, 8.660254037844387298, 2.775557561562891351E-14 ) ) ;
#14202=EDGE_CURVE ( 'NONE', #13652, #23080, #28709, .T. ) ;
#14203=CARTESIAN_POINT ( 'NONE',  ( 5.000000000000000000, 8.660254037844385522, -174.6250000040968189 ) ) ;
#14205=CARTESIAN_POINT ( 'NONE',  ( -5.405949406249996869, 9.363379034771805109, -18.84375000204835260 ) ) ;
#14207=CARTESIAN_POINT ( 'NONE',  ( -10.81189881249999729, 6.242252689847871849, -131.2187500020483810 ) ) ;
#14209=CARTESIAN_POINT ( 'NONE',  ( -2.293366432827344421E-15, -12.48450537969573659, -31.90625000204835970 ) ) ;
#14211=CARTESIAN_POINT ( 'NONE',  ( 7.070501591499376803E-16, 11.54700538379251284, -158.0000000040968189 ) ) ;
#14212=CARTESIAN_POINT ( 'NONE',  ( 7.070501591499377789E-16, 11.54700538379251284, -63.12499999999998579 ) ) ;
#14213=CARTESIAN_POINT ( 'NONE',  ( -2.293366432827344421E-15, -12.48450537969573659, -126.4062500020483952 ) ) ;
#14217=CARTESIAN_POINT ( 'NONE',  ( -2.121150477449813534E-15, -11.54700538379251284, -98.75000000409677625 ) ) ;
#14218=DIRECTION ( 'NONE',  ( -0.000000000000000000, -0.000000000000000000, -1.000000000000000000 ) ) ;
#14220=CARTESIAN_POINT ( 'NONE',  ( 10.81189881249999729, 0.000000000000000000, -58.34375000204835970 ) ) ;
#14226=CARTESIAN_POINT ( 'NONE',  ( -9.999999999999998224, 5.773502691896259087, -31.75000000409675138 ) ) ;
#14233=ORIENTED_EDGE ( 'NONE', *, *, #41980, .T. ) ;
#14234=FACE_OUTER_BOUND ( 'NONE', #15082, .T. ) ;
#14235=CARTESIAN_POINT ( 'NONE',  ( 5.000000000000000000, 8.660254037844385522, -174.6250000040968189 ) ) ;
#14237=CARTESIAN_POINT ( 'NONE',  ( 10.81189881249999729, 0.000000000000000000, -199.5312500020484094 ) ) ;
#14243=CARTESIAN_POINT ( 'NONE',  ( 5.405949406249999534, 9.363379034771803333, -121.0937500020483952 ) ) ;
#14244=CARTESIAN_POINT ( 'NONE',  ( -2.121150477449813534E-15, -11.54700538379251284, -197.7500000040967905 ) ) ;
#14245=CARTESIAN_POINT ( 'NONE',  ( -5.405949406249996869, 9.363379034771805109, -124.0312500020483952 ) ) ;
#14247=CARTESIAN_POINT ( 'NONE',  ( -10.81189881249999729, -6.242252689847864744, -126.4687500020483810 ) ) ;
#14250=CARTESIAN_POINT ( 'NONE',  ( -9.999999999999998224, 5.773502691896259087, -157.3749999999999716 ) ) ;
#14251=CARTESIAN_POINT ( 'NONE',  ( -10.00000000000000000, -5.773502691896251982, -17.62499999999997158 ) ) ;
#14256=CARTESIAN_POINT ( 'NONE',  ( -10.81189881249999907, -6.242252689847864744, -48.46875000204837391 ) ) ;
#14258=CARTESIAN_POINT ( 'NONE',  ( 10.81189881249999551, -6.242252689847874514, -157.4687500020484094 ) ) ;
#14261=CARTESIAN_POINT ( 'NONE',  ( 9.169708609005772004, 5.423292144399351145, -179.9999999999999716 ) ) ;
#14262=CARTESIAN_POINT ( 'NONE',  ( -2.121150477449813534E-15, -11.54700538379251284, -84.87500000000000000 ) ) ;
#14266=CARTESIAN_POINT ( 'NONE',  ( -5.405949406249996869, 9.363379034771805109, -104.5312500020483810 ) ) ;
#14267=CARTESIAN_POINT ( 'NONE',  ( 5.000000000000000000, 8.660254037844385522, -123.6250000040967905 ) ) ;
#14271=CARTESIAN_POINT ( 'NONE',  ( 10.81189881249999907, 6.242252689847868297, -55.40625000204837391 ) ) ;
#14272=LINE ( 'NONE', #24248, #37957 ) ;
#14275=CARTESIAN_POINT ( 'NONE',  ( 9.999999999999998224, 0.000000000000000000, -143.0000000000000000 ) ) ;
#14283=ORIENTED_EDGE ( 'NONE', *, *, #18832, .F. ) ;
#14295=CARTESIAN_POINT ( 'NONE',  ( -10.81189881249999907, -6.242252689847864744, -141.4687500020484094 ) ) ;
#14296=CARTESIAN_POINT ( 'NONE',  ( -10.81189881249999729, 1.324075727343319199E-15, -155.0937500020483810 ) ) ;
#14298=CARTESIAN_POINT ( 'NONE',  ( 7.070501591499377789E-16, 11.54700538379251284, -181.6250000000000000 ) ) ;
#14300=CARTESIAN_POINT ( 'NONE',  ( -9.999999999999998224, 1.224646799147353059E-15, -148.6250000040967905 ) ) ;
#14303=CARTESIAN_POINT ( 'NONE',  ( 7.644554776091147741E-16, 12.48450537969573659, -180.9687500020484094 ) ) ;
#14307=CARTESIAN_POINT ( 'NONE',  ( 9.999999999999998224, 0.000000000000000000, -137.0000000000000000 ) ) ;
#14308=CARTESIAN_POINT ( 'NONE',  ( 5.405949406249992428, -9.363379034771808662, -48.28125000204838813 ) ) ;
#14310=CARTESIAN_POINT ( 'NONE',  ( 10.00000000000000000, 5.773502691896255534, -108.3749999999999858 ) ) ;
#14312=CARTESIAN_POINT ( 'NONE',  ( 5.405949406249999534, 9.363379034771803333, -122.7812500020483952 ) ) ;
#14313=CARTESIAN_POINT ( 'NONE',  ( -10.00000000000000000, -5.773502691896251982, -148.5000000040967905 ) ) ;
#14314=CARTESIAN_POINT ( 'NONE',  ( 5.405949406249992428, -9.363379034771808662, -145.7812500020483810 ) ) ;
#14320=CARTESIAN_POINT ( 'NONE',  ( 10.81189881249999729, 0.000000000000000000, -178.3437500020483810 ) ) ;
#14326=CARTESIAN_POINT ( 'NONE',  ( 10.81189881249999729, 0.000000000000000000, -73.53125000204838102 ) ) ;
#14328=CARTESIAN_POINT ( 'NONE',  ( 5.000000000000000000, 8.660254037844385522, -53.12500000409675494 ) ) ;
#14329=CARTESIAN_POINT ( 'NONE',  ( 10.81189881249999729, 0.000000000000000000, -13.34375000204834905 ) ) ;
#14332=CARTESIAN_POINT ( 'NONE',  ( 5.405949406249992428, -9.363379034771808662, -6.281250002048377468 ) ) ;
#14333=DIRECTION ( 'NONE',  ( 0.000000000000000000, 0.000000000000000000, 1.000000000000000000 ) ) ;
#14336=CARTESIAN_POINT ( 'NONE',  ( -9.999999999999998224, 0.000000000000000000, -99.99999999999998579 ) ) ;
#14341=SHAPE_REPRESENTATION_RELATIONSHIP ( 'NONE' , 'NONE' ,  #6779, #27907 ) ;
#14350=CARTESIAN_POINT ( 'NONE',  ( 9.999999999999998224, 0.000000000000000000, -43.99999999999998579 ) ) ;
#14354=CARTESIAN_POINT ( 'NONE',  ( -10.81189881249999729, 1.324075727343319199E-15, -162.5937500020484094 ) ) ;
#14355=CARTESIAN_POINT ( 'NONE',  ( 5.405949406249999534, 9.363379034771803333, -179.5937500020484094 ) ) ;
#14360=LINE ( 'NONE', #41339, #18364 ) ;
#14363=CARTESIAN_POINT ( 'NONE',  ( 7.644554776091147741E-16, 12.48450537969573659, -66.96875000204838102 ) ) ;
#14364=CARTESIAN_POINT ( 'NONE',  ( 10.81189881249999907, 6.242252689847868297, -76.40625000204839523 ) ) ;
#14366=CARTESIAN_POINT ( 'NONE',  ( -9.999999999999998224, 1.224646799147353059E-15, -128.7499999999999716 ) ) ;
#14368=CARTESIAN_POINT ( 'NONE',  ( -10.81189881249999729, 6.242252689847871849, -159.9062500020483810 ) ) ;
#14369=CARTESIAN_POINT ( 'NONE',  ( -10.81189881249999729, 1.324075727343319199E-15, -170.2812500020484094 ) ) ;
#14370=DIRECTION ( 'NONE',  ( -1.000000000000000000, 0.000000000000000000, 0.000000000000000000 ) ) ;
#14371=CARTESIAN_POINT ( 'NONE',  ( 7.070501591499376803E-16, 11.54700538379251284, -159.5000000040968189 ) ) ;
#14372=CARTESIAN_POINT ( 'NONE',  ( -10.81189881249999907, -6.242252689847864744, -106.9687500020483668 ) ) ;
#14373=CARTESIAN_POINT ( 'NONE',  ( -9.999999999999998224, 0.000000000000000000, -99.99999999999998579 ) ) ;
#14375=CARTESIAN_POINT ( 'NONE',  ( 10.81189881249999729, 0.000000000000000000, -3.031250002048374803 ) ) ;
#14378=CARTESIAN_POINT ( 'NONE',  ( 7.644554776091147741E-16, 12.48450537969573659, -103.1562500020483952 ) ) ;
#14380=CARTESIAN_POINT ( 'NONE',  ( -2.121150477449813534E-15, -11.54700538379251284, -79.25000000409677625 ) ) ;
#14382=CARTESIAN_POINT ( 'NONE',  ( -2.293366432827344421E-15, -12.48450537969573659, -30.21875000204835260 ) ) ;
#14385=CARTESIAN_POINT ( 'NONE',  ( 7.644554776091147741E-16, 12.48450537969573659, -26.65625000204838102 ) ) ;
#14388=CARTESIAN_POINT ( 'NONE',  ( 10.00000000000000000, 5.773502691896255534, -0.7500000040967513826 ) ) ;
#14392=AXIS2_PLACEMENT_3D ( 'NONE', #8573, #4471, #37704 ) ;
#14394=ORIENTED_EDGE ( 'NONE', *, *, #4298, .T. ) ;
#14396=ORIENTED_EDGE ( 'NONE', *, *, #1965, .T. ) ;
#14398=( BOUNDED_CURVE ( )  B_SPLINE_CURVE ( 2, ( #17175, #10702, #32753, #40060, #16963, #29731, #13507 ),
 .UNSPECIFIED., .F., .F. ) 
 B_SPLINE_CURVE_WITH_KNOTS ( ( 3, 2, 2, 3 ),
 ( 0.3843283582089552786, 0.3855721393034826638, 0.3868159203980099936, 0.3880597014925373789 ),
 .UNSPECIFIED. ) 
 CURVE ( )  GEOMETRIC_REPRESENTATION_ITEM ( )  RATIONAL_B_SPLINE_CURVE ( ( 0.9999999999999940048, 0.8660254037844447028, 1.000000000000000000, 0.8660254037844387076, 1.000000000000000000, 0.8660254037844327124, 1.000000000000005995 ) ) 
 REPRESENTATION_ITEM ( '' )  );
#14407=CARTESIAN_POINT ( 'NONE',  ( 10.81189881249999551, -6.242252689847874514, -171.1562500020484094 ) ) ;
#14411=CARTESIAN_POINT ( 'NONE',  ( 10.81189881249999551, -6.242252689847874514, -95.96875000204838102 ) ) ;
#14413=CARTESIAN_POINT ( 'NONE',  ( 9.999999999999742428, 5.773502691896404748, -154.8749999999999716 ) ) ;
#14414=CARTESIAN_POINT ( 'NONE',  ( -10.81189881249999907, -6.242252689847864744, -99.65625000204839523 ) ) ;
#14416=CARTESIAN_POINT ( 'NONE',  ( -5.405949406249996869, 9.363379034771805109, -105.8437500020483810 ) ) ;
#14420=CARTESIAN_POINT ( 'NONE',  ( 7.644554776091147741E-16, 12.48450537969573659, -194.6562500020484094 ) ) ;
#14423=CARTESIAN_POINT ( 'NONE',  ( -9.999999999999998224, 5.773502691896259087, -172.7500000040967905 ) ) ;
#14425=CARTESIAN_POINT ( 'NONE',  ( -2.293366432827344421E-15, -12.48450537969573659, -24.21875000204837036 ) ) ;
#14427=CARTESIAN_POINT ( 'NONE',  ( 5.405949406249999534, 9.363379034771803333, -127.0937500020483668 ) ) ;
#14429=CARTESIAN_POINT ( 'NONE',  ( -10.81189881249999729, 1.324075727343319199E-15, -27.78125000204837036 ) ) ;
#14431=CARTESIAN_POINT ( 'NONE',  ( 9.999999999999998224, 0.000000000000000000, -102.5000000000000000 ) ) ;
#14432=CARTESIAN_POINT ( 'NONE',  ( 5.000000000000000000, 8.660254037844385522, -54.24999999999996447 ) ) ;
#14433=CARTESIAN_POINT ( 'NONE',  ( 5.405949406249992428, -9.363379034771808662, -121.7812500020483952 ) ) ;
#14438=CARTESIAN_POINT ( 'NONE',  ( 9.999999999999998224, 0.000000000000000000, -101.3750000040967905 ) ) ;
#14441=CARTESIAN_POINT ( 'NONE',  ( -10.81189881249999907, -6.242252689847864744, -57.46875000204836681 ) ) ;
#14447=CARTESIAN_POINT ( 'NONE',  ( 5.000000000000000000, 8.660254037844385522, -24.62500000409675849 ) ) ;
#14448=CARTESIAN_POINT ( 'NONE',  ( 5.000000000000000000, 8.660254037844385522, -168.2500000000000000 ) ) ;
#14452=ORIENTED_EDGE ( 'NONE', *, *, #4812, .T. ) ;
#14455=ORIENTED_EDGE ( 'NONE', *, *, #3225, .F. ) ;
#14456=DIRECTION ( 'NONE',  ( -0.000000000000000000, -0.000000000000000000, -1.000000000000000000 ) ) ;
#14460=CARTESIAN_POINT ( 'NONE',  ( -10.81189881249999729, 6.242252689847871849, -198.9062500020484094 ) ) ;
#14466=CARTESIAN_POINT ( 'NONE',  ( -10.81189881249999907, -6.242252689847864744, -117.4687500020483952 ) ) ;
#14467=CARTESIAN_POINT ( 'NONE',  ( -9.999999999999998224, 5.773502691896259087, -195.2500000040967905 ) ) ;
#14468=CARTESIAN_POINT ( 'NONE',  ( -10.81189881249999907, -6.242252689847864744, -122.1562500020484094 ) ) ;
#14470=CARTESIAN_POINT ( 'NONE',  ( -10.81189881249999729, 1.324075727343319199E-15, -134.0937500020483810 ) ) ;
#14471=CARTESIAN_POINT ( 'NONE',  ( 9.999999999999998224, 0.000000000000000000, -123.5000000000000000 ) ) ;
#14472=CARTESIAN_POINT ( 'NONE',  ( -9.999999999999998224, 1.224646799147353059E-15, -146.7500000000000000 ) ) ;
#14473=CARTESIAN_POINT ( 'NONE',  ( 9.999999999999996447, -5.773502691896262640, -21.62499999999997868 ) ) ;
#14476=CARTESIAN_POINT ( 'NONE',  ( -5.000000000000003553, -8.660254037844383745, -170.5000000000000000 ) ) ;
#14478=CARTESIAN_POINT ( 'NONE',  ( 5.405949406249992428, -9.363379034771808662, -45.09375000204837391 ) ) ;
#14480=CARTESIAN_POINT ( 'NONE',  ( 10.81189881249999551, -6.242252689847874514, -155.9687500020484094 ) ) ;
#14483=CARTESIAN_POINT ( 'NONE',  ( 6.569481213899460492, 8.192167785318885009, -179.9999999999999716 ) ) ;
#14484=CARTESIAN_POINT ( 'NONE',  ( 10.00000000000000000, 5.773502691896255534, -79.87499999999998579 ) ) ;
#14487=CARTESIAN_POINT ( 'NONE',  ( 10.81189881249999729, 0.000000000000000000, -103.5312500020483810 ) ) ;
#14488=CARTESIAN_POINT ( 'NONE',  ( -10.00000000000000000, -5.773502691896251982, -126.0000000040967905 ) ) ;
#14489=CARTESIAN_POINT ( 'NONE',  ( 9.999999999999998224, 0.000000000000000000, -153.8750000040967905 ) ) ;
#14494=CARTESIAN_POINT ( 'NONE',  ( 5.405949406249999534, 9.363379034771803333, -44.78125000204838102 ) ) ;
#14501=ORIENTED_EDGE ( 'NONE', *, *, #18720, .F. ) ;
#14502=ORIENTED_EDGE ( 'NONE', *, *, #28516, .F. ) ;
#14514=CARTESIAN_POINT ( 'NONE',  ( 7.644554776091147741E-16, 12.48450537969573659, -144.9687500020483810 ) ) ;
#14515=CARTESIAN_POINT ( 'NONE',  ( -10.81189881249999729, 6.242252689847871849, -146.4062500020484094 ) ) ;
#14517=CARTESIAN_POINT ( 'NONE',  ( -2.293366432827344421E-15, -12.48450537969573659, -154.7187500020483810 ) ) ;
#14520=CARTESIAN_POINT ( 'NONE',  ( -9.999999999999998224, 5.773502691896259087, -178.3750000000000000 ) ) ;
#14522=LINE ( 'NONE', #40853, #5899 ) ;
#14525=CARTESIAN_POINT ( 'NONE',  ( -5.405949406250003975, -9.363379034771801557, -181.8437500020483810 ) ) ;
#14528=CARTESIAN_POINT ( 'NONE',  ( 0.000000000000000000, 0.000000000000000000, -99.99999999999998579 ) ) ;
#14529=CARTESIAN_POINT ( 'NONE',  ( 10.81189881249999551, -6.242252689847874514, -48.15625000204837391 ) ) ;
#14531=CARTESIAN_POINT ( 'NONE',  ( -2.121150477449813534E-15, -11.54700538379251284, -107.3749999999999716 ) ) ;
#14533=CARTESIAN_POINT ( 'NONE',  ( -10.81189881249999729, 1.324075727343319199E-15, -129.7812500020483810 ) ) ;
#14534=CARTESIAN_POINT ( 'NONE',  ( 7.070501591499377789E-16, 11.54700538379251284, -144.5000000040967905 ) ) ;
#14535=CARTESIAN_POINT ( 'NONE',  ( -5.000000000000003553, -8.660254037844383745, -167.5000000000000000 ) ) ;
#14537=ORIENTED_EDGE ( 'NONE', *, *, #36496, .F. ) ;
#14539=CARTESIAN_POINT ( 'NONE',  ( 10.81189881249999907, 6.242252689847868297, -173.7187500020484094 ) ) ;
#14541=EDGE_CURVE ( 'NONE', #33113, #37078, #24031, .T. ) ;
#14545=CARTESIAN_POINT ( 'NONE',  ( -2.293366432827344421E-15, -12.48450537969573659, -70.90625000204839523 ) ) ;
#14548=CARTESIAN_POINT ( 'NONE',  ( -4.999999999999996447, 8.660254037844387298, -42.37500000409677625 ) ) ;
#14549=CARTESIAN_POINT ( 'NONE',  ( 5.405949406249992428, -9.363379034771808662, -3.093750002048367698 ) ) ;
#14550=CARTESIAN_POINT ( 'NONE',  ( -9.999999999999998224, 0.000000000000000000, -99.99999999999998579 ) ) ;
#14554=CARTESIAN_POINT ( 'NONE',  ( -9.999999999999998224, 0.000000000000000000, -99.99999999999998579 ) ) ;
#14556=DIRECTION ( 'NONE',  ( -0.000000000000000000, -0.000000000000000000, -1.000000000000000000 ) ) ;
#14560=ORIENTED_EDGE ( 'NONE', *, *, #14541, .F. ) ;
#14570=CARTESIAN_POINT ( 'NONE',  ( 9.999999999999998224, 0.000000000000000000, -42.49999999999998579 ) ) ;
#14573=CARTESIAN_POINT ( 'NONE',  ( -10.81189881249999729, 6.242252689847871849, -165.7187500020483810 ) ) ;
#14575=CARTESIAN_POINT ( 'NONE',  ( 5.405949406249992428, -9.363379034771808662, -177.0937500020484094 ) ) ;
#14578=DIRECTION ( 'NONE',  ( 0.000000000000000000, 0.000000000000000000, 1.000000000000000000 ) ) ;
#14585=CARTESIAN_POINT ( 'NONE',  ( 5.405949406249999534, 9.363379034771803333, -62.59375000204836681 ) ) ;
#14586=CARTESIAN_POINT ( 'NONE',  ( -10.81189881249999907, -6.242252689847864744, -68.15625000204839523 ) ) ;
#14588=CARTESIAN_POINT ( 'NONE',  ( -5.000000000000003553, -8.660254037844383745, -130.0000000000000000 ) ) ;
#14589=CARTESIAN_POINT ( 'NONE',  ( 10.81189881249999729, 6.242252689847867408, -154.4062500020483810 ) ) ;
#14590=CARTESIAN_POINT ( 'NONE',  ( 5.405949406249992428, -9.363379034771808662, -165.2812500020484094 ) ) ;
#14591=AXIS2_PLACEMENT_3D ( 'NONE', #20227, #6647, #10296 ) ;
#14592=FACE_BOUND ( 'NONE', #23078, .T. ) ;
#14593=CARTESIAN_POINT ( 'NONE',  ( -5.405949406249996869, 9.363379034771805109, -98.34375000204838102 ) ) ;
#14596=CARTESIAN_POINT ( 'NONE',  ( 7.644554776091147741E-16, 12.48450537969573659, -192.9687500020483810 ) ) ;
#14600=CARTESIAN_POINT ( 'NONE',  ( -10.81189881249999907, -6.242252689847864744, -98.15625000204839523 ) ) ;
#14603=CARTESIAN_POINT ( 'NONE',  ( -9.999999999999998224, 5.773502691896259087, -76.75000000409676204 ) ) ;
#14605=CARTESIAN_POINT ( 'NONE',  ( 7.644554776091147741E-16, 12.48450537969573659, -36.96875000204835260 ) ) ;
#14609=CARTESIAN_POINT ( 'NONE',  ( -10.81189881249999907, -6.242252689847864744, -24.65625000204838102 ) ) ;
#14612=CARTESIAN_POINT ( 'NONE',  ( 4.999999999999992006, -8.660254037844389075, -4.125000004096768258 ) ) ;
#14614=VECTOR ( 'NONE', #24587, 1000.000000000000000 ) ;
#14628=CARTESIAN_POINT ( 'NONE',  ( 4.607092693325971489, 9.672354888048561250, -99.99999999999998579 ) ) ;
#14630=CARTESIAN_POINT ( 'NONE',  ( 5.405949406249992428, -9.363379034771808662, -168.2812500020484094 ) ) ;
#14633=CARTESIAN_POINT ( 'NONE',  ( 10.81189881249999907, 6.242252689847868297, -85.21875000204836681 ) ) ;
#14635=CARTESIAN_POINT ( 'NONE',  ( 5.405949406249992428, -9.363379034771808662, -198.0937500020484094 ) ) ;
#14636=CARTESIAN_POINT ( 'NONE',  ( 5.405949406249992428, -9.363379034771808662, -88.78125000204838102 ) ) ;
#14638=CARTESIAN_POINT ( 'NONE',  ( 7.644554776091147741E-16, 12.48450537969573659, -107.4687500020483668 ) ) ;
#14641=CARTESIAN_POINT ( 'NONE',  ( 10.81189881249999729, 0.000000000000000000, -171.0312500020484094 ) ) ;
#14642=CARTESIAN_POINT ( 'NONE',  ( -2.293366432827344421E-15, -12.48450537969573659, -184.9062500020484094 ) ) ;
#14644=CARTESIAN_POINT ( 'NONE',  ( -4.999999999999996447, 8.660254037844387298, -175.8750000040967905 ) ) ;
#14646=CARTESIAN_POINT ( 'NONE',  ( -10.81189881249999729, 1.324075727343319199E-15, -24.59375000204835970 ) ) ;
#14648=CARTESIAN_POINT ( 'NONE',  ( 10.81189881249999907, 6.242252689847868297, -118.2187500020483810 ) ) ;
#14650=CARTESIAN_POINT ( 'NONE',  ( -10.81189881249999729, 1.324075727343319199E-15, -29.28125000204837036 ) ) ;
#14653=CARTESIAN_POINT ( 'NONE',  ( 9.999999999999998224, 0.000000000000000000, -52.99999999999996447 ) ) ;
#14654=CARTESIAN_POINT ( 'NONE',  ( -10.81189881249999729, 1.324075727343319199E-15, -120.7812500020483952 ) ) ;
#14657=CARTESIAN_POINT ( 'NONE',  ( -10.00000000000000000, -5.773502691896251982, -103.5000000040967763 ) ) ;
#14660=CARTESIAN_POINT ( 'NONE',  ( 10.81189881249999551, -6.242252689847874514, -56.96875000204838102 ) ) ;
#14666=CARTESIAN_POINT ( 'NONE',  ( 9.999999999999998224, 0.000000000000000000, -27.87500000409676204 ) ) ;
#14667=( BOUNDED_CURVE ( )  B_SPLINE_CURVE ( 2, ( #26900, #29727, #16314, #40056, #29942, #23246, #29510 ),
 .UNSPECIFIED., .F., .F. ) 
 B_SPLINE_CURVE_WITH_KNOTS ( ( 3, 2, 2, 3 ),
 ( 0.4141791044776120256, 0.4154228855721394109, 0.4166666666666667962, 0.4179104477611941260 ),
 .UNSPECIFIED. ) 
 CURVE ( )  GEOMETRIC_REPRESENTATION_ITEM ( )  RATIONAL_B_SPLINE_CURVE ( ( 0.9999999999999880096, 0.8660254037844506980, 1.000000000000000000, 0.8660254037844387076, 1.000000000000000000, 0.8660254037844267172, 1.000000000000011990 ) ) 
 REPRESENTATION_ITEM ( '' )  );
#14678=CARTESIAN_POINT ( 'NONE',  ( -9.999999999999998224, 1.224646799147353059E-15, -126.1250000040967620 ) ) ;
#14680=CARTESIAN_POINT ( 'NONE',  ( -10.81189881249999729, 1.324075727343319199E-15, -189.7812500020484094 ) ) ;
#14686=CARTESIAN_POINT ( 'NONE',  ( 10.81189881249999551, -6.242252689847874514, -113.9687500020483810 ) ) ;
#14687=CARTESIAN_POINT ( 'NONE',  ( 10.81189881249999729, 0.000000000000000000, -127.5312500020483952 ) ) ;
#14689=CARTESIAN_POINT ( 'NONE',  ( 10.81189881249999729, 0.000000000000000000, -131.8437500020484094 ) ) ;
#14691=FACE_OUTER_BOUND ( 'NONE', #4375, .T. ) ;
#14692=CARTESIAN_POINT ( 'NONE',  ( 7.070501591499377789E-16, 11.54700538379251284, -148.6250000000000000 ) ) ;
#14693=CARTESIAN_POINT ( 'NONE',  ( -5.000000000000003553, -8.660254037844383745, -20.49999999999996447 ) ) ;
#14698=CARTESIAN_POINT ( 'NONE',  ( -2.293366432827344421E-15, -12.48450537969573659, -42.21875000204835970 ) ) ;
#14699=CYLINDRICAL_SURFACE ( 'NONE', #30932, 9.999999999999998224 ) ;
#14700=CARTESIAN_POINT ( 'NONE',  ( -5.405949406250003975, -9.363379034771801557, -154.8437500020483810 ) ) ;
#14703=CARTESIAN_POINT ( 'NONE',  ( 10.00000000000000000, 5.773502691896255534, -73.87499999999995737 ) ) ;
#14706=CARTESIAN_POINT ( 'NONE',  ( 7.644554776091147741E-16, 12.48450537969573659, -100.1562500020483952 ) ) ;
#14707=CARTESIAN_POINT ( 'NONE',  ( 7.070501591499377789E-16, 11.54700538379251284, -125.0000000040967763 ) ) ;
#14709=CARTESIAN_POINT ( 'NONE',  ( -10.81189881249999907, -6.242252689847864744, -85.96875000204836681 ) ) ;
#14712=CARTESIAN_POINT ( 'NONE',  ( -5.405949406249996869, 9.363379034771805109, -43.03125000204838102 ) ) ;
#14718=CARTESIAN_POINT ( 'NONE',  ( 7.070501591499376803E-16, 11.54700538379251284, -177.1250000000000000 ) ) ;
#14719=ORIENTED_EDGE ( 'NONE', *, *, #17580, .T. ) ;
#14731=CARTESIAN_POINT ( 'NONE',  ( 10.81189881249999729, 0.000000000000000000, -140.8437500020483810 ) ) ;
#14732=CARTESIAN_POINT ( 'NONE',  ( -10.81189881249999907, -6.242252689847864744, -152.1562500020484094 ) ) ;
#14733=CARTESIAN_POINT ( 'NONE',  ( -10.81189881249999729, -6.242252689847864744, -153.4687500020484094 ) ) ;
#14736=CARTESIAN_POINT ( 'NONE',  ( -2.121150477449813534E-15, -11.54700538379251284, -170.3750000000000284 ) ) ;
#14741=CARTESIAN_POINT ( 'NONE',  ( -5.405949406250003975, -9.363379034771801557, -180.3437500020483810 ) ) ;
#14744=DIRECTION ( 'NONE',  ( -1.000000000000000000, 0.000000000000000000, 0.000000000000000000 ) ) ;
#14745=CARTESIAN_POINT ( 'NONE',  ( 10.81189881249999551, -6.242252689847874514, -42.15625000204836681 ) ) ;
#14747=CARTESIAN_POINT ( 'NONE',  ( -9.999999999999998224, 5.773502691896259087, -95.87499999999998579 ) ) ;
#14748=VERTEX_POINT ( 'NONE', #5839 ) ;
#14749=CARTESIAN_POINT ( 'NONE',  ( 10.81189881249999729, 0.000000000000000000, -124.5312500020483952 ) ) ;
#14750=CARTESIAN_POINT ( 'NONE',  ( 10.00000000000000000, 5.773502691896255534, -150.7500000040967905 ) ) ;
#14751=CARTESIAN_POINT ( 'NONE',  ( 0.000000000000000000, 0.000000000000000000, -99.99999999999998579 ) ) ;
#14754=CARTESIAN_POINT ( 'NONE',  ( -10.81189881249999729, 1.324075727343319199E-15, -173.0937500020484094 ) ) ;
#14758=CARTESIAN_POINT ( 'NONE',  ( -10.81189881249999729, 1.324075727343319199E-15, -71.28125000204838102 ) ) ;
#14760=CARTESIAN_POINT ( 'NONE',  ( 7.070501591499377789E-16, 11.54700538379251284, -45.50000000409676915 ) ) ;
#14761=CARTESIAN_POINT ( 'NONE',  ( 10.81189881249999907, 6.242252689847868297, -1.218750002048352155 ) ) ;
#14764=CARTESIAN_POINT ( 'NONE',  ( 9.999999999999998224, 0.000000000000000000, -149.0000000000000000 ) ) ;
#14765=ORIENTED_EDGE ( 'NONE', *, *, #23660, .T. ) ;
#14781=EDGE_CURVE ( 'NONE', #41753, #32304, #31761, .T. ) ;
#14782=CARTESIAN_POINT ( 'NONE',  ( -5.000000000000003553, -8.660254037844383745, -36.99999999999997868 ) ) ;
#14784=CARTESIAN_POINT ( 'NONE',  ( 10.81189881249999907, 6.242252689847868297, -166.2187500020484094 ) ) ;
#14785=CARTESIAN_POINT ( 'NONE',  ( -10.81189881249999729, 1.324075727343319199E-15, -176.0937500020484094 ) ) ;
#14790=CARTESIAN_POINT ( 'NONE',  ( 7.070501591499377789E-16, 11.54700538379251284, -192.1250000000000000 ) ) ;
#14795=CARTESIAN_POINT ( 'NONE',  ( -5.405949406249996869, 9.363379034771805109, -62.34375000204836681 ) ) ;
#14796=CARTESIAN_POINT ( 'NONE',  ( 5.405949406249999534, 9.363379034771803333, -68.78125000204838102 ) ) ;
#14798=CARTESIAN_POINT ( 'NONE',  ( 10.00000000000000000, 5.773502691896255534, -127.8749999999999858 ) ) ;
#14799=CARTESIAN_POINT ( 'NONE',  ( -5.405949406250003975, -9.363379034771801557, -152.0312500020484094 ) ) ;
#14800=CARTESIAN_POINT ( 'NONE',  ( -5.405949406249996869, 9.363379034771805109, -167.5312500020484094 ) ) ;
#14803=CARTESIAN_POINT ( 'NONE',  ( 5.405949406249992428, -9.363379034771808662, -100.5937500020483810 ) ) ;
#14806=CARTESIAN_POINT ( 'NONE',  ( 5.405949406249992428, -9.363379034771808662, -195.0937500020484094 ) ) ;
#14808=CARTESIAN_POINT ( 'NONE',  ( -8.660253955908514101, -5.000000141917089636, -180.0000000000000284 ) ) ;
#14809=CARTESIAN_POINT ( 'NONE',  ( 10.81189881249999907, 6.242252689847868297, -94.40625000204836681 ) ) ;
#14812=CARTESIAN_POINT ( 'NONE',  ( -9.999999999999998224, 5.773502691896259087, -67.75000000409677625 ) ) ;
#14813=CARTESIAN_POINT ( 'NONE',  ( 7.070501591499376803E-16, 11.54700538379251284, -135.1250000000000000 ) ) ;
#14814=CARTESIAN_POINT ( 'NONE',  ( 10.81189881249999729, 0.000000000000000000, -28.34375000204836326 ) ) ;
#14817=CARTESIAN_POINT ( 'NONE',  ( 10.81189881249999907, 6.242252689847868297, -22.40625000204838102 ) ) ;
#14819=CARTESIAN_POINT ( 'NONE',  ( 10.00000000000000000, 5.773502691896255534, -5.250000004096754935 ) ) ;
#14820=FACE_OUTER_BOUND ( 'NONE', #2940, .T. ) ;
#14826=DIRECTION ( 'NONE',  ( 1.000000000000000000, 0.000000000000000000, 0.000000000000000000 ) ) ;
#14827=ORIENTED_EDGE ( 'NONE', *, *, #11385, .T. ) ;
#14833=EDGE_CURVE ( 'NONE', #3489, #9539, #13535, .T. ) ;
#14834=CARTESIAN_POINT ( 'NONE',  ( -5.000000000000003553, -8.660254037844383745, -108.9999999999999858 ) ) ;
#14836=VECTOR ( 'NONE', #15421, 1000.000000000000000 ) ;
#14838=DIRECTION ( 'NONE',  ( -0.000000000000000000, -0.000000000000000000, -1.000000000000000000 ) ) ;
#14839=CARTESIAN_POINT ( 'NONE',  ( -5.405949406250003975, -9.363379034771801557, -168.5312500020484094 ) ) ;
#14844=CARTESIAN_POINT ( 'NONE',  ( -5.405949406249996869, 9.363379034771805109, -87.84375000204836681 ) ) ;
#14846=CARTESIAN_POINT ( 'NONE',  ( -2.293366432827344421E-15, -12.48450537969573659, -192.2187500020484379 ) ) ;
#14847=CARTESIAN_POINT ( 'NONE',  ( -5.405949406250003975, -9.363379034771801557, -92.03125000204838102 ) ) ;
#14851=CARTESIAN_POINT ( 'NONE',  ( -10.81189881249999729, -6.242252689847864744, -174.6562500020484094 ) ) ;
#14852=CARTESIAN_POINT ( 'NONE',  ( 10.81189881249999551, -6.242252689847874514, -187.6562500020484379 ) ) ;
#14854=CARTESIAN_POINT ( 'NONE',  ( 10.00000000000000000, 5.773502691896255534, -161.2500000040967905 ) ) ;
#14856=CARTESIAN_POINT ( 'NONE',  ( -10.81189881249999729, 6.242252689847871849, -14.21875000204836326 ) ) ;
#14858=CARTESIAN_POINT ( 'NONE',  ( -5.405949406249996869, 9.363379034771805109, -123.8437500020483952 ) ) ;
#14860=CARTESIAN_POINT ( 'NONE',  ( -5.405949406249996869, 9.363379034771805109, -23.53125000204836681 ) ) ;
#14862=CARTESIAN_POINT ( 'NONE',  ( -2.121150477449813534E-15, -11.54700538379251284, -136.2500000040967905 ) ) ;
#14863=CARTESIAN_POINT ( 'NONE',  ( 10.00000000000000000, 5.773502691896255534, -49.87499999999997158 ) ) ;
#14864=CARTESIAN_POINT ( 'NONE',  ( 5.405949406249999534, 9.363379034771803333, -113.7812500020483952 ) ) ;
#14867=CARTESIAN_POINT ( 'NONE',  ( -10.00000000000000000, -5.773502691896251982, -91.50000000409677625 ) ) ;
#14870=CARTESIAN_POINT ( 'NONE',  ( 5.405949406249999534, 9.363379034771803333, -52.09375000204835260 ) ) ;
#14877=( BOUNDED_CURVE ( )  B_SPLINE_CURVE ( 2, ( #32431, #19662, #2856, #6305, #32850, #42113, #6722 ),
 .UNSPECIFIED., .F., .F. ) 
 B_SPLINE_CURVE_WITH_KNOTS ( ( 3, 2, 2, 3 ),
 ( 0.1641791044776119424, 0.1654228855721392999, 0.1666666666666666574, 0.1679104477611940427 ),
 .UNSPECIFIED. ) 
 CURVE ( )  GEOMETRIC_REPRESENTATION_ITEM ( )  RATIONAL_B_SPLINE_CURVE ( ( 1.000000000000000000, 0.8660254037844387076, 1.000000000000000000, 0.8660254037844387076, 1.000000000000000000, 0.8660254037844387076, 1.000000000000000000 ) ) 
 REPRESENTATION_ITEM ( '' )  );
#14878=CARTESIAN_POINT ( 'NONE',  ( 5.000000000000000000, 8.660254037844385522, -29.12500000409676204 ) ) ;
#14880=CARTESIAN_POINT ( 'NONE',  ( 0.000000000000000000, 0.000000000000000000, -99.99999999999998579 ) ) ;
#14885=ORIENTED_EDGE ( 'NONE', *, *, #23304, .F. ) ;
#14893=CARTESIAN_POINT ( 'NONE',  ( 5.405949406249999534, 9.363379034771803333, -190.2812500020484094 ) ) ;
#14898=CARTESIAN_POINT ( 'NONE',  ( 10.81189881249999907, 6.242252689847868297, -107.7187500020483810 ) ) ;
#14900=CARTESIAN_POINT ( 'NONE',  ( -10.81189881249999729, 1.324075727343319199E-15, -117.7812500020483952 ) ) ;
#14902=CARTESIAN_POINT ( 'NONE',  ( -10.81189881249999729, 1.324075727343319199E-15, -128.0937500020483810 ) ) ;
#14904=CARTESIAN_POINT ( 'NONE',  ( 9.999999999999996447, -5.773502691896262640, -147.6250000000000000 ) ) ;
#14905=CARTESIAN_POINT ( 'NONE',  ( -5.000000000000003553, -8.660254037844383745, -12.99999999999995559 ) ) ;
#14909=CARTESIAN_POINT ( 'NONE',  ( -5.000000000000003553, -8.660254037844383745, -190.3750000040967905 ) ) ;
#14911=CARTESIAN_POINT ( 'NONE',  ( 5.405949406249992428, -9.363379034771808662, -36.09375000204836681 ) ) ;
#14913=CARTESIAN_POINT ( 'NONE',  ( -2.293366432827344421E-15, -12.48450537969573659, -144.2187500020483810 ) ) ;
#14915=DIRECTION ( 'NONE',  ( -0.000000000000000000, -0.000000000000000000, -1.000000000000000000 ) ) ;
#14916=CARTESIAN_POINT ( 'NONE',  ( 10.00000000000000000, 5.773502691896255534, -75.37499999999998579 ) ) ;
#14920=CARTESIAN_POINT ( 'NONE',  ( -2.121150477449813534E-15, -11.54700538379251284, -164.3749999999999716 ) ) ;
#14921=CARTESIAN_POINT ( 'NONE',  ( -10.00000000000000000, -5.773502691896251982, -121.5000000040967905 ) ) ;
#14923=CARTESIAN_POINT ( 'NONE',  ( -5.405949406249996869, 9.363379034771805109, -75.84375000204838102 ) ) ;
#14926=CARTESIAN_POINT ( 'NONE',  ( 5.405949406249999534, 9.363379034771803333, -41.78125000204838102 ) ) ;
#14932=CARTESIAN_POINT ( 'NONE',  ( -2.121150477449813534E-15, -11.54700538379251284, -120.8749999999999858 ) ) ;
#14933=ORIENTED_EDGE ( 'NONE', *, *, #15138, .F. ) ;
#14944=CARTESIAN_POINT ( 'NONE',  ( -10.81189881249999729, 1.324075727343319199E-15, -134.0937500020483810 ) ) ;
#14945=CARTESIAN_POINT ( 'NONE',  ( 10.81189881249999551, -6.242252689847874514, -141.1562500020484094 ) ) ;
#14946=CARTESIAN_POINT ( 'NONE',  ( 10.81189881249999551, -6.242252689847874514, -154.4687500020484094 ) ) ;
#14949=CARTESIAN_POINT ( 'NONE',  ( 9.999999999999998224, 0.000000000000000000, -168.5000000000000000 ) ) ;
#14950=ADVANCED_FACE ( 'NONE', ( #15102 ), #28089, .F. ) ;
#14955=CARTESIAN_POINT ( 'NONE',  ( 10.81189881249999729, 0.000000000000000000, -167.8437500020484094 ) ) ;
#14959=CARTESIAN_POINT ( 'NONE',  ( -10.81189881249999729, 1.324075727343319199E-15, -42.78125000204838102 ) ) ;
#14961=CARTESIAN_POINT ( 'NONE',  ( -5.000000000000003553, -8.660254037844383745, -98.49999999999998579 ) ) ;
#14963=CARTESIAN_POINT ( 'NONE',  ( 10.81189881249999551, -6.242252689847874514, -129.1562500020483810 ) ) ;
#14964=CARTESIAN_POINT ( 'NONE',  ( 5.000000000000000000, 8.660254037844385522, -150.6250000040967905 ) ) ;
#14967=EDGE_LOOP ( 'NONE', ( #1528, #12908, #41541, #29064 ) ) ;
#14968=CARTESIAN_POINT ( 'NONE',  ( -5.405949406250003975, -9.363379034771801557, -171.3437500020484094 ) ) ;
#14972=CARTESIAN_POINT ( 'NONE',  ( 10.81189881249999551, -6.242252689847874514, -67.65625000204838102 ) ) ;
#14974=CARTESIAN_POINT ( 'NONE',  ( -10.00000000000000000, -5.773502691896251982, -40.50000000409675494 ) ) ;
#14975=CARTESIAN_POINT ( 'NONE',  ( -10.81189881249999907, -6.242252689847864744, -1.968750002048352599 ) ) ;
#14976=CARTESIAN_POINT ( 'NONE',  ( 7.070501591499376803E-16, 11.54700538379251284, -147.5000000040967905 ) ) ;
#14986=EDGE_LOOP ( 'NONE', ( #29593, #5684, #30939, #23031 ) ) ;
#14990=( BOUNDED_CURVE ( )  B_SPLINE_CURVE ( 2, ( #6916, #3690, #12942, #39079, #13370, #22688, #32625 ),
 .UNSPECIFIED., .F., .F. ) 
 B_SPLINE_CURVE_WITH_KNOTS ( ( 3, 2, 2, 3 ),
 ( 0.4402985074626867279, 0.4415422885572141132, 0.4427860696517414429, 0.4440298507462688282 ),
 .UNSPECIFIED. ) 
 CURVE ( )  GEOMETRIC_REPRESENTATION_ITEM ( )  RATIONAL_B_SPLINE_CURVE ( ( 0.9999999999999820144, 0.8660254037844566932, 1.000000000000000000, 0.8660254037844387076, 1.000000000000000000, 0.8660254037844207220, 1.000000000000017986 ) ) 
 REPRESENTATION_ITEM ( '' )  );
#14991=ORIENTED_EDGE ( 'NONE', *, *, #5559, .T. ) ;
#14996=CARTESIAN_POINT ( 'NONE',  ( 7.070501591499376803E-16, 11.54700538379251284, -112.6249999999999858 ) ) ;
#14998=CARTESIAN_POINT ( 'NONE',  ( 4.999999999999992006, -8.660254037844389075, -36.74999999999997868 ) ) ;
#15000=CARTESIAN_POINT ( 'NONE',  ( -5.405949406250003975, -9.363379034771801557, -163.8437500020484094 ) ) ;
#15005=CARTESIAN_POINT ( 'NONE',  ( 5.000000000000000000, 8.660254037844385522, -192.2500000000000000 ) ) ;
#15011=CARTESIAN_POINT ( 'NONE',  ( -5.405949406249996869, 9.363379034771805109, -65.53125000204838102 ) ) ;
#15013=CARTESIAN_POINT ( 'NONE',  ( -9.999999999999998224, 5.773502691896259087, -127.3750000000000000 ) ) ;
#15014=CARTESIAN_POINT ( 'NONE',  ( 10.81189881249999729, 6.242252689847867408, -146.9062500020484379 ) ) ;
#15015=CARTESIAN_POINT ( 'NONE',  ( 10.81189881249999551, -6.242252689847874514, -163.6562500020484094 ) ) ;
#15018=CARTESIAN_POINT ( 'NONE',  ( -10.81189881249999729, 1.324075727343319199E-15, -101.0937500020483810 ) ) ;
#15021=CARTESIAN_POINT ( 'NONE',  ( 10.81189881249999729, 0.000000000000000000, -199.3437500020484094 ) ) ;
#15023=CARTESIAN_POINT ( 'NONE',  ( 1.257163379650654722, -10.41811935602516392, -180.0000000000000568 ) ) ;
#15024=CARTESIAN_POINT ( 'NONE',  ( -5.405949406250003975, -9.363379034771801557, -89.03125000204838102 ) ) ;
#15026=CARTESIAN_POINT ( 'NONE',  ( 5.000000000000000000, 8.660254037844385522, -68.12500000409677625 ) ) ;
#15028=CARTESIAN_POINT ( 'NONE',  ( 5.405949406249992428, -9.363379034771808662, -24.09375000204835970 ) ) ;
#15031=CARTESIAN_POINT ( 'NONE',  ( -10.81189881249999907, -6.242252689847864744, -21.65625000204838102 ) ) ;
#15037=CARTESIAN_POINT ( 'NONE',  ( 5.000000000000000000, 8.660254037844385522, -152.1250000040967905 ) ) ;
#15046=ORIENTED_EDGE ( 'NONE', *, *, #24107, .T. ) ;
#15051=CARTESIAN_POINT ( 'NONE',  ( 8.850157141833594920, 5.572544619961112389, -99.99999999999998579 ) ) ;
#15053=CARTESIAN_POINT ( 'NONE',  ( -5.405949406249996869, 9.363379034771805109, -163.0312500020484094 ) ) ;
#15056=CARTESIAN_POINT ( 'NONE',  ( -5.405949406249996869, 9.363379034771805109, -84.84375000204836681 ) ) ;
#15058=CARTESIAN_POINT ( 'NONE',  ( -10.81189881249999729, 6.242252689847871849, -191.2187500020484663 ) ) ;
#15059=CARTESIAN_POINT ( 'NONE',  ( -10.81189881249999729, 1.324075727343319199E-15, -93.78125000204838102 ) ) ;
#15062=CARTESIAN_POINT ( 'NONE',  ( 7.644554776091147741E-16, 12.48450537969573659, -175.1562500020484094 ) ) ;
#15063=CARTESIAN_POINT ( 'NONE',  ( -5.405949406249996869, 9.363379034771805109, -191.5312500020484094 ) ) ;
#15065=CARTESIAN_POINT ( 'NONE',  ( 9.999999999999998224, 0.000000000000000000, -164.3750000040967905 ) ) ;
#15067=CARTESIAN_POINT ( 'NONE',  ( -10.81189881249999729, 6.242252689847871849, -15.71875000204836503 ) ) ;
#15068=CARTESIAN_POINT ( 'NONE',  ( -10.81189881249999907, -6.242252689847864744, -121.9687500020483952 ) ) ;
#15070=CARTESIAN_POINT ( 'NONE',  ( -10.81189881249999729, 1.324075727343319199E-15, -17.28125000204835970 ) ) ;
#15074=CARTESIAN_POINT ( 'NONE',  ( 9.999999999999998224, 0.000000000000000000, -49.99999999999998579 ) ) ;
#15075=CARTESIAN_POINT ( 'NONE',  ( 5.405949406249992428, -9.363379034771808662, -120.2812500020483952 ) ) ;
#15078=CARTESIAN_POINT ( 'NONE',  ( 5.000000000000000000, 8.660254037844385522, -89.12500000409677625 ) ) ;
#15081=CARTESIAN_POINT ( 'NONE',  ( 10.81189881249999729, 0.000000000000000000, -50.84375000204835260 ) ) ;
#15082=EDGE_LOOP ( 'NONE', ( #882, #34327, #4230, #25792 ) ) ;
#15085=AXIS2_PLACEMENT_3D ( 'NONE', #30176, #11146, #14370 ) ;
#15086=EDGE_CURVE ( 'NONE', #23116, #40511, #32854, .T. ) ;
#15089=CARTESIAN_POINT ( 'NONE',  ( 4.999999999999992006, -8.660254037844389075, -23.62500000409675849 ) ) ;
#15098=EDGE_LOOP ( 'NONE', ( #2798, #11591, #39506, #13159 ) ) ;
#15099=ORIENTED_EDGE ( 'NONE', *, *, #6940, .F. ) ;
#15100=EDGE_CURVE ( 'NONE', #5147, #25998, #35970, .T. ) ;
#15102=FACE_OUTER_BOUND ( 'NONE', #40675, .T. ) ;
#15104=CARTESIAN_POINT ( 'NONE',  ( 10.81189881249999551, -6.242252689847874514, -189.1562500020484379 ) ) ;
#15110=CARTESIAN_POINT ( 'NONE',  ( -10.81189881249999907, -6.242252689847864744, -111.4687500020483810 ) ) ;
#15112=CARTESIAN_POINT ( 'NONE',  ( 10.81189881249999907, 6.242252689847868297, -119.9062500020483810 ) ) ;
#15114=CARTESIAN_POINT ( 'NONE',  ( -5.405949406249996869, 9.363379034771805109, -123.8437500020483952 ) ) ;
#15116=CARTESIAN_POINT ( 'NONE',  ( 5.000000000000000000, 8.660254037844385522, -179.1250000040968189 ) ) ;
#15117=CARTESIAN_POINT ( 'NONE',  ( -2.121150477449813534E-15, -11.54700538379251284, -144.8750000000000000 ) ) ;
#15118=CARTESIAN_POINT ( 'NONE',  ( 5.000000000000000000, 8.660254037844385522, -9.249999999999952038 ) ) ;
#15121=CARTESIAN_POINT ( 'NONE',  ( -4.999999999999996447, 8.660254037844387298, -187.8750000040967905 ) ) ;
#15123=CARTESIAN_POINT ( 'NONE',  ( -10.81189881249999907, -6.242252689847864744, -37.96875000204835970 ) ) ;
#15125=CARTESIAN_POINT ( 'NONE',  ( -5.405949406249996869, 9.363379034771805109, -149.3437500020483810 ) ) ;
#15128=CARTESIAN_POINT ( 'NONE',  ( 9.999999999999998224, 0.000000000000000000, -137.0000000000000000 ) ) ;
#15129=CARTESIAN_POINT ( 'NONE',  ( -10.00000000000000000, -5.773502691896251982, -73.12499999999995737 ) ) ;
#15130=CARTESIAN_POINT ( 'NONE',  ( 10.81189881249999729, 0.000000000000000000, -138.0312500020484094 ) ) ;
#15133=CARTESIAN_POINT ( 'NONE',  ( -5.405949406249996869, 9.363379034771805109, -101.5312500020483952 ) ) ;
#15134=CARTESIAN_POINT ( 'NONE',  ( 9.999999999999996447, -5.773502691896262640, -113.5000000040967763 ) ) ;
#15136=CARTESIAN_POINT ( 'NONE',  ( 10.81189881249999729, 0.000000000000000000, -77.84375000204838102 ) ) ;
#15138=EDGE_CURVE ( 'NONE', #31616, #41954, #17324, .T. ) ;
#15140=CARTESIAN_POINT ( 'NONE',  ( -10.81189881249999907, -6.242252689847864744, -45.65625000204837391 ) ) ;
#15144=AXIS2_PLACEMENT_3D ( 'NONE', #161, #39619, #40455 ) ;
#15148=DIRECTION ( 'NONE',  ( -0.000000000000000000, -0.000000000000000000, -1.000000000000000000 ) ) ;
#15160=CARTESIAN_POINT ( 'NONE',  ( 5.405949406249999534, 9.363379034771803333, -137.5937500020483810 ) ) ;
#15161=CARTESIAN_POINT ( 'NONE',  ( 10.81189881249999729, 0.000000000000000000, -141.0312500020483810 ) ) ;
#15162=CARTESIAN_POINT ( 'NONE',  ( 10.81189881249999729, 6.242252689847867408, -148.2187500020484094 ) ) ;
#15164=( BOUNDED_CURVE ( )  B_SPLINE_CURVE ( 2, ( #17516, #30714, #11689, #14920, #8477, #31574, #9105 ),
 .UNSPECIFIED., .F., .F. ) 
 B_SPLINE_CURVE_WITH_KNOTS ( ( 3, 2, 2, 3 ),
 ( 0.1753731343283582433, 0.1766169154228856009, 0.1778606965174129861, 0.1791044776119403437 ),
 .UNSPECIFIED. ) 
 CURVE ( )  GEOMETRIC_REPRESENTATION_ITEM ( )  RATIONAL_B_SPLINE_CURVE ( ( 0.9999999999999970024, 0.8660254037844417052, 1.000000000000000000, 0.8660254037844387076, 1.000000000000000000, 0.8660254037844327124, 1.000000000000005995 ) ) 
 REPRESENTATION_ITEM ( '' )  );
#15166=CARTESIAN_POINT ( 'NONE',  ( 4.999999999999992006, -8.660254037844389075, -168.7500000000000000 ) ) ;
#15169=DIRECTION ( 'NONE',  ( -0.000000000000000000, -0.000000000000000000, -1.000000000000000000 ) ) ;
#15171=CARTESIAN_POINT ( 'NONE',  ( 9.999999999999998224, 0.000000000000000000, -149.0000000000000000 ) ) ;
#15172=CARTESIAN_POINT ( 'NONE',  ( -10.81189881249999729, 6.242252689847871849, -170.2187500020483810 ) ) ;
#15176=CARTESIAN_POINT ( 'NONE',  ( -2.293366432827344421E-15, -12.48450537969573659, -45.40625000204837391 ) ) ;
#15178=CARTESIAN_POINT ( 'NONE',  ( 7.070501591499377789E-16, 11.54700538379251284, -102.1250000000000000 ) ) ;
#15181=CARTESIAN_POINT ( 'NONE',  ( 10.81189881249999729, 6.242252689847867408, -122.9062500020483810 ) ) ;
#15182=CARTESIAN_POINT ( 'NONE',  ( 9.999999999999996447, -5.773502691896262640, -143.5000000040967905 ) ) ;
#15186=CARTESIAN_POINT ( 'NONE',  ( 10.81189881249999907, 6.242252689847868297, -175.2187500020484094 ) ) ;
#15190=CARTESIAN_POINT ( 'NONE',  ( -10.81189881249999907, -6.242252689847864744, -66.65625000204839523 ) ) ;
#15191=CARTESIAN_POINT ( 'NONE',  ( 4.999999999999992006, -8.660254037844389075, -41.62500000409677625 ) ) ;
#15192=CARTESIAN_POINT ( 'NONE',  ( 10.81189881249999729, 0.000000000000000000, -5.843750002048370362 ) ) ;
#15197=ORIENTED_EDGE ( 'NONE', *, *, #13005, .F. ) ;
#15198=CARTESIAN_POINT ( 'NONE',  ( -9.999999999999998224, 1.224646799147353059E-15, -159.1250000040967905 ) ) ;
#15204=ORIENTED_EDGE ( 'NONE', *, *, #6913, .F. ) ;
#15205=LINE ( 'NONE', #32064, #11659 ) ;
#15214=CARTESIAN_POINT ( 'NONE',  ( -4.999999999999996447, 8.660254037844387298, -34.49999999999997158 ) ) ;
#15217=CARTESIAN_POINT ( 'NONE',  ( 5.405949406249999534, 9.363379034771803333, -155.5937500020483810 ) ) ;
#15219=CARTESIAN_POINT ( 'NONE',  ( -5.405949406249996869, 9.363379034771805109, -179.3437500020483810 ) ) ;
#15222=CARTESIAN_POINT ( 'NONE',  ( -10.00000000000000000, -5.773502691896251982, -194.6250000000000284 ) ) ;
#15227=CARTESIAN_POINT ( 'NONE',  ( 10.81189881249999729, 0.000000000000000000, -66.03125000204838102 ) ) ;
#15229=CARTESIAN_POINT ( 'NONE',  ( -4.999999999999996447, 8.660254037844387298, -126.0000000000000000 ) ) ;
#15231=ORIENTED_EDGE ( 'NONE', *, *, #13676, .F. ) ;
#15232=CARTESIAN_POINT ( 'NONE',  ( -5.405949406249996869, 9.363379034771805109, -149.5312500020483810 ) ) ;
#15233=CARTESIAN_POINT ( 'NONE',  ( 10.81189881249999551, -6.242252689847874514, -165.1562500020483526 ) ) ;
#15235=CARTESIAN_POINT ( 'NONE',  ( 9.999999999999998224, 1.224646799147353059E-15, -99.99999999999998579 ) ) ;
#15236=CARTESIAN_POINT ( 'NONE',  ( 10.70731569305653252, 1.500182182591227154, -180.0000000000000284 ) ) ;
#15237=CARTESIAN_POINT ( 'NONE',  ( 10.81189881249999551, -6.242252689847874514, -101.9687500020483810 ) ) ;
#15240=CARTESIAN_POINT ( 'NONE',  ( 5.405949406249999534, 9.363379034771803333, 0.2187499979516283055 ) ) ;
#15242=CARTESIAN_POINT ( 'NONE',  ( 0.000000000000000000, 0.000000000000000000, -99.99999999999998579 ) ) ;
#15243=CARTESIAN_POINT ( 'NONE',  ( -5.405949406249996869, 9.363379034771805109, -91.03125000204838102 ) ) ;
#15245=CARTESIAN_POINT ( 'NONE',  ( -10.00000000000000000, -5.773502691896251982, -70.50000000409677625 ) ) ;
#15247=CARTESIAN_POINT ( 'NONE',  ( -5.405949406249996869, 9.363379034771805109, -23.34375000204835970 ) ) ;
#15250=CARTESIAN_POINT ( 'NONE',  ( 10.81189881249999907, 6.242252689847868297, -23.90625000204838102 ) ) ;
#15252=CARTESIAN_POINT ( 'NONE',  ( 7.070501591499376803E-16, 11.54700538379251284, -160.6250000000000284 ) ) ;
#15259=CARTESIAN_POINT ( 'NONE',  ( -9.999999999999998224, 1.224646799147353059E-15, -119.7500000000000000 ) ) ;
#15261=ORIENTED_EDGE ( 'NONE', *, *, #31687, .F. ) ;
#15268=VERTEX_POINT ( 'NONE', #7901 ) ;
#15272=CARTESIAN_POINT ( 'NONE',  ( 8.891868809992706346, -4.636149425435562854, -99.99999999999998579 ) ) ;
#15274=CARTESIAN_POINT ( 'NONE',  ( -5.405949406250003975, -9.363379034771801557, -162.5312500020484094 ) ) ;
#15277=LINE ( 'NONE', #28684, #26034 ) ;
#15279=CARTESIAN_POINT ( 'NONE',  ( 5.405949406249992428, -9.363379034771808662, -85.59375000204836681 ) ) ;
#15280=CARTESIAN_POINT ( 'NONE',  ( 10.81189881249999729, 0.000000000000000000, -194.8437500020484094 ) ) ;
#15281=CARTESIAN_POINT ( 'NONE',  ( 5.405949406249999534, 9.363379034771803333, -92.78125000204838102 ) ) ;
#15285=CARTESIAN_POINT ( 'NONE',  ( -10.81189881249999729, 6.242252689847871849, -174.9062500020484094 ) ) ;
#15286=CARTESIAN_POINT ( 'NONE',  ( -5.405949406249996869, 9.363379034771805109, -187.0312500020484094 ) ) ;
#15288=CARTESIAN_POINT ( 'NONE',  ( -10.00000000000000000, -5.773502691896251982, -160.5000000040967905 ) ) ;
#15290=CARTESIAN_POINT ( 'NONE',  ( 10.81189881249999551, -6.242252689847874514, -16.46875000204836681 ) ) ;
#15292=CARTESIAN_POINT ( 'NONE',  ( -2.293366432827344421E-15, -12.48450537969573659, -121.7187500020483952 ) ) ;
#15294=CARTESIAN_POINT ( 'NONE',  ( 10.81189881249999907, 6.242252689847868297, -19.40625000204837747 ) ) ;
#15296=CARTESIAN_POINT ( 'NONE',  ( -9.999999999999227285, -5.773502691896698735, -136.5000000040967620 ) ) ;
#15297=CARTESIAN_POINT ( 'NONE',  ( -9.999999999999998224, 5.773502691896259087, -52.37499999999997868 ) ) ;
#15298=CARTESIAN_POINT ( 'NONE',  ( 10.81189881249999907, 6.242252689847868297, -116.9062500020483952 ) ) ;
#15302=CARTESIAN_POINT ( 'NONE',  ( -9.999999999999998224, 5.773502691896259087, -91.75000000409677625 ) ) ;
#15305=CARTESIAN_POINT ( 'NONE',  ( 5.405949406249999534, 9.363379034771803333, -53.59375000204835970 ) ) ;
#15306=VERTEX_POINT ( 'NONE', #36595 ) ;
#15310=CARTESIAN_POINT ( 'NONE',  ( 10.00000000000000000, 5.773502691896255534, -18.75000000409676915 ) ) ;
#15320=ORIENTED_EDGE ( 'NONE', *, *, #3134, .T. ) ;
#15323=CARTESIAN_POINT ( 'NONE',  ( -9.999999999999998224, 0.000000000000000000, -99.99999999999998579 ) ) ;
#15325=CARTESIAN_POINT ( 'NONE',  ( 5.405949406249999534, 9.363379034771803333, -191.7812500020484094 ) ) ;
#15329=CARTESIAN_POINT ( 'NONE',  ( -10.81189881249999907, -6.242252689847864744, -109.9687500020483668 ) ) ;
#15331=CARTESIAN_POINT ( 'NONE',  ( -10.81189881249999729, 6.242252689847871849, -114.9062500020483952 ) ) ;
#15333=CARTESIAN_POINT ( 'NONE',  ( -10.81189881249999729, -6.242252689847864744, -121.9687500020484237 ) ) ;
#15335=DIRECTION ( 'NONE',  ( -1.000000000000000000, 0.000000000000000000, 0.000000000000000000 ) ) ;
#15336=CARTESIAN_POINT ( 'NONE',  ( -5.000000000000003553, -8.660254037844383745, -146.5000000000000000 ) ) ;
#15337=CARTESIAN_POINT ( 'NONE',  ( -9.999999999999998224, 1.224646799147353059E-15, -10.24999999999995381 ) ) ;
#15340=CARTESIAN_POINT ( 'NONE',  ( 7.070501591499377789E-16, 11.54700538379251284, -186.5000000040967905 ) ) ;
#15342=CARTESIAN_POINT ( 'NONE',  ( -5.405949406249996869, 9.363379034771805109, -41.34375000204837391 ) ) ;
#15343=CARTESIAN_POINT ( 'NONE',  ( -10.81189881249999729, 6.242252689847871849, -149.2187500020484379 ) ) ;
#15345=CARTESIAN_POINT ( 'NONE',  ( 5.000000000000000000, 8.660254037844385522, -136.7499999999999716 ) ) ;
#15346=CARTESIAN_POINT ( 'NONE',  ( 7.070501591499377789E-16, 11.54700538379251284, -75.12500000000000000 ) ) ;
#15347=CARTESIAN_POINT ( 'NONE',  ( 7.644554776091147741E-16, 12.48450537969573659, -143.6562500020484094 ) ) ;
#15350=CARTESIAN_POINT ( 'NONE',  ( 5.000000000000000000, 8.660254037844385522, -120.6250000040967905 ) ) ;
#15351=CARTESIAN_POINT ( 'NONE',  ( 5.000000000000000000, 8.660254037844385522, -119.1250000040967905 ) ) ;
#15353=CARTESIAN_POINT ( 'NONE',  ( 10.81189881249999907, 6.242252689847868297, -74.71875000204838102 ) ) ;
#15357=CARTESIAN_POINT ( 'NONE',  ( 10.81189881249999551, -6.242252689847874514, -40.65625000204835970 ) ) ;
#15365=ORIENTED_EDGE ( 'NONE', *, *, #24079, .T. ) ;
#15370=ADVANCED_FACE ( 'NONE', ( #10472 ), #16087, .F. ) ;
#15374=CARTESIAN_POINT ( 'NONE',  ( -10.81189881249999729, 6.242252689847871849, -134.2187500020483810 ) ) ;
#15375=CARTESIAN_POINT ( 'NONE',  ( 5.405949406249992428, -9.363379034771808662, -138.2812500020483810 ) ) ;
#15376=CARTESIAN_POINT ( 'NONE',  ( 10.81189881249999729, 6.242252689847867408, -149.7187500020483810 ) ) ;
#15380=CARTESIAN_POINT ( 'NONE',  ( 9.999999999999996447, -5.773502691896262640, -171.6250000000000284 ) ) ;
#15385=CARTESIAN_POINT ( 'NONE',  ( -6.979918204473413823, 8.247283589362350398, -99.99999999999998579 ) ) ;
#15386=CARTESIAN_POINT ( 'NONE',  ( 10.81189881249999551, -6.242252689847874514, -170.9687500020483810 ) ) ;
#15391=CARTESIAN_POINT ( 'NONE',  ( -10.81189881249999907, -6.242252689847864744, -33.65625000204835970 ) ) ;
#15393=CARTESIAN_POINT ( 'NONE',  ( -5.000000000000003553, -8.660254037844383745, -101.5000000000000000 ) ) ;
#15395=CARTESIAN_POINT ( 'NONE',  ( -5.405949406250003975, -9.363379034771801557, -117.5312500020483952 ) ) ;
#15396=CARTESIAN_POINT ( 'NONE',  ( -5.000000000000003553, -8.660254037844383745, -140.8750000040967905 ) ) ;
#15402=CARTESIAN_POINT ( 'NONE',  ( 7.644554776091147741E-16, 12.48450537969573659, -65.65625000204838102 ) ) ;
#15408=ORIENTED_EDGE ( 'NONE', *, *, #29872, .T. ) ;
#15411=( BOUNDED_CURVE ( )  B_SPLINE_CURVE ( 2, ( #374, #3813, #35979, #23029, #33390, #40047, #9645 ),
 .UNSPECIFIED., .F., .F. ) 
 B_SPLINE_CURVE_WITH_KNOTS ( ( 3, 2, 2, 3 ),
 ( 0.1902985074626866169, 0.1915422885572139744, 0.1927860696517413319, 0.1940298507462686894 ),
 .UNSPECIFIED. ) 
 CURVE ( )  GEOMETRIC_REPRESENTATION_ITEM ( )  RATIONAL_B_SPLINE_CURVE ( ( 0.9999999999999940048, 0.8660254037844447028, 1.000000000000000000, 0.8660254037844387076, 1.000000000000000000, 0.8660254037844357100, 1.000000000000003109 ) ) 
 REPRESENTATION_ITEM ( '' )  );
#15420=( BOUNDED_CURVE ( )  B_SPLINE_CURVE ( 2, ( #39294, #29813, #36281, #32837, #33049, #254, #13375 ),
 .UNSPECIFIED., .F., .F. ) 
 B_SPLINE_CURVE_WITH_KNOTS ( ( 3, 2, 2, 3 ),
 ( 0.2835820895522389029, 0.2848258706467662882, 0.2860696517412936180, 0.2873134328358210032 ),
 .UNSPECIFIED. ) 
 CURVE ( )  GEOMETRIC_REPRESENTATION_ITEM ( )  RATIONAL_B_SPLINE_CURVE ( ( 0.9999999999999880096, 0.8660254037844506980, 1.000000000000000000, 0.8660254037844387076, 1.000000000000000000, 0.8660254037844267172, 1.000000000000011990 ) ) 
 REPRESENTATION_ITEM ( '' )  );
#15421=DIRECTION ( 'NONE',  ( -0.000000000000000000, -0.000000000000000000, -1.000000000000000000 ) ) ;
#15425=CARTESIAN_POINT ( 'NONE',  ( 0.000000000000000000, 0.000000000000000000, -180.0000000000000000 ) ) ;
#15426=CARTESIAN_POINT ( 'NONE',  ( -5.000000000000003553, -8.660254037844383745, -38.49999999999997868 ) ) ;
#15429=CARTESIAN_POINT ( 'NONE',  ( -2.293366432827344421E-15, -12.48450537969573659, -160.7187500020483810 ) ) ;
#15430=CARTESIAN_POINT ( 'NONE',  ( 5.405949406249992428, -9.363379034771808662, -166.5937500020484094 ) ) ;
#15434=CARTESIAN_POINT ( 'NONE',  ( -2.121150477449813534E-15, -11.54700538379251284, -198.8750000000000284 ) ) ;
#15439=CARTESIAN_POINT ( 'NONE',  ( -5.405949406250003975, -9.363379034771801557, -68.03125000204838102 ) ) ;
#15441=CARTESIAN_POINT ( 'NONE',  ( 10.00000000000000000, 5.773502691896255534, -126.3749999999999858 ) ) ;
#15443=CARTESIAN_POINT ( 'NONE',  ( 5.405949406249999534, 9.363379034771803333, -152.7812500020484094 ) ) ;
#15444=CARTESIAN_POINT ( 'NONE',  ( 10.81189881249999907, 6.242252689847868297, -164.9062500020484094 ) ) ;
#15448=CARTESIAN_POINT ( 'NONE',  ( -10.81189881249999729, 6.242252689847871849, -95.21875000204838102 ) ) ;
#15451=CARTESIAN_POINT ( 'NONE',  ( -2.293366432827344421E-15, -12.48450537969573659, -196.7187500020484094 ) ) ;
#15453=CARTESIAN_POINT ( 'NONE',  ( 7.428843778402297815, -7.774210255481911247, -179.9999999999999716 ) ) ;
#15454=CARTESIAN_POINT ( 'NONE',  ( -2.121150477449813534E-15, -11.54700538379251284, -144.8750000000000000 ) ) ;
#15455=CARTESIAN_POINT ( 'NONE',  ( -2.293366432827344421E-15, -12.48450537969573659, -91.90625000204838102 ) ) ;
#15457=CARTESIAN_POINT ( 'NONE',  ( 7.070501591499377789E-16, 11.54700538379251284, -69.50000000409679046 ) ) ;
#15459=CARTESIAN_POINT ( 'NONE',  ( 5.405949406249999534, 9.363379034771803333, -28.09375000204836326 ) ) ;
#15460=CARTESIAN_POINT ( 'NONE',  ( -9.999999999999998224, 1.224646799147353059E-15, -100.2499999999999858 ) ) ;
#15462=CARTESIAN_POINT ( 'NONE',  ( -5.405949406250003975, -9.363379034771801557, -21.53125000204836326 ) ) ;
#15471=ORIENTED_EDGE ( 'NONE', *, *, #39473, .F. ) ;
#15476=CARTESIAN_POINT ( 'NONE',  ( -5.000000000000003553, -8.660254037844383745, -173.5000000000000284 ) ) ;
#15479=CARTESIAN_POINT ( 'NONE',  ( -10.81189881249999729, 1.324075727343319199E-15, -165.7812500020484094 ) ) ;
#15484=CARTESIAN_POINT ( 'NONE',  ( 5.405949406249999534, 9.363379034771803333, -85.09375000204836681 ) ) ;
#15485=CARTESIAN_POINT ( 'NONE',  ( 10.81189881249999907, 6.242252689847868297, -91.40625000204836681 ) ) ;
#15489=CARTESIAN_POINT ( 'NONE',  ( -10.81189881249999729, 6.242252689847871849, -173.4062500020483810 ) ) ;
#15490=CARTESIAN_POINT ( 'NONE',  ( 10.81189881249999551, -6.242252689847874514, -189.1562500020484379 ) ) ;
#15492=CARTESIAN_POINT ( 'NONE',  ( -9.999999999999998224, 5.773502691896259087, -165.2500000040967905 ) ) ;
#15494=CARTESIAN_POINT ( 'NONE',  ( -2.293366432827344421E-15, -12.48450537969573659, -15.21875000204836326 ) ) ;
#15495=CARTESIAN_POINT ( 'NONE',  ( -10.81189881249999729, 6.242252689847871849, -120.7187500020483952 ) ) ;
#15497=CARTESIAN_POINT ( 'NONE',  ( 5.405949406249999534, 9.363379034771803333, -23.78125000204836681 ) ) ;
#15501=CARTESIAN_POINT ( 'NONE',  ( -5.405949406249996869, 9.363379034771805109, -115.0312500020483952 ) ) ;
#15503=EDGE_LOOP ( 'NONE', ( #39360, #7610, #8107, #14885 ) ) ;
#15505=CARTESIAN_POINT ( 'NONE',  ( -2.121150477449813534E-15, -11.54700538379251284, -94.25000000409677625 ) ) ;
#15508=CARTESIAN_POINT ( 'NONE',  ( -10.81189881249999729, 1.324075727343319199E-15, -50.09375000204835260 ) ) ;
#15509=VERTEX_POINT ( 'NONE', #34231 ) ;
#15513=CARTESIAN_POINT ( 'NONE',  ( -2.121150477449813534E-15, -11.54700538379251284, -16.25000000409676559 ) ) ;
#15520=ORIENTED_EDGE ( 'NONE', *, *, #4340, .T. ) ;
#15525=VERTEX_POINT ( 'NONE', #8105 ) ;
#15526=VECTOR ( 'NONE', #36545, 1000.000000000000114 ) ;
#15530=CARTESIAN_POINT ( 'NONE',  ( 5.405949406249992428, -9.363379034771808662, -189.2812500020484094 ) ) ;
#15532=DIRECTION ( 'NONE',  ( 0.000000000000000000, 0.000000000000000000, 1.000000000000000000 ) ) ;
#15535=CARTESIAN_POINT ( 'NONE',  ( -10.81189881249999729, 1.324075727343319199E-15, -113.0937500020483810 ) ) ;
#15537=CARTESIAN_POINT ( 'NONE',  ( -5.405949406249996869, 9.363379034771805109, -119.5312500020483952 ) ) ;
#15539=CARTESIAN_POINT ( 'NONE',  ( 7.644554776091147741E-16, 12.48450537969573659, -123.9687500020483952 ) ) ;
#15543=CARTESIAN_POINT ( 'NONE',  ( 9.999999999999996447, -5.773502691896262640, -140.1250000000000000 ) ) ;
#15544=CARTESIAN_POINT ( 'NONE',  ( 7.070501591499377789E-16, 11.54700538379251284, -12.12499999999996980 ) ) ;
#15547=CARTESIAN_POINT ( 'NONE',  ( -9.999999999999998224, 1.224646799147353059E-15, -186.1250000040967905 ) ) ;
#15549=CARTESIAN_POINT ( 'NONE',  ( 10.81189881249999729, 0.000000000000000000, -40.34375000204837391 ) ) ;
#15550=CARTESIAN_POINT ( 'NONE',  ( -9.999999999999479527, -5.773502691896549521, -106.1249999999999716 ) ) ;
#15551=CARTESIAN_POINT ( 'NONE',  ( 10.81189881249999551, -6.242252689847874514, -146.9687500020484094 ) ) ;
#15554=AXIS2_PLACEMENT_3D ( 'NONE', #25334, #12768, #41916 ) ;
#15555=CARTESIAN_POINT ( 'NONE',  ( 4.999999999999992006, -8.660254037844389075, -75.74999999999998579 ) ) ;
#15556=CARTESIAN_POINT ( 'NONE',  ( -10.81189881249999729, 6.242252689847871849, -140.4062500020484094 ) ) ;
#15561=CARTESIAN_POINT ( 'NONE',  ( -9.999999999999998224, 1.224646799147353059E-15, -118.6250000040967905 ) ) ;
#15563=CARTESIAN_POINT ( 'NONE',  ( -5.405949406249996869, 9.363379034771805109, -77.34375000204838102 ) ) ;
#15567=CARTESIAN_POINT ( 'NONE',  ( -9.999999999999998224, 1.224646799147353059E-15, -118.6250000040967905 ) ) ;
#15568=CARTESIAN_POINT ( 'NONE',  ( 7.644554776091147741E-16, 12.48450537969573659, -34.15625000204835970 ) ) ;
#15572=EDGE_CURVE ( 'NONE', #33599, #7201, #36630, .T. ) ;
#15585=CARTESIAN_POINT ( 'NONE',  ( 5.405949406249999534, 9.363379034771803333, -133.0937500020483810 ) ) ;
#15586=CARTESIAN_POINT ( 'NONE',  ( -10.81189881249999729, 6.242252689847871849, -137.4062500020484094 ) ) ;
#15588=CARTESIAN_POINT ( 'NONE',  ( 5.405949406249999534, 9.363379034771803333, -145.0937500020483810 ) ) ;
#15591=CARTESIAN_POINT ( 'NONE',  ( 7.070501591499377789E-16, 11.54700538379251284, -168.1250000000000000 ) ) ;
#15594=CARTESIAN_POINT ( 'NONE',  ( -10.81189881249999729, 1.324075727343319199E-15, -63.59375000204836681 ) ) ;
#15596=CARTESIAN_POINT ( 'NONE',  ( -10.81189881249999907, -6.242252689847864744, -169.9687500020484094 ) ) ;
#15600=CARTESIAN_POINT ( 'NONE',  ( 10.81189881249999907, 6.242252689847868297, -40.40625000204836681 ) ) ;
#15602=CARTESIAN_POINT ( 'NONE',  ( -4.999999999999996447, 8.660254037844387298, -100.4999999999999858 ) ) ;
#15604=CARTESIAN_POINT ( 'NONE',  ( 10.81189881249999729, 6.242252689847867408, -119.9062500020483810 ) ) ;
#15605=CARTESIAN_POINT ( 'NONE',  ( 9.999999999999996447, -5.773502691896262640, -139.0000000040967905 ) ) ;
#15610=CARTESIAN_POINT ( 'NONE',  ( -10.81189881249999729, 1.324075727343319199E-15, -63.78125000204837391 ) ) ;
#15611=CARTESIAN_POINT ( 'NONE',  ( -9.999999999999998224, 1.224646799147353059E-15, -147.1250000040967905 ) ) ;
#15613=CARTESIAN_POINT ( 'NONE',  ( -9.999999999999227285, -5.773502691896698735, -106.5000000040967336 ) ) ;
#15616=ORIENTED_EDGE ( 'NONE', *, *, #22890, .F. ) ;
#15629=ORIENTED_EDGE ( 'NONE', *, *, #18282, .T. ) ;
#15630=CARTESIAN_POINT ( 'NONE',  ( 10.00000000000051159, -5.773502691895965988, -109.0000000040967620 ) ) ;
#15631=CARTESIAN_POINT ( 'NONE',  ( 9.999999999999998224, 0.000000000000000000, -37.99999999999997868 ) ) ;
#15635=CARTESIAN_POINT ( 'NONE',  ( -2.293366432827344421E-15, -12.48450537969573659, -156.2187500020483810 ) ) ;
#15636=CARTESIAN_POINT ( 'NONE',  ( 5.405949406249999534, 9.363379034771803333, -169.0937500020484094 ) ) ;
#15639=ADVANCED_FACE ( 'NONE', ( #33798 ), #17574, .F. ) ;
#15640=CARTESIAN_POINT ( 'NONE',  ( 7.070501591499377789E-16, 11.54700538379251284, -196.6250000000000284 ) ) ;
#15646=CARTESIAN_POINT ( 'NONE',  ( 5.405949406249999534, 9.363379034771803333, -58.28125000204836681 ) ) ;
#15648=CARTESIAN_POINT ( 'NONE',  ( -10.00000000000000000, -5.773502691896251982, -121.1250000000000000 ) ) ;
#15650=CARTESIAN_POINT ( 'NONE',  ( -5.405949406250003975, -9.363379034771801557, -143.0312500020483810 ) ) ;
#15651=CARTESIAN_POINT ( 'NONE',  ( 10.81189881249999907, 6.242252689847868297, -155.9062500020484094 ) ) ;
#15654=CARTESIAN_POINT ( 'NONE',  ( 10.81189881249999551, -6.242252689847874514, -91.46875000204838102 ) ) ;
#15657=CARTESIAN_POINT ( 'NONE',  ( -10.81189881249999907, -6.242252689847864744, -184.9687500020484094 ) ) ;
#15661=CARTESIAN_POINT ( 'NONE',  ( -10.81189881249999729, 1.324075727343319199E-15, -92.28125000204838102 ) ) ;
#15664=CARTESIAN_POINT ( 'NONE',  ( -10.00000000000000000, -5.773502691896251982, -66.00000000409679046 ) ) ;
#15666=CARTESIAN_POINT ( 'NONE',  ( 5.405949406249999534, 9.363379034771803333, -22.09375000204835615 ) ) ;
#15669=CARTESIAN_POINT ( 'NONE',  ( 10.81189881249999551, -6.242252689847874514, -19.65625000204837747 ) ) ;
#15671=CARTESIAN_POINT ( 'NONE',  ( -9.999999999999998224, 1.224646799147353059E-15, -117.1250000040967905 ) ) ;
#15672=CARTESIAN_POINT ( 'NONE',  ( -5.000000000000003553, -8.660254037844383745, 0.1249999959032355168 ) ) ;
#15674=ADVANCED_FACE ( 'NONE', ( #1208 ), #24308, .F. ) ;
#15679=CARTESIAN_POINT ( 'NONE',  ( 10.00000000000000000, 5.773502691896255534, -170.2500000040967905 ) ) ;
#15680=ORIENTED_EDGE ( 'NONE', *, *, #36507, .F. ) ;
#15681=ORIENTED_EDGE ( 'NONE', *, *, #7351, .T. ) ;
#15693=CARTESIAN_POINT ( 'NONE',  ( -10.81189881249999907, -6.242252689847864744, -158.1562500020484094 ) ) ;
#15695=CARTESIAN_POINT ( 'NONE',  ( -2.121150477449813534E-15, -11.54700538379251284, -172.2500000040968189 ) ) ;
#15698=CARTESIAN_POINT ( 'NONE',  ( 10.81189881249999729, 0.000000000000000000, -80.84375000204838102 ) ) ;
#15699=CARTESIAN_POINT ( 'NONE',  ( 10.81189881249999551, -6.242252689847874514, -84.15625000204838102 ) ) ;
#15702=CARTESIAN_POINT ( 'NONE',  ( -10.81189881249999729, 6.242252689847871849, -170.4062500020484094 ) ) ;
#15703=CARTESIAN_POINT ( 'NONE',  ( 10.81189881249999907, 6.242252689847868297, -182.9062500020484094 ) ) ;
#15705=CARTESIAN_POINT ( 'NONE',  ( 10.00000000000000000, 5.773502691896255534, -162.7500000040967905 ) ) ;
#15707=CARTESIAN_POINT ( 'NONE',  ( 7.644554776091147741E-16, 12.48450537969573659, -11.46875000204836148 ) ) ;
#15709=CARTESIAN_POINT ( 'NONE',  ( -10.81189881249999729, 6.242252689847871849, -117.7187500020483952 ) ) ;
#15711=CARTESIAN_POINT ( 'NONE',  ( 10.81189881249999729, 0.000000000000000000, -24.03125000204836681 ) ) ;
#15714=CARTESIAN_POINT ( 'NONE',  ( 10.81189881249999551, -6.242252689847874514, -112.6562500020483810 ) ) ;
#15717=CARTESIAN_POINT ( 'NONE',  ( 5.000000000000000000, 8.660254037844385522, -92.12500000409677625 ) ) ;
#15718=CARTESIAN_POINT ( 'NONE',  ( -5.000000000000003553, -8.660254037844383745, -99.99999999999998579 ) ) ;
#15720=CARTESIAN_POINT ( 'NONE',  ( -5.405949406250003975, -9.363379034771801557, -49.84375000204838102 ) ) ;
#15725=CARTESIAN_POINT ( 'NONE',  ( -2.121150477449813534E-15, -11.54700538379251284, -17.75000000409676559 ) ) ;
#15726=LINE ( 'NONE', #12695, #8438 ) ;
#15728=EDGE_LOOP ( 'NONE', ( #14050, #42202, #12063, #18338 ) ) ;
#15733=EDGE_CURVE ( 'NONE', #19924, #35515, #12160, .T. ) ;
#15737=CARTESIAN_POINT ( 'NONE',  ( 9.999999999999479527, 5.773502691896553074, -175.8749999999999716 ) ) ;
#15740=CARTESIAN_POINT ( 'NONE',  ( 5.405949406249992428, -9.363379034771808662, -180.2812500020484094 ) ) ;
#15744=( BOUNDED_CURVE ( )  B_SPLINE_CURVE ( 2, ( #25443, #35155, #25234, #15695, #18522, #5580, #1927 ),
 .UNSPECIFIED., .F., .F. ) 
 B_SPLINE_CURVE_WITH_KNOTS ( ( 3, 2, 2, 3 ),
 ( 0.1305970149253731227, 0.1318407960199005080, 0.1330845771144278378, 0.1343283582089551953 ),
 .UNSPECIFIED. ) 
 CURVE ( )  GEOMETRIC_REPRESENTATION_ITEM ( )  RATIONAL_B_SPLINE_CURVE ( ( 1.000000000000000000, 0.8660254037844387076, 1.000000000000000000, 0.8660254037844387076, 1.000000000000000000, 0.8660254037844417052, 0.9999999999999970024 ) ) 
 REPRESENTATION_ITEM ( '' )  );
#15745=CARTESIAN_POINT ( 'NONE',  ( -10.81189881249999907, -6.242252689847864744, -112.9687500020483810 ) ) ;
#15747=CARTESIAN_POINT ( 'NONE',  ( -5.405949406250003975, -9.363379034771801557, -113.0312500020483952 ) ) ;
#15749=CARTESIAN_POINT ( 'NONE',  ( 7.644554776091147741E-16, 12.48450537969573659, -125.4687500020483952 ) ) ;
#15753=CARTESIAN_POINT ( 'NONE',  ( 10.00000000000000000, 5.773502691896255534, -141.3750000000000000 ) ) ;
#15754=CARTESIAN_POINT ( 'NONE',  ( 9.999999999999996447, -5.773502691896262640, -11.12499999999996980 ) ) ;
#15757=CARTESIAN_POINT ( 'NONE',  ( -9.999999999999998224, 1.224646799147353059E-15, -189.1250000040967905 ) ) ;
#15759=CARTESIAN_POINT ( 'NONE',  ( -5.405949406249996869, 9.363379034771805109, -35.34375000204836681 ) ) ;
#15761=CARTESIAN_POINT ( 'NONE',  ( 7.644554776091147741E-16, 12.48450537969573659, -146.4687500020484094 ) ) ;
#15764=CARTESIAN_POINT ( 'NONE',  ( 7.070501591499377789E-16, 11.54700538379251284, -67.62500000000000000 ) ) ;
#15765=CARTESIAN_POINT ( 'NONE',  ( -5.405949406250003975, -9.363379034771801557, -143.0312500020483810 ) ) ;
#15769=CARTESIAN_POINT ( 'NONE',  ( -4.999999999999996447, 8.660254037844387298, -118.8750000040967905 ) ) ;
#15770=CARTESIAN_POINT ( 'NONE',  ( 9.999999999999998224, 0.000000000000000000, -170.0000000000000000 ) ) ;
#15771=CARTESIAN_POINT ( 'NONE',  ( -5.405949406250003975, -9.363379034771801557, -70.84375000204836681 ) ) ;
#15775=CARTESIAN_POINT ( 'NONE',  ( -9.999999999999998224, 1.224646799147353059E-15, -132.1250000040967620 ) ) ;
#15776=CARTESIAN_POINT ( 'NONE',  ( -5.405949406250003975, -9.363379034771801557, -35.03125000204837391 ) ) ;
#15777=CARTESIAN_POINT ( 'NONE',  ( -9.999999999999998224, 1.224646799147353059E-15, -139.2499999999999716 ) ) ;
#15780=CARTESIAN_POINT ( 'NONE',  ( -10.00000000000000000, -5.773502691896252870, -165.0000000040967905 ) ) ;
#15783=AXIS2_PLACEMENT_3D ( 'NONE', #4046, #13943, #4261 ) ;
#15784=ORIENTED_EDGE ( 'NONE', *, *, #20684, .F. ) ;
#15786=CARTESIAN_POINT ( 'NONE',  ( 9.999999999999998224, 0.000000000000000000, -176.3750000040967905 ) ) ;
#15791=CARTESIAN_POINT ( 'NONE',  ( -2.121150477449813534E-15, -11.54700538379251284, -130.2500000040967905 ) ) ;
#15795=CARTESIAN_POINT ( 'NONE',  ( 10.81189881249999551, -6.242252689847874514, -131.9687500020483810 ) ) ;
#15796=CARTESIAN_POINT ( 'NONE',  ( 5.405949406249999534, 9.363379034771803333, -143.7812500020483810 ) ) ;
#15798=CARTESIAN_POINT ( 'NONE',  ( 5.405949406249999534, 9.363379034771803333, -143.5937500020483810 ) ) ;
#15801=CARTESIAN_POINT ( 'NONE',  ( -9.999999999999998224, 1.224646799147353059E-15, -163.2500000000000000 ) ) ;
#15804=CARTESIAN_POINT ( 'NONE',  ( -2.293366432827344421E-15, -12.48450537969573659, -64.71875000204838102 ) ) ;
#15807=CARTESIAN_POINT ( 'NONE',  ( 10.81189881249999729, 0.000000000000000000, -173.8437500020484094 ) ) ;
#15812=CARTESIAN_POINT ( 'NONE',  ( 10.00000000000000000, 5.773502691896255534, -88.87499999999998579 ) ) ;
#15814=CARTESIAN_POINT ( 'NONE',  ( -5.405949406249996869, 9.363379034771805109, -118.0312500020483952 ) ) ;
#15815=CARTESIAN_POINT ( 'NONE',  ( -4.999999999999996447, 8.660254037844387298, -136.8750000040967905 ) ) ;
#15821=CARTESIAN_POINT ( 'NONE',  ( -10.81189881249999907, -6.242252689847864744, -62.15625000204838102 ) ) ;
#15831=EDGE_LOOP ( 'NONE', ( #39761, #3073, #15838 ) ) ;
#15832=VERTEX_POINT ( 'NONE', #38091 ) ;
#15834=CARTESIAN_POINT ( 'NONE',  ( 9.999999999999479527, 5.773502691896553074, -126.7500000040967478 ) ) ;
#15838=ORIENTED_EDGE ( 'NONE', *, *, #15572, .F. ) ;
#15839=CARTESIAN_POINT ( 'NONE',  ( -9.999999999999227285, -5.773502691896698735, -109.5000000040967478 ) ) ;
#15840=CARTESIAN_POINT ( 'NONE',  ( 10.00000000000000000, 5.773502691896255534, -25.87499999999998224 ) ) ;
#15843=CARTESIAN_POINT ( 'NONE',  ( 5.405949406249999534, 9.363379034771803333, -160.0937500020484094 ) ) ;
#15844=CARTESIAN_POINT ( 'NONE',  ( 5.405949406249992428, -9.363379034771808662, -172.5937500020484094 ) ) ;
#15846=CARTESIAN_POINT ( 'NONE',  ( -9.999999999999998224, 1.224646799147353059E-15, -127.2499999999999716 ) ) ;
#15847=CARTESIAN_POINT ( 'NONE',  ( -10.00000000000000000, -5.773502691896251982, -185.6250000000000284 ) ) ;
#15854=EDGE_CURVE ( 'NONE', #5830, #15993, #29830, .T. ) ;
#15855=CARTESIAN_POINT ( 'NONE',  ( 5.405949406249992428, -9.363379034771808662, -60.28125000204836681 ) ) ;
#15857=CARTESIAN_POINT ( 'NONE',  ( -9.999999999999998224, 1.224646799147353059E-15, -124.2500000000000000 ) ) ;
#15859=CARTESIAN_POINT ( 'NONE',  ( -2.293366432827344421E-15, -12.48450537969573659, -139.9062500020484094 ) ) ;
#15860=CARTESIAN_POINT ( 'NONE',  ( 5.405949406249992428, -9.363379034771808662, -154.7812500020484094 ) ) ;
#15862=CARTESIAN_POINT ( 'NONE',  ( 5.405949406249999534, 9.363379034771803333, -92.59375000204838102 ) ) ;
#15865=CARTESIAN_POINT ( 'NONE',  ( 10.81189881249999729, 0.000000000000000000, -187.3437500020483810 ) ) ;
#15867=DIRECTION ( 'NONE',  ( -0.000000000000000000, -0.000000000000000000, -1.000000000000000000 ) ) ;
#15868=CARTESIAN_POINT ( 'NONE',  ( -2.293366432827344421E-15, -12.48450537969573659, -87.40625000204838102 ) ) ;
#15870=CARTESIAN_POINT ( 'NONE',  ( -10.00000000000000000, -5.773502691896251982, -61.50000000409677625 ) ) ;
#15871=CARTESIAN_POINT ( 'NONE',  ( -5.405949406249996869, 9.363379034771805109, -14.34375000204834905 ) ) ;
#15875=CARTESIAN_POINT ( 'NONE',  ( -10.81189881249999729, 6.242252689847871849, -8.406250002048365033 ) ) ;
#15892=DIRECTION ( 'NONE',  ( 0.7071067811865463515, 8.659560562354918067E-17, -0.7071067811865487940 ) ) ;
#15895=CARTESIAN_POINT ( 'NONE',  ( 10.81189881249999907, 6.242252689847868297, -158.9062500020483810 ) ) ;
#15897=FACE_OUTER_BOUND ( 'NONE', #23241, .T. ) ;
#15903=CARTESIAN_POINT ( 'NONE',  ( 7.644554776091147741E-16, 12.48450537969573659, -75.96875000204838102 ) ) ;
#15904=CARTESIAN_POINT ( 'NONE',  ( 5.405949406249999534, 9.363379034771803333, -86.78125000204838102 ) ) ;
#15909=CARTESIAN_POINT ( 'NONE',  ( 10.81189881249999729, 0.000000000000000000, -168.0312500020484094 ) ) ;
#15910=CARTESIAN_POINT ( 'NONE',  ( 7.644554776091147741E-16, 12.48450537969573659, -178.1562500020484094 ) ) ;
#15912=CARTESIAN_POINT ( 'NONE',  ( 9.999999999999996447, -5.773502691896262640, -152.5000000040967905 ) ) ;
#15914=CARTESIAN_POINT ( 'NONE',  ( -10.81189881249999729, 6.242252689847871849, -2.218750002048353043 ) ) ;
#15915=CARTESIAN_POINT ( 'NONE',  ( -10.00000000000012434, 5.773502691896184480, -162.2500000040967905 ) ) ;
#15916=CARTESIAN_POINT ( 'NONE',  ( 7.644554776091147741E-16, 12.48450537969573659, -113.4687500020483952 ) ) ;
#15918=CARTESIAN_POINT ( 'NONE',  ( 5.405949406249999534, 9.363379034771803333, -11.78125000204835438 ) ) ;
#15922=CARTESIAN_POINT ( 'NONE',  ( 5.405949406249992428, -9.363379034771808662, -111.2812500020483810 ) ) ;
#15924=VERTEX_POINT ( 'NONE', #13642 ) ;
#15925=CARTESIAN_POINT ( 'NONE',  ( 5.000000000000000000, 8.660254037844385522, -84.62500000409677625 ) ) ;
#15926=CARTESIAN_POINT ( 'NONE',  ( -9.999999999999998224, 1.224646799147353059E-15, -101.7500000000000000 ) ) ;
#15927=CARTESIAN_POINT ( 'NONE',  ( 10.81189881249999907, 6.242252689847868297, -38.71875000204835260 ) ) ;
#15928=ORIENTED_EDGE ( 'NONE', *, *, #31528, .F. ) ;
#15932=CARTESIAN_POINT ( 'NONE',  ( 10.00000000000000000, 5.773502691896255534, -17.25000000409676559 ) ) ;
#15945=EDGE_LOOP ( 'NONE', ( #28396, #14233, #4117, #33315 ) ) ;
#15946=ORIENTED_EDGE ( 'NONE', *, *, #7249, .F. ) ;
#15949=CARTESIAN_POINT ( 'NONE',  ( -5.405949406250003975, -9.363379034771801557, -183.5312500020484094 ) ) ;
#15951=CARTESIAN_POINT ( 'NONE',  ( -2.121150477449813534E-15, -11.54700538379251284, -132.8750000000000000 ) ) ;
#15954=CARTESIAN_POINT ( 'NONE',  ( 10.81189881249999551, -6.242252689847874514, -101.9687500020483810 ) ) ;
#15956=CARTESIAN_POINT ( 'NONE',  ( -5.405949406249996869, 9.363379034771805109, -106.0312500020483810 ) ) ;
#15958=CARTESIAN_POINT ( 'NONE',  ( -5.405949406250003975, -9.363379034771801557, -123.3437500020483952 ) ) ;
#15962=CARTESIAN_POINT ( 'NONE',  ( -10.00000000000000000, -5.773502691896251982, -140.6249999999999716 ) ) ;
#15963=CARTESIAN_POINT ( 'NONE',  ( -2.121150477449813534E-15, -11.54700538379251284, -3.874999999999961808 ) ) ;
#15966=CARTESIAN_POINT ( 'NONE',  ( -4.999999999999996447, 8.660254037844387298, -178.8750000040967905 ) ) ;
#15968=CARTESIAN_POINT ( 'NONE',  ( 5.405949406249992428, -9.363379034771808662, -28.59375000204836326 ) ) ;
#15969=CARTESIAN_POINT ( 'NONE',  ( -5.000000000000003553, -8.660254037844383745, -142.3750000040967905 ) ) ;
#15970=CARTESIAN_POINT ( 'NONE',  ( 10.81189881249999729, 0.000000000000000000, -140.8437500020483810 ) ) ;
#15973=CARTESIAN_POINT ( 'NONE',  ( 5.000000000000000000, 8.660254037844385522, -70.74999999999998579 ) ) ;
#15974=CARTESIAN_POINT ( 'NONE',  ( -10.81189881249999729, 1.324075727343319199E-15, -131.2812500020483810 ) ) ;
#15978=CARTESIAN_POINT ( 'NONE',  ( 10.00000000000000000, 5.773502691896255534, -114.7500000040967763 ) ) ;
#15980=CARTESIAN_POINT ( 'NONE',  ( -5.405949406249996869, 9.363379034771805109, -62.34375000204836681 ) ) ;
#15986=CARTESIAN_POINT ( 'NONE',  ( -9.999999999999998224, 1.224646799147353059E-15, -46.62500000409677625 ) ) ;
#15987=CARTESIAN_POINT ( 'NONE',  ( 5.405949406249999534, 9.363379034771803333, -32.78125000204837391 ) ) ;
#15988=DIRECTION ( 'NONE',  ( -0.000000000000000000, -0.000000000000000000, -1.000000000000000000 ) ) ;
#15993=VERTEX_POINT ( 'NONE', #13219 ) ;
#15997=CARTESIAN_POINT ( 'NONE',  ( 10.00000000000000000, 5.773502691896255534, -135.7500000040967905 ) ) ;
#16003=LINE ( 'NONE', #19052, #7280 ) ;
#16004=CARTESIAN_POINT ( 'NONE',  ( -5.405949406250003975, -9.363379034771801557, -124.8437500020483810 ) ) ;
#16005=CARTESIAN_POINT ( 'NONE',  ( -5.405949406250003975, -9.363379034771801557, -132.5312500020484094 ) ) ;
#16007=CARTESIAN_POINT ( 'NONE',  ( -10.81189881249999729, 6.242252689847871849, -147.7187500020484094 ) ) ;
#16010=CARTESIAN_POINT ( 'NONE',  ( -10.00000000000000000, -5.773502691896251982, -166.1249999999999716 ) ) ;
#16011=CARTESIAN_POINT ( 'NONE',  ( -5.405949406250003975, -9.363379034771801557, -0.5312500020483723606 ) ) ;
#16014=CARTESIAN_POINT ( 'NONE',  ( -5.405949406250003975, -9.363379034771801557, -63.34375000204836681 ) ) ;
#16015=CARTESIAN_POINT ( 'NONE',  ( 9.999999999999998224, 1.224646799147353059E-15, -99.99999999999998579 ) ) ;
#16016=CARTESIAN_POINT ( 'NONE',  ( -10.81189881249999907, -6.242252689847864744, -160.9687500020484094 ) ) ;
#16019=LINE ( 'NONE', #12787, #9614 ) ;
#16021=CARTESIAN_POINT ( 'NONE',  ( -10.00000000000000000, -5.773502691896251982, -91.12499999999998579 ) ) ;
#16023=CARTESIAN_POINT ( 'NONE',  ( -10.81189881249999729, 1.324075727343319199E-15, -114.7812500020483952 ) ) ;
#16024=CARTESIAN_POINT ( 'NONE',  ( 9.999999999999998224, 0.000000000000000000, -138.8750000040968189 ) ) ;
#16030=CARTESIAN_POINT ( 'NONE',  ( -10.81189881249999907, -6.242252689847864744, -63.65625000204838102 ) ) ;
#16039=( BOUNDED_CURVE ( )  B_SPLINE_CURVE ( 2, ( #31798, #34599, #31150, #37608, #2229, #41034, #8051 ),
 .UNSPECIFIED., .F., .F. ) 
 B_SPLINE_CURVE_WITH_KNOTS ( ( 3, 2, 2, 3 ),
 ( 0.3432835820895522860, 0.3445273631840797268, 0.3457711442786070566, 0.3470149253731344974 ),
 .UNSPECIFIED. ) 
 CURVE ( )  GEOMETRIC_REPRESENTATION_ITEM ( )  RATIONAL_B_SPLINE_CURVE ( ( 0.9999999999999940048, 0.8660254037844447028, 1.000000000000000000, 0.8660254037844387076, 1.000000000000000000, 0.8660254037844207220, 1.000000000000017986 ) ) 
 REPRESENTATION_ITEM ( '' )  );
#16041=VERTEX_POINT ( 'NONE', #19712 ) ;
#16051=CARTESIAN_POINT ( 'NONE',  ( -9.999999999999998224, 1.224646799147353059E-15, -172.6250000040968189 ) ) ;
#16052=CARTESIAN_POINT ( 'NONE',  ( 9.999999999999996447, -5.773502691896262640, -30.62499999999995737 ) ) ;
#16055=CARTESIAN_POINT ( 'NONE',  ( 5.405949406249999534, 9.363379034771803333, -148.0937500020483810 ) ) ;
#16056=CARTESIAN_POINT ( 'NONE',  ( -10.81189881249999729, -6.242252689847864744, -172.9687500020483526 ) ) ;
#16059=CARTESIAN_POINT ( 'NONE',  ( 9.999999999999996447, -5.773502691896262640, -188.1250000000000284 ) ) ;
#16064=CARTESIAN_POINT ( 'NONE',  ( -2.293366432827344421E-15, -12.48450537969573659, -195.2187500020484094 ) ) ;
#16066=CARTESIAN_POINT ( 'NONE',  ( 5.405949406249992428, -9.363379034771808662, -61.78125000204837391 ) ) ;
#16068=CARTESIAN_POINT ( 'NONE',  ( -10.00000000000000000, -5.773502691896251982, -112.1249999999999858 ) ) ;
#16070=CARTESIAN_POINT ( 'NONE',  ( 7.644554776091147741E-16, 12.48450537969573659, -143.6562500020484094 ) ) ;
#16071=CARTESIAN_POINT ( 'NONE',  ( 5.405949406249992428, -9.363379034771808662, -153.2812500020484094 ) ) ;
#16074=CARTESIAN_POINT ( 'NONE',  ( -5.405949406249996869, 9.363379034771805109, -93.84375000204838102 ) ) ;
#16077=CARTESIAN_POINT ( 'NONE',  ( -5.405949406250003975, -9.363379034771801557, -189.3437500020483810 ) ) ;
#16080=CARTESIAN_POINT ( 'NONE',  ( -2.293366432827344421E-15, -12.48450537969573659, -81.40625000204838102 ) ) ;
#16082=CARTESIAN_POINT ( 'NONE',  ( -4.999999999999996447, 8.660254037844387298, -58.87500000409676204 ) ) ;
#16083=CARTESIAN_POINT ( 'NONE',  ( 10.81189881249999551, -6.242252689847874514, -20.96875000204837036 ) ) ;
#16086=CARTESIAN_POINT ( 'NONE',  ( 10.81189881249999907, 6.242252689847868297, -10.40625000204836859 ) ) ;
#16087=CYLINDRICAL_SURFACE ( 'NONE', #20088, 9.999999999999998224 ) ;
#16094=ORIENTED_EDGE ( 'NONE', *, *, #16994, .F. ) ;
#16097=ORIENTED_EDGE ( 'NONE', *, *, #11416, .T. ) ;
#16106=CARTESIAN_POINT ( 'NONE',  ( 10.81189881249999729, 0.000000000000000000, -154.5312500020484094 ) ) ;
#16113=CARTESIAN_POINT ( 'NONE',  ( 5.405949406249999534, 9.363379034771803333, -77.59375000204838102 ) ) ;
#16114=CARTESIAN_POINT ( 'NONE',  ( 10.81189881249999907, 6.242252689847868297, -82.40625000204836681 ) ) ;
#16117=CARTESIAN_POINT ( 'NONE',  ( -2.293366432827344421E-15, -12.48450537969573659, -169.9062500020484379 ) ) ;
#16118=CARTESIAN_POINT ( 'NONE',  ( -10.81189881249999729, 1.324075727343319199E-15, -177.7812500020484094 ) ) ;
#16119=CARTESIAN_POINT ( 'NONE',  ( 5.000000000000000000, 8.660254037844385522, -158.1250000040967905 ) ) ;
#16121=CARTESIAN_POINT ( 'NONE',  ( 10.81189881249999729, 0.000000000000000000, -7.343750002048343717 ) ) ;
#16123=CARTESIAN_POINT ( 'NONE',  ( -10.81189881249999907, -6.242252689847864744, -117.4687500020483952 ) ) ;
#16125=CARTESIAN_POINT ( 'NONE',  ( -5.405949406249996869, 9.363379034771805109, -13.03125000204835615 ) ) ;
#16128=CARTESIAN_POINT ( 'NONE',  ( 5.405949406249992428, -9.363379034771808662, -108.2812500020483810 ) ) ;
#16131=CARTESIAN_POINT ( 'NONE',  ( -9.999999999999998224, 5.773502691896259087, -87.25000000409676204 ) ) ;
#16133=CARTESIAN_POINT ( 'NONE',  ( 10.81189881249999551, -6.242252689847874514, -38.96875000204835970 ) ) ;
#16137=CARTESIAN_POINT ( 'NONE',  ( 10.00000000000000000, 5.773502691896255534, -9.750000004096758488 ) ) ;
#16141=CARTESIAN_POINT ( 'NONE',  ( -9.999999999999742428, -5.773502691896402084, -152.6249999999999716 ) ) ;
#16155=CARTESIAN_POINT ( 'NONE',  ( 10.81189881249999551, -6.242252689847874514, -177.1562500020484094 ) ) ;
#16157=CARTESIAN_POINT ( 'NONE',  ( 10.00000000000051159, -5.773502691895965988, -146.5000000040967620 ) ) ;
#16160=CARTESIAN_POINT ( 'NONE',  ( -10.81189881249999729, 6.242252689847871849, -102.7187500020483810 ) ) ;
#16162=CARTESIAN_POINT ( 'NONE',  ( -5.405949406249996869, 9.363379034771805109, -110.5312500020483810 ) ) ;
#16164=CARTESIAN_POINT ( 'NONE',  ( -10.81189881249999729, -6.242252689847864744, -112.9687500020483810 ) ) ;
#16167=CARTESIAN_POINT ( 'NONE',  ( 7.070501591499377789E-16, 11.54700538379251284, -141.1250000000000000 ) ) ;
#16168=CARTESIAN_POINT ( 'NONE',  ( -10.00000000000000000, -5.773502691896251982, -4.124999999999961808 ) ) ;
#16169=EDGE_CURVE ( 'NONE', #22978, #14748, #31737, .T. ) ;
#16172=CARTESIAN_POINT ( 'NONE',  ( -10.00000000000000000, -5.773502691896251982, -180.0000000040967905 ) ) ;
#16174=CARTESIAN_POINT ( 'NONE',  ( 10.81189881249999551, -6.242252689847874514, -28.46875000204837391 ) ) ;
#16176=CARTESIAN_POINT ( 'NONE',  ( -10.81189881249999907, -6.242252689847864744, -135.4687500020483810 ) ) ;
#16178=CARTESIAN_POINT ( 'NONE',  ( -4.999999999999996447, 8.660254037844387298, -64.49999999999997158 ) ) ;
#16179=CARTESIAN_POINT ( 'NONE',  ( -10.81189881249999729, 6.242252689847871849, -135.9062500020484094 ) ) ;
#16183=CARTESIAN_POINT ( 'NONE',  ( -4.999999999999996447, 8.660254037844387298, -108.3750000040967763 ) ) ;
#16185=CARTESIAN_POINT ( 'NONE',  ( -5.405949406250003975, -9.363379034771801557, -69.34375000204836681 ) ) ;
#16192=CARTESIAN_POINT ( 'NONE',  ( -10.00000000000000000, -5.773502691896251982, -37.50000000409675494 ) ) ;
#16193=CARTESIAN_POINT ( 'NONE',  ( -5.405949406249996869, 9.363379034771805109, -38.53125000204838102 ) ) ;
#16197=CARTESIAN_POINT ( 'NONE',  ( -9.999999999999998224, 1.224646799147353059E-15, -150.1250000040967905 ) ) ;
#16201=CARTESIAN_POINT ( 'NONE',  ( -9.999999999999998224, 0.000000000000000000, -99.99999999999998579 ) ) ;
#16209=CARTESIAN_POINT ( 'NONE',  ( -10.81189881249999729, 1.324075727343319199E-15, -129.5937500020483810 ) ) ;
#16210=AXIS2_PLACEMENT_3D ( 'NONE', #13822, #17067, #33296 ) ;
#16211=CARTESIAN_POINT ( 'NONE',  ( -5.405949406249996869, 9.363379034771805109, -133.0312500020484094 ) ) ;
#16213=CARTESIAN_POINT ( 'NONE',  ( -10.81189881249999729, 1.324075727343319199E-15, -135.5937500020483810 ) ) ;
#16215=VECTOR ( 'NONE', #15988, 1000.000000000000000 ) ;
#16216=CARTESIAN_POINT ( 'NONE',  ( -2.121150477449813534E-15, -11.54700538379251284, -102.8749999999999858 ) ) ;
#16217=CARTESIAN_POINT ( 'NONE',  ( -5.000000000000003553, -8.660254037844383745, -160.0000000000000000 ) ) ;
#16221=CARTESIAN_POINT ( 'NONE',  ( 10.81189881249999551, -6.242252689847874514, -56.96875000204838102 ) ) ;
#16223=CARTESIAN_POINT ( 'NONE',  ( 7.644554776091147741E-16, 12.48450537969573659, -164.4687500020483810 ) ) ;
#16225=VECTOR ( 'NONE', #4983, 1000.000000000000000 ) ;
#16227=CARTESIAN_POINT ( 'NONE',  ( -9.999999999999998224, 1.224646799147353059E-15, -173.7500000000000284 ) ) ;
#16229=CARTESIAN_POINT ( 'NONE',  ( -9.999999999999998224, 5.773502691896259087, -88.37499999999998579 ) ) ;
#16231=CARTESIAN_POINT ( 'NONE',  ( 7.644554776091147741E-16, 12.48450537969573659, -119.6562500020484094 ) ) ;
#16232=CARTESIAN_POINT ( 'NONE',  ( -2.121150477449813534E-15, -11.54700538379251284, -134.7500000040967905 ) ) ;
#16233=CARTESIAN_POINT ( 'NONE',  ( -9.999999999999998224, 1.224646799147353059E-15, -176.7500000000000284 ) ) ;
#16237=CARTESIAN_POINT ( 'NONE',  ( -10.81189881249999729, 6.242252689847871849, -60.90625000204837391 ) ) ;
#16241=CARTESIAN_POINT ( 'NONE',  ( -4.999999999999996447, 8.660254037844387298, -166.8750000040967905 ) ) ;
#16242=DIRECTION ( 'NONE',  ( -0.000000000000000000, -0.000000000000000000, -1.000000000000000000 ) ) ;
#16257=CARTESIAN_POINT ( 'NONE',  ( -9.999999999999998224, 1.224646799147353059E-15, -143.7500000000000000 ) ) ;
#16258=CARTESIAN_POINT ( 'NONE',  ( 10.00000000000000000, 5.773502691896255534, -27.37499999999998224 ) ) ;
#16261=CARTESIAN_POINT ( 'NONE',  ( -2.293366432827344421E-15, -12.48450537969573659, -147.2187500020484094 ) ) ;
#16262=CARTESIAN_POINT ( 'NONE',  ( 10.81189881249999729, 0.000000000000000000, -169.3437500020484094 ) ) ;
#16264=CARTESIAN_POINT ( 'NONE',  ( -9.999999999999872102, -5.773502691896326589, -162.0000000040967620 ) ) ;
#16265=CARTESIAN_POINT ( 'NONE',  ( -9.999999999999998224, 5.773502691896259087, -187.3750000000000000 ) ) ;
#16270=CARTESIAN_POINT ( 'NONE',  ( 10.81189881249999551, -6.242252689847874514, -182.9687500020484094 ) ) ;
#16272=CARTESIAN_POINT ( 'NONE',  ( 10.81189881249999907, 6.242252689847868297, -62.90625000204838813 ) ) ;
#16274=CARTESIAN_POINT ( 'NONE',  ( 4.999999999999992006, -8.660254037844389075, -111.7499999999999858 ) ) ;
#16277=CARTESIAN_POINT ( 'NONE',  ( 10.81189881249999729, 0.000000000000000000, -139.5312500020484094 ) ) ;
#16279=CARTESIAN_POINT ( 'NONE',  ( -10.81189881249999907, -6.242252689847864744, -156.6562500020483810 ) ) ;
#16281=CARTESIAN_POINT ( 'NONE',  ( -9.999999999999998224, 1.224646799147353059E-15, -127.2499999999999716 ) ) ;
#16282=CARTESIAN_POINT ( 'NONE',  ( -10.81189881249999907, -6.242252689847864744, -87.46875000204838102 ) ) ;
#16285=CARTESIAN_POINT ( 'NONE',  ( -10.81189881249999907, -6.242252689847864744, -186.4687500020484094 ) ) ;
#16287=CARTESIAN_POINT ( 'NONE',  ( -10.00000000000012434, 5.773502691896184480, -164.8749999999999716 ) ) ;
#16289=CARTESIAN_POINT ( 'NONE',  ( -5.405949406249996869, 9.363379034771805109, -83.53125000204838102 ) ) ;
#16292=CARTESIAN_POINT ( 'NONE',  ( 5.000000000000000000, 8.660254037844385522, -62.12500000409676204 ) ) ;
#16293=CARTESIAN_POINT ( 'NONE',  ( -2.293366432827344421E-15, -12.48450537969573659, -21.21875000204837036 ) ) ;
#16296=CARTESIAN_POINT ( 'NONE',  ( -5.405949406249996869, 9.363379034771805109, -13.03125000204835615 ) ) ;
#16298=CARTESIAN_POINT ( 'NONE',  ( -9.999999999999479527, -5.773502691896549521, -148.5000000040967336 ) ) ;
#16305=ORIENTED_EDGE ( 'NONE', *, *, #13997, .F. ) ;
#16307=CARTESIAN_POINT ( 'NONE',  ( 5.405949406249992428, -9.363379034771808662, -100.5937500020483810 ) ) ;
#16314=CARTESIAN_POINT ( 'NONE',  ( -5.000000000000003553, -8.660254037844383745, -115.3750000040967905 ) ) ;
#16317=CARTESIAN_POINT ( 'NONE',  ( -9.999999999999998224, 0.000000000000000000, -99.99999999999998579 ) ) ;
#16318=CARTESIAN_POINT ( 'NONE',  ( -5.405949406249996869, 9.363379034771805109, -158.5312500020484094 ) ) ;
#16324=CARTESIAN_POINT ( 'NONE',  ( -10.81189881249999729, 1.324075727343319199E-15, -75.59375000204838102 ) ) ;
#16325=CARTESIAN_POINT ( 'NONE',  ( -5.405949406250003975, -9.363379034771801557, -84.53125000204838102 ) ) ;
#16328=CARTESIAN_POINT ( 'NONE',  ( -5.405949406250003975, -9.363379034771801557, -170.0312500020484094 ) ) ;
#16329=CARTESIAN_POINT ( 'NONE',  ( -5.405949406249996869, 9.363379034771805109, -176.5312500020483810 ) ) ;
#16330=CARTESIAN_POINT ( 'NONE',  ( -4.999999999999996447, 8.660254037844387298, -153.3750000040967905 ) ) ;
#16332=CARTESIAN_POINT ( 'NONE',  ( 10.81189881249999551, -6.242252689847874514, -5.968750002048355263 ) ) ;
#16334=CARTESIAN_POINT ( 'NONE',  ( -10.81189881249999907, -6.242252689847864744, -115.9687500020483810 ) ) ;
#16335=EDGE_CURVE ( 'NONE', #7903, #24042, #330, .T. ) ;
#16337=CARTESIAN_POINT ( 'NONE',  ( 5.405949406249999534, 9.363379034771803333, -13.28125000204835615 ) ) ;
#16340=CARTESIAN_POINT ( 'NONE',  ( -10.81189881249999729, 1.324075727343319199E-15, -111.7812500020483810 ) ) ;
#16342=ORIENTED_EDGE ( 'NONE', *, *, #31063, .T. ) ;
#16343=CARTESIAN_POINT ( 'NONE',  ( 7.070501591499377789E-16, 11.54700538379251284, -87.50000000409677625 ) ) ;
#16344=CARTESIAN_POINT ( 'NONE',  ( -5.405949406249996869, 9.363379034771805109, -41.34375000204837391 ) ) ;
#16348=CARTESIAN_POINT ( 'NONE',  ( -10.00000000000000000, -5.773502691896251982, -15.00000000409676559 ) ) ;
#16351=ORIENTED_EDGE ( 'NONE', *, *, #36721, .F. ) ;
#16352=VECTOR ( 'NONE', #9865, 1000.000000000000000 ) ;
#16361=( BOUNDED_CURVE ( )  B_SPLINE_CURVE ( 2, ( #28705, #15296, #37759, #14862, #2162, #5174, #5391 ),
 .UNSPECIFIED., .F., .F. ) 
 B_SPLINE_CURVE_WITH_KNOTS ( ( 3, 2, 2, 3 ),
 ( 0.3097014925373136052, 0.3109452736318408794, 0.3121890547263682092, 0.3134328358208955390 ),
 .UNSPECIFIED. ) 
 CURVE ( )  GEOMETRIC_REPRESENTATION_ITEM ( )  RATIONAL_B_SPLINE_CURVE ( ( 0.9999999999999820144, 0.8660254037844566932, 1.000000000000000000, 0.8660254037844387076, 1.000000000000000000, 0.8660254037844387076, 1.000000000000000000 ) ) 
 REPRESENTATION_ITEM ( '' )  );
#16364=CARTESIAN_POINT ( 'NONE',  ( 5.405949406249992428, -9.363379034771808662, -178.7812500020484094 ) ) ;
#16366=DIRECTION ( 'NONE',  ( 0.000000000000000000, 0.000000000000000000, 1.000000000000000000 ) ) ;
#16368=CARTESIAN_POINT ( 'NONE',  ( -2.293366432827344421E-15, -12.48450537969573659, -105.2187500020483952 ) ) ;
#16370=CARTESIAN_POINT ( 'NONE',  ( -5.405949406249996869, 9.363379034771805109, -109.0312500020483810 ) ) ;
#16372=CARTESIAN_POINT ( 'NONE',  ( 10.81189881249999551, -6.242252689847874514, -112.4687500020483810 ) ) ;
#16376=CARTESIAN_POINT ( 'NONE',  ( 10.00000000000000000, 5.773502691896255534, -139.8750000000000000 ) ) ;
#16377=CARTESIAN_POINT ( 'NONE',  ( 9.999999999999998224, 0.000000000000000000, -7.999999999999952038 ) ) ;
#16380=CARTESIAN_POINT ( 'NONE',  ( 9.999999999999998224, 0.000000000000000000, -179.3750000040967905 ) ) ;
#16383=CARTESIAN_POINT ( 'NONE',  ( 10.81189881249999729, 0.000000000000000000, -31.34375000204836681 ) ) ;
#16384=CARTESIAN_POINT ( 'NONE',  ( 9.999999999999998224, 0.000000000000000000, -141.8750000040967905 ) ) ;
#16385=CARTESIAN_POINT ( 'NONE',  ( -5.405949406250003975, -9.363379034771801557, -139.8437500020484094 ) ) ;
#16388=CARTESIAN_POINT ( 'NONE',  ( -10.81189881249999729, 6.242252689847871849, -35.40625000204835970 ) ) ;
#16389=FACE_OUTER_BOUND ( 'NONE', #15098, .T. ) ;
#16391=CARTESIAN_POINT ( 'NONE',  ( -2.121150477449813534E-15, -11.54700538379251284, -65.37499999999998579 ) ) ;
#16392=CARTESIAN_POINT ( 'NONE',  ( -2.293366432827344421E-15, -12.48450537969573659, -135.4062500020483810 ) ) ;
#16396=CARTESIAN_POINT ( 'NONE',  ( -10.00000000000000000, -5.773502691896251982, -111.0000000040967763 ) ) ;
#16397=CARTESIAN_POINT ( 'NONE',  ( 4.999999999999992006, -8.660254037844389075, -107.2499999999999858 ) ) ;
#16398=CARTESIAN_POINT ( 'NONE',  ( 7.644554776091147741E-16, 12.48450537969573659, -69.96875000204838102 ) ) ;
#16404=CARTESIAN_POINT ( 'NONE',  ( 9.999999999999998224, 0.000000000000000000, -32.37500000409676204 ) ) ;
#16409=CARTESIAN_POINT ( 'NONE',  ( 9.999999999999479527, 5.773502691896553074, -122.2500000040967763 ) ) ;
#16412=EDGE_LOOP ( 'NONE', ( #38947, #9891, #378, #22159 ) ) ;
#16413=ADVANCED_FACE ( 'NONE', ( #18124 ), #31319, .F. ) ;
#16422=CARTESIAN_POINT ( 'NONE',  ( 9.999999999999998224, 0.000000000000000000, -115.9999999999999858 ) ) ;
#16423=CARTESIAN_POINT ( 'NONE',  ( -10.81189881249999729, 6.242252689847871849, -123.7187500020483952 ) ) ;
#16424=CARTESIAN_POINT ( 'NONE',  ( 10.81189881249999907, 6.242252689847868297, -131.9062500020484094 ) ) ;
#16426=CARTESIAN_POINT ( 'NONE',  ( 7.644554776091147741E-16, 12.48450537969573659, -138.9687500020483810 ) ) ;
#16427=CARTESIAN_POINT ( 'NONE',  ( 9.999999999999998224, 0.000000000000000000, -129.5000000000000000 ) ) ;
#16428=CARTESIAN_POINT ( 'NONE',  ( -5.000000000000003553, -8.660254037844383745, -103.0000000000000000 ) ) ;
#16429=CARTESIAN_POINT ( 'NONE',  ( -9.999999999999998224, 1.224646799147353059E-15, -161.7500000000000000 ) ) ;
#16430=CARTESIAN_POINT ( 'NONE',  ( 10.81189881249999907, 6.242252689847868297, -1.406250002048359260 ) ) ;
#16433=CARTESIAN_POINT ( 'NONE',  ( -10.81189881249999729, 6.242252689847871849, -57.71875000204837391 ) ) ;
#16435=CARTESIAN_POINT ( 'NONE',  ( 10.81189881249999729, 0.000000000000000000, -160.3437500020484094 ) ) ;
#16441=CARTESIAN_POINT ( 'NONE',  ( -2.121150477449813534E-15, -11.54700538379251284, -93.87499999999997158 ) ) ;
#16444=CARTESIAN_POINT ( 'NONE',  ( 10.81189881249999729, 0.000000000000000000, -111.0312500020483810 ) ) ;
#16445=CARTESIAN_POINT ( 'NONE',  ( 9.999999999999996447, -5.773502691896262640, -131.5000000040967905 ) ) ;
#16447=EDGE_CURVE ( 'NONE', #19819, #22601, #15726, .T. ) ;
#16450=CIRCLE ( 'NONE', #39881, 24.99999999999999645 ) ;
#16452=CARTESIAN_POINT ( 'NONE',  ( 10.81189881249999907, 6.242252689847868297, -61.40625000204838102 ) ) ;
#16458=LINE ( 'NONE', #19923, #30323 ) ;
#16461=ADVANCED_FACE ( 'NONE', ( #39044 ), #29134, .T. ) ;
#16473=CARTESIAN_POINT ( 'NONE',  ( -4.999999999999996447, 8.660254037844387298, -29.99999999999997158 ) ) ;
#16476=CARTESIAN_POINT ( 'NONE',  ( 10.81189881249999729, 0.000000000000000000, -148.3437500020483810 ) ) ;
#16477=CARTESIAN_POINT ( 'NONE',  ( -2.293366432827344421E-15, -12.48450537969573659, -165.2187500020483810 ) ) ;
#16478=CARTESIAN_POINT ( 'NONE',  ( 7.070501591499376803E-16, 11.54700538379251284, -123.5000000040967905 ) ) ;
#16480=CARTESIAN_POINT ( 'NONE',  ( -2.121150477449813534E-15, -11.54700538379251284, -188.3750000000000284 ) ) ;
#16485=DIRECTION ( 'NONE',  ( -0.000000000000000000, -0.000000000000000000, -1.000000000000000000 ) ) ;
#16486=CARTESIAN_POINT ( 'NONE',  ( 7.644554776091147741E-16, 12.48450537969573659, -189.9687500020484094 ) ) ;
#16488=CARTESIAN_POINT ( 'NONE',  ( 10.81189881249999729, 0.000000000000000000, -64.53125000204836681 ) ) ;
#16490=CARTESIAN_POINT ( 'NONE',  ( 9.999999999999996447, -5.773502691896262640, -114.6249999999999858 ) ) ;
#16492=AXIS2_PLACEMENT_3D ( 'NONE', #37859, #39859, #399 ) ;
#16493=CARTESIAN_POINT ( 'NONE',  ( 7.644554776091147741E-16, 12.48450537969573659, -145.1562500020484094 ) ) ;
#16494=CARTESIAN_POINT ( 'NONE',  ( 10.81189881249999907, 6.242252689847868297, -152.9062500020483810 ) ) ;
#16496=DIRECTION ( 'NONE',  ( -0.000000000000000000, -0.000000000000000000, -1.000000000000000000 ) ) ;
#16497=CARTESIAN_POINT ( 'NONE',  ( 5.405949406249992428, -9.363379034771808662, -93.09375000204838102 ) ) ;
#16500=CARTESIAN_POINT ( 'NONE',  ( -10.81189881249999729, 6.242252689847871849, -186.7187500020483810 ) ) ;
#16505=CARTESIAN_POINT ( 'NONE',  ( -10.81189881249999907, -6.242252689847864744, -87.65625000204836681 ) ) ;
#16507=CARTESIAN_POINT ( 'NONE',  ( -9.999999999999998224, 5.773502691896259087, -58.75000000409677625 ) ) ;
#16508=CARTESIAN_POINT ( 'NONE',  ( -5.405949406250003975, -9.363379034771801557, -18.34375000204835260 ) ) ;
#16511=EDGE_CURVE ( 'NONE', #41044, #12598, #4727, .T. ) ;
#16512=CARTESIAN_POINT ( 'NONE',  ( -10.81189881249999729, 1.324075727343319199E-15, -14.28125000204835615 ) ) ;
#16518=CARTESIAN_POINT ( 'NONE',  ( 9.999999999999998224, 0.000000000000000000, -159.5000000000000000 ) ) ;
#16524=ORIENTED_EDGE ( 'NONE', *, *, #12285, .F. ) ;
#16535=CARTESIAN_POINT ( 'NONE',  ( -10.81189881249999729, 1.324075727343319199E-15, -146.2812500020483810 ) ) ;
#16537=CARTESIAN_POINT ( 'NONE',  ( 7.070501591499376803E-16, 11.54700538379251284, -121.6249999999999858 ) ) ;
#16541=CARTESIAN_POINT ( 'NONE',  ( 10.81189881249999907, 6.242252689847868297, -77.71875000204838102 ) ) ;
#16542=CARTESIAN_POINT ( 'NONE',  ( 10.81189881249999729, 0.000000000000000000, -84.03125000204838102 ) ) ;
#16546=CARTESIAN_POINT ( 'NONE',  ( -10.81189881249999729, 6.242252689847871849, -162.9062500020483810 ) ) ;
#16547=CARTESIAN_POINT ( 'NONE',  ( -10.81189881249999729, 6.242252689847871849, -182.4062500020483810 ) ) ;
#16549=CARTESIAN_POINT ( 'NONE',  ( 4.999999999999992006, -8.660254037844389075, -154.1250000040967905 ) ) ;
#16551=CARTESIAN_POINT ( 'NONE',  ( 5.405949406249992428, -9.363379034771808662, -4.593750002048368586 ) ) ;
#16553=CARTESIAN_POINT ( 'NONE',  ( 5.405949406249992428, -9.363379034771808662, -114.0937500020483810 ) ) ;
#16555=CARTESIAN_POINT ( 'NONE',  ( -10.81189881249999907, -6.242252689847864744, -12.65625000204837036 ) ) ;
#16557=CARTESIAN_POINT ( 'NONE',  ( -9.999999999999998224, 0.000000000000000000, -99.99999999999998579 ) ) ;
#16558=CARTESIAN_POINT ( 'NONE',  ( 10.81189881249999551, -6.242252689847874514, -111.1562500020483952 ) ) ;
#16560=ORIENTED_EDGE ( 'NONE', *, *, #22628, .T. ) ;
#16562=CARTESIAN_POINT ( 'NONE',  ( -2.121150477449813534E-15, -11.54700538379251284, -83.75000000409677625 ) ) ;
#16563=CARTESIAN_POINT ( 'NONE',  ( 10.00000000000051159, -5.773502691895965988, -140.5000000040967620 ) ) ;
#16564=CARTESIAN_POINT ( 'NONE',  ( 10.81189881249999729, 0.000000000000000000, -40.34375000204837391 ) ) ;
#16565=ORIENTED_EDGE ( 'NONE', *, *, #17901, .F. ) ;
#16569=CARTESIAN_POINT ( 'NONE',  ( 7.070501591499377789E-16, 11.54700538379251284, -15.50000000409676382 ) ) ;
#16575=EDGE_LOOP ( 'NONE', ( #25482, #41835, #24745, #16305 ) ) ;
#16582=CARTESIAN_POINT ( 'NONE',  ( 9.999999999999998224, 0.000000000000000000, -128.3750000040967905 ) ) ;
#16583=CARTESIAN_POINT ( 'NONE',  ( 10.81189881249999729, 0.000000000000000000, -178.5312500020483810 ) ) ;
#16586=CARTESIAN_POINT ( 'NONE',  ( -5.405949406249996869, 9.363379034771805109, -104.3437500020483810 ) ) ;
#16588=CARTESIAN_POINT ( 'NONE',  ( 7.644554776091147741E-16, 12.48450537969573659, -112.1562500020483810 ) ) ;
#16590=CARTESIAN_POINT ( 'NONE',  ( -5.405949406249996869, 9.363379034771805109, -114.8437500020483810 ) ) ;
#16594=CARTESIAN_POINT ( 'NONE',  ( 5.000000000000000000, 8.660254037844385522, -135.2499999999999716 ) ) ;
#16595=CARTESIAN_POINT ( 'NONE',  ( -4.999999999999996447, 8.660254037844387298, -1.499999999999973577 ) ) ;
#16598=CARTESIAN_POINT ( 'NONE',  ( 5.000000000000000000, 8.660254037844385522, -182.1250000040967905 ) ) ;
#16600=CARTESIAN_POINT ( 'NONE',  ( -10.81189881249999729, 1.324075727343319199E-15, -32.09375000204836681 ) ) ;
#16602=CARTESIAN_POINT ( 'NONE',  ( 7.644554776091147741E-16, 12.48450537969573659, -137.4687500020483810 ) ) ;
#16604=CARTESIAN_POINT ( 'NONE',  ( 10.81189881249999907, 6.242252689847868297, -35.90625000204835970 ) ) ;
#16606=CARTESIAN_POINT ( 'NONE',  ( 9.999999999999996447, -5.773502691896262640, -66.62499999999998579 ) ) ;
#16607=CARTESIAN_POINT ( 'NONE',  ( -2.293366432827344421E-15, -12.48450537969573659, -129.4062500020483810 ) ) ;
#16612=CARTESIAN_POINT ( 'NONE',  ( 10.00000000000000000, 5.773502691896255534, -111.7500000040967763 ) ) ;
#16613=CARTESIAN_POINT ( 'NONE',  ( -10.81189881249999729, 1.324075727343319199E-15, -69.59375000204836681 ) ) ;
#16614=ORIENTED_EDGE ( 'NONE', *, *, #5437, .F. ) ;
#16620=CARTESIAN_POINT ( 'NONE',  ( 9.999999999999996447, -5.773502691896262640, -38.50000000409676204 ) ) ;
#16630=ADVANCED_FACE ( 'NONE', ( #29317 ), #36424, .F. ) ;
#16635=CARTESIAN_POINT ( 'NONE',  ( 5.000000000000000000, 8.660254037844385522, -144.6250000040967905 ) ) ;
#16639=CARTESIAN_POINT ( 'NONE',  ( -10.81189881249999907, -6.242252689847864744, -123.4687500020483810 ) ) ;
#16640=CARTESIAN_POINT ( 'NONE',  ( -5.405949406249996869, 9.363379034771805109, -134.5312500020484094 ) ) ;
#16642=CARTESIAN_POINT ( 'NONE',  ( 10.81189881249999729, 6.242252689847867408, -140.7187500020483810 ) ) ;
#16645=CARTESIAN_POINT ( 'NONE',  ( -5.000000000000003553, -8.660254037844383745, -161.5000000000000000 ) ) ;
#16650=CARTESIAN_POINT ( 'NONE',  ( 10.81189881249999729, 0.000000000000000000, -52.34375000204835260 ) ) ;
#16652=CARTESIAN_POINT ( 'NONE',  ( -2.293366432827344421E-15, -12.48450537969573659, -162.2187500020483810 ) ) ;
#16657=CARTESIAN_POINT ( 'NONE',  ( 4.999999999999992006, -8.660254037844389075, -90.74999999999998579 ) ) ;
#16658=ORIENTED_EDGE ( 'NONE', *, *, #39473, .T. ) ;
#16659=CARTESIAN_POINT ( 'NONE',  ( -2.293366432827344421E-15, -12.48450537969573659, -114.4062500020483952 ) ) ;
#16660=CARTESIAN_POINT ( 'NONE',  ( 4.999999999999992006, -8.660254037844389075, -130.1250000040967620 ) ) ;
#16665=CARTESIAN_POINT ( 'NONE',  ( -10.81189881249999907, -6.242252689847864744, -51.65625000204837391 ) ) ;
#16679=ADVANCED_FACE ( 'NONE', ( #26083 ), #39650, .F. ) ;
#16683=EDGE_CURVE ( 'NONE', #18938, #40615, #33204, .T. ) ;
#16692=CARTESIAN_POINT ( 'NONE',  ( -10.81189881249999729, 1.324075727343319199E-15, -153.5937500020483810 ) ) ;
#16693=CARTESIAN_POINT ( 'NONE',  ( 10.81189881249999729, 6.242252689847867408, -164.7187500020483810 ) ) ;
#16696=CARTESIAN_POINT ( 'NONE',  ( -10.00000000000000000, -5.773502691896251982, -184.1250000000000284 ) ) ;
#16700=CARTESIAN_POINT ( 'NONE',  ( 0.000000000000000000, 0.000000000000000000, -99.99999999999998579 ) ) ;
#16701=CARTESIAN_POINT ( 'NONE',  ( -5.405949406249996869, 9.363379034771805109, -186.8437500020483810 ) ) ;
#16704=CARTESIAN_POINT ( 'NONE',  ( 5.405949406249999534, 9.363379034771803333, -50.78125000204835970 ) ) ;
#16706=CARTESIAN_POINT ( 'NONE',  ( 9.999999999999996447, -5.773502691896262640, -113.1250000000000000 ) ) ;
#16708=CARTESIAN_POINT ( 'NONE',  ( 7.644554776091147741E-16, 12.48450537969573659, -131.6562500020483810 ) ) ;
#16709=CARTESIAN_POINT ( 'NONE',  ( 10.81189881249999907, 6.242252689847868297, -151.4062500020484094 ) ) ;
#16710=ADVANCED_FACE ( 'NONE', ( #3205 ), #9672, .F. ) ;
#16711=VECTOR ( 'NONE', #39246, 1000.000000000000000 ) ;
#16714=CARTESIAN_POINT ( 'NONE',  ( 10.81189881249999729, 0.000000000000000000, -85.34375000204836681 ) ) ;
#16715=ORIENTED_EDGE ( 'NONE', *, *, #18180, .F. ) ;
#16717=CARTESIAN_POINT ( 'NONE',  ( -5.405949406249996869, 9.363379034771805109, -183.8437500020483810 ) ) ;
#16720=DIRECTION ( 'NONE',  ( -1.000000000000000000, 0.000000000000000000, 0.000000000000000000 ) ) ;
#16721=CARTESIAN_POINT ( 'NONE',  ( 5.405949406249999534, 9.363379034771803333, -76.28125000204838102 ) ) ;
#16723=CARTESIAN_POINT ( 'NONE',  ( 9.999999999999996447, -5.773502691896262640, -58.00000000409677625 ) ) ;
#16724=CARTESIAN_POINT ( 'NONE',  ( 5.405949406249992428, -9.363379034771808662, -9.093750002048345493 ) ) ;
#16725=CARTESIAN_POINT ( 'NONE',  ( 9.999999999999994671, -5.773502691896262640, -137.5000000040967905 ) ) ;
#16727=CARTESIAN_POINT ( 'NONE',  ( -10.81189881249999907, -6.242252689847864744, -14.15625000204837036 ) ) ;
#16747=CARTESIAN_POINT ( 'NONE',  ( -5.405949406250003975, -9.363379034771801557, -152.0312500020484094 ) ) ;
#16750=EDGE_CURVE ( 'NONE', #5023, #33176, #16762, .T. ) ;
#16752=DIRECTION ( 'NONE',  ( -1.000000000000000000, 0.000000000000000000, 0.000000000000000000 ) ) ;
#16756=CARTESIAN_POINT ( 'NONE',  ( 10.81189881249999907, 6.242252689847868297, -68.71875000204838102 ) ) ;
#16757=CARTESIAN_POINT ( 'NONE',  ( 10.81189881249999907, 6.242252689847868297, -74.90625000204839523 ) ) ;
#16760=CARTESIAN_POINT ( 'NONE',  ( 10.81189881249999729, 0.000000000000000000, -162.0312500020484094 ) ) ;
#16761=CARTESIAN_POINT ( 'NONE',  ( 10.81189881249999729, 0.000000000000000000, -169.5312500020484094 ) ) ;
#16762=LINE ( 'NONE', #9881, #18733 ) ;
#16763=CARTESIAN_POINT ( 'NONE',  ( -10.81189881249999729, 1.324075727343319199E-15, -2.093750002048366810 ) ) ;
#16765=CARTESIAN_POINT ( 'NONE',  ( 5.405949406249999534, 9.363379034771803333, -104.5937500020483810 ) ) ;
#16767=CARTESIAN_POINT ( 'NONE',  ( 10.81189881249999551, -6.242252689847874514, -9.156250002048365033 ) ) ;
#16769=CARTESIAN_POINT ( 'NONE',  ( -2.121150477449813534E-15, -11.54700538379251284, -133.2500000040967905 ) ) ;
#16770=CARTESIAN_POINT ( 'NONE',  ( 7.644554776091147741E-16, 12.48450537969573659, -112.1562500020483810 ) ) ;
#16772=VERTEX_POINT ( 'NONE', #23483 ) ;
#16773=CARTESIAN_POINT ( 'NONE',  ( 10.00000000000000000, 5.773502691896255534, -86.25000000409677625 ) ) ;
#16775=CARTESIAN_POINT ( 'NONE',  ( 10.81189881249999551, -6.242252689847874514, -41.96875000204836681 ) ) ;
#16776=VERTEX_POINT ( 'NONE', #12889 ) ;
#16780=CARTESIAN_POINT ( 'NONE',  ( 7.070501591499377789E-16, 11.54700538379251284, -14.00000000409676382 ) ) ;
#16782=FACE_OUTER_BOUND ( 'NONE', #28647, .T. ) ;
#16794=CARTESIAN_POINT ( 'NONE',  ( -10.00000000000076916, 5.773502691895813221, -127.7500000040967763 ) ) ;
#16795=( BOUNDED_CURVE ( )  B_SPLINE_CURVE ( 2, ( #12425, #26455, #6189, #39606, #19130, #23222, #9626 ),
 .UNSPECIFIED., .F., .F. ) 
 B_SPLINE_CURVE_WITH_KNOTS ( ( 3, 2, 2, 3 ),
 ( 0.2910447761194031036, 0.2922885572139304333, 0.2935323383084578186, 0.2947761194029852039 ),
 .UNSPECIFIED. ) 
 CURVE ( )  GEOMETRIC_REPRESENTATION_ITEM ( )  RATIONAL_B_SPLINE_CURVE ( ( 0.9999999999999880096, 0.8660254037844506980, 1.000000000000000000, 0.8660254037844387076, 1.000000000000000000, 0.8660254037844267172, 1.000000000000011990 ) ) 
 REPRESENTATION_ITEM ( '' )  );
#16796=CARTESIAN_POINT ( 'NONE',  ( 10.81189881249999729, 0.000000000000000000, -172.5312500020484094 ) ) ;
#16797=CARTESIAN_POINT ( 'NONE',  ( 7.070501591499376803E-16, 11.54700538379251284, -155.0000000040968189 ) ) ;
#16799=CARTESIAN_POINT ( 'NONE',  ( 5.405949406249999534, 9.363379034771803333, -97.09375000204838102 ) ) ;
#16800=CARTESIAN_POINT ( 'NONE',  ( -9.999999999999998224, 1.224646799147353059E-15, -106.2499999999999858 ) ) ;
#16801=CARTESIAN_POINT ( 'NONE',  ( -5.405949406249996869, 9.363379034771805109, -112.0312500020483810 ) ) ;
#16803=CARTESIAN_POINT ( 'NONE',  ( 5.405949406249992428, -9.363379034771808662, -115.5937500020483810 ) ) ;
#16807=CARTESIAN_POINT ( 'NONE',  ( 10.00000000000051159, -5.773502691895965988, -114.6249999999999574 ) ) ;
#16808=CARTESIAN_POINT ( 'NONE',  ( -10.00000000000000000, -5.773502691896251982, -1.124999999999959366 ) ) ;
#16811=CARTESIAN_POINT ( 'NONE',  ( 7.070501591499377789E-16, 11.54700538379251284, -182.0000000040968189 ) ) ;
#16813=CARTESIAN_POINT ( 'NONE',  ( 5.405949406249992428, -9.363379034771808662, -31.59375000204836681 ) ) ;
#16815=CARTESIAN_POINT ( 'NONE',  ( -10.81189881249999729, 1.324075727343319199E-15, -138.5937500020483810 ) ) ;
#16817=CARTESIAN_POINT ( 'NONE',  ( -10.81189881249999907, -6.242252689847864744, -35.15625000204835970 ) ) ;
#16819=CARTESIAN_POINT ( 'NONE',  ( -2.121150477449813534E-15, -11.54700538379251284, -57.87499999999997868 ) ) ;
#16820=CARTESIAN_POINT ( 'NONE',  ( -2.293366432827344421E-15, -12.48450537969573659, -133.9062500020483810 ) ) ;
#16825=CARTESIAN_POINT ( 'NONE',  ( -9.999999999999998224, 1.224646799147353059E-15, -106.6250000040967763 ) ) ;
#16826=CARTESIAN_POINT ( 'NONE',  ( -2.121150477449813534E-15, -11.54700538379251284, -107.3749999999999858 ) ) ;
#16827=CARTESIAN_POINT ( 'NONE',  ( -10.81189881249999729, 1.324075727343319199E-15, -68.09375000204836681 ) ) ;
#16832=CARTESIAN_POINT ( 'NONE',  ( -4.999999999999996447, 8.660254037844387298, -124.8750000040967763 ) ) ;
#16833=CARTESIAN_POINT ( 'NONE',  ( 10.00000000000000000, 5.773502691896255534, -32.25000000409675494 ) ) ;
#16840=ORIENTED_EDGE ( 'NONE', *, *, #11687, .T. ) ;
#16844=VECTOR ( 'NONE', #29755, 1000.000000000000000 ) ;
#16845=CARTESIAN_POINT ( 'NONE',  ( -10.81189881249999729, 6.242252689847871849, -192.9062500020484094 ) ) ;
#16847=CARTESIAN_POINT ( 'NONE',  ( 9.999999999999998224, 0.000000000000000000, -155.0000000000000000 ) ) ;
#16852=CARTESIAN_POINT ( 'NONE',  ( -10.81189881249999907, -6.242252689847864744, -129.4687500020483810 ) ) ;
#16853=CARTESIAN_POINT ( 'NONE',  ( 10.81189881249999729, 0.000000000000000000, -132.0312500020484094 ) ) ;
#16855=CARTESIAN_POINT ( 'NONE',  ( -5.405949406250003975, -9.363379034771801557, -139.8437500020484094 ) ) ;
#16856=CARTESIAN_POINT ( 'NONE',  ( -9.999999999999227285, -5.773502691896698735, -130.1249999999999716 ) ) ;
#16858=CARTESIAN_POINT ( 'NONE',  ( 7.070501591499377789E-16, 11.54700538379251284, -156.1250000000000000 ) ) ;
#16863=CARTESIAN_POINT ( 'NONE',  ( 5.405949406249999534, 9.363379034771803333, -55.09375000204835970 ) ) ;
#16865=CARTESIAN_POINT ( 'NONE',  ( -10.81189881249999907, -6.242252689847864744, -163.9687500020484094 ) ) ;
#16869=CARTESIAN_POINT ( 'NONE',  ( 4.999999999999992006, -8.660254037844389075, -81.74999999999998579 ) ) ;
#16871=CARTESIAN_POINT ( 'NONE',  ( 10.81189881249999551, -6.242252689847874514, -108.1562500020483810 ) ) ;
#16872=CARTESIAN_POINT ( 'NONE',  ( 10.00000000000000000, 5.773502691896255534, -129.7500000040967905 ) ) ;
#16873=CARTESIAN_POINT ( 'NONE',  ( -35.00000000000000711, 0.000000000000000000, -169.9999999999999716 ) ) ;
#16877=( BOUNDED_CURVE ( )  B_SPLINE_CURVE ( 2, ( #37194, #24484, #27072, #1388, #4403, #1175, #27712 ),
 .UNSPECIFIED., .F., .F. ) 
 B_SPLINE_CURVE_WITH_KNOTS ( ( 3, 2, 2, 3 ),
 ( 0.2947761194029852039, 0.2960199004975125336, 0.2972636815920398634, 0.2985074626865671932 ),
 .UNSPECIFIED. ) 
 CURVE ( )  GEOMETRIC_REPRESENTATION_ITEM ( )  RATIONAL_B_SPLINE_CURVE ( ( 0.9999999999999880096, 0.8660254037844506980, 1.000000000000000000, 0.8660254037844387076, 1.000000000000000000, 0.8660254037844327124, 1.000000000000005995 ) ) 
 REPRESENTATION_ITEM ( '' )  );
#16879=CARTESIAN_POINT ( 'NONE',  ( -10.81189881249999729, 1.324075727343319199E-15, -54.78125000204836681 ) ) ;
#16880=VECTOR ( 'NONE', #14915, 1000.000000000000000 ) ;
#16886=EDGE_LOOP ( 'NONE', ( #33178, #39310, #41583, #11536 ) ) ;
#16887=CARTESIAN_POINT ( 'NONE',  ( 9.999999999999998224, 0.000000000000000000, -131.3750000040967905 ) ) ;
#16902=CARTESIAN_POINT ( 'NONE',  ( -10.81189881249999907, -6.242252689847864744, -148.9687500020484094 ) ) ;
#16903=CARTESIAN_POINT ( 'NONE',  ( -10.81189881249999729, 6.242252689847871849, -165.7187500020483810 ) ) ;
#16904=LINE ( 'NONE', #23195, #36406 ) ;
#16906=CARTESIAN_POINT ( 'NONE',  ( -5.000000000000003553, -8.660254037844383745, -178.0000000000000000 ) ) ;
#16908=CARTESIAN_POINT ( 'NONE',  ( -10.00000000000051337, 5.773502691895962435, -151.3750000000000284 ) ) ;
#16911=CARTESIAN_POINT ( 'NONE',  ( -5.405949406250003975, -9.363379034771801557, -183.3437500020483810 ) ) ;
#16914=CARTESIAN_POINT ( 'NONE',  ( -5.405949406249996869, 9.363379034771805109, -52.03125000204835970 ) ) ;
#16916=CARTESIAN_POINT ( 'NONE',  ( 5.000000000000000000, 8.660254037844385522, -114.2499999999999858 ) ) ;
#16919=CARTESIAN_POINT ( 'NONE',  ( 10.81189881249999551, -6.242252689847874514, -132.1562500020483810 ) ) ;
#16920=CARTESIAN_POINT ( 'NONE',  ( -10.81189881249999729, 1.324075727343319199E-15, -144.7812500020483810 ) ) ;
#16922=LINE ( 'NONE', #30123, #38536 ) ;
#16923=CARTESIAN_POINT ( 'NONE',  ( -5.405949406249996869, 9.363379034771805109, -83.34375000204836681 ) ) ;
#16926=CARTESIAN_POINT ( 'NONE',  ( 7.644554776091147741E-16, 12.48450537969573659, -183.9687500020484094 ) ) ;
#16930=CARTESIAN_POINT ( 'NONE',  ( 4.999999999999992006, -8.660254037844389075, -158.2500000000000000 ) ) ;
#16932=CARTESIAN_POINT ( 'NONE',  ( 5.405949406249999534, 9.363379034771803333, -74.78125000204838102 ) ) ;
#16936=CARTESIAN_POINT ( 'NONE',  ( -4.999999999999996447, 8.660254037844387298, -54.37500000409675494 ) ) ;
#16937=CARTESIAN_POINT ( 'NONE',  ( -5.405949406250003975, -9.363379034771801557, -9.343750002048345493 ) ) ;
#16940=CARTESIAN_POINT ( 'NONE',  ( -2.293366432827344421E-15, -12.48450537969573659, -7.906250002048365921 ) ) ;
#16943=DIRECTION ( 'NONE',  ( -1.000000000000000000, 0.000000000000000000, 0.000000000000000000 ) ) ;
#16949=CARTESIAN_POINT ( 'NONE',  ( -5.405949406249996869, 9.363379034771805109, -102.8437500020483810 ) ) ;
#16951=VERTEX_POINT ( 'NONE', #17779 ) ;
#16958=CARTESIAN_POINT ( 'NONE',  ( 9.999999999999998224, 0.000000000000000000, -40.99999999999997868 ) ) ;
#16963=CARTESIAN_POINT ( 'NONE',  ( 4.999999999999992006, -8.660254037844389075, -121.1250000040967905 ) ) ;
#16965=CARTESIAN_POINT ( 'NONE',  ( -5.405949406249996869, 9.363379034771805109, -152.5312500020484094 ) ) ;
#16972=CARTESIAN_POINT ( 'NONE',  ( 10.81189881249999551, -6.242252689847874514, -71.96875000204836681 ) ) ;
#16973=CARTESIAN_POINT ( 'NONE',  ( 5.405949406249999534, 9.363379034771803333, -79.28125000204838102 ) ) ;
#16975=CARTESIAN_POINT ( 'NONE',  ( -2.293366432827344421E-15, -12.48450537969573659, -157.9062500020483810 ) ) ;
#16976=CARTESIAN_POINT ( 'NONE',  ( 7.644554776091147741E-16, 12.48450537969573659, -172.1562500020484094 ) ) ;
#16980=CARTESIAN_POINT ( 'NONE',  ( -10.81189881249999729, 1.324075727343319199E-15, -110.0937500020483810 ) ) ;
#16982=CARTESIAN_POINT ( 'NONE',  ( 5.405949406249999534, 9.363379034771803333, -7.281250002048378356 ) ) ;
#16985=CARTESIAN_POINT ( 'NONE',  ( -5.405949406250003975, -9.363379034771801557, -104.0312500020483810 ) ) ;
#16989=CARTESIAN_POINT ( 'NONE',  ( 10.00000000000000000, 5.773502691896255534, -74.25000000409677625 ) ) ;
#16991=CARTESIAN_POINT ( 'NONE',  ( -10.81189881249999729, 1.324075727343319199E-15, -33.59375000204836681 ) ) ;
#16994=EDGE_CURVE ( 'NONE', #24042, #30416, #12405, .T. ) ;
#16995=CARTESIAN_POINT ( 'NONE',  ( 5.405949406249992428, -9.363379034771808662, -36.28125000204837391 ) ) ;
#16997=CARTESIAN_POINT ( 'NONE',  ( 9.999999999999998224, 1.224646799147353059E-15, -99.99999999999998579 ) ) ;
#16998=CARTESIAN_POINT ( 'NONE',  ( 9.999999999999998224, 0.000000000000000000, -12.87500000409674783 ) ) ;
#17000=CYLINDRICAL_SURFACE ( 'NONE', #27546, 9.999999999999998224 ) ;
#17007=ADVANCED_FACE ( 'NONE', ( #4633 ), #1405, .F. ) ;
#17015=CARTESIAN_POINT ( 'NONE',  ( 5.405949406249992428, -9.363379034771808662, -171.2812500020484094 ) ) ;
#17018=CARTESIAN_POINT ( 'NONE',  ( 10.81189881249999729, 0.000000000000000000, -95.84375000204838102 ) ) ;
#17019=CARTESIAN_POINT ( 'NONE',  ( 5.405949406249999534, 9.363379034771803333, -100.2812500020483952 ) ) ;
#17021=CARTESIAN_POINT ( 'NONE',  ( 10.81189881249999729, 6.242252689847867408, -110.7187500020483810 ) ) ;
#17023=CARTESIAN_POINT ( 'NONE',  ( -9.999999999999479527, -5.773502691896549521, -105.0000000040967620 ) ) ;
#17024=CARTESIAN_POINT ( 'NONE',  ( -2.293366432827344421E-15, -12.48450537969573659, -178.9062500020484379 ) ) ;
#17025=CARTESIAN_POINT ( 'NONE',  ( -2.293366432827344421E-15, -12.48450537969573659, -193.9062500020484094 ) ) ;
#17028=CARTESIAN_POINT ( 'NONE',  ( -4.999999999999996447, 8.660254037844387298, -174.3750000040968189 ) ) ;
#17030=CARTESIAN_POINT ( 'NONE',  ( -5.405949406250003975, -9.363379034771801557, -21.34375000204835615 ) ) ;
#17032=CARTESIAN_POINT ( 'NONE',  ( 5.405949406249999534, 9.363379034771803333, -128.5937500020483810 ) ) ;
#17034=CARTESIAN_POINT ( 'NONE',  ( -10.81189881249999729, 1.324075727343319199E-15, -24.78125000204836681 ) ) ;
#17036=CARTESIAN_POINT ( 'NONE',  ( -5.000000000000003553, -8.660254037844383745, -56.49999999999996447 ) ) ;
#17037=CARTESIAN_POINT ( 'NONE',  ( 10.81189881249999551, -6.242252689847874514, -124.6562500020483952 ) ) ;
#17041=CARTESIAN_POINT ( 'NONE',  ( -2.121150477449813534E-15, -11.54700538379251284, -104.7500000040967763 ) ) ;
#17042=CARTESIAN_POINT ( 'NONE',  ( -9.999999999999998224, 1.224646799147353059E-15, -107.7499999999999858 ) ) ;
#17043=CARTESIAN_POINT ( 'NONE',  ( 5.405949406249999534, 9.363379034771803333, -61.09375000204836681 ) ) ;
#17047=LINE ( 'NONE', #7360, #41424 ) ;
#17048=CARTESIAN_POINT ( 'NONE',  ( -5.000000000000003553, -8.660254037844383745, -38.87500000409676915 ) ) ;
#17050=CARTESIAN_POINT ( 'NONE',  ( -9.999999999999998224, 1.224646799147353059E-15, -130.2499999999999716 ) ) ;
#17053=CARTESIAN_POINT ( 'NONE',  ( 9.999999999999742428, 5.773502691896404748, -129.7500000040967905 ) ) ;
#17055=( BOUNDED_CURVE ( )  B_SPLINE_CURVE ( 2, ( #22533, #38724, #25779, #6349, #19705, #35706, #22325 ),
 .UNSPECIFIED., .F., .F. ) 
 B_SPLINE_CURVE_WITH_KNOTS ( ( 3, 2, 2, 3 ),
 ( 0.1977611940298507898, 0.1990049751243781750, 0.2002487562189055326, 0.2014925373134328901 ),
 .UNSPECIFIED. ) 
 CURVE ( )  GEOMETRIC_REPRESENTATION_ITEM ( )  RATIONAL_B_SPLINE_CURVE ( ( 0.9999999999999940048, 0.8660254037844447028, 1.000000000000000000, 0.8660254037844387076, 1.000000000000000000, 0.8660254037844327124, 1.000000000000005995 ) ) 
 REPRESENTATION_ITEM ( '' )  );
#17061=CYLINDRICAL_SURFACE ( 'NONE', #26128, 9.999999999999998224 ) ;
#17067=DIRECTION ( 'NONE',  ( -0.000000000000000000, -0.000000000000000000, -1.000000000000000000 ) ) ;
#17068=CARTESIAN_POINT ( 'NONE',  ( 10.81189881249999729, 0.000000000000000000, -118.3437500020483810 ) ) ;
#17069=CARTESIAN_POINT ( 'NONE',  ( 9.999999999999996447, -5.773502691896262640, -193.0000000040968473 ) ) ;
#17070=CARTESIAN_POINT ( 'NONE',  ( -2.293366432827344421E-15, -12.48450537969573659, -126.4062500020483952 ) ) ;
#17072=CARTESIAN_POINT ( 'NONE',  ( -10.81189881249999729, 1.324075727343319199E-15, -137.0937500020483810 ) ) ;
#17075=CARTESIAN_POINT ( 'NONE',  ( 4.999999999999992006, -8.660254037844389075, -153.7500000000000000 ) ) ;
#17076=CARTESIAN_POINT ( 'NONE',  ( -9.999999999999998224, 5.773502691896259087, -19.37499999999997868 ) ) ;
#17080=CARTESIAN_POINT ( 'NONE',  ( -10.81189881249999729, 1.324075727343319199E-15, -56.09375000204835970 ) ) ;
#17081=CARTESIAN_POINT ( 'NONE',  ( 9.999999999999998224, 0.000000000000000000, -110.3750000040967763 ) ) ;
#17082=CARTESIAN_POINT ( 'NONE',  ( -5.405949406250003975, -9.363379034771801557, -151.8437500020483810 ) ) ;
#17085=CARTESIAN_POINT ( 'NONE',  ( -4.263623593850985216, 9.091409269767630974, -180.0000000000000000 ) ) ;
#17086=CARTESIAN_POINT ( 'NONE',  ( 9.999999999999998224, 0.000000000000000000, -84.49999999999997158 ) ) ;
#17089=CARTESIAN_POINT ( 'NONE',  ( 7.644554776091147741E-16, 12.48450537969573659, -110.6562500020483810 ) ) ;
#17090=CARTESIAN_POINT ( 'NONE',  ( 10.00000000000000000, 5.773502691896255534, -132.7500000040967905 ) ) ;
#17094=CARTESIAN_POINT ( 'NONE',  ( -2.293366432827344421E-15, -12.48450537969573659, -51.40625000204837391 ) ) ;
#17096=DIRECTION ( 'NONE',  ( -0.000000000000000000, -0.000000000000000000, -1.000000000000000000 ) ) ;
#17117=CARTESIAN_POINT ( 'NONE',  ( -5.405949406250003975, -9.363379034771801557, -139.8437500020484094 ) ) ;
#17118=CARTESIAN_POINT ( 'NONE',  ( -2.293366432827344421E-15, -12.48450537969573659, -159.2187500020483526 ) ) ;
#17121=CARTESIAN_POINT ( 'NONE',  ( 9.999999999999998224, 0.000000000000000000, -177.5000000000000000 ) ) ;
#17126=CARTESIAN_POINT ( 'NONE',  ( -5.405949406249996869, 9.363379034771805109, -188.3437500020483810 ) ) ;
#17131=CARTESIAN_POINT ( 'NONE',  ( -10.81189881249999729, 1.324075727343319199E-15, -53.28125000204836681 ) ) ;
#17133=CARTESIAN_POINT ( 'NONE',  ( 9.999999999999996447, -5.773502691896262640, -108.6249999999999858 ) ) ;
#17135=CARTESIAN_POINT ( 'NONE',  ( 7.644554776091147741E-16, 12.48450537969573659, -133.1562500020483810 ) ) ;
#17136=CARTESIAN_POINT ( 'NONE',  ( 7.644554776091147741E-16, 12.48450537969573659, -148.1562500020484094 ) ) ;
#17139=CARTESIAN_POINT ( 'NONE',  ( -5.405949406249996869, 9.363379034771805109, -78.84375000204838102 ) ) ;
#17140=VERTEX_POINT ( 'NONE', #38289 ) ;
#17142=CARTESIAN_POINT ( 'NONE',  ( -2.293366432827344421E-15, -12.48450537969573659, -178.7187500020484094 ) ) ;
#17144=CARTESIAN_POINT ( 'NONE',  ( -5.000000000000003553, -8.660254037844383745, -110.4999999999999858 ) ) ;
#17146=CARTESIAN_POINT ( 'NONE',  ( -5.405949406249996869, 9.363379034771805109, -73.03125000204838102 ) ) ;
#17148=CARTESIAN_POINT ( 'NONE',  ( 10.00000000000000000, 5.773502691896255534, -50.25000000409676204 ) ) ;
#17149=CARTESIAN_POINT ( 'NONE',  ( -2.293366432827344421E-15, -12.48450537969573659, -6.218750002048356151 ) ) ;
#17152=CARTESIAN_POINT ( 'NONE',  ( -5.405949406250003975, -9.363379034771801557, -5.031250002048376579 ) ) ;
#17154=CARTESIAN_POINT ( 'NONE',  ( 7.070501591499376803E-16, 11.54700538379251284, -176.0000000040967905 ) ) ;
#17155=DIRECTION ( 'NONE',  ( -1.000000000000000000, 0.000000000000000000, 0.000000000000000000 ) ) ;
#17156=CARTESIAN_POINT ( 'NONE',  ( 4.999999999999992006, -8.660254037844389075, -134.6250000040967620 ) ) ;
#17168=CARTESIAN_POINT ( 'NONE',  ( 4.999999999999992006, -8.660254037844389075, -122.2500000000000000 ) ) ;
#17170=CARTESIAN_POINT ( 'NONE',  ( -9.999999999999998224, 1.224646799147353059E-15, -46.24999999999998579 ) ) ;
#17175=CARTESIAN_POINT ( 'NONE',  ( -9.999999999999998224, 1.224646799147353059E-15, -121.6250000040967905 ) ) ;
#17179=CARTESIAN_POINT ( 'NONE',  ( -9.999999999999998224, 1.224646799147353059E-15, -126.1250000040967620 ) ) ;
#17184=CARTESIAN_POINT ( 'NONE',  ( 5.405949406249992428, -9.363379034771808662, -70.59375000204836681 ) ) ;
#17185=CARTESIAN_POINT ( 'NONE',  ( -10.81189881249999729, 1.324075727343319199E-15, -74.28125000204838102 ) ) ;
#17187=CARTESIAN_POINT ( 'NONE',  ( -10.81189881249999729, -6.242252689847864744, -155.1562500020484663 ) ) ;
#17188=CARTESIAN_POINT ( 'NONE',  ( 10.81189881249999907, 6.242252689847868297, -175.4062500020484094 ) ) ;
#17189=CYLINDRICAL_SURFACE ( 'NONE', #33032, 9.999999999999998224 ) ;
#17190=CARTESIAN_POINT ( 'NONE',  ( 7.070501591499376803E-16, 11.54700538379251284, -108.5000000040967763 ) ) ;
#17191=CARTESIAN_POINT ( 'NONE',  ( -10.81189881249999907, -6.242252689847864744, -103.9687500020483668 ) ) ;
#17192=CARTESIAN_POINT ( 'NONE',  ( 5.000000000000000000, 8.660254037844385522, -156.2500000000000000 ) ) ;
#17194=CARTESIAN_POINT ( 'NONE',  ( -10.81189881249999907, -6.242252689847864744, -5.156250002048362369 ) ) ;
#17196=CARTESIAN_POINT ( 'NONE',  ( 7.644554776091147741E-16, 12.48450537969573659, -101.6562500020483952 ) ) ;
#17198=CARTESIAN_POINT ( 'NONE',  ( -2.121150477449813534E-15, -11.54700538379251284, -77.75000000409677625 ) ) ;
#17200=CARTESIAN_POINT ( 'NONE',  ( -2.293366432827344421E-15, -12.48450537969573659, -34.71875000204835260 ) ) ;
#17201=ORIENTED_EDGE ( 'NONE', *, *, #18251, .F. ) ;
#17203=CARTESIAN_POINT ( 'NONE',  ( -2.293366432827344421E-15, -12.48450537969573659, -25.90625000204838102 ) ) ;
#17206=CARTESIAN_POINT ( 'NONE',  ( 9.999999999999998224, 0.000000000000000000, -3.875000004096768258 ) ) ;
#17213=VERTEX_POINT ( 'NONE', #10507 ) ;
#17219=EDGE_CURVE ( 'NONE', #24467, #36911, #8311, .T. ) ;
#17220=ORIENTED_EDGE ( 'NONE', *, *, #1751, .T. ) ;
#17224=CARTESIAN_POINT ( 'NONE',  ( -10.81189881249999729, 6.242252689847871849, -171.9062500020484094 ) ) ;
#17226=AXIS2_PLACEMENT_3D ( 'NONE', #2695, #29025, #9164 ) ;
#17227=EDGE_CURVE ( 'NONE', #40108, #41753, #2241, .T. ) ;
#17230=CARTESIAN_POINT ( 'NONE',  ( -10.81189881249999729, 1.324075727343319199E-15, -96.59375000204838102 ) ) ;
#17231=CARTESIAN_POINT ( 'NONE',  ( 5.000000000000000000, 8.660254037844385522, -154.7500000000000000 ) ) ;
#17232=CARTESIAN_POINT ( 'NONE',  ( -5.405949406250003975, -9.363379034771801557, -101.0312500020483952 ) ) ;
#17234=CARTESIAN_POINT ( 'NONE',  ( -5.405949406250003975, -9.363379034771801557, -103.8437500020483810 ) ) ;
#17236=CARTESIAN_POINT ( 'NONE',  ( 4.999999999999992006, -8.660254037844389075, -104.6250000040967763 ) ) ;
#17238=CARTESIAN_POINT ( 'NONE',  ( -10.81189881249999729, 1.324075727343319199E-15, -192.7812500020484094 ) ) ;
#17241=CARTESIAN_POINT ( 'NONE',  ( -9.999999999999998224, 1.224646799147353059E-15, -169.6250000040967905 ) ) ;
#17243=CARTESIAN_POINT ( 'NONE',  ( -10.81189881249999907, -6.242252689847864744, -22.96875000204837036 ) ) ;
#17245=CARTESIAN_POINT ( 'NONE',  ( -10.81189881249999729, 6.242252689847871849, -129.7187500020483810 ) ) ;
#17247=CARTESIAN_POINT ( 'NONE',  ( 5.405949406249999534, 9.363379034771803333, -28.28125000204837036 ) ) ;
#17249=CARTESIAN_POINT ( 'NONE',  ( -2.121150477449813534E-15, -11.54700538379251284, -56.37499999999997868 ) ) ;
#17250=CARTESIAN_POINT ( 'NONE',  ( -5.405949406250003975, -9.363379034771801557, -122.0312500020483952 ) ) ;
#17253=CARTESIAN_POINT ( 'NONE',  ( -9.999999999999998224, 1.224646799147353059E-15, -128.7499999999999716 ) ) ;
#17254=CARTESIAN_POINT ( 'NONE',  ( 10.00000000000000000, 5.773502691896255534, -101.2500000040967905 ) ) ;
#17256=CARTESIAN_POINT ( 'NONE',  ( -2.293366432827344421E-15, -12.48450537969573659, -54.21875000204837391 ) ) ;
#17257=VERTEX_POINT ( 'NONE', #29012 ) ;
#17261=CARTESIAN_POINT ( 'NONE',  ( 4.999999999999992006, -8.660254037844389075, -28.12500000409676204 ) ) ;
#17267=VERTEX_POINT ( 'NONE', #6132 ) ;
#17272=CARTESIAN_POINT ( 'NONE',  ( -10.81189881249999907, -6.242252689847864744, -195.6562500020484094 ) ) ;
#17278=CARTESIAN_POINT ( 'NONE',  ( -2.293366432827344421E-15, -12.48450537969573659, -118.7187500020483952 ) ) ;
#17279=CARTESIAN_POINT ( 'NONE',  ( -9.999999999999998224, 1.224646799147353059E-15, -198.1250000040967905 ) ) ;
#17280=CARTESIAN_POINT ( 'NONE',  ( -5.405949406249996869, 9.363379034771805109, -125.5312500020483952 ) ) ;
#17282=CARTESIAN_POINT ( 'NONE',  ( -5.405949406249996869, 9.363379034771805109, -131.3437500020484094 ) ) ;
#17283=AXIS2_PLACEMENT_3D ( 'NONE', #10575, #36915, #3913 ) ;
#17284=CARTESIAN_POINT ( 'NONE',  ( -9.999999999999998224, 1.224646799147353059E-15, -162.1250000040967905 ) ) ;
#17286=CARTESIAN_POINT ( 'NONE',  ( -2.121150477449813534E-15, -11.54700538379251284, -156.8750000000000000 ) ) ;
#17287=CARTESIAN_POINT ( 'NONE',  ( -10.00000000000000000, -5.773502691896251982, -20.62499999999997868 ) ) ;
#17294=CARTESIAN_POINT ( 'NONE',  ( 5.405949406249999534, 9.363379034771803333, -47.59375000204838102 ) ) ;
#17295=CARTESIAN_POINT ( 'NONE',  ( -5.405949406249996869, 9.363379034771805109, -156.8437500020483810 ) ) ;
#17299=CARTESIAN_POINT ( 'NONE',  ( 7.070501591499377789E-16, 11.54700538379251284, -87.12499999999997158 ) ) ;
#17301=( BOUNDED_CURVE ( )  B_SPLINE_CURVE ( 2, ( #14764, #5081, #40665, #21687, #11105, #38092, #1209 ),
 .UNSPECIFIED., .F., .F. ) 
 B_SPLINE_CURVE_WITH_KNOTS ( ( 3, 2, 2, 3 ),
 ( 0.2537313432835822113, 0.2549751243781095411, 0.2562189054726369264, 0.2574626865671643117 ),
 .UNSPECIFIED. ) 
 CURVE ( )  GEOMETRIC_REPRESENTATION_ITEM ( )  RATIONAL_B_SPLINE_CURVE ( ( 0.9999999999999880096, 0.8660254037844506980, 1.000000000000000000, 0.8660254037844387076, 1.000000000000000000, 0.8660254037844267172, 1.000000000000011990 ) ) 
 REPRESENTATION_ITEM ( '' )  );
#17303=CARTESIAN_POINT ( 'NONE',  ( 10.81189881249999551, -6.242252689847874514, -114.1562500020483952 ) ) ;
#17304=CARTESIAN_POINT ( 'NONE',  ( -4.999999999999996447, 8.660254037844387298, -124.8750000040967763 ) ) ;
#17305=CARTESIAN_POINT ( 'NONE',  ( 4.999999999999992006, -8.660254037844389075, -111.7499999999999858 ) ) ;
#17309=CARTESIAN_POINT ( 'NONE',  ( -10.81189881249999729, 1.324075727343319199E-15, -56.28125000204836681 ) ) ;
#17313=CARTESIAN_POINT ( 'NONE',  ( -9.999999999999998224, 1.224646799147353059E-15, -109.2499999999999858 ) ) ;
#17318=VERTEX_POINT ( 'NONE', #22322 ) ;
#17324=CIRCLE ( 'NONE', #4259, 24.99999999999999645 ) ;
#17327=CARTESIAN_POINT ( 'NONE',  ( 0.000000000000000000, 0.000000000000000000, -99.99999999999998579 ) ) ;
#17331=CARTESIAN_POINT ( 'NONE',  ( -10.81189881249999729, 6.242252689847871849, -138.7187500020483810 ) ) ;
#17332=CARTESIAN_POINT ( 'NONE',  ( 7.644554776091147741E-16, 12.48450537969573659, -161.4687500020484094 ) ) ;
#17335=CARTESIAN_POINT ( 'NONE',  ( -4.999999999999996447, 8.660254037844387298, -177.0000000000000000 ) ) ;
#17337=CYLINDRICAL_SURFACE ( 'NONE', #34164, 9.999999999999998224 ) ;
#17339=CARTESIAN_POINT ( 'NONE',  ( -10.81189881249999729, 6.242252689847871849, -174.7187500020483810 ) ) ;
#17342=CARTESIAN_POINT ( 'NONE',  ( 10.81189881249999551, -6.242252689847874514, -51.15625000204837391 ) ) ;
#17344=CARTESIAN_POINT ( 'NONE',  ( 5.000000000000000000, 8.660254037844385522, -108.2499999999999858 ) ) ;
#17346=CARTESIAN_POINT ( 'NONE',  ( -10.81189881249999729, -6.242252689847864744, -135.6562500020484094 ) ) ;
#17347=CARTESIAN_POINT ( 'NONE',  ( 4.999999999999992006, -8.660254037844389075, -158.6250000040967905 ) ) ;
#17348=CARTESIAN_POINT ( 'NONE',  ( 10.81189881249999551, -6.242252689847874514, -148.6562500020484094 ) ) ;
#17350=CARTESIAN_POINT ( 'NONE',  ( 5.405949406249992428, -9.363379034771808662, -82.59375000204836681 ) ) ;
#17353=CARTESIAN_POINT ( 'NONE',  ( -2.293366432827344421E-15, -12.48450537969573659, -177.2187500020484094 ) ) ;
#17355=CARTESIAN_POINT ( 'NONE',  ( -5.000000000000003553, -8.660254037844383745, -172.0000000000000000 ) ) ;
#17356=CYLINDRICAL_SURFACE ( 'NONE', #41516, 9.999999999999998224 ) ;
#17357=CARTESIAN_POINT ( 'NONE',  ( 10.81189881249999551, -6.242252689847874514, -76.65625000204838102 ) ) ;
#17360=CARTESIAN_POINT ( 'NONE',  ( 5.000000000000000000, 8.660254037844385522, -54.62500000409675494 ) ) ;
#17361=CARTESIAN_POINT ( 'NONE',  ( 5.405949406249999534, 9.363379034771803333, -11.59375000204834727 ) ) ;
#17364=CARTESIAN_POINT ( 'NONE',  ( -5.405949406250003975, -9.363379034771801557, -2.031250002048373915 ) ) ;
#17374=VERTEX_POINT ( 'NONE', #16233 ) ;
#17375=ORIENTED_EDGE ( 'NONE', *, *, #37933, .F. ) ;
#17376=VECTOR ( 'NONE', #40443, 1000.000000000000000 ) ;
#17380=CARTESIAN_POINT ( 'NONE',  ( -5.000000000000003553, -8.660254037844383745, -122.5000000000000000 ) ) ;
#17381=CARTESIAN_POINT ( 'NONE',  ( -5.000000000000003553, -8.660254037844383745, -42.99999999999998579 ) ) ;
#17384=CARTESIAN_POINT ( 'NONE',  ( 10.81189881249999907, 6.242252689847868297, -167.7187500020483810 ) ) ;
#17386=CARTESIAN_POINT ( 'NONE',  ( -9.999999999999998224, 1.224646799147353059E-15, -100.2499999999999858 ) ) ;
#17387=CARTESIAN_POINT ( 'NONE',  ( -10.00000000000051337, 5.773502691895962435, -146.8749999999999716 ) ) ;
#17390=FACE_OUTER_BOUND ( 'NONE', #39662, .T. ) ;
#17395=CARTESIAN_POINT ( 'NONE',  ( 10.81189881249999907, 6.242252689847868297, -67.21875000204838102 ) ) ;
#17396=CARTESIAN_POINT ( 'NONE',  ( -2.293366432827344421E-15, -12.48450537969573659, -79.90625000204839523 ) ) ;
#17398=CARTESIAN_POINT ( 'NONE',  ( 10.00000000000000000, 5.773502691896255534, -130.8750000000000000 ) ) ;
#17399=CARTESIAN_POINT ( 'NONE',  ( -10.81189881249999729, 1.324075727343319199E-15, -159.7812500020484094 ) ) ;
#17400=CARTESIAN_POINT ( 'NONE',  ( 5.405949406249992428, -9.363379034771808662, -175.7812500020484094 ) ) ;
#17403=CARTESIAN_POINT ( 'NONE',  ( -10.81189881249999729, 1.324075727343319199E-15, -108.5937500020483810 ) ) ;
#17406=CARTESIAN_POINT ( 'NONE',  ( -5.405949406249996869, 9.363379034771805109, -5.531250002048376579 ) ) ;
#17408=CARTESIAN_POINT ( 'NONE',  ( 9.999999999999994671, -5.773502691896262640, -168.6250000000000000 ) ) ;
#17409=CARTESIAN_POINT ( 'NONE',  ( -5.405949406249996869, 9.363379034771805109, -98.53125000204839523 ) ) ;
#17411=CARTESIAN_POINT ( 'NONE',  ( 9.999999999999998224, 0.000000000000000000, -72.87500000409677625 ) ) ;
#17413=CARTESIAN_POINT ( 'NONE',  ( 10.81189881249999729, 0.000000000000000000, -31.34375000204836681 ) ) ;
#17416=CARTESIAN_POINT ( 'NONE',  ( -2.293366432827344421E-15, -12.48450537969573659, -28.90625000204835615 ) ) ;
#17419=CARTESIAN_POINT ( 'NONE',  ( 9.999999999999998224, 0.000000000000000000, -116.3750000040967905 ) ) ;
#17420=CARTESIAN_POINT ( 'NONE',  ( -5.000000000000003553, -8.660254037844383745, -7.375000004096743389 ) ) ;
#17423=CARTESIAN_POINT ( 'NONE',  ( -9.999999999999998224, 0.000000000000000000, -99.99999999999998579 ) ) ;
#17425=ORIENTED_EDGE ( 'NONE', *, *, #20666, .T. ) ;
#17429=( BOUNDED_CURVE ( )  B_SPLINE_CURVE ( 2, ( #39746, #16856, #10181, #502, #13617, #23367, #16427 ),
 .UNSPECIFIED., .F., .F. ) 
 B_SPLINE_CURVE_WITH_KNOTS ( ( 3, 2, 2, 3 ),
 ( 0.3470149253731344974, 0.3482587064676618271, 0.3495024875621891569, 0.3507462686567164867 ),
 .UNSPECIFIED. ) 
 CURVE ( )  GEOMETRIC_REPRESENTATION_ITEM ( )  RATIONAL_B_SPLINE_CURVE ( ( 0.9999999999999820144, 0.8660254037844566932, 1.000000000000000000, 0.8660254037844387076, 1.000000000000000000, 0.8660254037844327124, 1.000000000000005995 ) ) 
 REPRESENTATION_ITEM ( '' )  );
#17436=CARTESIAN_POINT ( 'NONE',  ( 10.81189881249999729, 0.000000000000000000, -174.0312500020484094 ) ) ;
#17439=CARTESIAN_POINT ( 'NONE',  ( 10.81189881249999729, 0.000000000000000000, -92.84375000204838102 ) ) ;
#17440=CARTESIAN_POINT ( 'NONE',  ( 7.070501591499376803E-16, 11.54700538379251284, -106.6249999999999858 ) ) ;
#17441=CARTESIAN_POINT ( 'NONE',  ( 10.81189881249999729, 0.000000000000000000, -103.5312500020483810 ) ) ;
#17443=CARTESIAN_POINT ( 'NONE',  ( 10.81189881249999729, 6.242252689847867408, -109.2187500020483810 ) ) ;
#17446=CARTESIAN_POINT ( 'NONE',  ( -9.999999999999998224, 1.224646799147353059E-15, -153.1250000040967905 ) ) ;
#17447=CARTESIAN_POINT ( 'NONE',  ( 10.81189881249999729, 0.000000000000000000, -195.0312500020484094 ) ) ;
#17450=CARTESIAN_POINT ( 'NONE',  ( -4.999999999999996447, 8.660254037844387298, -168.3750000040967905 ) ) ;
#17452=CARTESIAN_POINT ( 'NONE',  ( -10.81189881249999907, -6.242252689847864744, -24.46875000204837036 ) ) ;
#17453=DIRECTION ( 'NONE',  ( -0.000000000000000000, -0.000000000000000000, -1.000000000000000000 ) ) ;
#17454=CARTESIAN_POINT ( 'NONE',  ( -5.405949406249996869, 9.363379034771805109, -129.8437500020484094 ) ) ;
#17456=CARTESIAN_POINT ( 'NONE',  ( 10.81189881249999551, -6.242252689847874514, -27.15625000204838102 ) ) ;
#17458=CARTESIAN_POINT ( 'NONE',  ( 9.999999999999742428, 5.773502691896404748, -158.2500000040967905 ) ) ;
#17459=CARTESIAN_POINT ( 'NONE',  ( 5.000000000000000000, 8.660254037844385522, -61.74999999999997158 ) ) ;
#17460=CARTESIAN_POINT ( 'NONE',  ( -10.81189881249999907, -6.242252689847864744, -126.6562500020483810 ) ) ;
#17462=VERTEX_POINT ( 'NONE', #2477 ) ;
#17464=CARTESIAN_POINT ( 'NONE',  ( -2.121150477449813534E-15, -11.54700538379251284, -101.7500000040967763 ) ) ;
#17466=CARTESIAN_POINT ( 'NONE',  ( 7.644554776091147741E-16, 12.48450537969573659, -59.46875000204837391 ) ) ;
#17467=ORIENTED_EDGE ( 'NONE', *, *, #32342, .T. ) ;
#17473=CARTESIAN_POINT ( 'NONE',  ( 9.999999999999998224, 0.000000000000000000, -161.0000000000000000 ) ) ;
#17474=CARTESIAN_POINT ( 'NONE',  ( 10.00000000000000000, 5.773502691896255534, -30.75000000409674783 ) ) ;
#17480=VERTEX_POINT ( 'NONE', #40188 ) ;
#17482=EDGE_LOOP ( 'NONE', ( #29831, #10797, #40102, #23183 ) ) ;
#17484=CYLINDRICAL_SURFACE ( 'NONE', #32794, 9.999999999999998224 ) ;
#17487=EDGE_CURVE ( 'NONE', #16776, #20876, #27296, .T. ) ;
#17488=CARTESIAN_POINT ( 'NONE',  ( 7.644554776091147741E-16, 12.48450537969573659, -194.6562500020484094 ) ) ;
#17494=CARTESIAN_POINT ( 'NONE',  ( 5.405949406249992428, -9.363379034771808662, -120.0937500020483952 ) ) ;
#17495=CARTESIAN_POINT ( 'NONE',  ( -5.405949406250003975, -9.363379034771801557, -0.3437500020483652552 ) ) ;
#17496=CARTESIAN_POINT ( 'NONE',  ( 5.405949406249999534, 9.363379034771803333, -124.2812500020483952 ) ) ;
#17498=CARTESIAN_POINT ( 'NONE',  ( -2.293366432827344421E-15, -12.48450537969573659, -127.7187500020483952 ) ) ;
#17500=CARTESIAN_POINT ( 'NONE',  ( 10.00000000000000000, 5.773502691896255534, -151.8750000000000000 ) ) ;
#17501=CARTESIAN_POINT ( 'NONE',  ( 10.00000000000000000, 5.773502691896255534, -19.87499999999997513 ) ) ;
#17506=CARTESIAN_POINT ( 'NONE',  ( 10.81189881249999551, -6.242252689847874514, -46.46875000204836681 ) ) ;
#17508=CARTESIAN_POINT ( 'NONE',  ( 5.405949406249999534, 9.363379034771803333, -151.0937500020483810 ) ) ;
#17512=CARTESIAN_POINT ( 'NONE',  ( 5.132169924948443374, 9.089318513147352618, -179.9999999999999432 ) ) ;
#17513=CARTESIAN_POINT ( 'NONE',  ( -10.00000000000000000, -5.773502691896251982, -86.62499999999997158 ) ) ;
#17515=ORIENTED_EDGE ( 'NONE', *, *, #11748, .F. ) ;
#17516=CARTESIAN_POINT ( 'NONE',  ( -9.999999999999998224, 1.224646799147353059E-15, -164.7500000000000000 ) ) ;
#17517=CARTESIAN_POINT ( 'NONE',  ( 7.070501591499377789E-16, 11.54700538379251284, -123.5000000040967905 ) ) ;
#17520=CARTESIAN_POINT ( 'NONE',  ( 10.81189881249999551, -6.242252689847874514, -51.15625000204837391 ) ) ;
#17531=CARTESIAN_POINT ( 'NONE',  ( 9.999999999998969713, 5.773502691896851502, -103.8750000000000000 ) ) ;
#17539=CARTESIAN_POINT ( 'NONE',  ( -10.81189881249999907, -6.242252689847864744, -144.4687500020484094 ) ) ;
#17540=( BOUNDED_CURVE ( )  B_SPLINE_CURVE ( 2, ( #215, #30199, #26941, #635, #7520, #40098, #20458 ),
 .UNSPECIFIED., .F., .F. ) 
 B_SPLINE_CURVE_WITH_KNOTS ( ( 3, 2, 2, 3 ),
 ( 0.3805970149253732338, 0.3818407960199006190, 0.3830845771144278933, 0.3843283582089552786 ),
 .UNSPECIFIED. ) 
 CURVE ( )  GEOMETRIC_REPRESENTATION_ITEM ( )  RATIONAL_B_SPLINE_CURVE ( ( 0.9999999999999880096, 0.8660254037844506980, 1.000000000000000000, 0.8660254037844387076, 1.000000000000000000, 0.8660254037844327124, 1.000000000000005995 ) ) 
 REPRESENTATION_ITEM ( '' )  );
#17541=CARTESIAN_POINT ( 'NONE',  ( 7.644554776091147741E-16, 12.48450537969573659, -155.4687500020484094 ) ) ;
#17543=CARTESIAN_POINT ( 'NONE',  ( -4.999999999999996447, 8.660254037844387298, -178.5000000000000000 ) ) ;
#17545=FACE_OUTER_BOUND ( 'NONE', #10631, .T. ) ;
#17548=CARTESIAN_POINT ( 'NONE',  ( 5.405949406249999534, 9.363379034771803333, -175.0937500020484094 ) ) ;
#17552=CARTESIAN_POINT ( 'NONE',  ( 5.405949406249999534, 9.363379034771803333, -55.28125000204836681 ) ) ;
#17554=CARTESIAN_POINT ( 'NONE',  ( 10.00000000000000000, 5.773502691896255534, -103.8750000000000000 ) ) ;
#17557=CARTESIAN_POINT ( 'NONE',  ( -2.293366432827344421E-15, -12.48450537969573659, -136.9062500020484094 ) ) ;
#17558=CARTESIAN_POINT ( 'NONE',  ( 7.070501591499377789E-16, 11.54700538379251284, -147.5000000040968189 ) ) ;
#17559=CARTESIAN_POINT ( 'NONE',  ( 5.405949406249999534, 9.363379034771803333, -151.2812500020484094 ) ) ;
#17563=CARTESIAN_POINT ( 'NONE',  ( 5.405949406249999534, 9.363379034771803333, -182.5937500020483810 ) ) ;
#17567=CARTESIAN_POINT ( 'NONE',  ( 10.81189881249999729, 0.000000000000000000, -75.03125000204838102 ) ) ;
#17569=CARTESIAN_POINT ( 'NONE',  ( 4.999999999999992006, -8.660254037844389075, -53.62500000409675494 ) ) ;
#17570=CARTESIAN_POINT ( 'NONE',  ( 7.644554776091147741E-16, 12.48450537969573659, -11.46875000204836148 ) ) ;
#17573=CARTESIAN_POINT ( 'NONE',  ( -2.293366432827344421E-15, -12.48450537969573659, -3.406250002048361036 ) ) ;
#17574=CYLINDRICAL_SURFACE ( 'NONE', #32554, 9.999999999999998224 ) ;
#17577=CARTESIAN_POINT ( 'NONE',  ( 9.999999999999998224, 1.224646799147353059E-15, -99.99999999999998579 ) ) ;
#17580=EDGE_CURVE ( 'NONE', #19560, #22477, #40258, .T. ) ;
#17582=VERTEX_POINT ( 'NONE', #729 ) ;
#17592=CARTESIAN_POINT ( 'NONE',  ( -5.000000000000003553, -8.660254037844383745, -41.49999999999997868 ) ) ;
#17594=CARTESIAN_POINT ( 'NONE',  ( -2.293366432827344421E-15, -12.48450537969573659, -169.7187500020483810 ) ) ;
#17595=EDGE_CURVE ( 'NONE', #25998, #18722, #39554, .T. ) ;
#17596=CARTESIAN_POINT ( 'NONE',  ( 10.81189881249999729, 6.242252689847867408, -179.7187500020484094 ) ) ;
#17598=FACE_OUTER_BOUND ( 'NONE', #8058, .T. ) ;
#17602=DIRECTION ( 'NONE',  ( -0.000000000000000000, -0.000000000000000000, -1.000000000000000000 ) ) ;
#17605=CARTESIAN_POINT ( 'NONE',  ( 5.405949406249999534, 9.363379034771803333, -70.09375000204836681 ) ) ;
#17606=CARTESIAN_POINT ( 'NONE',  ( 10.81189881249999551, -6.242252689847874514, -75.15625000204838102 ) ) ;
#17608=CARTESIAN_POINT ( 'NONE',  ( -2.121150477449813534E-15, -11.54700538379251284, -132.8750000000000000 ) ) ;
#17609=AXIS2_PLACEMENT_3D ( 'NONE', #13491, #6412, #16943 ) ;
#17610=CARTESIAN_POINT ( 'NONE',  ( -5.405949406250003975, -9.363379034771801557, -155.0312500020484094 ) ) ;
#17611=CARTESIAN_POINT ( 'NONE',  ( 10.81189881249999907, 6.242252689847868297, -172.4062500020484094 ) ) ;
#17614=CARTESIAN_POINT ( 'NONE',  ( -2.293366432827344421E-15, -12.48450537969573659, -109.7187500020483668 ) ) ;
#17617=CARTESIAN_POINT ( 'NONE',  ( -2.293366432827344421E-15, -12.48450537969573659, -1.906250002048359704 ) ) ;
#17619=AXIS2_PLACEMENT_3D ( 'NONE', #12299, #32184, #2819 ) ;
#17621=CARTESIAN_POINT ( 'NONE',  ( 7.644554776091147741E-16, 12.48450537969573659, -97.15625000204839523 ) ) ;
#17623=CARTESIAN_POINT ( 'NONE',  ( 4.999999999999992006, -8.660254037844389075, -76.12500000409677625 ) ) ;
#17625=CARTESIAN_POINT ( 'NONE',  ( 10.81189881249999551, -6.242252689847874514, -31.46875000204835260 ) ) ;
#17628=CARTESIAN_POINT ( 'NONE',  ( -5.405949406249996869, 9.363379034771805109, -26.53125000204836681 ) ) ;
#17631=CARTESIAN_POINT ( 'NONE',  ( -2.121150477449813534E-15, -11.54700538379251284, -7.250000004096756712 ) ) ;
#17635=CARTESIAN_POINT ( 'NONE',  ( 5.000000000000000000, 8.660254037844385522, -120.2500000000000000 ) ) ;
#17641=VERTEX_POINT ( 'NONE', #24026 ) ;
#17645=FACE_OUTER_BOUND ( 'NONE', #41963, .T. ) ;
#17647=CARTESIAN_POINT ( 'NONE',  ( -5.405949406249996869, 9.363379034771805109, -176.5312500020483810 ) ) ;
#17648=ADVANCED_FACE ( 'NONE', ( #37166 ), #32885, .F. ) ;
#17650=CARTESIAN_POINT ( 'NONE',  ( -10.81189881249999729, 6.242252689847871849, -93.71875000204838102 ) ) ;
#17652=CARTESIAN_POINT ( 'NONE',  ( -10.00000000000051337, 5.773502691895962435, -112.7500000040967620 ) ) ;
#17653=CARTESIAN_POINT ( 'NONE',  ( -10.81189881249999907, -6.242252689847864744, -102.6562500020483952 ) ) ;
#17655=CARTESIAN_POINT ( 'NONE',  ( 10.81189881249999729, 0.000000000000000000, -104.8437500020483810 ) ) ;
#17659=CARTESIAN_POINT ( 'NONE',  ( 5.405949406249999534, 9.363379034771803333, -194.7812500020484094 ) ) ;
#17662=CARTESIAN_POINT ( 'NONE',  ( 10.00000000000000000, 5.773502691896255534, -174.7500000040968189 ) ) ;
#17664=CARTESIAN_POINT ( 'NONE',  ( 10.81189881249999729, 0.000000000000000000, -20.84375000204835615 ) ) ;
#17666=CARTESIAN_POINT ( 'NONE',  ( 10.81189881249999729, 0.000000000000000000, -127.3437500020483952 ) ) ;
#17668=CARTESIAN_POINT ( 'NONE',  ( 10.81189881249999551, -6.242252689847874514, -31.65625000204835615 ) ) ;
#17670=CARTESIAN_POINT ( 'NONE',  ( -9.999999999999998224, 1.224646799147353059E-15, -61.24999999999997158 ) ) ;
#17671=CARTESIAN_POINT ( 'NONE',  ( -10.81189881249999729, 6.242252689847871849, -123.9062500020483952 ) ) ;
#17673=ORIENTED_EDGE ( 'NONE', *, *, #34120, .F. ) ;
#17675=CARTESIAN_POINT ( 'NONE',  ( 9.999999999999998224, 0.000000000000000000, -98.37500000409677625 ) ) ;
#17676=CARTESIAN_POINT ( 'NONE',  ( 0.000000000000000000, 0.000000000000000000, -99.99999999999998579 ) ) ;
#17678=CARTESIAN_POINT ( 'NONE',  ( -10.81189881249999907, -6.242252689847864744, -58.96875000204838102 ) ) ;
#17683=CYLINDRICAL_SURFACE ( 'NONE', #22863, 9.999999999999998224 ) ;
#17684=CARTESIAN_POINT ( 'NONE',  ( 9.999999999999996447, -5.773502691896262640, -31.00000000409675138 ) ) ;
#17689=CARTESIAN_POINT ( 'NONE',  ( -10.00000000000076916, 5.773502691895813221, -129.2500000040967905 ) ) ;
#17693=ORIENTED_EDGE ( 'NONE', *, *, #35673, .T. ) ;
#17697=CARTESIAN_POINT ( 'NONE',  ( -2.293366432827344421E-15, -12.48450537969573659, -195.4062500020484094 ) ) ;
#17703=ADVANCED_FACE ( 'NONE', ( #23385 ), #36534, .F. ) ;
#17705=CARTESIAN_POINT ( 'NONE',  ( 5.405949406249999534, 9.363379034771803333, -115.0937500020483810 ) ) ;
#17706=CARTESIAN_POINT ( 'NONE',  ( 9.999999999999998224, 0.000000000000000000, -197.3750000040967905 ) ) ;
#17707=CARTESIAN_POINT ( 'NONE',  ( -5.405949406249996869, 9.363379034771805109, -122.5312500020483952 ) ) ;
#17709=CARTESIAN_POINT ( 'NONE',  ( -10.81189881249999729, -6.242252689847864744, -130.9687500020483810 ) ) ;
#17712=CARTESIAN_POINT ( 'NONE',  ( -5.000000000000003553, -8.660254037844383745, -154.0000000000000000 ) ) ;
#17713=CARTESIAN_POINT ( 'NONE',  ( 5.000000000000000000, 8.660254037844385522, -22.74999999999996447 ) ) ;
#17718=CARTESIAN_POINT ( 'NONE',  ( 10.81189881249999907, 6.242252689847868297, -44.71875000204835970 ) ) ;
#17720=CARTESIAN_POINT ( 'NONE',  ( -10.81189881249999729, 1.324075727343319199E-15, -153.5937500020483810 ) ) ;
#17723=DIRECTION ( 'NONE',  ( -1.000000000000000000, 0.000000000000000000, 0.000000000000000000 ) ) ;
#17724=CARTESIAN_POINT ( 'NONE',  ( -10.00000000000000000, -5.773502691896251982, -80.62499999999998579 ) ) ;
#17727=CARTESIAN_POINT ( 'NONE',  ( -2.293366432827344421E-15, -12.48450537969573659, -102.4062500020484094 ) ) ;
#17728=CARTESIAN_POINT ( 'NONE',  ( -5.000000000000003553, -8.660254037844383745, -125.8750000040967905 ) ) ;
#17733=CARTESIAN_POINT ( 'NONE',  ( 7.644554776091147741E-16, 12.48450537969573659, -47.65625000204837391 ) ) ;
#17741=VERTEX_POINT ( 'NONE', #24887 ) ;
#17746=VECTOR ( 'NONE', #5691, 1000.000000000000000 ) ;
#17750=DIRECTION ( 'NONE',  ( -0.000000000000000000, -0.000000000000000000, -1.000000000000000000 ) ) ;
#17752=EDGE_CURVE ( 'NONE', #26823, #28777, #1979, .T. ) ;
#17755=( BOUNDED_CURVE ( )  B_SPLINE_CURVE ( 2, ( #32367, #9888, #29122, #25879, #26090, #9253, #9679 ),
 .UNSPECIFIED., .F., .F. ) 
 B_SPLINE_CURVE_WITH_KNOTS ( ( 3, 2, 2, 3 ),
 ( 0.1380597014925373234, 0.1393034825870646809, 0.1405472636815920384, 0.1417910447761193959 ),
 .UNSPECIFIED. ) 
 CURVE ( )  GEOMETRIC_REPRESENTATION_ITEM ( )  RATIONAL_B_SPLINE_CURVE ( ( 1.000000000000000000, 0.8660254037844387076, 1.000000000000000000, 0.8660254037844387076, 1.000000000000000000, 0.8660254037844387076, 1.000000000000000000 ) ) 
 REPRESENTATION_ITEM ( '' )  );
#17757=CARTESIAN_POINT ( 'NONE',  ( 10.81189881249999551, -6.242252689847874514, -139.4687500020483810 ) ) ;
#17758=CARTESIAN_POINT ( 'NONE',  ( 10.81189881249999907, 6.242252689847868297, -146.9062500020484094 ) ) ;
#17759=CARTESIAN_POINT ( 'NONE',  ( 10.81189881249999729, 0.000000000000000000, -155.8437500020483810 ) ) ;
#17760=EDGE_CURVE ( 'NONE', #25374, #23494, #38898, .T. ) ;
#17763=CARTESIAN_POINT ( 'NONE',  ( -9.999999999999998224, 1.224646799147353059E-15, -181.2500000000000284 ) ) ;
#17769=CARTESIAN_POINT ( 'NONE',  ( -2.293366432827344421E-15, -12.48450537969573659, -174.2187500020484094 ) ) ;
#17772=FACE_OUTER_BOUND ( 'NONE', #18236, .T. ) ;
#17773=CARTESIAN_POINT ( 'NONE',  ( 7.644554776091147741E-16, 12.48450537969573659, -41.65625000204837391 ) ) ;
#17775=CARTESIAN_POINT ( 'NONE',  ( -9.999999999999998224, 1.224646799147353059E-15, -106.2499999999999858 ) ) ;
#17777=CARTESIAN_POINT ( 'NONE',  ( 7.644554776091147741E-16, 12.48450537969573659, -130.1562500020483810 ) ) ;
#17778=CARTESIAN_POINT ( 'NONE',  ( 9.999999999999996447, -5.773502691896262640, -146.5000000040967905 ) ) ;
#17779=CARTESIAN_POINT ( 'NONE',  ( -9.999999999999998224, 1.224646799147353059E-15, -160.2500000000000000 ) ) ;
#17783=CARTESIAN_POINT ( 'NONE',  ( -10.81189881249999907, -6.242252689847864744, -175.9687500020483526 ) ) ;
#17788=CARTESIAN_POINT ( 'NONE',  ( -10.81189881249999907, -6.242252689847864744, -69.65625000204839523 ) ) ;
#17791=CARTESIAN_POINT ( 'NONE',  ( 5.000000000000000000, 8.660254037844385522, -50.12500000409675494 ) ) ;
#17792=CARTESIAN_POINT ( 'NONE',  ( 10.81189881249999551, -6.242252689847874514, -5.968750002048355263 ) ) ;
#17796=CARTESIAN_POINT ( 'NONE',  ( 7.070501591499376803E-16, 11.54700538379251284, -138.5000000040967905 ) ) ;
#17801=VERTEX_POINT ( 'NONE', #24675 ) ;
#17803=CYLINDRICAL_SURFACE ( 'NONE', #39941, 9.999999999999998224 ) ;
#17804=ORIENTED_EDGE ( 'NONE', *, *, #31687, .T. ) ;
#17812=CARTESIAN_POINT ( 'NONE',  ( 5.000000000000000000, 8.660254037844385522, -46.74999999999998579 ) ) ;
#17815=CARTESIAN_POINT ( 'NONE',  ( 10.81189881249999551, -6.242252689847874514, -161.9687500020484094 ) ) ;
#17816=CARTESIAN_POINT ( 'NONE',  ( -10.81189881249999729, 6.242252689847871849, -179.2187500020484379 ) ) ;
#17825=CARTESIAN_POINT ( 'NONE',  ( 5.405949406249992428, -9.363379034771808662, -63.09375000204836681 ) ) ;
#17826=CARTESIAN_POINT ( 'NONE',  ( -10.81189881249999907, -6.242252689847864744, -71.15625000204839523 ) ) ;
#17828=CARTESIAN_POINT ( 'NONE',  ( 9.999999999999996447, -5.773502691896262640, -129.6250000000000000 ) ) ;
#17829=CARTESIAN_POINT ( 'NONE',  ( -5.405949406249996869, 9.363379034771805109, -154.0312500020484094 ) ) ;
#17830=CARTESIAN_POINT ( 'NONE',  ( 10.81189881249999729, 0.000000000000000000, -168.0312500020484094 ) ) ;
#17832=CARTESIAN_POINT ( 'NONE',  ( 7.644554776091147741E-16, 12.48450537969573659, -0.9687500020483519325 ) ) ;
#17833=CARTESIAN_POINT ( 'NONE',  ( -5.405949406250003975, -9.363379034771801557, -96.34375000204838102 ) ) ;
#17836=CARTESIAN_POINT ( 'NONE',  ( -10.81189881249999907, -6.242252689847864744, -0.6562500020483587049 ) ) ;
#17839=CARTESIAN_POINT ( 'NONE',  ( -5.405949406250003975, -9.363379034771801557, -101.0312500020483952 ) ) ;
#17841=CARTESIAN_POINT ( 'NONE',  ( 10.00000000000000000, 5.773502691896255534, -77.25000000409677625 ) ) ;
#17843=CARTESIAN_POINT ( 'NONE',  ( 5.405949406249992428, -9.363379034771808662, -37.59375000204837391 ) ) ;
#17844=ORIENTED_EDGE ( 'NONE', *, *, #24680, .T. ) ;
#17846=CARTESIAN_POINT ( 'NONE',  ( 5.405949406249999534, 9.363379034771803333, -28.28125000204837036 ) ) ;
#17849=CARTESIAN_POINT ( 'NONE',  ( 7.070501591499377789E-16, 11.54700538379251284, -5.000000004096755823 ) ) ;
#17863=CARTESIAN_POINT ( 'NONE',  ( -9.999999999999998224, 1.224646799147353059E-15, -101.7500000000000000 ) ) ;
#17865=CARTESIAN_POINT ( 'NONE',  ( -10.00000000000051337, 5.773502691895962435, -105.2500000040967620 ) ) ;
#17866=CARTESIAN_POINT ( 'NONE',  ( 10.81189881249999729, 0.000000000000000000, -165.0312500020484094 ) ) ;
#17869=CARTESIAN_POINT ( 'NONE',  ( 10.81189881249999551, -6.242252689847874514, -82.46875000204836681 ) ) ;
#17871=CARTESIAN_POINT ( 'NONE',  ( 10.81189881249999907, 6.242252689847868297, -196.2187500020484094 ) ) ;
#17872=CARTESIAN_POINT ( 'NONE',  ( -10.81189881249999907, -6.242252689847864744, -89.15625000204839523 ) ) ;
#17874=CARTESIAN_POINT ( 'NONE',  ( -5.405949406249996869, 9.363379034771805109, -104.3437500020483810 ) ) ;
#17878=CARTESIAN_POINT ( 'NONE',  ( -5.405949406250003975, -9.363379034771801557, -194.0312500020484094 ) ) ;
#17880=CARTESIAN_POINT ( 'NONE',  ( -5.000000000000003553, -8.660254037844383745, -169.3750000040967905 ) ) ;
#17882=CARTESIAN_POINT ( 'NONE',  ( -5.405949406249996869, 9.363379034771805109, -23.34375000204835970 ) ) ;
#17883=CARTESIAN_POINT ( 'NONE',  ( -10.81189881249999729, 6.242252689847871849, -128.2187500020483810 ) ) ;
#17885=CARTESIAN_POINT ( 'NONE',  ( 5.405949406249999534, 9.363379034771803333, -29.78125000204837036 ) ) ;
#17888=CARTESIAN_POINT ( 'NONE',  ( -9.999999999999998224, 1.224646799147353059E-15, -49.24999999999998579 ) ) ;
#17889=CARTESIAN_POINT ( 'NONE',  ( 10.81189881249999729, 0.000000000000000000, -121.5312500020483952 ) ) ;
#17892=CARTESIAN_POINT ( 'NONE',  ( -5.000000000000003553, -8.660254037844383745, -97.37500000409677625 ) ) ;
#17893=CARTESIAN_POINT ( 'NONE',  ( 9.999999999999998224, 0.000000000000000000, -112.9999999999999858 ) ) ;
#17895=CARTESIAN_POINT ( 'NONE',  ( -10.81189881249999729, 6.242252689847871849, -56.21875000204837391 ) ) ;
#17901=EDGE_CURVE ( 'NONE', #22578, #7470, #9395, .T. ) ;
#17904=CARTESIAN_POINT ( 'NONE',  ( -9.999999999999998224, 5.773502691896259087, -27.25000000409677625 ) ) ;
#17905=CARTESIAN_POINT ( 'NONE',  ( -4.999999999999996447, 8.660254037844387298, -168.0000000000000000 ) ) ;
#17908=CYLINDRICAL_SURFACE ( 'NONE', #32802, 9.999999999999998224 ) ;
#17917=CARTESIAN_POINT ( 'NONE',  ( -5.405949406250003975, -9.363379034771801557, -192.5312500020484094 ) ) ;
#17923=CARTESIAN_POINT ( 'NONE',  ( -10.81189881249999729, 6.242252689847871849, -114.7187500020483810 ) ) ;
#17925=CARTESIAN_POINT ( 'NONE',  ( -10.81189881249999729, 1.324075727343319199E-15, -125.2812500020483668 ) ) ;
#17927=CARTESIAN_POINT ( 'NONE',  ( 10.81189881249999729, 6.242252689847867408, -131.7187500020483810 ) ) ;
#17928=CARTESIAN_POINT ( 'NONE',  ( 7.070501591499376803E-16, 11.54700538379251284, -163.6250000000000284 ) ) ;
#17930=CARTESIAN_POINT ( 'NONE',  ( -5.000000000000003553, -8.660254037844383745, -149.5000000000000000 ) ) ;
#17931=CARTESIAN_POINT ( 'NONE',  ( -2.121150477449813534E-15, -11.54700538379251284, -23.37499999999997868 ) ) ;
#17936=CARTESIAN_POINT ( 'NONE',  ( 10.81189881249999907, 6.242252689847868297, -43.21875000204835970 ) ) ;
#17938=CARTESIAN_POINT ( 'NONE',  ( -10.81189881249999907, -6.242252689847864744, -153.4687500020484094 ) ) ;
#17942=CARTESIAN_POINT ( 'NONE',  ( -5.000000000000003553, -8.660254037844383745, -75.99999999999998579 ) ) ;
#17946=CARTESIAN_POINT ( 'NONE',  ( -10.81189881249999729, -6.242252689847864744, -101.1562500020483952 ) ) ;
#17947=CARTESIAN_POINT ( 'NONE',  ( -4.999999999999996447, 8.660254037844387298, -120.3750000040967905 ) ) ;
#17950=VECTOR ( 'NONE', #40448, 1000.000000000000000 ) ;
#17951=CARTESIAN_POINT ( 'NONE',  ( 10.81189881249999729, 0.000000000000000000, -43.53125000204838102 ) ) ;
#17961=ORIENTED_EDGE ( 'NONE', *, *, #41735, .F. ) ;
#17972=CARTESIAN_POINT ( 'NONE',  ( -5.405949406250003975, -9.363379034771801557, -141.3437500020483810 ) ) ;
#17973=CARTESIAN_POINT ( 'NONE',  ( -10.81189881249999729, 6.242252689847871849, -144.9062500020484094 ) ) ;
#17974=CARTESIAN_POINT ( 'NONE',  ( 7.644554776091147741E-16, 12.48450537969573659, -150.9687500020484094 ) ) ;
#17976=CARTESIAN_POINT ( 'NONE',  ( 0.000000000000000000, 0.000000000000000000, -99.99999999999998579 ) ) ;
#17977=CARTESIAN_POINT ( 'NONE',  ( 4.999999999999992006, -8.660254037844389075, -173.2500000000000284 ) ) ;
#17979=DIRECTION ( 'NONE',  ( -0.000000000000000000, -0.000000000000000000, -1.000000000000000000 ) ) ;
#17982=CARTESIAN_POINT ( 'NONE',  ( -10.81189881249999729, 1.324075727343319199E-15, -176.0937500020484094 ) ) ;
#17986=CARTESIAN_POINT ( 'NONE',  ( -10.81189881249999907, -6.242252689847864744, -41.15625000204836681 ) ) ;
#17988=CARTESIAN_POINT ( 'NONE',  ( 10.00000000000000000, 5.773502691896255534, -106.8749999999999716 ) ) ;
#17990=CARTESIAN_POINT ( 'NONE',  ( -10.81189881249999729, 6.242252689847871849, -123.9062500020483810 ) ) ;
#17991=CARTESIAN_POINT ( 'NONE',  ( -9.999999999999998224, 1.224646799147353059E-15, -145.6250000040967905 ) ) ;
#17995=CARTESIAN_POINT ( 'NONE',  ( -2.293366432827344421E-15, -12.48450537969573659, -172.7187500020484094 ) ) ;
#17997=DIRECTION ( 'NONE',  ( -0.7071067811865451302, 8.659560562354903276E-17, 0.7071067811865500152 ) ) ;
#17999=CARTESIAN_POINT ( 'NONE',  ( -10.81189881249999907, -6.242252689847864744, -71.15625000204839523 ) ) ;
#18001=CARTESIAN_POINT ( 'NONE',  ( -2.121150477449813534E-15, -11.54700538379251284, -47.75000000409676204 ) ) ;
#18002=CARTESIAN_POINT ( 'NONE',  ( 5.405949406249999534, 9.363379034771803333, -2.593750002048367254 ) ) ;
#18007=DIRECTION ( 'NONE',  ( -0.000000000000000000, -0.000000000000000000, -1.000000000000000000 ) ) ;
#18012=EDGE_CURVE ( 'NONE', #27414, #36340, #6626, .T. ) ;
#18015=CARTESIAN_POINT ( 'NONE',  ( -9.999999999999998224, 1.224646799147353059E-15, -127.6250000040967620 ) ) ;
#18028=EDGE_LOOP ( 'NONE', ( #35948, #24849, #14452, #38544 ) ) ;
#18030=CARTESIAN_POINT ( 'NONE',  ( 7.070501591499377789E-16, 11.54700538379251284, -39.12499999999997158 ) ) ;
#18032=CARTESIAN_POINT ( 'NONE',  ( -10.81189881249999729, 1.324075727343319199E-15, -168.5937500020484094 ) ) ;
#18034=CARTESIAN_POINT ( 'NONE',  ( 10.81189881249999729, 0.000000000000000000, -179.8437500020483810 ) ) ;
#18035=CARTESIAN_POINT ( 'NONE',  ( 9.999999999999998224, 0.000000000000000000, -167.3750000040967905 ) ) ;
#18036=CARTESIAN_POINT ( 'NONE',  ( -4.999999999999996447, 8.660254037844387298, -103.8750000040967763 ) ) ;
#18038=CARTESIAN_POINT ( 'NONE',  ( 7.070501591499377789E-16, 11.54700538379251284, -195.1250000000000284 ) ) ;
#18043=CARTESIAN_POINT ( 'NONE',  ( -10.81189881249999729, 6.242252689847871849, -59.21875000204837391 ) ) ;
#18044=CARTESIAN_POINT ( 'NONE',  ( 7.644554776091147741E-16, 12.48450537969573659, -68.65625000204839523 ) ) ;
#18046=CARTESIAN_POINT ( 'NONE',  ( 9.999999999999998224, 0.000000000000000000, -128.0000000000000000 ) ) ;
#18047=CARTESIAN_POINT ( 'NONE',  ( 5.405949406249992428, -9.363379034771808662, -153.2812500020484094 ) ) ;
#18048=CARTESIAN_POINT ( 'NONE',  ( 5.405949406249992428, -9.363379034771808662, -160.7812500020484094 ) ) ;
#18052=CARTESIAN_POINT ( 'NONE',  ( 10.81189881249999551, -6.242252689847874514, -100.4687500020483952 ) ) ;
#18055=CARTESIAN_POINT ( 'NONE',  ( 7.644554776091147741E-16, 12.48450537969573659, -198.9687500020484094 ) ) ;
#18058=CARTESIAN_POINT ( 'NONE',  ( 2.519142624249889106, -10.23978606567555083, -180.0000000000000000 ) ) ;
#18059=CARTESIAN_POINT ( 'NONE',  ( -10.81189881249999729, 6.242252689847871849, -90.90625000204838102 ) ) ;
#18061=CARTESIAN_POINT ( 'NONE',  ( -4.999999999999996447, 8.660254037844387298, -69.37500000409677625 ) ) ;
#18062=CARTESIAN_POINT ( 'NONE',  ( -9.999999999999998224, 1.224646799147353059E-15, -118.2500000000000000 ) ) ;
#18063=CARTESIAN_POINT ( 'NONE',  ( -10.81189881249999907, -6.242252689847864744, -27.46875000204837391 ) ) ;
#18066=CARTESIAN_POINT ( 'NONE',  ( -10.81189881249999729, 6.242252689847871849, -18.90625000204837391 ) ) ;
#18068=CARTESIAN_POINT ( 'NONE',  ( -9.999999999999998224, 1.224646799147353059E-15, -119.7500000000000000 ) ) ;
#18069=CARTESIAN_POINT ( 'NONE',  ( -9.999999999999998224, 1.224646799147353059E-15, -3.125000004096767370 ) ) ;
#18072=VECTOR ( 'NONE', #32127, 1000.000000000000000 ) ;
#18085=FACE_OUTER_BOUND ( 'NONE', #8008, .T. ) ;
#18086=CARTESIAN_POINT ( 'NONE',  ( -9.999999999999998224, 1.224646799147353059E-15, -129.1250000040967620 ) ) ;
#18088=CARTESIAN_POINT ( 'NONE',  ( -10.81189881249999729, 6.242252689847871849, -165.9062500020483810 ) ) ;
#18091=CARTESIAN_POINT ( 'NONE',  ( 10.81189881249999907, 6.242252689847868297, -83.71875000204836681 ) ) ;
#18093=CARTESIAN_POINT ( 'NONE',  ( -10.81189881249999907, -6.242252689847864744, -192.4687500020484094 ) ) ;
#18094=CARTESIAN_POINT ( 'NONE',  ( 10.81189881249999729, 0.000000000000000000, -91.53125000204838102 ) ) ;
#18098=CARTESIAN_POINT ( 'NONE',  ( 7.644554776091147741E-16, 12.48450537969573659, -178.1562500020484094 ) ) ;
#18099=CARTESIAN_POINT ( 'NONE',  ( 5.405949406249999534, 9.363379034771803333, -187.2812500020484094 ) ) ;
#18101=CARTESIAN_POINT ( 'NONE',  ( -2.121150477449813534E-15, -11.54700538379251284, -161.7500000040967620 ) ) ;
#18103=CARTESIAN_POINT ( 'NONE',  ( -2.293366432827344421E-15, -12.48450537969573659, -16.71875000204836681 ) ) ;
#18105=CARTESIAN_POINT ( 'NONE',  ( 10.81189881249999729, 0.000000000000000000, -124.3437500020483952 ) ) ;
#18107=CARTESIAN_POINT ( 'NONE',  ( -10.81189881249999907, -6.242252689847864744, -21.65625000204838102 ) ) ;
#18110=CARTESIAN_POINT ( 'NONE',  ( 4.999999999999992006, -8.660254037844389075, -50.24999999999998579 ) ) ;
#18111=CARTESIAN_POINT ( 'NONE',  ( 10.81189881249999907, 6.242252689847868297, -112.4062500020483952 ) ) ;
#18114=CARTESIAN_POINT ( 'NONE',  ( 4.999999999999992006, -8.660254037844389075, -100.1250000040967905 ) ) ;
#18117=CARTESIAN_POINT ( 'NONE',  ( -5.405949406250003975, -9.363379034771801557, -46.84375000204838102 ) ) ;
#18123=CARTESIAN_POINT ( 'NONE',  ( -2.121150477449813534E-15, -11.54700538379251284, -29.75000000409674783 ) ) ;
#18124=FACE_OUTER_BOUND ( 'NONE', #19356, .T. ) ;
#18132=ORIENTED_EDGE ( 'NONE', *, *, #23049, .F. ) ;
#18133=ORIENTED_EDGE ( 'NONE', *, *, #18202, .T. ) ;
#18134=FACE_OUTER_BOUND ( 'NONE', #7739, .T. ) ;
#18137=CARTESIAN_POINT ( 'NONE',  ( -2.293366432827344421E-15, -12.48450537969573659, -184.9062500020484094 ) ) ;
#18142=CARTESIAN_POINT ( 'NONE',  ( -2.293366432827344421E-15, -12.48450537969573659, -109.7187500020483668 ) ) ;
#18143=CARTESIAN_POINT ( 'NONE',  ( -9.999999999999998224, 1.224646799147353059E-15, -144.1250000040967905 ) ) ;
#18144=CARTESIAN_POINT ( 'NONE',  ( -2.293366432827344421E-15, -12.48450537969573659, -120.4062500020483952 ) ) ;
#18146=CARTESIAN_POINT ( 'NONE',  ( -10.81189881249999729, 6.242252689847871849, -131.2187500020483810 ) ) ;
#18150=CARTESIAN_POINT ( 'NONE',  ( -10.00000000000000000, -5.773502691896251982, -146.6249999999999716 ) ) ;
#18151=CARTESIAN_POINT ( 'NONE',  ( 7.070501591499377789E-16, 11.54700538379251284, -13.62499999999996980 ) ) ;
#18154=CARTESIAN_POINT ( 'NONE',  ( 7.070501591499377789E-16, 11.54700538379251284, -185.0000000040967905 ) ) ;
#18156=CARTESIAN_POINT ( 'NONE',  ( 5.405949406249992428, -9.363379034771808662, -39.09375000204837391 ) ) ;
#18158=CARTESIAN_POINT ( 'NONE',  ( 10.81189881249999729, 0.000000000000000000, -148.3437500020483810 ) ) ;
#18160=( BOUNDED_CURVE ( )  B_SPLINE_CURVE ( 2, ( #41036, #8484, #11479, #21416, #5240, #1800, #28770 ),
 .UNSPECIFIED., .F., .F. ) 
 B_SPLINE_CURVE_WITH_KNOTS ( ( 3, 2, 2, 3 ),
 ( 0.3097014925373136052, 0.3109452736318408794, 0.3121890547263682092, 0.3134328358208955390 ),
 .UNSPECIFIED. ) 
 CURVE ( )  GEOMETRIC_REPRESENTATION_ITEM ( )  RATIONAL_B_SPLINE_CURVE ( ( 0.9999999999999820144, 0.8660254037844566932, 1.000000000000000000, 0.8660254037844387076, 1.000000000000000000, 0.8660254037844387076, 1.000000000000000000 ) ) 
 REPRESENTATION_ITEM ( '' )  );
#18162=CARTESIAN_POINT ( 'NONE',  ( 10.00000000000000000, 5.773502691896255534, -76.87499999999997158 ) ) ;
#18165=CARTESIAN_POINT ( 'NONE',  ( -10.81189881249999729, 6.242252689847871849, -102.9062500020483952 ) ) ;
#18166=CARTESIAN_POINT ( 'NONE',  ( -10.00000000000000000, -5.773502691896251982, -127.5000000040967905 ) ) ;
#18167=CARTESIAN_POINT ( 'NONE',  ( -9.999999999999479527, -5.773502691896549521, -144.0000000040967620 ) ) ;
#18168=CARTESIAN_POINT ( 'NONE',  ( 10.81189881249999729, 0.000000000000000000, -80.84375000204838102 ) ) ;
#18171=CARTESIAN_POINT ( 'NONE',  ( 10.81189881249999551, -6.242252689847874514, -42.15625000204836681 ) ) ;
#18178=CARTESIAN_POINT ( 'NONE',  ( -5.000000000000003553, -8.660254037844383745, -121.0000000000000000 ) ) ;
#18179=ORIENTED_EDGE ( 'NONE', *, *, #40656, .T. ) ;
#18180=EDGE_CURVE ( 'NONE', #15306, #38211, #25173, .T. ) ;
#18191=CARTESIAN_POINT ( 'NONE',  ( -10.81189881249999729, 1.324075727343319199E-15, -132.5937500020483810 ) ) ;
#18192=CARTESIAN_POINT ( 'NONE',  ( 10.81189881249999551, -6.242252689847874514, -138.1562500020484094 ) ) ;
#18193=CARTESIAN_POINT ( 'NONE',  ( -10.81189881249999729, 6.242252689847871849, -158.2187500020483810 ) ) ;
#18194=CARTESIAN_POINT ( 'NONE',  ( -9.999999999999998224, 1.224646799147353059E-15, -127.2499999999999716 ) ) ;
#18195=( BOUNDED_CURVE ( )  B_SPLINE_CURVE ( 2, ( #30869, #27416, #18919, #35338, #40552, #4532, #32102 ),
 .UNSPECIFIED., .F., .F. ) 
 B_SPLINE_CURVE_WITH_KNOTS ( ( 3, 2, 2, 3 ),
 ( 0.4067164179104478250, 0.4079601990049751548, 0.4092039800995025400, 0.4104477611940299253 ),
 .UNSPECIFIED. ) 
 CURVE ( )  GEOMETRIC_REPRESENTATION_ITEM ( )  RATIONAL_B_SPLINE_CURVE ( ( 0.9999999999999940048, 0.8660254037844447028, 1.000000000000000000, 0.8660254037844387076, 1.000000000000000000, 0.8660254037844327124, 1.000000000000005995 ) ) 
 REPRESENTATION_ITEM ( '' )  );
#18197=CARTESIAN_POINT ( 'NONE',  ( 10.00000000000000000, 5.773502691896255534, -169.8750000000000000 ) ) ;
#18199=CARTESIAN_POINT ( 'NONE',  ( 9.999999999999998224, 0.000000000000000000, -135.5000000000000000 ) ) ;
#18202=EDGE_CURVE ( 'NONE', #33493, #22601, #41136, .T. ) ;
#18203=CARTESIAN_POINT ( 'NONE',  ( 5.405949406249992428, -9.363379034771808662, -177.0937500020484094 ) ) ;
#18207=CARTESIAN_POINT ( 'NONE',  ( 5.405949406249992428, -9.363379034771808662, -46.78125000204838813 ) ) ;
#18209=CARTESIAN_POINT ( 'NONE',  ( 9.999999999999998224, 0.000000000000000000, -102.5000000000000000 ) ) ;
#18212=CARTESIAN_POINT ( 'NONE',  ( 7.644554776091147741E-16, 12.48450537969573659, -125.6562500020483810 ) ) ;
#18213=CARTESIAN_POINT ( 'NONE',  ( 7.070501591499377789E-16, 11.54700538379251284, -149.0000000040968189 ) ) ;
#18214=DIRECTION ( 'NONE',  ( -1.000000000000000000, 0.000000000000000000, 0.000000000000000000 ) ) ;
#18217=CARTESIAN_POINT ( 'NONE',  ( -10.81189881249999907, -6.242252689847864744, -172.9687500020484094 ) ) ;
#18219=CARTESIAN_POINT ( 'NONE',  ( -9.999999999999998224, 1.224646799147353059E-15, -166.2500000000000000 ) ) ;
#18220=CARTESIAN_POINT ( 'NONE',  ( 9.999999999999998224, 0.000000000000000000, -131.3750000040967905 ) ) ;
#18221=CARTESIAN_POINT ( 'NONE',  ( 10.81189881249999551, -6.242252689847874514, -72.15625000204836681 ) ) ;
#18222=CARTESIAN_POINT ( 'NONE',  ( -9.999999999999998224, 1.224646799147353059E-15, -40.62500000409677625 ) ) ;
#18223=CARTESIAN_POINT ( 'NONE',  ( 10.81189881249999551, -6.242252689847874514, -4.468750002048355263 ) ) ;
#18226=CARTESIAN_POINT ( 'NONE',  ( 10.00000000000012257, -5.773502691896188921, -162.6250000000000568 ) ) ;
#18228=ORIENTED_EDGE ( 'NONE', *, *, #11385, .F. ) ;
#18233=VERTEX_POINT ( 'NONE', #26357 ) ;
#18236=EDGE_LOOP ( 'NONE', ( #9014, #3664, #36344, #1807 ) ) ;
#18243=CARTESIAN_POINT ( 'NONE',  ( -2.121150477449813534E-15, -11.54700538379251284, -109.2500000040967763 ) ) ;
#18244=CARTESIAN_POINT ( 'NONE',  ( -2.121150477449813534E-15, -11.54700538379251284, -39.87499999999996447 ) ) ;
#18247=CARTESIAN_POINT ( 'NONE',  ( -10.81189881249999729, 6.242252689847871849, -164.2187500020483810 ) ) ;
#18248=CARTESIAN_POINT ( 'NONE',  ( -2.293366432827344421E-15, -12.48450537969573659, -178.7187500020484094 ) ) ;
#18250=CARTESIAN_POINT ( 'NONE',  ( 5.000000000000000000, 8.660254037844385522, -195.2500000000000000 ) ) ;
#18251=EDGE_CURVE ( 'NONE', #35515, #5023, #1722, .T. ) ;
#18257=CARTESIAN_POINT ( 'NONE',  ( 10.81189881249999907, 6.242252689847868297, -65.71875000204838102 ) ) ;
#18259=CARTESIAN_POINT ( 'NONE',  ( 5.405949406249992428, -9.363379034771808662, -69.28125000204838102 ) ) ;
#18261=CARTESIAN_POINT ( 'NONE',  ( -10.00000000000000000, -5.773502691896251982, -122.6250000000000000 ) ) ;
#18262=CARTESIAN_POINT ( 'NONE',  ( -10.81189881249999729, 1.324075727343319199E-15, -147.7812500020483810 ) ) ;
#18263=CARTESIAN_POINT ( 'NONE',  ( -10.81189881249999729, 6.242252689847871849, -162.9062500020484094 ) ) ;
#18266=CARTESIAN_POINT ( 'NONE',  ( 10.81189881249999729, 0.000000000000000000, -95.84375000204838102 ) ) ;
#18267=ORIENTED_EDGE ( 'NONE', *, *, #29898, .T. ) ;
#18269=CARTESIAN_POINT ( 'NONE',  ( 10.81189881249999907, 6.242252689847868297, -199.2187500020484094 ) ) ;
#18272=CARTESIAN_POINT ( 'NONE',  ( 10.81189881249999551, -6.242252689847874514, -93.15625000204838102 ) ) ;
#18274=CARTESIAN_POINT ( 'NONE',  ( 7.070501591499377789E-16, 11.54700538379251284, -68.00000000409679046 ) ) ;
#18276=CARTESIAN_POINT ( 'NONE',  ( 10.81189881249999551, -6.242252689847874514, -25.46875000204837391 ) ) ;
#18277=ORIENTED_EDGE ( 'NONE', *, *, #28344, .T. ) ;
#18279=CARTESIAN_POINT ( 'NONE',  ( 5.405949406249999534, 9.363379034771803333, -22.28125000204836326 ) ) ;
#18281=CARTESIAN_POINT ( 'NONE',  ( -9.999999999999998224, 1.224646799147353059E-15, -120.1250000040967905 ) ) ;
#18282=EDGE_CURVE ( 'NONE', #40199, #4599, #11910, .T. ) ;
#18284=( BOUNDED_CURVE ( )  B_SPLINE_CURVE ( 2, ( #38227, #1560, #22256, #35426, #8672, #2202, #5854 ),
 .UNSPECIFIED., .F., .F. ) 
 B_SPLINE_CURVE_WITH_KNOTS ( ( 3, 2, 2, 3 ),
 ( 0.2089552238805970630, 0.2101990049751244205, 0.2114427860696518058, 0.2126865671641791633 ),
 .UNSPECIFIED. ) 
 CURVE ( )  GEOMETRIC_REPRESENTATION_ITEM ( )  RATIONAL_B_SPLINE_CURVE ( ( 0.9999999999999940048, 0.8660254037844447028, 1.000000000000000000, 0.8660254037844387076, 1.000000000000000000, 0.8660254037844327124, 1.000000000000005995 ) ) 
 REPRESENTATION_ITEM ( '' )  );
#18285=CARTESIAN_POINT ( 'NONE',  ( -9.999999999999998224, 1.224646799147353059E-15, -109.2499999999999858 ) ) ;
#18301=CARTESIAN_POINT ( 'NONE',  ( 4.999999999999992006, -8.660254037844389075, -108.7499999999999858 ) ) ;
#18304=CARTESIAN_POINT ( 'NONE',  ( -4.999999999999996447, 8.660254037844387298, -156.3750000040967905 ) ) ;
#18305=CARTESIAN_POINT ( 'NONE',  ( 10.81189881249999729, 0.000000000000000000, -163.5312500020484094 ) ) ;
#18308=VECTOR ( 'NONE', #8650, 1000.000000000000000 ) ;
#18309=CARTESIAN_POINT ( 'NONE',  ( -2.293366432827344421E-15, -12.48450537969573659, -88.71875000204838102 ) ) ;
#18311=CARTESIAN_POINT ( 'NONE',  ( 5.405949406249999534, 9.363379034771803333, -194.5937500020484094 ) ) ;
#18312=CARTESIAN_POINT ( 'NONE',  ( 10.81189881249999907, 6.242252689847868297, -92.90625000204839523 ) ) ;
#18316=CARTESIAN_POINT ( 'NONE',  ( 10.81189881249999729, 0.000000000000000000, -175.5312500020483810 ) ) ;
#18317=CARTESIAN_POINT ( 'NONE',  ( -10.81189881249999729, 6.242252689847871849, -186.9062500020484094 ) ) ;
#18320=CARTESIAN_POINT ( 'NONE',  ( -10.00000000000000000, -5.773502691896251982, -165.0000000040967905 ) ) ;
#18322=CARTESIAN_POINT ( 'NONE',  ( 5.405949406249999534, 9.363379034771803333, -14.59375000204835082 ) ) ;
#18324=CARTESIAN_POINT ( 'NONE',  ( -2.293366432827344421E-15, -12.48450537969573659, -120.2187500020483952 ) ) ;
#18326=CARTESIAN_POINT ( 'NONE',  ( -10.81189881249999729, 6.242252689847871849, -17.40625000204837391 ) ) ;
#18329=CARTESIAN_POINT ( 'NONE',  ( -4.999999999999996447, 8.660254037844387298, -52.49999999999996447 ) ) ;
#18330=CARTESIAN_POINT ( 'NONE',  ( -2.293366432827344421E-15, -12.48450537969573659, -117.4062500020483952 ) ) ;
#18334=CARTESIAN_POINT ( 'NONE',  ( -9.999999999999998224, 5.773502691896259087, -94.75000000409677625 ) ) ;
#18337=CARTESIAN_POINT ( 'NONE',  ( -10.81189881249999907, -6.242252689847864744, -52.96875000204837391 ) ) ;
#18338=ORIENTED_EDGE ( 'NONE', *, *, #6321, .F. ) ;
#18343=CARTESIAN_POINT ( 'NONE',  ( 10.00000000000000000, 5.773502691896255534, -23.25000000409676915 ) ) ;
#18344=AXIS2_PLACEMENT_3D ( 'NONE', #9700, #7, #36038 ) ;
#18345=EDGE_CURVE ( 'NONE', #30831, #38366, #23519, .T. ) ;
#18349=DIRECTION ( 'NONE',  ( -0.000000000000000000, -0.000000000000000000, -1.000000000000000000 ) ) ;
#18354=ORIENTED_EDGE ( 'NONE', *, *, #35728, .T. ) ;
#18356=CARTESIAN_POINT ( 'NONE',  ( -4.999999999999996447, 8.660254037844387298, -171.0000000000000000 ) ) ;
#18358=CARTESIAN_POINT ( 'NONE',  ( -2.293366432827344421E-15, -12.48450537969573659, -192.4062500020484094 ) ) ;
#18362=CARTESIAN_POINT ( 'NONE',  ( -5.405949406250003975, -9.363379034771801557, -106.8437500020483810 ) ) ;
#18364=VECTOR ( 'NONE', #1447, 1000.000000000000000 ) ;
#18365=CARTESIAN_POINT ( 'NONE',  ( 10.81189881249999729, 0.000000000000000000, -118.5312500020483952 ) ) ;
#18367=CARTESIAN_POINT ( 'NONE',  ( -10.81189881249999729, 6.242252689847871849, -123.7187500020483952 ) ) ;
#18370=CARTESIAN_POINT ( 'NONE',  ( 4.999999999999992006, -8.660254037844389075, -149.2500000000000000 ) ) ;
#18371=CARTESIAN_POINT ( 'NONE',  ( -2.121150477449813534E-15, -11.54700538379251284, -9.874999999999966249 ) ) ;
#18374=CARTESIAN_POINT ( 'NONE',  ( -9.999999999999998224, 1.224646799147353059E-15, -190.6250000040967905 ) ) ;
#18376=CARTESIAN_POINT ( 'NONE',  ( -2.293366432827344421E-15, -12.48450537969573659, -34.71875000204835260 ) ) ;
#18378=CARTESIAN_POINT ( 'NONE',  ( 10.81189881249999907, 6.242252689847868297, -148.2187500020484094 ) ) ;
#18380=CARTESIAN_POINT ( 'NONE',  ( 5.000000000000000000, 8.660254037844385522, -145.7500000000000000 ) ) ;
#18381=CARTESIAN_POINT ( 'NONE',  ( 4.999999999999992006, -8.660254037844389075, -74.24999999999998579 ) ) ;
#18382=CARTESIAN_POINT ( 'NONE',  ( -5.405949406250003975, -9.363379034771801557, -140.0312500020484094 ) ) ;
#18384=ORIENTED_EDGE ( 'NONE', *, *, #24323, .T. ) ;
#18385=CARTESIAN_POINT ( 'NONE',  ( 9.999999999999996447, -5.773502691896262640, -115.0000000040967763 ) ) ;
#18387=CARTESIAN_POINT ( 'NONE',  ( -5.405949406249996869, 9.363379034771805109, -71.34375000204836681 ) ) ;
#18390=PRODUCT ( 'reaction body', 'reaction body', '', ( #14182 ) ) ;
#18392=CARTESIAN_POINT ( 'NONE',  ( -2.293366432827344421E-15, -12.48450537969573659, -43.90625000204837391 ) ) ;
#18396=CARTESIAN_POINT ( 'NONE',  ( 9.999999999999612754, 5.773502691896477579, -153.3749999999999716 ) ) ;
#18399=EDGE_CURVE ( 'NONE', #9953, #36081, #36744, .T. ) ;
#18405=CARTESIAN_POINT ( 'NONE',  ( -5.000000000000003553, -8.660254037844383745, -130.3750000040967905 ) ) ;
#18409=CARTESIAN_POINT ( 'NONE',  ( 10.81189881249999729, 0.000000000000000000, -130.3437500020484094 ) ) ;
#18410=CARTESIAN_POINT ( 'NONE',  ( -10.81189881249999907, -6.242252689847864744, -138.6562500020484094 ) ) ;
#18411=CARTESIAN_POINT ( 'NONE',  ( -10.81189881249999729, 6.242252689847871849, -150.7187500020483810 ) ) ;
#18412=CARTESIAN_POINT ( 'NONE',  ( 9.999999999999998224, 1.224646799147353059E-15, -99.99999999999998579 ) ) ;
#18414=CARTESIAN_POINT ( 'NONE',  ( -2.121150477449813534E-15, -11.54700538379251284, -174.8750000000000000 ) ) ;
#18418=CARTESIAN_POINT ( 'NONE',  ( -6.438708744581160381, -7.749506880439706258, -99.99999999999995737 ) ) ;
#18419=CARTESIAN_POINT ( 'NONE',  ( -2.293366432827344421E-15, -12.48450537969573659, -169.7187500020483810 ) ) ;
#18423=CARTESIAN_POINT ( 'NONE',  ( 5.405949406249992428, -9.363379034771808662, -45.28125000204838102 ) ) ;
#18425=CARTESIAN_POINT ( 'NONE',  ( -10.00000000000000000, -5.773502691896251982, -100.1249999999999858 ) ) ;
#18426=EDGE_CURVE ( 'NONE', #30416, #22978, #21143, .T. ) ;
#18427=ORIENTED_EDGE ( 'NONE', *, *, #41255, .F. ) ;
#18428=CARTESIAN_POINT ( 'NONE',  ( 5.405949406249999534, 9.363379034771803333, -128.7812500020483810 ) ) ;
#18429=CARTESIAN_POINT ( 'NONE',  ( -9.999999999999998224, 1.224646799147353059E-15, -150.1250000040967905 ) ) ;
#18432=ORIENTED_EDGE ( 'NONE', *, *, #6065, .T. ) ;
#18433=CARTESIAN_POINT ( 'NONE',  ( 5.405949406249999534, 9.363379034771803333, -173.5937500020484094 ) ) ;
#18436=CARTESIAN_POINT ( 'NONE',  ( -5.000000000000003553, -8.660254037844383745, -155.5000000000000000 ) ) ;
#18437=CARTESIAN_POINT ( 'NONE',  ( -2.293366432827344421E-15, -12.48450537969573659, -66.40625000204838102 ) ) ;
#18438=CARTESIAN_POINT ( 'NONE',  ( 4.999999999999992006, -8.660254037844389075, -43.12500000409677625 ) ) ;
#18439=CARTESIAN_POINT ( 'NONE',  ( -10.81189881249999729, 1.324075727343319199E-15, -0.5937500020483654772 ) ) ;
#18442=AXIS2_PLACEMENT_3D ( 'NONE', #9029, #42027, #31711 ) ;
#18448=CARTESIAN_POINT ( 'NONE',  ( -4.999999999999996447, 8.660254037844387298, -172.8750000040968189 ) ) ;
#18449=( BOUNDED_CURVE ( )  B_SPLINE_CURVE ( 2, ( #21744, #5345, #2122, #15252, #40504, #10949, #6198 ),
 .UNSPECIFIED., .F., .F. ) 
 B_SPLINE_CURVE_WITH_KNOTS ( ( 3, 2, 2, 3 ),
 ( 0.1940298507462686894, 0.1952736318407960470, 0.1965174129353234322, 0.1977611940298507898 ),
 .UNSPECIFIED. ) 
 CURVE ( )  GEOMETRIC_REPRESENTATION_ITEM ( )  RATIONAL_B_SPLINE_CURVE ( ( 0.9999999999999970024, 0.8660254037844417052, 1.000000000000000000, 0.8660254037844387076, 1.000000000000000000, 0.8660254037844327124, 1.000000000000005995 ) ) 
 REPRESENTATION_ITEM ( '' )  );
#18453=ORIENTED_EDGE ( 'NONE', *, *, #11974, .F. ) ;
#18456=( BOUNDED_CURVE ( )  B_SPLINE_CURVE ( 2, ( #39698, #41925, #28581, #32242, #35481, #16807, #13143 ),
 .UNSPECIFIED., .F., .F. ) 
 B_SPLINE_CURVE_WITH_KNOTS ( ( 3, 2, 2, 3 ),
 ( 0.4216417910447762818, 0.4228855721393036671, 0.4241293532338309413, 0.4253731343283583266 ),
 .UNSPECIFIED. ) 
 CURVE ( )  GEOMETRIC_REPRESENTATION_ITEM ( )  RATIONAL_B_SPLINE_CURVE ( ( 0.9999999999999820144, 0.8660254037844566932, 1.000000000000000000, 0.8660254037844387076, 1.000000000000000000, 0.8660254037844267172, 1.000000000000011990 ) ) 
 REPRESENTATION_ITEM ( '' )  );
#18461=CARTESIAN_POINT ( 'NONE',  ( 0.000000000000000000, 0.000000000000000000, -99.99999999999998579 ) ) ;
#18462=CARTESIAN_POINT ( 'NONE',  ( 9.999999999999996447, -5.773502691896262640, -38.12499999999997158 ) ) ;
#18465=CARTESIAN_POINT ( 'NONE',  ( 10.81189881249999907, 6.242252689847868297, -160.2187500020483810 ) ) ;
#18466=CARTESIAN_POINT ( 'NONE',  ( -10.81189881249999729, 1.324075727343319199E-15, -177.5937500020484094 ) ) ;
#18469=CARTESIAN_POINT ( 'NONE',  ( 9.999999999999998224, 0.000000000000000000, -144.5000000000000000 ) ) ;
#18470=CARTESIAN_POINT ( 'NONE',  ( 9.999999999999998224, 0.000000000000000000, -197.0000000000000000 ) ) ;
#18473=CONICAL_SURFACE ( 'NONE', #27441, 31.99999999999997158, 0.7853981633974447263 ) ;
#18476=CARTESIAN_POINT ( 'NONE',  ( -2.293366432827344421E-15, -12.48450537969573659, -64.90625000204838102 ) ) ;
#18478=CARTESIAN_POINT ( 'NONE',  ( -5.000000000000003553, -8.660254037844383745, -127.0000000000000000 ) ) ;
#18479=ORIENTED_EDGE ( 'NONE', *, *, #31528, .T. ) ;
#18480=CARTESIAN_POINT ( 'NONE',  ( 10.81189881249999551, -6.242252689847874514, -150.1562500020484094 ) ) ;
#18481=CARTESIAN_POINT ( 'NONE',  ( 5.405949406249999534, 9.363379034771803333, -166.2812500020484094 ) ) ;
#18484=CARTESIAN_POINT ( 'NONE',  ( 10.81189881249999551, -6.242252689847874514, -97.46875000204838102 ) ) ;
#18485=ORIENTED_EDGE ( 'NONE', *, *, #5390, .T. ) ;
#18487=CARTESIAN_POINT ( 'NONE',  ( -10.81189881249999907, -6.242252689847864744, -193.9687500020484094 ) ) ;
#18489=CARTESIAN_POINT ( 'NONE',  ( -2.138652185739045919, -10.15658843976767400, -179.9999999999999716 ) ) ;
#18491=CARTESIAN_POINT ( 'NONE',  ( 5.405949406249992428, -9.363379034771808662, -94.78125000204838102 ) ) ;
#18493=CARTESIAN_POINT ( 'NONE',  ( -5.000000000000003553, -8.660254037844383745, -70.37500000409677625 ) ) ;
#18494=FACE_OUTER_BOUND ( 'NONE', #39052, .T. ) ;
#18495=CARTESIAN_POINT ( 'NONE',  ( 10.81189881249999907, 6.242252689847868297, -23.71875000204837036 ) ) ;
#18498=CARTESIAN_POINT ( 'NONE',  ( -10.81189881249999729, 1.324075727343319199E-15, -20.28125000204836326 ) ) ;
#18500=CARTESIAN_POINT ( 'NONE',  ( -5.000000000000003553, -8.660254037844383745, -118.3750000040967905 ) ) ;
#18508=CARTESIAN_POINT ( 'NONE',  ( -4.999999999999996447, 8.660254037844387298, -169.8750000040967905 ) ) ;
#18512=ADVANCED_FACE ( 'NONE', ( #27199 ), #4534, .F. ) ;
#18520=CARTESIAN_POINT ( 'NONE',  ( 10.81189881249999729, 0.000000000000000000, -162.0312500020484094 ) ) ;
#18522=CARTESIAN_POINT ( 'NONE',  ( 4.999999999999992006, -8.660254037844389075, -172.1250000040968189 ) ) ;
#18524=CARTESIAN_POINT ( 'NONE',  ( 5.405949406249999534, 9.363379034771803333, -88.09375000204836681 ) ) ;
#18525=CARTESIAN_POINT ( 'NONE',  ( 10.81189881249999729, 0.000000000000000000, -191.8437500020484094 ) ) ;
#18526=CARTESIAN_POINT ( 'NONE',  ( 5.405949406249992428, -9.363379034771808662, -90.28125000204838102 ) ) ;
#18530=CARTESIAN_POINT ( 'NONE',  ( 5.405949406249992428, -9.363379034771808662, -172.7812500020484094 ) ) ;
#18531=CARTESIAN_POINT ( 'NONE',  ( 10.81189881249999729, 0.000000000000000000, -184.5312500020484094 ) ) ;
#18533=CARTESIAN_POINT ( 'NONE',  ( -9.999999999999998224, 5.773502691896259087, -162.2500000040967620 ) ) ;
#18535=CARTESIAN_POINT ( 'NONE',  ( 5.405949406249999534, 9.363379034771803333, -13.09375000204834905 ) ) ;
#18537=CARTESIAN_POINT ( 'NONE',  ( 10.81189881249999907, 6.242252689847868297, -122.7187500020483810 ) ) ;
#18539=CARTESIAN_POINT ( 'NONE',  ( 5.405949406249992428, -9.363379034771808662, -24.28125000204836681 ) ) ;
#18541=VECTOR ( 'NONE', #9975, 1000.000000000000000 ) ;
#18542=( BOUNDED_CURVE ( )  B_SPLINE_CURVE ( 2, ( #11551, #37250, #24760, #4888, #40266, #37689, #18035 ),
 .UNSPECIFIED., .F., .F. ) 
 B_SPLINE_CURVE_WITH_KNOTS ( ( 3, 2, 2, 3 ),
 ( 0.1529850746268656692, 0.1542288557213930267, 0.1554726368159203842, 0.1567164179104477695 ),
 .UNSPECIFIED. ) 
 CURVE ( )  GEOMETRIC_REPRESENTATION_ITEM ( )  RATIONAL_B_SPLINE_CURVE ( ( 1.000000000000000000, 0.8660254037844387076, 1.000000000000000000, 0.8660254037844387076, 1.000000000000000000, 0.8660254037844387076, 1.000000000000000000 ) ) 
 REPRESENTATION_ITEM ( '' )  );
#18544=CARTESIAN_POINT ( 'NONE',  ( -5.000000000000003553, -8.660254037844383745, -50.49999999999998579 ) ) ;
#18545=CARTESIAN_POINT ( 'NONE',  ( -2.293366432827344421E-15, -12.48450537969573659, -115.9062500020483810 ) ) ;
#18548=CARTESIAN_POINT ( 'NONE',  ( -10.00000000000000000, -5.773502691896251982, -90.00000000409677625 ) ) ;
#18551=CARTESIAN_POINT ( 'NONE',  ( 7.644554776091147741E-16, 12.48450537969573659, -51.96875000204836681 ) ) ;
#18554=VECTOR ( 'NONE', #11358, 1000.000000000000000 ) ;
#18557=CARTESIAN_POINT ( 'NONE',  ( 9.999999999999998224, 0.000000000000000000, -18.87500000409675494 ) ) ;
#18563=CARTESIAN_POINT ( 'NONE',  ( 9.999999999999998224, 1.224646799147353059E-15, -99.99999999999998579 ) ) ;
#18571=ORIENTED_EDGE ( 'NONE', *, *, #5126, .T. ) ;
#18572=CARTESIAN_POINT ( 'NONE',  ( 5.000000000000000000, 8.660254037844385522, -175.7500000000000284 ) ) ;
#18576=CARTESIAN_POINT ( 'NONE',  ( 5.405949406249992428, -9.363379034771808662, -184.7812500020484094 ) ) ;
#18579=CARTESIAN_POINT ( 'NONE',  ( -10.81189881249999729, 6.242252689847871849, -107.2187500020483810 ) ) ;
#18581=CARTESIAN_POINT ( 'NONE',  ( -10.81189881249999729, 6.242252689847871849, -119.4062500020483952 ) ) ;
#18583=CARTESIAN_POINT ( 'NONE',  ( -10.81189881249999729, 1.324075727343319199E-15, -122.0937500020483952 ) ) ;
#18587=CARTESIAN_POINT ( 'NONE',  ( -9.999999999999998224, 5.773502691896259087, -151.3750000000000000 ) ) ;
#18588=CARTESIAN_POINT ( 'NONE',  ( 5.000000000000000000, 8.660254037844385522, -13.74999999999995737 ) ) ;
#18592=CARTESIAN_POINT ( 'NONE',  ( -10.00000000000000000, -5.773502691896251982, -184.5000000040968189 ) ) ;
#18594=CARTESIAN_POINT ( 'NONE',  ( -5.405949406250003975, -9.363379034771801557, -37.84375000204837391 ) ) ;
#18595=CARTESIAN_POINT ( 'NONE',  ( -2.293366432827344421E-15, -12.48450537969573659, -142.7187500020484094 ) ) ;
#18597=CARTESIAN_POINT ( 'NONE',  ( -9.999999999999998224, 1.224646799147353059E-15, -136.2499999999999716 ) ) ;
#18598=CARTESIAN_POINT ( 'NONE',  ( -4.999999999999996447, 8.660254037844387298, -76.49999999999998579 ) ) ;
#18599=CARTESIAN_POINT ( 'NONE',  ( -10.81189881249999729, 1.324075727343319199E-15, -143.2812500020483810 ) ) ;
#18602=CARTESIAN_POINT ( 'NONE',  ( -4.999999999999996447, 8.660254037844387298, -117.3750000040967905 ) ) ;
#18604=CARTESIAN_POINT ( 'NONE',  ( 10.81189881249999907, 6.242252689847868297, -77.71875000204838102 ) ) ;
#18608=CARTESIAN_POINT ( 'NONE',  ( -5.405949406249996869, 9.363379034771805109, -46.03125000204838813 ) ) ;
#18623=CARTESIAN_POINT ( 'NONE',  ( 9.999999999999998224, 1.224646799147353059E-15, -99.99999999999998579 ) ) ;
#18624=CARTESIAN_POINT ( 'NONE',  ( -10.81189881249999907, -6.242252689847864744, -132.4687500020483810 ) ) ;
#18625=CARTESIAN_POINT ( 'NONE',  ( 7.644554776091147741E-16, 12.48450537969573659, -139.1562500020483810 ) ) ;
#18626=CARTESIAN_POINT ( 'NONE',  ( -10.81189881249999729, 6.242252689847871849, -144.7187500020484094 ) ) ;
#18629=CARTESIAN_POINT ( 'NONE',  ( 9.999999999999998224, 0.000000000000000000, -171.5000000000000000 ) ) ;
#18634=CARTESIAN_POINT ( 'NONE',  ( -10.00000000000076916, 5.773502691895813221, -133.3749999999999716 ) ) ;
#18635=CARTESIAN_POINT ( 'NONE',  ( 10.81189881249999551, -6.242252689847874514, -173.9687500020484094 ) ) ;
#18639=CARTESIAN_POINT ( 'NONE',  ( 7.644554776091147741E-16, 12.48450537969573659, -34.15625000204835970 ) ) ;
#18641=CARTESIAN_POINT ( 'NONE',  ( -9.999999999999998224, 1.224646799147353059E-15, -103.2500000000000000 ) ) ;
#18643=CARTESIAN_POINT ( 'NONE',  ( 10.81189881249999729, 6.242252689847867408, -125.9062500020483810 ) ) ;
#18644=CARTESIAN_POINT ( 'NONE',  ( 4.999999999999992006, -8.660254037844389075, -143.6250000040967905 ) ) ;
#18647=VERTEX_POINT ( 'NONE', #15718 ) ;
#18650=CARTESIAN_POINT ( 'NONE',  ( 7.644554776091147741E-16, 12.48450537969573659, -68.65625000204839523 ) ) ;
#18651=DIRECTION ( 'NONE',  ( -1.000000000000000000, 0.000000000000000000, 0.000000000000000000 ) ) ;
#18655=ORIENTED_EDGE ( 'NONE', *, *, #23971, .T. ) ;
#18656=FACE_OUTER_BOUND ( 'NONE', #35813, .T. ) ;
#18663=CARTESIAN_POINT ( 'NONE',  ( 10.00000000000051159, -5.773502691895965988, -178.0000000040967336 ) ) ;
#18670=EDGE_LOOP ( 'NONE', ( #41374, #24067, #6710, #35722 ) ) ;
#18672=CARTESIAN_POINT ( 'NONE',  ( 4.999999999999992006, -8.660254037844389075, -33.74999999999997158 ) ) ;
#18675=CARTESIAN_POINT ( 'NONE',  ( 5.405949406249999534, 9.363379034771803333, -161.5937500020484094 ) ) ;
#18676=CARTESIAN_POINT ( 'NONE',  ( -2.293366432827344421E-15, -12.48450537969573659, -174.2187500020483810 ) ) ;
#18678=CARTESIAN_POINT ( 'NONE',  ( 0.000000000000000000, 0.000000000000000000, -99.99999999999998579 ) ) ;
#18679=CARTESIAN_POINT ( 'NONE',  ( 9.999999999999998224, 0.000000000000000000, -195.5000000000000000 ) ) ;
#18684=CARTESIAN_POINT ( 'NONE',  ( 10.81189881249999551, -6.242252689847874514, -69.15625000204839523 ) ) ;
#18686=CARTESIAN_POINT ( 'NONE',  ( 10.00000000000000000, 5.773502691896255534, -123.3749999999999858 ) ) ;
#18687=ADVANCED_FACE ( 'NONE', ( #35606 ), #31739, .F. ) ;
#18688=AXIS2_PLACEMENT_3D ( 'NONE', #40561, #11430, #24419 ) ;
#18689=ORIENTED_EDGE ( 'NONE', *, *, #38167, .F. ) ;
#18690=CARTESIAN_POINT ( 'NONE',  ( 10.81189881249999551, -6.242252689847874514, -151.6562500020484094 ) ) ;
#18691=CARTESIAN_POINT ( 'NONE',  ( -2.293366432827344421E-15, -12.48450537969573659, -166.9062500020483810 ) ) ;
#18694=CARTESIAN_POINT ( 'NONE',  ( 9.999999999999998224, 0.000000000000000000, -102.8750000040967763 ) ) ;
#18695=CARTESIAN_POINT ( 'NONE',  ( 5.405949406249992428, -9.363379034771808662, -94.59375000204838102 ) ) ;
#18698=CARTESIAN_POINT ( 'NONE',  ( 10.81189881249999551, -6.242252689847874514, -193.4687500020484094 ) ) ;
#18700=CARTESIAN_POINT ( 'NONE',  ( -6.604780291884596366, -7.711322195483102604, -180.0000000000000000 ) ) ;
#18702=CARTESIAN_POINT ( 'NONE',  ( -10.81189881249999729, 1.324075727343319199E-15, -95.28125000204838102 ) ) ;
#18705=CARTESIAN_POINT ( 'NONE',  ( -9.999999999999998224, 5.773502691896259087, -64.75000000409677625 ) ) ;
#18707=CARTESIAN_POINT ( 'NONE',  ( -5.405949406250003975, -9.363379034771801557, -28.84375000204836326 ) ) ;
#18710=VECTOR ( 'NONE', #19461, 1000.000000000000000 ) ;
#18711=CARTESIAN_POINT ( 'NONE',  ( 10.81189881249999729, 0.000000000000000000, -16.53125000204835970 ) ) ;
#18720=EDGE_CURVE ( 'NONE', #19924, #13418, #38194, .T. ) ;
#18721=CARTESIAN_POINT ( 'NONE',  ( -8.660253955908514101, -5.000000141917089636, -180.0000000000000284 ) ) ;
#18722=VERTEX_POINT ( 'NONE', #35815 ) ;
#18723=ORIENTED_EDGE ( 'NONE', *, *, #36718, .F. ) ;
#18728=CARTESIAN_POINT ( 'NONE',  ( -2.121150477449813534E-15, -11.54700538379251284, -173.3750000000000000 ) ) ;
#18730=CARTESIAN_POINT ( 'NONE',  ( 9.999999999999742428, 5.773502691896404748, -124.8749999999999858 ) ) ;
#18731=CARTESIAN_POINT ( 'NONE',  ( -10.81189881249999729, 1.324075727343319199E-15, -161.2812500020484094 ) ) ;
#18733=VECTOR ( 'NONE', #3413, 1000.000000000000000 ) ;
#18737=CARTESIAN_POINT ( 'NONE',  ( 7.644554776091147741E-16, 12.48450537969573659, -87.96875000204838102 ) ) ;
#18738=CARTESIAN_POINT ( 'NONE',  ( -10.81189881249999907, -6.242252689847864744, -190.9687500020484379 ) ) ;
#18739=CARTESIAN_POINT ( 'NONE',  ( 10.81189881249999551, -6.242252689847874514, -94.65625000204838102 ) ) ;
#18743=CARTESIAN_POINT ( 'NONE',  ( -5.405949406250003975, -9.363379034771801557, -171.5312500020484094 ) ) ;
#18744=CARTESIAN_POINT ( 'NONE',  ( 5.405949406249992428, -9.363379034771808662, -190.7812500020484094 ) ) ;
#18746=CARTESIAN_POINT ( 'NONE',  ( -4.999999999999996447, 8.660254037844387298, -165.3750000040967905 ) ) ;
#18748=CARTESIAN_POINT ( 'NONE',  ( -10.81189881249999907, -6.242252689847864744, -12.46875000204836326 ) ) ;
#18750=CARTESIAN_POINT ( 'NONE',  ( -10.81189881249999729, 1.324075727343319199E-15, -123.5937500020483952 ) ) ;
#18753=CARTESIAN_POINT ( 'NONE',  ( 10.81189881249999907, 6.242252689847868297, -23.90625000204838102 ) ) ;
#18755=CARTESIAN_POINT ( 'NONE',  ( -10.00000000000012434, 5.773502691896184480, -157.7500000040967905 ) ) ;
#18756=CARTESIAN_POINT ( 'NONE',  ( 5.405949406249992428, -9.363379034771808662, -118.7812500020483952 ) ) ;
#18759=VECTOR ( 'NONE', #4935, 1000.000000000000000 ) ;
#18760=CARTESIAN_POINT ( 'NONE',  ( -5.000000000000003553, -8.660254037844383745, -88.37500000409677625 ) ) ;
#18761=DIRECTION ( 'NONE',  ( -0.000000000000000000, -0.000000000000000000, -1.000000000000000000 ) ) ;
#18763=CARTESIAN_POINT ( 'NONE',  ( -10.81189881249999729, 1.324075727343319199E-15, -51.59375000204835260 ) ) ;
#18768=CARTESIAN_POINT ( 'NONE',  ( -9.999999999999998224, 5.773502691896259087, -19.75000000409676915 ) ) ;
#18773=CARTESIAN_POINT ( 'NONE',  ( -2.121150477449813534E-15, -11.54700538379251284, -152.3749999999999716 ) ) ;
#18774=CARTESIAN_POINT ( 'NONE',  ( -4.999999999999996447, 8.660254037844387298, -142.8750000040967905 ) ) ;
#18775=ORIENTED_EDGE ( 'NONE', *, *, #9727, .F. ) ;
#18782=CARTESIAN_POINT ( 'NONE',  ( 9.999999999999998224, 0.000000000000000000, -171.5000000000000000 ) ) ;
#18784=CARTESIAN_POINT ( 'NONE',  ( 7.644554776091147741E-16, 12.48450537969573659, -188.6562500020484379 ) ) ;
#18789=CARTESIAN_POINT ( 'NONE',  ( -10.81189881249999729, 6.242252689847871849, -111.7187500020483810 ) ) ;
#18791=CARTESIAN_POINT ( 'NONE',  ( 5.405949406249999534, 9.363379034771803333, -115.2812500020483952 ) ) ;
#18793=CARTESIAN_POINT ( 'NONE',  ( 7.644554776091147741E-16, 12.48450537969573659, -120.9687500020483952 ) ) ;
#18796=CARTESIAN_POINT ( 'NONE',  ( -5.000000000000003553, -8.660254037844383745, -140.5000000000000000 ) ) ;
#18797=CARTESIAN_POINT ( 'NONE',  ( 7.070501591499377789E-16, 11.54700538379251284, -15.12499999999997158 ) ) ;
#18801=CARTESIAN_POINT ( 'NONE',  ( 10.00000000000000000, 5.773502691896255534, -186.7500000040967905 ) ) ;
#18803=CARTESIAN_POINT ( 'NONE',  ( -2.293366432827344421E-15, -12.48450537969573659, -36.21875000204835970 ) ) ;
#18805=CARTESIAN_POINT ( 'NONE',  ( -10.81189881249999729, 1.324075727343319199E-15, -144.5937500020483810 ) ) ;
#18809=CARTESIAN_POINT ( 'NONE',  ( 7.070501591499376803E-16, 11.54700538379251284, -145.6250000000000000 ) ) ;
#18811=CARTESIAN_POINT ( 'NONE',  ( -9.999999999999998224, 5.773502691896259087, -74.87499999999997158 ) ) ;
#18812=CARTESIAN_POINT ( 'NONE',  ( -2.293366432827344421E-15, -12.48450537969573659, -136.9062500020484094 ) ) ;
#18814=EDGE_CURVE ( 'NONE', #28805, #16041, #3102, .T. ) ;
#18817=CARTESIAN_POINT ( 'NONE',  ( -9.999999999999998224, 1.224646799147353059E-15, -112.6250000040967763 ) ) ;
#18819=CARTESIAN_POINT ( 'NONE',  ( 5.405949406249999534, 9.363379034771803333, -74.59375000204838102 ) ) ;
#18823=CARTESIAN_POINT ( 'NONE',  ( -2.121150477449813534E-15, -11.54700538379251284, -157.2500000040968189 ) ) ;
#18824=CARTESIAN_POINT ( 'NONE',  ( 10.81189881249999907, 6.242252689847868297, -34.40625000204835970 ) ) ;
#18828=CARTESIAN_POINT ( 'NONE',  ( 9.999999999999998224, 0.000000000000000000, -153.5000000000000000 ) ) ;
#18832=EDGE_CURVE ( 'NONE', #20303, #29817, #41837, .T. ) ;
#18837=( BOUNDED_CURVE ( )  B_SPLINE_CURVE ( 2, ( #9600, #19733, #19943, #26430, #36562, #29890, #26854 ),
 .UNSPECIFIED., .F., .F. ) 
 B_SPLINE_CURVE_WITH_KNOTS ( ( 3, 2, 2, 3 ),
 ( 0.4552238805970150737, 0.4564676616915424590, 0.4577114427860698442, 0.4589552238805971740 ),
 .UNSPECIFIED. ) 
 CURVE ( )  GEOMETRIC_REPRESENTATION_ITEM ( )  RATIONAL_B_SPLINE_CURVE ( ( 0.9999999999999820144, 0.8660254037844566932, 1.000000000000000000, 0.8660254037844387076, 1.000000000000000000, 0.8660254037844207220, 1.000000000000017986 ) ) 
 REPRESENTATION_ITEM ( '' )  );
#18843=EDGE_CURVE ( 'NONE', #12639, #6263, #35376, .T. ) ;
#18845=CARTESIAN_POINT ( 'NONE',  ( -5.405949406249996869, 9.363379034771805109, -132.8437500020484094 ) ) ;
#18846=CARTESIAN_POINT ( 'NONE',  ( -10.81189881249999729, 1.324075727343319199E-15, -140.2812500020483810 ) ) ;
#18847=CARTESIAN_POINT ( 'NONE',  ( 9.999999999999479527, 5.773502691896553074, -144.3750000000000000 ) ) ;
#18848=CARTESIAN_POINT ( 'NONE',  ( 10.81189881249999551, -6.242252689847874514, -145.4687500020484094 ) ) ;
#18852=CARTESIAN_POINT ( 'NONE',  ( -2.121150477449813534E-15, -11.54700538379251284, -168.8750000000000000 ) ) ;
#18857=CARTESIAN_POINT ( 'NONE',  ( -5.405949406250003975, -9.363379034771801557, -172.8437500020484094 ) ) ;
#18861=CARTESIAN_POINT ( 'NONE',  ( -2.293366432827344421E-15, -12.48450537969573659, -33.40625000204835970 ) ) ;
#18863=CARTESIAN_POINT ( 'NONE',  ( -10.00000000000000000, -5.773502691896251982, -97.12500000000000000 ) ) ;
#18866=CARTESIAN_POINT ( 'NONE',  ( 5.405949406249992428, -9.363379034771808662, -121.7812500020483952 ) ) ;
#18867=CARTESIAN_POINT ( 'NONE',  ( -4.999999999999996447, 8.660254037844387298, -138.3750000040967905 ) ) ;
#18871=FACE_OUTER_BOUND ( 'NONE', #20980, .T. ) ;
#18872=CARTESIAN_POINT ( 'NONE',  ( -10.81189881249999907, -6.242252689847864744, -60.65625000204838813 ) ) ;
#18875=CARTESIAN_POINT ( 'NONE',  ( -9.999999999999998224, 1.224646799147353059E-15, -163.2500000000000000 ) ) ;
#18882=ORIENTED_EDGE ( 'NONE', *, *, #27828, .T. ) ;
#18893=CARTESIAN_POINT ( 'NONE',  ( -4.999999999999996447, 8.660254037844387298, -35.99999999999997868 ) ) ;
#18896=CARTESIAN_POINT ( 'NONE',  ( -10.81189881249999729, 6.242252689847871849, -156.7187500020483810 ) ) ;
#18897=CARTESIAN_POINT ( 'NONE',  ( -10.81189881249999729, 1.324075727343319199E-15, -171.5937500020484094 ) ) ;
#18899=CARTESIAN_POINT ( 'NONE',  ( -9.999999999999998224, 1.224646799147353059E-15, -131.7499999999999716 ) ) ;
#18900=CARTESIAN_POINT ( 'NONE',  ( 4.999999999999992006, -8.660254037844389075, -192.7500000000000000 ) ) ;
#18905=CARTESIAN_POINT ( 'NONE',  ( 5.405949406249999534, 9.363379034771803333, -61.28125000204837391 ) ) ;
#18907=CARTESIAN_POINT ( 'NONE',  ( -2.121150477449813534E-15, -11.54700538379251284, -123.8749999999999858 ) ) ;
#18909=CARTESIAN_POINT ( 'NONE',  ( -10.81189881249999729, 6.242252689847871849, -138.9062500020484094 ) ) ;
#18910=CARTESIAN_POINT ( 'NONE',  ( -10.81189881249999729, 1.324075727343319199E-15, -159.7812500020484094 ) ) ;
#18912=CARTESIAN_POINT ( 'NONE',  ( 9.999999999999998224, 0.000000000000000000, -105.4999999999999858 ) ) ;
#18913=CARTESIAN_POINT ( 'NONE',  ( -10.81189881249999729, 6.242252689847871849, -86.21875000204838102 ) ) ;
#18916=CARTESIAN_POINT ( 'NONE',  ( 10.81189881249999551, -6.242252689847874514, -196.4687500020484094 ) ) ;
#18918=CARTESIAN_POINT ( 'NONE',  ( 9.999999999999998224, 0.000000000000000000, -165.5000000000000000 ) ) ;
#18919=CARTESIAN_POINT ( 'NONE',  ( -5.000000000000003553, -8.660254037844383745, -118.0000000000000000 ) ) ;
#18920=CARTESIAN_POINT ( 'NONE',  ( -5.405949406249996869, 9.363379034771805109, -92.53125000204838102 ) ) ;
#18922=CARTESIAN_POINT ( 'NONE',  ( -10.00000000000000000, -5.773502691896251982, -72.00000000409674783 ) ) ;
#18924=CARTESIAN_POINT ( 'NONE',  ( 5.405949406249992428, -9.363379034771808662, -22.59375000204835615 ) ) ;
#18925=EDGE_LOOP ( 'NONE', ( #5604, #15408, #20995, #10321 ) ) ;
#18927=EDGE_CURVE ( 'NONE', #4329, #17318, #27927, .T. ) ;
#18928=CARTESIAN_POINT ( 'NONE',  ( 7.644554776091147741E-16, 12.48450537969573659, -20.65625000204837747 ) ) ;
#18930=CARTESIAN_POINT ( 'NONE',  ( 9.999999999999998224, 0.000000000000000000, -137.3750000040967905 ) ) ;
#18938=VERTEX_POINT ( 'NONE', #39664 ) ;
#18943=CARTESIAN_POINT ( 'NONE',  ( 4.999999999999992006, -8.660254037844389075, -173.2500000000000284 ) ) ;
#18946=CARTESIAN_POINT ( 'NONE',  ( -10.00000000000076916, 5.773502691895813221, -128.8749999999999716 ) ) ;
#18947=CARTESIAN_POINT ( 'NONE',  ( -2.293366432827344421E-15, -12.48450537969573659, -156.4062500020483810 ) ) ;
#18951=CARTESIAN_POINT ( 'NONE',  ( -10.81189881249999907, -6.242252689847864744, -73.96875000204836681 ) ) ;
#18952=CARTESIAN_POINT ( 'NONE',  ( -2.293366432827344421E-15, -12.48450537969573659, -81.40625000204838102 ) ) ;
#18954=( BOUNDED_CURVE ( )  B_SPLINE_CURVE ( 2, ( #13547, #4282, #23933, #13334, #10530, #7097, #20249 ),
 .UNSPECIFIED., .F., .F. ) 
 B_SPLINE_CURVE_WITH_KNOTS ( ( 3, 2, 2, 3 ),
 ( 0.2126865671641791633, 0.2139303482587065208, 0.2151741293532339061, 0.2164179104477612636 ),
 .UNSPECIFIED. ) 
 CURVE ( )  GEOMETRIC_REPRESENTATION_ITEM ( )  RATIONAL_B_SPLINE_CURVE ( ( 0.9999999999999940048, 0.8660254037844447028, 1.000000000000000000, 0.8660254037844387076, 1.000000000000000000, 0.8660254037844297148, 1.000000000000008882 ) ) 
 REPRESENTATION_ITEM ( '' )  );
#18956=CARTESIAN_POINT ( 'NONE',  ( 5.405949406249992428, -9.363379034771808662, -171.2812500020484094 ) ) ;
#18957=CARTESIAN_POINT ( 'NONE',  ( -5.405949406249996869, 9.363379034771805109, -185.5312500020484094 ) ) ;
#18959=CARTESIAN_POINT ( 'NONE',  ( -5.000000000000003553, -8.660254037844383745, -164.8750000040967905 ) ) ;
#18961=CARTESIAN_POINT ( 'NONE',  ( -10.81189881249999729, 6.242252689847871849, -17.21875000204836681 ) ) ;
#18963=CARTESIAN_POINT ( 'NONE',  ( 10.81189881249999551, -6.242252689847874514, -118.4687500020483810 ) ) ;
#18965=CARTESIAN_POINT ( 'NONE',  ( 5.405949406249992428, -9.363379034771808662, -22.78125000204836326 ) ) ;
#18968=CARTESIAN_POINT ( 'NONE',  ( -2.293366432827344421E-15, -12.48450537969573659, -112.9062500020483952 ) ) ;
#18970=EDGE_LOOP ( 'NONE', ( #21841, #26210, #30785, #14501 ) ) ;
#18973=CARTESIAN_POINT ( 'NONE',  ( -5.000000000000003553, -8.660254037844383745, -89.87500000409677625 ) ) ;
#18976=CARTESIAN_POINT ( 'NONE',  ( 5.405949406249992428, -9.363379034771808662, -48.09375000204838102 ) ) ;
#18981=CARTESIAN_POINT ( 'NONE',  ( 9.999999999999998224, 0.000000000000000000, -20.37500000409675494 ) ) ;
#18987=EDGE_LOOP ( 'NONE', ( #26449, #9798, #24801, #21909, #30622 ) ) ;
#18998=CARTESIAN_POINT ( 'NONE',  ( -10.81189881249999907, -6.242252689847864744, -177.6562500020484094 ) ) ;
#19002=CARTESIAN_POINT ( 'NONE',  ( 5.405949406249999534, 9.363379034771803333, -106.0937500020483810 ) ) ;
#19003=CARTESIAN_POINT ( 'NONE',  ( 9.999999999999998224, 0.000000000000000000, -143.0000000000000000 ) ) ;
#19004=CARTESIAN_POINT ( 'NONE',  ( 5.405949406249999534, 9.363379034771803333, -116.7812500020483952 ) ) ;
#19006=CARTESIAN_POINT ( 'NONE',  ( -5.405949406249996869, 9.363379034771805109, -119.3437500020483810 ) ) ;
#19009=CARTESIAN_POINT ( 'NONE',  ( 5.000000000000000000, 8.660254037844385522, -136.7499999999999716 ) ) ;
#19010=CARTESIAN_POINT ( 'NONE',  ( -4.999999999999996447, 8.660254037844387298, -14.99999999999995737 ) ) ;
#19013=CARTESIAN_POINT ( 'NONE',  ( -2.121150477449813534E-15, -11.54700538379251284, -191.7500000040967905 ) ) ;
#19015=CARTESIAN_POINT ( 'NONE',  ( 10.81189881249999907, 6.242252689847868297, -40.21875000204835970 ) ) ;
#19016=CARTESIAN_POINT ( 'NONE',  ( -9.999999999999998224, 1.224646799147353059E-15, -116.7499999999999858 ) ) ;
#19017=CARTESIAN_POINT ( 'NONE',  ( 5.405949406249999534, 9.363379034771803333, -148.0937500020483810 ) ) ;
#19019=CARTESIAN_POINT ( 'NONE',  ( -5.000000000000003553, -8.660254037844383745, -101.8750000040967905 ) ) ;
#19020=CARTESIAN_POINT ( 'NONE',  ( -4.999999999999996447, 8.660254037844387298, -70.49999999999998579 ) ) ;
#19021=CARTESIAN_POINT ( 'NONE',  ( 5.405949406249992428, -9.363379034771808662, -139.7812500020483810 ) ) ;
#19026=CARTESIAN_POINT ( 'NONE',  ( 7.070501591499377789E-16, 11.54700538379251284, -119.0000000040967763 ) ) ;
#19028=CARTESIAN_POINT ( 'NONE',  ( -10.81189881249999729, 1.324075727343319199E-15, -71.09375000204836681 ) ) ;
#19033=CARTESIAN_POINT ( 'NONE',  ( 9.999999999999994671, -5.773502691896262640, -131.5000000040967905 ) ) ;
#19034=CARTESIAN_POINT ( 'NONE',  ( 7.644554776091147741E-16, 12.48450537969573659, -40.15625000204836681 ) ) ;
#19039=ORIENTED_EDGE ( 'NONE', *, *, #11302, .F. ) ;
#19041=EDGE_CURVE ( 'NONE', #23457, #270, #20473, .T. ) ;
#19052=CARTESIAN_POINT ( 'NONE',  ( 35.00000000000000711, 4.286263797015737285E-15, -169.9999999999999716 ) ) ;
#19053=CARTESIAN_POINT ( 'NONE',  ( -5.405949406250003975, -9.363379034771801557, -132.3437500020484094 ) ) ;
#19054=CARTESIAN_POINT ( 'NONE',  ( 10.81189881249999551, -6.242252689847874514, -144.1562500020484094 ) ) ;
#19056=CARTESIAN_POINT ( 'NONE',  ( -10.81189881249999729, 6.242252689847871849, -146.2187500020484094 ) ) ;
#19057=CARTESIAN_POINT ( 'NONE',  ( -4.999999999999996447, 8.660254037844387298, -127.5000000000000000 ) ) ;
#19059=CARTESIAN_POINT ( 'NONE',  ( 9.999999999999996447, -5.773502691896262640, -164.1249999999999716 ) ) ;
#19063=CARTESIAN_POINT ( 'NONE',  ( 10.81189881249999907, 6.242252689847868297, -58.21875000204838102 ) ) ;
#19065=CARTESIAN_POINT ( 'NONE',  ( -5.405949406249996869, 9.363379034771805109, -170.3437500020484094 ) ) ;
#19070=CARTESIAN_POINT ( 'NONE',  ( -2.121150477449813534E-15, -11.54700538379251284, -99.87500000000000000 ) ) ;
#19072=CARTESIAN_POINT ( 'NONE',  ( 5.405949406249992428, -9.363379034771808662, -118.7812500020483952 ) ) ;
#19073=CARTESIAN_POINT ( 'NONE',  ( -5.000000000000003553, -8.660254037844383745, -139.3750000040968189 ) ) ;
#19077=EDGE_CURVE ( 'NONE', #1644, #25640, #29330, .T. ) ;
#19079=CARTESIAN_POINT ( 'NONE',  ( -5.405949406249996869, 9.363379034771805109, -62.53125000204837391 ) ) ;
#19101=FACE_OUTER_BOUND ( 'NONE', #41536, .T. ) ;
#19102=CARTESIAN_POINT ( 'NONE',  ( -4.999999999999996447, 8.660254037844387298, -26.99999999999996803 ) ) ;
#19105=CARTESIAN_POINT ( 'NONE',  ( -10.81189881249999729, 1.324075727343319199E-15, -159.5937500020484094 ) ) ;
#19106=CARTESIAN_POINT ( 'NONE',  ( 5.405949406249999534, 9.363379034771803333, -170.5937500020484094 ) ) ;
#19107=CYLINDRICAL_SURFACE ( 'NONE', #5427, 9.999999999999998224 ) ;
#19109=CARTESIAN_POINT ( 'NONE',  ( -9.999999999999998224, 5.773502691896259087, -184.3750000000000000 ) ) ;
#19115=CARTESIAN_POINT ( 'NONE',  ( -2.293366432827344421E-15, -12.48450537969573659, -57.40625000204838102 ) ) ;
#19117=CARTESIAN_POINT ( 'NONE',  ( -4.999999999999996447, 8.660254037844387298, -121.5000000000000000 ) ) ;
#19120=CARTESIAN_POINT ( 'NONE',  ( -10.81189881249999729, 6.242252689847871849, -146.4062500020484094 ) ) ;
#19121=CARTESIAN_POINT ( 'NONE',  ( -2.293366432827344421E-15, -12.48450537969573659, -156.4062500020483810 ) ) ;
#19124=CARTESIAN_POINT ( 'NONE',  ( -5.405949406249996869, 9.363379034771805109, -92.34375000204838102 ) ) ;
#19127=CARTESIAN_POINT ( 'NONE',  ( 5.405949406249992428, -9.363379034771808662, -184.5937500020483810 ) ) ;
#19130=CARTESIAN_POINT ( 'NONE',  ( -4.999999999999996447, 8.660254037844387298, -139.8750000040968189 ) ) ;
#19131=CARTESIAN_POINT ( 'NONE',  ( -10.81189881249999729, 6.242252689847871849, -84.90625000204838102 ) ) ;
#19133=CARTESIAN_POINT ( 'NONE',  ( 7.070501591499377789E-16, 11.54700538379251284, -57.50000000409677625 ) ) ;
#19134=CARTESIAN_POINT ( 'NONE',  ( 10.81189881249999729, 0.000000000000000000, -14.84375000204835082 ) ) ;
#19137=CARTESIAN_POINT ( 'NONE',  ( -5.405949406249996869, 9.363379034771805109, -8.531250002048352599 ) ) ;
#19153=CARTESIAN_POINT ( 'NONE',  ( 9.099922391974125446, -4.256835254723014828, -100.0000000000000000 ) ) ;
#19154=CARTESIAN_POINT ( 'NONE',  ( -9.999999999999998224, 0.000000000000000000, -180.0000000000000000 ) ) ;
#19155=CARTESIAN_POINT ( 'NONE',  ( -2.293366432827344421E-15, -12.48450537969573659, -159.4062500020483810 ) ) ;
#19163=CARTESIAN_POINT ( 'NONE',  ( 5.405949406249999534, 9.363379034771803333, -80.59375000204838102 ) ) ;
#19164=CARTESIAN_POINT ( 'NONE',  ( 10.81189881249999551, -6.242252689847874514, -82.65625000204836681 ) ) ;
#19167=CARTESIAN_POINT ( 'NONE',  ( -10.81189881249999729, -6.242252689847864744, -164.1562500020483810 ) ) ;
#19168=CARTESIAN_POINT ( 'NONE',  ( 10.81189881249999729, 0.000000000000000000, -178.5312500020483810 ) ) ;
#19170=CARTESIAN_POINT ( 'NONE',  ( -10.00000000000000000, -5.773502691896251982, -153.0000000040967905 ) ) ;
#19172=CARTESIAN_POINT ( 'NONE',  ( -10.81189881249999729, 6.242252689847871849, -3.718750002048354819 ) ) ;
#19174=CARTESIAN_POINT ( 'NONE',  ( 5.405949406249999534, 9.363379034771803333, -110.5937500020483810 ) ) ;
#19176=CARTESIAN_POINT ( 'NONE',  ( 5.405949406249992428, -9.363379034771808662, -15.28125000204835793 ) ) ;
#19179=CARTESIAN_POINT ( 'NONE',  ( -10.81189881249999729, 6.242252689847871849, -107.4062500020483810 ) ) ;
#19182=CARTESIAN_POINT ( 'NONE',  ( 4.999999999999992006, -8.660254037844389075, -95.62500000409677625 ) ) ;
#19183=CARTESIAN_POINT ( 'NONE',  ( 0.000000000000000000, 0.000000000000000000, -99.99999999999998579 ) ) ;
#19184=CARTESIAN_POINT ( 'NONE',  ( 10.81189881249999907, 6.242252689847868297, -40.21875000204835970 ) ) ;
#19185=ORIENTED_EDGE ( 'NONE', *, *, #26161, .T. ) ;
#19189=CARTESIAN_POINT ( 'NONE',  ( -5.000000000000003553, -8.660254037844383745, -19.37500000409675494 ) ) ;
#19199=VERTEX_POINT ( 'NONE', #23923 ) ;
#19200=ORIENTED_EDGE ( 'NONE', *, *, #11974, .T. ) ;
#19205=CARTESIAN_POINT ( 'NONE',  ( -10.81189881249999729, 1.324075727343319199E-15, -182.2812500020483810 ) ) ;
#19209=CARTESIAN_POINT ( 'NONE',  ( -10.81189881249999729, 1.324075727343319199E-15, -98.09375000204838102 ) ) ;
#19210=CARTESIAN_POINT ( 'NONE',  ( 4.999999999999992006, -8.660254037844389075, -143.2500000000000000 ) ) ;
#19211=CARTESIAN_POINT ( 'NONE',  ( 10.81189881249999729, 0.000000000000000000, -108.0312500020483810 ) ) ;
#19213=CARTESIAN_POINT ( 'NONE',  ( 10.81189881249999551, -6.242252689847874514, -118.4687500020483810 ) ) ;
#19216=CARTESIAN_POINT ( 'NONE',  ( -2.121150477449813534E-15, -11.54700538379251284, -141.8750000000000000 ) ) ;
#19217=CARTESIAN_POINT ( 'NONE',  ( 10.00000000000000000, 5.773502691896255534, -3.374999999999961364 ) ) ;
#19220=CARTESIAN_POINT ( 'NONE',  ( 7.070501591499377789E-16, 11.54700538379251284, -177.5000000040967905 ) ) ;
#19222=CARTESIAN_POINT ( 'NONE',  ( 10.81189881249999907, 6.242252689847868297, -29.71875000204834549 ) ) ;
#19223=CARTESIAN_POINT ( 'NONE',  ( 7.070501591499376803E-16, 11.54700538379251284, -117.1249999999999858 ) ) ;
#19224=CARTESIAN_POINT ( 'NONE',  ( 10.81189881249999551, -6.242252689847874514, -140.9687500020483810 ) ) ;
#19227=CARTESIAN_POINT ( 'NONE',  ( 9.999999999999998224, 0.000000000000000000, -67.99999999999997158 ) ) ;
#19228=CARTESIAN_POINT ( 'NONE',  ( 10.81189881249999907, 6.242252689847868297, -136.4062500020484094 ) ) ;
#19230=EDGE_CURVE ( 'NONE', #37069, #36923, #32355, .T. ) ;
#19231=ORIENTED_EDGE ( 'NONE', *, *, #29132, .F. ) ;
#19233=CARTESIAN_POINT ( 'NONE',  ( -10.00000000000000000, -5.773502691896251982, -118.5000000040967905 ) ) ;
#19235=CARTESIAN_POINT ( 'NONE',  ( 5.405949406249999534, 9.363379034771803333, -76.09375000204838102 ) ) ;
#19240=CARTESIAN_POINT ( 'NONE',  ( -5.000000000000003553, -8.660254037844383745, -46.37500000409677625 ) ) ;
#19241=CARTESIAN_POINT ( 'NONE',  ( -2.293366432827344421E-15, -12.48450537969573659, -36.40625000204835970 ) ) ;
#19246=CARTESIAN_POINT ( 'NONE',  ( 9.999999999999998224, 0.000000000000000000, -150.8750000040967905 ) ) ;
#19257=CARTESIAN_POINT ( 'NONE',  ( -10.81189881249999907, -6.242252689847864744, -127.9687500020483810 ) ) ;
#19258=CARTESIAN_POINT ( 'NONE',  ( 10.81189881249999907, 6.242252689847868297, -136.4062500020484094 ) ) ;
#19260=CARTESIAN_POINT ( 'NONE',  ( -2.293366432827344421E-15, -12.48450537969573659, -150.2187500020484094 ) ) ;
#19261=CARTESIAN_POINT ( 'NONE',  ( 9.999999999999998224, 0.000000000000000000, -125.3750000040967905 ) ) ;
#19262=CARTESIAN_POINT ( 'NONE',  ( 4.999999999999992006, -8.660254037844389075, -165.7500000000000000 ) ) ;
#19265=CARTESIAN_POINT ( 'NONE',  ( -10.81189881249999907, -6.242252689847864744, -64.96875000204838102 ) ) ;
#19267=CARTESIAN_POINT ( 'NONE',  ( 5.405949406249992428, -9.363379034771808662, -159.0937500020484094 ) ) ;
#19271=CARTESIAN_POINT ( 'NONE',  ( 9.999999999999996447, -5.773502691896262640, -89.12499999999997158 ) ) ;
#19272=ORIENTED_EDGE ( 'NONE', *, *, #16750, .T. ) ;
#19273=CARTESIAN_POINT ( 'NONE',  ( -5.405949406249996869, 9.363379034771805109, -119.5312500020483952 ) ) ;
#19274=CARTESIAN_POINT ( 'NONE',  ( 9.999999999999998224, 0.000000000000000000, -143.3750000040967905 ) ) ;
#19275=CARTESIAN_POINT ( 'NONE',  ( 5.000000000000000000, 8.660254037844385522, -159.2500000000000000 ) ) ;
#19278=EDGE_CURVE ( 'NONE', #23210, #25155, #28192, .T. ) ;
#19281=CARTESIAN_POINT ( 'NONE',  ( 10.81189881249999729, 0.000000000000000000, -61.53125000204837391 ) ) ;
#19300=CARTESIAN_POINT ( 'NONE',  ( 5.000000000000000000, 8.660254037844385522, -30.24999999999997158 ) ) ;
#19303=CARTESIAN_POINT ( 'NONE',  ( -10.81189881249999907, -6.242252689847864744, -154.9687500020484094 ) ) ;
#19304=CARTESIAN_POINT ( 'NONE',  ( 10.81189881249999729, 6.242252689847867408, -169.2187500020483810 ) ) ;
#19307=CARTESIAN_POINT ( 'NONE',  ( 5.000000000000000000, 8.660254037844385522, -187.7500000000000000 ) ) ;
#19314=CARTESIAN_POINT ( 'NONE',  ( -10.81189881249999729, 6.242252689847871849, -63.90625000204838813 ) ) ;
#19316=CARTESIAN_POINT ( 'NONE',  ( 4.999999999999992006, -8.660254037844389075, -114.7499999999999858 ) ) ;
#19318=CARTESIAN_POINT ( 'NONE',  ( 5.405949406249999534, 9.363379034771803333, -142.2812500020483810 ) ) ;
#19319=CARTESIAN_POINT ( 'NONE',  ( -10.81189881249999729, 6.242252689847871849, -159.9062500020483810 ) ) ;
#19321=CARTESIAN_POINT ( 'NONE',  ( 9.999999999999998224, 0.000000000000000000, -161.3750000040967905 ) ) ;
#19322=CARTESIAN_POINT ( 'NONE',  ( 10.81189881249999907, 6.242252689847868297, -91.21875000204838102 ) ) ;
#19325=CARTESIAN_POINT ( 'NONE',  ( -10.81189881249999729, 6.242252689847871849, -189.7187500020484379 ) ) ;
#19328=ADVANCED_FACE ( 'NONE', ( #18494 ), #1898, .F. ) ;
#19329=CARTESIAN_POINT ( 'NONE',  ( -9.999999999999998224, 1.224646799147353059E-15, -164.7500000000000000 ) ) ;
#19330=CARTESIAN_POINT ( 'NONE',  ( -2.121150477449813534E-15, -11.54700538379251284, -123.8749999999999858 ) ) ;
#19332=CARTESIAN_POINT ( 'NONE',  ( -5.405949406250003975, -9.363379034771801557, -83.03125000204838102 ) ) ;
#19335=( BOUNDED_CURVE ( )  B_SPLINE_CURVE ( 2, ( #29603, #6930, #20084, #36289, #16832, #30031, #26784 ),
 .UNSPECIFIED., .F., .F. ) 
 B_SPLINE_CURVE_WITH_KNOTS ( ( 3, 2, 2, 3 ),
 ( 0.3656716417910448325, 0.3669154228855722177, 0.3681592039800996030, 0.3694029850746269883 ),
 .UNSPECIFIED. ) 
 CURVE ( )  GEOMETRIC_REPRESENTATION_ITEM ( )  RATIONAL_B_SPLINE_CURVE ( ( 0.9999999999999940048, 0.8660254037844447028, 1.000000000000000000, 0.8660254037844387076, 1.000000000000000000, 0.8660254037844267172, 1.000000000000011990 ) ) 
 REPRESENTATION_ITEM ( '' )  );
#19336=CARTESIAN_POINT ( 'NONE',  ( 9.999999999999998224, 0.000000000000000000, -60.87500000409676204 ) ) ;
#19337=CARTESIAN_POINT ( 'NONE',  ( 7.644554776091147741E-16, 12.48450537969573659, -18.96875000204837036 ) ) ;
#19341=CARTESIAN_POINT ( 'NONE',  ( 10.81189881249999907, 6.242252689847868297, -11.90625000204836859 ) ) ;
#19347=CARTESIAN_POINT ( 'NONE',  ( 24.99999999999999645, 3.061616997868382648E-15, -169.9999999999999716 ) ) ;
#19348=( BOUNDED_CURVE ( )  B_SPLINE_CURVE ( 2, ( #18086, #21327, #37520, #31280, #34515, #30630, #37735 ),
 .UNSPECIFIED., .F., .F. ) 
 B_SPLINE_CURVE_WITH_KNOTS ( ( 3, 2, 2, 3 ),
 ( 0.3470149253731344974, 0.3482587064676618271, 0.3495024875621891569, 0.3507462686567164867 ),
 .UNSPECIFIED. ) 
 CURVE ( )  GEOMETRIC_REPRESENTATION_ITEM ( )  RATIONAL_B_SPLINE_CURVE ( ( 0.9999999999999820144, 0.8660254037844566932, 1.000000000000000000, 0.8660254037844387076, 1.000000000000000000, 0.8660254037844327124, 1.000000000000005995 ) ) 
 REPRESENTATION_ITEM ( '' )  );
#19350=CARTESIAN_POINT ( 'NONE',  ( 9.999999999999998224, 0.000000000000000000, -120.5000000000000000 ) ) ;
#19353=CARTESIAN_POINT ( 'NONE',  ( -7.320507999635632146, -7.320508119598070351, -179.9330127040876732 ) ) ;
#19356=EDGE_LOOP ( 'NONE', ( #21579, #29340, #15520, #39675 ) ) ;
#19366=CARTESIAN_POINT ( 'NONE',  ( -10.81189881249999729, 6.242252689847871849, -159.9062500020483810 ) ) ;
#19372=EDGE_CURVE ( 'NONE', #22578, #12639, #12013, .T. ) ;
#19373=CARTESIAN_POINT ( 'NONE',  ( 7.644554776091147741E-16, 12.48450537969573659, -77.46875000204838102 ) ) ;
#19374=CARTESIAN_POINT ( 'NONE',  ( -10.81189881249999907, -6.242252689847864744, -87.65625000204836681 ) ) ;
#19376=CARTESIAN_POINT ( 'NONE',  ( -9.999999999999998224, 0.000000000000000000, -99.99999999999998579 ) ) ;
#19377=CARTESIAN_POINT ( 'NONE',  ( 7.644554776091147741E-16, 12.48450537969573659, -169.1562500020484094 ) ) ;
#19378=CARTESIAN_POINT ( 'NONE',  ( -5.405949406249996869, 9.363379034771805109, -178.0312500020483810 ) ) ;
#19379=CARTESIAN_POINT ( 'NONE',  ( 9.999999999999998224, 0.000000000000000000, -159.8750000040967905 ) ) ;
#19380=CARTESIAN_POINT ( 'NONE',  ( -10.81189881249999907, -6.242252689847864744, -9.468750002048357928 ) ) ;
#19382=CARTESIAN_POINT ( 'NONE',  ( -2.293366432827344421E-15, -12.48450537969573659, -111.2187500020483668 ) ) ;
#19384=CARTESIAN_POINT ( 'NONE',  ( -5.405949406250003975, -9.363379034771801557, -15.53125000204835793 ) ) ;
#19387=CARTESIAN_POINT ( 'NONE',  ( -5.405949406249996869, 9.363379034771805109, -107.5312500020483810 ) ) ;
#19390=CARTESIAN_POINT ( 'NONE',  ( -9.999999999999998224, 5.773502691896259087, -84.25000000409677625 ) ) ;
#19392=CARTESIAN_POINT ( 'NONE',  ( 10.81189881249999551, -6.242252689847874514, -40.46875000204835970 ) ) ;
#19396=CARTESIAN_POINT ( 'NONE',  ( 9.999999999999998224, 0.000000000000000000, -9.875000004096746054 ) ) ;
#19397=VECTOR ( 'NONE', #28768, 1000.000000000000000 ) ;
#19399=CARTESIAN_POINT ( 'NONE',  ( 9.999999999999998224, 0.000000000000000000, -119.3750000040967905 ) ) ;
#19404=ORIENTED_EDGE ( 'NONE', *, *, #25324, .T. ) ;
#19410=ORIENTED_EDGE ( 'NONE', *, *, #15854, .T. ) ;
#19411=( BOUNDED_CURVE ( )  B_SPLINE_CURVE ( 2, ( #26877, #27093, #17144, #40442, #10886, #30345, #10462 ),
 .UNSPECIFIED., .F., .F. ) 
 B_SPLINE_CURVE_WITH_KNOTS ( ( 3, 2, 2, 3 ),
 ( 0.4440298507462688282, 0.4452736318407962135, 0.4465174129353234878, 0.4477611940298508730 ),
 .UNSPECIFIED. ) 
 CURVE ( )  GEOMETRIC_REPRESENTATION_ITEM ( )  RATIONAL_B_SPLINE_CURVE ( ( 0.9999999999999820144, 0.8660254037844566932, 1.000000000000000000, 0.8660254037844387076, 1.000000000000000000, 0.8660254037844267172, 1.000000000000011990 ) ) 
 REPRESENTATION_ITEM ( '' )  );
#19414=CARTESIAN_POINT ( 'NONE',  ( 7.644554776091147741E-16, 12.48450537969573659, -184.1562500020484094 ) ) ;
#19417=CARTESIAN_POINT ( 'NONE',  ( 10.81189881249999907, 6.242252689847868297, -103.2187500020483810 ) ) ;
#19419=CARTESIAN_POINT ( 'NONE',  ( -10.81189881249999907, -6.242252689847864744, -105.6562500020483952 ) ) ;
#19421=CARTESIAN_POINT ( 'NONE',  ( -5.405949406249996869, 9.363379034771805109, -116.3437500020483810 ) ) ;
#19425=CARTESIAN_POINT ( 'NONE',  ( -10.00000000000000000, -5.773502691896251982, -136.1250000000000000 ) ) ;
#19426=CARTESIAN_POINT ( 'NONE',  ( -10.00000000000000000, -5.773502691896251982, -8.624999999999966249 ) ) ;
#19429=CARTESIAN_POINT ( 'NONE',  ( 10.00000000000000000, 5.773502691896255534, -176.2500000040968189 ) ) ;
#19431=CARTESIAN_POINT ( 'NONE',  ( 7.644554776091147741E-16, 12.48450537969573659, -29.46875000204835260 ) ) ;
#19432=CARTESIAN_POINT ( 'NONE',  ( 5.405949406249999534, 9.363379034771803333, -136.0937500020483810 ) ) ;
#19434=CARTESIAN_POINT ( 'NONE',  ( 9.999999999999998224, 0.000000000000000000, -69.49999999999997158 ) ) ;
#19435=CARTESIAN_POINT ( 'NONE',  ( -5.405949406250003975, -9.363379034771801557, -134.0312500020484094 ) ) ;
#19439=CARTESIAN_POINT ( 'NONE',  ( -10.00000000000000000, -5.773502691896251982, -108.0000000040967763 ) ) ;
#19441=CARTESIAN_POINT ( 'NONE',  ( -5.405949406250003975, -9.363379034771801557, -66.34375000204836681 ) ) ;
#19448=CARTESIAN_POINT ( 'NONE',  ( -9.999999999999998224, 5.773502691896259087, -40.75000000409676204 ) ) ;
#19449=CARTESIAN_POINT ( 'NONE',  ( -5.405949406250003975, -9.363379034771801557, -39.53125000204838102 ) ) ;
#19450=CARTESIAN_POINT ( 'NONE',  ( 9.999999999999998224, 0.000000000000000000, -141.5000000000000000 ) ) ;
#19459=VERTEX_POINT ( 'NONE', #22377 ) ;
#19461=DIRECTION ( 'NONE',  ( -0.000000000000000000, -0.000000000000000000, -1.000000000000000000 ) ) ;
#19468=CARTESIAN_POINT ( 'NONE',  ( 4.999999999999992006, -8.660254037844389075, -119.2500000000000000 ) ) ;
#19469=CARTESIAN_POINT ( 'NONE',  ( 10.81189881249999551, -6.242252689847874514, -122.9687500020483810 ) ) ;
#19470=CARTESIAN_POINT ( 'NONE',  ( -5.405949406250003975, -9.363379034771801557, -135.5312500020484094 ) ) ;
#19472=CARTESIAN_POINT ( 'NONE',  ( -10.81189881249999729, -6.242252689847864744, -135.4687500020483810 ) ) ;
#19473=CARTESIAN_POINT ( 'NONE',  ( 4.999999999999992006, -8.660254037844389075, -125.6250000040967620 ) ) ;
#19474=CARTESIAN_POINT ( 'NONE',  ( -10.00000000000000000, -5.773502691896251982, -161.6250000000000284 ) ) ;
#19478=CARTESIAN_POINT ( 'NONE',  ( -10.81189881249999729, 6.242252689847871849, -50.21875000204837391 ) ) ;
#19480=CARTESIAN_POINT ( 'NONE',  ( -10.81189881249999729, 6.242252689847871849, -161.2187500020483526 ) ) ;
#19485=CARTESIAN_POINT ( 'NONE',  ( 7.070501591499377789E-16, 11.54700538379251284, -88.62500000000000000 ) ) ;
#19486=ORIENTED_EDGE ( 'NONE', *, *, #15086, .F. ) ;
#19487=CARTESIAN_POINT ( 'NONE',  ( -10.81189881249999729, -6.242252689847864744, -114.6562500020483952 ) ) ;
#19488=CARTESIAN_POINT ( 'NONE',  ( -2.121150477449813534E-15, -11.54700538379251284, -128.7500000040967620 ) ) ;
#19494=CARTESIAN_POINT ( 'NONE',  ( 5.405949406249992428, -9.363379034771808662, -58.78125000204836681 ) ) ;
#19499=CARTESIAN_POINT ( 'NONE',  ( 10.00000000000000000, 5.773502691896255534, -167.2500000040967905 ) ) ;
#19504=ORIENTED_EDGE ( 'NONE', *, *, #21741, .T. ) ;
#19512=CARTESIAN_POINT ( 'NONE',  ( 4.999999999999992006, -8.660254037844389075, -112.1250000040967763 ) ) ;
#19514=CARTESIAN_POINT ( 'NONE',  ( -10.00000000000000000, -5.773502691896251982, -29.62499999999995737 ) ) ;
#19517=CARTESIAN_POINT ( 'NONE',  ( 7.644554776091147741E-16, 12.48450537969573659, -150.9687500020483810 ) ) ;
#19518=CARTESIAN_POINT ( 'NONE',  ( 10.81189881249999729, 0.000000000000000000, -167.8437500020484094 ) ) ;
#19519=CARTESIAN_POINT ( 'NONE',  ( -9.999999999999998224, 1.224646799147353059E-15, -159.1250000040967905 ) ) ;
#19520=DIRECTION ( 'NONE',  ( -1.000000000000000000, 0.000000000000000000, 0.000000000000000000 ) ) ;
#19521=CARTESIAN_POINT ( 'NONE',  ( -2.121150477449813534E-15, -11.54700538379251284, -186.8750000000000284 ) ) ;
#19525=DIRECTION ( 'NONE',  ( -0.000000000000000000, -0.000000000000000000, -1.000000000000000000 ) ) ;
#19526=CARTESIAN_POINT ( 'NONE',  ( -5.405949406250003975, -9.363379034771801557, -184.8437500020483810 ) ) ;
#19528=CARTESIAN_POINT ( 'NONE',  ( 7.644554776091147741E-16, 12.48450537969573659, -56.65625000204838813 ) ) ;
#19530=CARTESIAN_POINT ( 'NONE',  ( -9.999999999999998224, 1.224646799147353059E-15, -112.2499999999999858 ) ) ;
#19532=CARTESIAN_POINT ( 'NONE',  ( -5.405949406250003975, -9.363379034771801557, -140.0312500020484094 ) ) ;
#19533=CARTESIAN_POINT ( 'NONE',  ( 10.81189881249999907, 6.242252689847868297, -157.4062500020483810 ) ) ;
#19535=CARTESIAN_POINT ( 'NONE',  ( -9.999999999999998224, 1.224646799147353059E-15, -104.7499999999999858 ) ) ;
#19536=CARTESIAN_POINT ( 'NONE',  ( 10.81189881249999907, 6.242252689847868297, -89.71875000204836681 ) ) ;
#19539=CARTESIAN_POINT ( 'NONE',  ( -10.81189881249999729, 6.242252689847871849, -188.2187500020483810 ) ) ;
#19543=CARTESIAN_POINT ( 'NONE',  ( -10.81189881249999729, 1.324075727343319199E-15, -81.78125000204839523 ) ) ;
#19545=CARTESIAN_POINT ( 'NONE',  ( 9.999999999999998224, 0.000000000000000000, -57.87500000409676204 ) ) ;
#19546=CARTESIAN_POINT ( 'NONE',  ( 10.81189881249999729, 0.000000000000000000, -20.84375000204835615 ) ) ;
#19547=CARTESIAN_POINT ( 'NONE',  ( -9.999999999999227285, -5.773502691896698735, -138.0000000040967620 ) ) ;
#19549=CARTESIAN_POINT ( 'NONE',  ( -5.405949406250003975, -9.363379034771801557, -15.53125000204835793 ) ) ;
#19558=CARTESIAN_POINT ( 'NONE',  ( 10.81189881249999551, -6.242252689847874514, -103.4687500020483668 ) ) ;
#19560=VERTEX_POINT ( 'NONE', #8287 ) ;
#19572=CARTESIAN_POINT ( 'NONE',  ( -10.81189881249999907, -6.242252689847864744, -153.6562500020484094 ) ) ;
#19574=CARTESIAN_POINT ( 'NONE',  ( 5.000000000000000000, 8.660254037844385522, -178.7500000000000284 ) ) ;
#19578=CARTESIAN_POINT ( 'NONE',  ( -10.81189881249999907, -6.242252689847864744, -75.46875000204836681 ) ) ;
#19579=CARTESIAN_POINT ( 'NONE',  ( 10.81189881249999729, 0.000000000000000000, -87.03125000204838102 ) ) ;
#19581=( BOUNDED_CURVE ( )  B_SPLINE_CURVE ( 2, ( #7700, #40904, #5697, #8926, #18036, #4889, #21064 ),
 .UNSPECIFIED., .F., .F. ) 
 B_SPLINE_CURVE_WITH_KNOTS ( ( 3, 2, 2, 3 ),
 ( 0.4701492537313434195, 0.4713930348258707492, 0.4726368159203981900, 0.4738805970149255198 ),
 .UNSPECIFIED. ) 
 CURVE ( )  GEOMETRIC_REPRESENTATION_ITEM ( )  RATIONAL_B_SPLINE_CURVE ( ( 0.9999999999999880096, 0.8660254037844506980, 1.000000000000000000, 0.8660254037844387076, 1.000000000000000000, 0.8660254037844207220, 1.000000000000017986 ) ) 
 REPRESENTATION_ITEM ( '' )  );
#19583=CARTESIAN_POINT ( 'NONE',  ( 10.81189881249999729, 0.000000000000000000, -163.5312500020484094 ) ) ;
#19584=CARTESIAN_POINT ( 'NONE',  ( 10.81189881249999729, 0.000000000000000000, -177.0312500020483810 ) ) ;
#19585=CARTESIAN_POINT ( 'NONE',  ( 7.070501591499377789E-16, 11.54700538379251284, -153.5000000040967905 ) ) ;
#19587=CARTESIAN_POINT ( 'NONE',  ( 10.81189881249999907, 6.242252689847868297, -8.718750002048359704 ) ) ;
#19589=CARTESIAN_POINT ( 'NONE',  ( 10.81189881249999907, 6.242252689847868297, -113.7187500020483810 ) ) ;
#19591=CARTESIAN_POINT ( 'NONE',  ( 10.81189881249999907, 6.242252689847868297, -11.90625000204836859 ) ) ;
#19595=CARTESIAN_POINT ( 'NONE',  ( 10.81189881249999729, 0.000000000000000000, -111.0312500020483810 ) ) ;
#19597=VERTEX_POINT ( 'NONE', #40845 ) ;
#19599=CARTESIAN_POINT ( 'NONE',  ( 5.000000000000000000, 8.660254037844385522, -81.62500000409676204 ) ) ;
#19601=CARTESIAN_POINT ( 'NONE',  ( 5.405949406249992428, -9.363379034771808662, -45.09375000204837391 ) ) ;
#19606=CARTESIAN_POINT ( 'NONE',  ( -5.000000000000003553, -8.660254037844383745, -14.87500000409674961 ) ) ;
#19621=CARTESIAN_POINT ( 'NONE',  ( 10.81189881249999551, -6.242252689847874514, -183.1562500020484094 ) ) ;
#19627=CARTESIAN_POINT ( 'NONE',  ( -2.293366432827344421E-15, -12.48450537969573659, -103.7187500020483668 ) ) ;
#19629=CARTESIAN_POINT ( 'NONE',  ( -5.405949406250003975, -9.363379034771801557, -105.5312500020483810 ) ) ;
#19631=CARTESIAN_POINT ( 'NONE',  ( -10.81189881249999729, -6.242252689847864744, -115.9687500020483810 ) ) ;
#19635=CARTESIAN_POINT ( 'NONE',  ( 5.000000000000000000, 8.660254037844385522, -141.2500000000000000 ) ) ;
#19636=CARTESIAN_POINT ( 'NONE',  ( -4.999999999999996447, 8.660254037844387298, -2.999999999999975131 ) ) ;
#19639=CARTESIAN_POINT ( 'NONE',  ( 5.000000000000000000, 8.660254037844385522, -183.6250000040967905 ) ) ;
#19641=CARTESIAN_POINT ( 'NONE',  ( -10.81189881249999729, 1.324075727343319199E-15, -29.09375000204836326 ) ) ;
#19643=CARTESIAN_POINT ( 'NONE',  ( -10.81189881249999729, 6.242252689847871849, -134.2187500020483810 ) ) ;
#19645=CARTESIAN_POINT ( 'NONE',  ( -5.405949406249996869, 9.363379034771805109, -37.03125000204837391 ) ) ;
#19647=CARTESIAN_POINT ( 'NONE',  ( 4.999999999999992006, -8.660254037844389075, -66.74999999999997158 ) ) ;
#19648=CARTESIAN_POINT ( 'NONE',  ( 5.405949406249999534, 9.363379034771803333, -130.2812500020483810 ) ) ;
#19651=ORIENTED_EDGE ( 'NONE', *, *, #3826, .F. ) ;
#19652=CARTESIAN_POINT ( 'NONE',  ( -2.121150477449813534E-15, -11.54700538379251284, -128.3750000000000000 ) ) ;
#19653=CARTESIAN_POINT ( 'NONE',  ( 9.999999999999998224, 0.000000000000000000, -107.3750000040967763 ) ) ;
#19654=CARTESIAN_POINT ( 'NONE',  ( 10.00000000000051159, -5.773502691895965988, -146.1250000000000284 ) ) ;
#19655=CARTESIAN_POINT ( 'NONE',  ( -10.81189881249999907, -6.242252689847864744, -63.46875000204838102 ) ) ;
#19656=EDGE_LOOP ( 'NONE', ( #9169, #19200, #12382, #16524 ) ) ;
#19660=CARTESIAN_POINT ( 'NONE',  ( 5.000000000000000000, 8.660254037844385522, -119.1250000040967905 ) ) ;
#19661=CARTESIAN_POINT ( 'NONE',  ( -2.121150477449813534E-15, -11.54700538379251284, -32.75000000409674783 ) ) ;
#19662=CARTESIAN_POINT ( 'NONE',  ( 10.00000000000000000, 5.773502691896255534, -166.8750000000000000 ) ) ;
#19667=VECTOR ( 'NONE', #12059, 1000.000000000000000 ) ;
#19677=CARTESIAN_POINT ( 'NONE',  ( 5.405949406249999534, 9.363379034771803333, -128.5937500020483810 ) ) ;
#19679=CARTESIAN_POINT ( 'NONE',  ( 7.644554776091147741E-16, 12.48450537969573659, -130.1562500020483810 ) ) ;
#19681=CARTESIAN_POINT ( 'NONE',  ( 7.644554776091147741E-16, 12.48450537969573659, -134.4687500020483810 ) ) ;
#19682=CARTESIAN_POINT ( 'NONE',  ( -9.999999999999998224, 1.224646799147353059E-15, -126.1250000040967620 ) ) ;
#19685=CARTESIAN_POINT ( 'NONE',  ( -4.999999999999996447, 8.660254037844387298, -165.0000000000000000 ) ) ;
#19686=CARTESIAN_POINT ( 'NONE',  ( -2.293366432827344421E-15, -12.48450537969573659, -0.4062500020483583718 ) ) ;
#19687=EDGE_CURVE ( 'NONE', #17374, #34823, #42533, .T. ) ;
#19690=CARTESIAN_POINT ( 'NONE',  ( -5.405949406249996869, 9.363379034771805109, -54.84375000204835970 ) ) ;
#19692=CARTESIAN_POINT ( 'NONE',  ( 10.81189881249999551, -6.242252689847874514, -164.9687500020484094 ) ) ;
#19696=FACE_OUTER_BOUND ( 'NONE', #22106, .T. ) ;
#19698=CARTESIAN_POINT ( 'NONE',  ( 9.999999999999996447, -5.773502691896262640, -87.62499999999998579 ) ) ;
#19700=CARTESIAN_POINT ( 'NONE',  ( -2.293366432827344421E-15, -12.48450537969573659, -118.9062500020483952 ) ) ;
#19701=CARTESIAN_POINT ( 'NONE',  ( 10.00000000000000000, 5.773502691896255534, -134.2500000040967905 ) ) ;
#19705=CARTESIAN_POINT ( 'NONE',  ( 4.999999999999992006, -8.660254037844389075, -159.7500000000000000 ) ) ;
#19706=CARTESIAN_POINT ( 'NONE',  ( 10.81189881249999729, 0.000000000000000000, -57.03125000204836681 ) ) ;
#19712=CARTESIAN_POINT ( 'NONE',  ( 9.999999999999998224, 0.000000000000000000, -100.9999999999999858 ) ) ;
#19714=VERTEX_POINT ( 'NONE', #35472 ) ;
#19718=ORIENTED_EDGE ( 'NONE', *, *, #21677, .T. ) ;
#19727=CARTESIAN_POINT ( 'NONE',  ( -9.999999999999998224, 5.773502691896259087, -31.37499999999995737 ) ) ;
#19730=CARTESIAN_POINT ( 'NONE',  ( -5.405949406250003975, -9.363379034771801557, -150.3437500020483810 ) ) ;
#19731=CARTESIAN_POINT ( 'NONE',  ( -2.293366432827344421E-15, -12.48450537969573659, -162.2187500020483810 ) ) ;
#19733=CARTESIAN_POINT ( 'NONE',  ( 9.999999999999227285, 5.773502691896701400, -107.2500000040967620 ) ) ;
#19735=CARTESIAN_POINT ( 'NONE',  ( 10.00000000000000000, 5.773502691896255534, -189.3750000000000000 ) ) ;
#19740=CARTESIAN_POINT ( 'NONE',  ( 5.405949406249992428, -9.363379034771808662, -189.0937500020483810 ) ) ;
#19742=CARTESIAN_POINT ( 'NONE',  ( 10.81189881249999551, -6.242252689847874514, -63.15625000204838813 ) ) ;
#19744=CARTESIAN_POINT ( 'NONE',  ( -2.121150477449813534E-15, -11.54700538379251284, -117.8749999999999858 ) ) ;
#19745=ORIENTED_EDGE ( 'NONE', *, *, #34029, .F. ) ;
#19746=CARTESIAN_POINT ( 'NONE',  ( -10.81189881249999729, -6.242252689847864744, -146.1562500020484094 ) ) ;
#19748=CARTESIAN_POINT ( 'NONE',  ( 7.644554776091147741E-16, 12.48450537969573659, -152.6562500020484094 ) ) ;
#19750=CARTESIAN_POINT ( 'NONE',  ( 10.81189881249999551, -6.242252689847874514, -92.96875000204838102 ) ) ;
#19751=ORIENTED_EDGE ( 'NONE', *, *, #10961, .F. ) ;
#19753=CARTESIAN_POINT ( 'NONE',  ( 10.81189881249999551, -6.242252689847874514, -188.9687500020484094 ) ) ;
#19757=CARTESIAN_POINT ( 'NONE',  ( 7.644554776091147741E-16, 12.48450537969573659, -86.65625000204838102 ) ) ;
#19759=CARTESIAN_POINT ( 'NONE',  ( -10.00000000000000000, -5.773502691896251982, -58.50000000409676915 ) ) ;
#19760=CARTESIAN_POINT ( 'NONE',  ( 7.644554776091147741E-16, 12.48450537969573659, -15.96875000204836503 ) ) ;
#19763=CARTESIAN_POINT ( 'NONE',  ( 10.81189881249999907, 6.242252689847868297, -14.90625000204837036 ) ) ;
#19773=CARTESIAN_POINT ( 'NONE',  ( -10.81189881249999729, -6.242252689847864744, -100.9687500020483668 ) ) ;
#19774=ORIENTED_EDGE ( 'NONE', *, *, #34237, .T. ) ;
#19780=DIRECTION ( 'NONE',  ( -0.000000000000000000, -0.000000000000000000, -1.000000000000000000 ) ) ;
#19784=CARTESIAN_POINT ( 'NONE',  ( -5.405949406249996869, 9.363379034771805109, -157.0312500020484094 ) ) ;
#19790=CARTESIAN_POINT ( 'NONE',  ( -10.81189881249999729, 1.324075727343319199E-15, -77.09375000204838102 ) ) ;
#19791=CARTESIAN_POINT ( 'NONE',  ( 10.81189881249999907, 6.242252689847868297, -86.90625000204836681 ) ) ;
#19794=CARTESIAN_POINT ( 'NONE',  ( 10.81189881249999729, 0.000000000000000000, -169.5312500020484094 ) ) ;
#19795=CARTESIAN_POINT ( 'NONE',  ( -2.293366432827344421E-15, -12.48450537969573659, -180.4062500020484379 ) ) ;
#19796=CARTESIAN_POINT ( 'NONE',  ( -5.000000000000003553, -8.660254037844383745, -158.8750000040967905 ) ) ;
#19797=DIRECTION ( 'NONE',  ( -1.000000000000000000, 0.000000000000000000, 0.000000000000000000 ) ) ;
#19798=CARTESIAN_POINT ( 'NONE',  ( 5.405949406249999534, 9.363379034771803333, -8.593750002048345493 ) ) ;
#19800=CARTESIAN_POINT ( 'NONE',  ( 5.405949406249999534, 9.363379034771803333, -118.0937500020483810 ) ) ;
#19802=CARTESIAN_POINT ( 'NONE',  ( -5.405949406249996869, 9.363379034771805109, -10.03125000204835260 ) ) ;
#19805=CARTESIAN_POINT ( 'NONE',  ( -10.81189881249999729, 1.324075727343319199E-15, -105.7812500020483810 ) ) ;
#19808=CARTESIAN_POINT ( 'NONE',  ( 9.999999999999998224, 0.000000000000000000, -87.87500000409677625 ) ) ;
#19809=CARTESIAN_POINT ( 'NONE',  ( -4.999999999999996447, 8.660254037844387298, -145.8750000040967905 ) ) ;
#19810=CARTESIAN_POINT ( 'NONE',  ( -10.81189881249999907, -6.242252689847864744, -43.96875000204835970 ) ) ;
#19813=EDGE_CURVE ( 'NONE', #2320, #33286, #5225, .T. ) ;
#19815=CARTESIAN_POINT ( 'NONE',  ( -9.999999999999998224, 1.224646799147353059E-15, -9.125000004096744277 ) ) ;
#19819=VERTEX_POINT ( 'NONE', #42338 ) ;
#19823=ORIENTED_EDGE ( 'NONE', *, *, #29925, .T. ) ;
#19832=( BOUNDED_CURVE ( )  B_SPLINE_CURVE ( 2, ( #33480, #6922, #20075, #33269, #3695, #3906, #29595 ),
 .UNSPECIFIED., .F., .F. ) 
 B_SPLINE_CURVE_WITH_KNOTS ( ( 3, 2, 2, 3 ),
 ( 0.3395522388059703522, 0.3407960199004976820, 0.3420398009950250118, 0.3432835820895522860 ),
 .UNSPECIFIED. ) 
 CURVE ( )  GEOMETRIC_REPRESENTATION_ITEM ( )  RATIONAL_B_SPLINE_CURVE ( ( 0.9999999999999761302, 0.8660254037844625774, 1.000000000000000000, 0.8660254037844387076, 1.000000000000000000, 0.8660254037844327124, 1.000000000000005995 ) ) 
 REPRESENTATION_ITEM ( '' )  );
#19833=CARTESIAN_POINT ( 'NONE',  ( -10.81189881249999729, 1.324075727343319199E-15, -180.7812500020484094 ) ) ;
#19836=CARTESIAN_POINT ( 'NONE',  ( 10.81189881249999729, 0.000000000000000000, -98.84375000204838102 ) ) ;
#19838=CARTESIAN_POINT ( 'NONE',  ( 5.405949406249992428, -9.363379034771808662, -108.2812500020483810 ) ) ;
#19840=CARTESIAN_POINT ( 'NONE',  ( 10.81189881249999729, 6.242252689847867408, -112.2187500020483810 ) ) ;
#19844=LINE ( 'NONE', #38488, #41025 ) ;
#19845=CARTESIAN_POINT ( 'NONE',  ( -9.999999999999998224, 5.773502691896259087, -133.3750000000000000 ) ) ;
#19846=CARTESIAN_POINT ( 'NONE',  ( 4.999999999999992006, -8.660254037844389075, -6.749999999999978684 ) ) ;
#19849=CARTESIAN_POINT ( 'NONE',  ( 5.000000000000000000, 8.660254037844385522, -177.6250000040968189 ) ) ;
#19851=VECTOR ( 'NONE', #21063, 1000.000000000000000 ) ;
#19852=CARTESIAN_POINT ( 'NONE',  ( 10.81189881249999907, 6.242252689847868297, -32.71875000204835260 ) ) ;
#19854=CARTESIAN_POINT ( 'NONE',  ( 5.405949406249992428, -9.363379034771808662, -135.0937500020483810 ) ) ;
#19856=CARTESIAN_POINT ( 'NONE',  ( -10.81189881249999729, 1.324075727343319199E-15, -35.28125000204837391 ) ) ;
#19859=CARTESIAN_POINT ( 'NONE',  ( -5.000000000000003553, -8.660254037844383745, -63.99999999999997158 ) ) ;
#19860=CARTESIAN_POINT ( 'NONE',  ( -2.293366432827344421E-15, -12.48450537969573659, -130.9062500020483810 ) ) ;
#19862=ORIENTED_EDGE ( 'NONE', *, *, #38049, .F. ) ;
#19863=CARTESIAN_POINT ( 'NONE',  ( 10.00000000000051159, -5.773502691895965988, -128.1250000000000000 ) ) ;
#19864=CARTESIAN_POINT ( 'NONE',  ( -10.00000000000000000, -5.773502691896251982, -109.5000000040967905 ) ) ;
#19865=CARTESIAN_POINT ( 'NONE',  ( 9.999999999999998224, 0.000000000000000000, -162.5000000000000000 ) ) ;
#19866=CARTESIAN_POINT ( 'NONE',  ( -2.293366432827344421E-15, -12.48450537969573659, -64.71875000204838102 ) ) ;
#19873=CARTESIAN_POINT ( 'NONE',  ( 10.00000000000000000, 5.773502691896255534, -35.25000000409675494 ) ) ;
#19874=EDGE_CURVE ( 'NONE', #5096, #25139, #9130, .T. ) ;
#19879=ORIENTED_EDGE ( 'NONE', *, *, #31089, .F. ) ;
#19881=EDGE_LOOP ( 'NONE', ( #29327, #3658, #15197, #12389 ) ) ;
#19891=CARTESIAN_POINT ( 'NONE',  ( -10.81189881249999729, 1.324075727343319199E-15, -123.5937500020483952 ) ) ;
#19892=CARTESIAN_POINT ( 'NONE',  ( -10.81189881249999907, -6.242252689847864744, -135.6562500020484094 ) ) ;
#19894=CARTESIAN_POINT ( 'NONE',  ( 10.81189881249999729, 6.242252689847867408, -137.7187500020483810 ) ) ;
#19897=CARTESIAN_POINT ( 'NONE',  ( 9.999999999999996447, -5.773502691896262640, -167.1250000000000000 ) ) ;
#19901=CARTESIAN_POINT ( 'NONE',  ( -10.81189881249999729, 1.324075727343319199E-15, -53.09375000204835970 ) ) ;
#19903=CARTESIAN_POINT ( 'NONE',  ( -10.81189881249999729, 6.242252689847871849, -162.7187500020483810 ) ) ;
#19908=CARTESIAN_POINT ( 'NONE',  ( -2.121150477449813534E-15, -11.54700538379251284, -92.37500000000000000 ) ) ;
#19910=CARTESIAN_POINT ( 'NONE',  ( 5.405949406249999534, 9.363379034771803333, -112.2812500020483952 ) ) ;
#19911=CARTESIAN_POINT ( 'NONE',  ( 9.999999999999996447, -5.773502691896262640, -128.5000000040967905 ) ) ;
#19917=CARTESIAN_POINT ( 'NONE',  ( 10.81189881249999729, 0.000000000000000000, -54.03125000204836681 ) ) ;
#19923=CARTESIAN_POINT ( 'NONE',  ( 9.999999999999998224, 1.224646799147353059E-15, -99.99999999999998579 ) ) ;
#19924=VERTEX_POINT ( 'NONE', #28358 ) ;
#19926=VECTOR ( 'NONE', #2572, 1000.000000000000000 ) ;
#19927=EDGE_CURVE ( 'NONE', #5147, #6299, #16003, .T. ) ;
#19933=ORIENTED_EDGE ( 'NONE', *, *, #27941, .T. ) ;
#19937=CARTESIAN_POINT ( 'NONE',  ( 9.999999999999998224, 0.000000000000000000, -134.0000000000000000 ) ) ;
#19938=CARTESIAN_POINT ( 'NONE',  ( 4.999999999999992006, -8.660254037844389075, -24.74999999999996803 ) ) ;
#19941=CARTESIAN_POINT ( 'NONE',  ( 10.81189881249999729, 0.000000000000000000, -146.8437500020483810 ) ) ;
#19942=CARTESIAN_POINT ( 'NONE',  ( -10.81189881249999729, 6.242252689847871849, -162.7187500020483810 ) ) ;
#19943=CARTESIAN_POINT ( 'NONE',  ( 5.000000000000000000, 8.660254037844385522, -107.1250000040967763 ) ) ;
#19945=CARTESIAN_POINT ( 'NONE',  ( 5.000000000000000000, 8.660254037844385522, -186.2500000000000000 ) ) ;
#19948=DIRECTION ( 'NONE',  ( -0.000000000000000000, -0.000000000000000000, -1.000000000000000000 ) ) ;
#19950=CARTESIAN_POINT ( 'NONE',  ( -4.999999999999996447, 8.660254037844387298, -180.0000000000000000 ) ) ;
#19951=CARTESIAN_POINT ( 'NONE',  ( 10.81189881249999551, -6.242252689847874514, -187.4687500020484094 ) ) ;
#19954=CARTESIAN_POINT ( 'NONE',  ( 10.81189881249999907, 6.242252689847868297, -55.40625000204837391 ) ) ;
#19956=CARTESIAN_POINT ( 'NONE',  ( 7.070501591499377789E-16, 11.54700538379251284, -118.6250000000000142 ) ) ;
#19959=AXIS2_PLACEMENT_3D ( 'NONE', #31185, #23262, #33200 ) ;
#19960=CARTESIAN_POINT ( 'NONE',  ( -10.81189881249999729, -6.242252689847864744, -131.1562500020483810 ) ) ;
#19961=CARTESIAN_POINT ( 'NONE',  ( -5.405949406249996869, 9.363379034771805109, -149.5312500020483810 ) ) ;
#19964=CARTESIAN_POINT ( 'NONE',  ( -2.293366432827344421E-15, -12.48450537969573659, -84.21875000204835260 ) ) ;
#19965=ORIENTED_EDGE ( 'NONE', *, *, #11078, .T. ) ;
#19967=CARTESIAN_POINT ( 'NONE',  ( -10.81189881249999729, 6.242252689847871849, -183.7187500020484379 ) ) ;
#19971=CARTESIAN_POINT ( 'NONE',  ( 10.81189881249999729, 0.000000000000000000, -81.03125000204839523 ) ) ;
#19973=CARTESIAN_POINT ( 'NONE',  ( -10.00000000000000000, -5.773502691896251982, -57.00000000409676915 ) ) ;
#19974=CARTESIAN_POINT ( 'NONE',  ( -10.81189881249999729, 1.324075727343319199E-15, -18.59375000204835260 ) ) ;
#19976=CARTESIAN_POINT ( 'NONE',  ( -2.293366432827344421E-15, -12.48450537969573659, -13.90625000204836859 ) ) ;
#19977=DIRECTION ( 'NONE',  ( -0.000000000000000000, -0.000000000000000000, -1.000000000000000000 ) ) ;
#19978=CARTESIAN_POINT ( 'NONE',  ( 9.999999999999548805, 5.773502691896514882, -176.2500000040967905 ) ) ;
#19979=CARTESIAN_POINT ( 'NONE',  ( -10.00000000000076916, 5.773502691895813221, -114.2500000040967905 ) ) ;
#19980=CARTESIAN_POINT ( 'NONE',  ( 10.00000000000025402, -5.773502691896113426, -134.5000000040967905 ) ) ;
#19998=CARTESIAN_POINT ( 'NONE',  ( -10.81189881249999729, 1.324075727343319199E-15, -147.7812500020483810 ) ) ;
#20002=CARTESIAN_POINT ( 'NONE',  ( 5.000000000000000000, 8.660254037844385522, -161.1250000040967905 ) ) ;
#20005=CARTESIAN_POINT ( 'NONE',  ( -5.405949406250003975, -9.363379034771801557, -66.34375000204836681 ) ) ;
#20006=CARTESIAN_POINT ( 'NONE',  ( -10.81189881249999729, 1.324075727343319199E-15, -78.78125000204838102 ) ) ;
#20009=CARTESIAN_POINT ( 'NONE',  ( -2.293366432827344421E-15, -12.48450537969573659, -159.4062500020483810 ) ) ;
#20010=CARTESIAN_POINT ( 'NONE',  ( 5.405949406249992428, -9.363379034771808662, -180.2812500020484094 ) ) ;
#20011=DIRECTION ( 'NONE',  ( -1.000000000000000000, 0.000000000000000000, 0.000000000000000000 ) ) ;
#20012=CARTESIAN_POINT ( 'NONE',  ( 10.81189881249999907, 6.242252689847868297, -2.718750002048353043 ) ) ;
#20014=CARTESIAN_POINT ( 'NONE',  ( 5.405949406249992428, -9.363379034771808662, -103.5937500020483668 ) ) ;
#20016=CARTESIAN_POINT ( 'NONE',  ( -5.405949406250003975, -9.363379034771801557, -9.531250002048352599 ) ) ;
#20019=CARTESIAN_POINT ( 'NONE',  ( 10.81189881249999551, -6.242252689847874514, -105.1562500020483810 ) ) ;
#20023=CARTESIAN_POINT ( 'NONE',  ( 10.00000000000000000, 5.773502691896255534, -81.75000000409677625 ) ) ;
#20024=CARTESIAN_POINT ( 'NONE',  ( 9.999999999999479527, 5.773502691896553074, -146.2500000040967905 ) ) ;
#20025=CARTESIAN_POINT ( 'NONE',  ( -5.405949406249996869, 9.363379034771805109, -42.84375000204837391 ) ) ;
#20030=CARTESIAN_POINT ( 'NONE',  ( -10.00000000000076916, 5.773502691895813221, -139.3750000000000000 ) ) ;
#20031=CARTESIAN_POINT ( 'NONE',  ( 4.999999999999992006, -8.660254037844389075, -11.62500000409674783 ) ) ;
#20044=CYLINDRICAL_SURFACE ( 'NONE', #18344, 9.999999999999998224 ) ;
#20046=CARTESIAN_POINT ( 'NONE',  ( -5.405949406249996869, 9.363379034771805109, -173.5312500020484094 ) ) ;
#20050=CARTESIAN_POINT ( 'NONE',  ( -5.405949406250003975, -9.363379034771801557, -100.8437500020483810 ) ) ;
#20052=CARTESIAN_POINT ( 'NONE',  ( -5.405949406250003975, -9.363379034771801557, -108.5312500020483810 ) ) ;
#20054=CARTESIAN_POINT ( 'NONE',  ( 5.405949406249999534, 9.363379034771803333, -116.5937500020483810 ) ) ;
#20057=CARTESIAN_POINT ( 'NONE',  ( 9.999999999999998224, 0.000000000000000000, -113.3750000040967763 ) ) ;
#20058=CARTESIAN_POINT ( 'NONE',  ( -4.999999999999996447, 8.660254037844387298, -129.0000000000000000 ) ) ;
#20059=CARTESIAN_POINT ( 'NONE',  ( 5.000000000000000000, 8.660254037844385522, -6.249999999999977796 ) ) ;
#20062=CARTESIAN_POINT ( 'NONE',  ( 9.999999999999998224, 0.000000000000000000, -183.8750000040967905 ) ) ;
#20064=CARTESIAN_POINT ( 'NONE',  ( -5.405949406249996869, 9.363379034771805109, -27.84375000204836326 ) ) ;
#20066=CARTESIAN_POINT ( 'NONE',  ( 10.81189881249999551, -6.242252689847874514, -134.9687500020483810 ) ) ;
#20068=CARTESIAN_POINT ( 'NONE',  ( 5.405949406249999534, 9.363379034771803333, -38.78125000204838102 ) ) ;
#20070=CARTESIAN_POINT ( 'NONE',  ( 4.999999999999992006, -8.660254037844389075, -62.24999999999997158 ) ) ;
#20071=CARTESIAN_POINT ( 'NONE',  ( 10.81189881249999907, 6.242252689847868297, -130.4062500020483810 ) ) ;
#20075=CARTESIAN_POINT ( 'NONE',  ( -5.000000000000003553, -8.660254037844383745, -131.5000000000000000 ) ) ;
#20076=CARTESIAN_POINT ( 'NONE',  ( -4.999999999999996447, 8.660254037844387298, -105.3750000040967763 ) ) ;
#20077=CARTESIAN_POINT ( 'NONE',  ( -9.999999999999227285, -5.773502691896698735, -107.6249999999999574 ) ) ;
#20078=CARTESIAN_POINT ( 'NONE',  ( 5.405949406249999534, 9.363379034771803333, -65.59375000204836681 ) ) ;
#20079=EDGE_LOOP ( 'NONE', ( #12080, #12811, #39512, #18689 ) ) ;
#20084=CARTESIAN_POINT ( 'NONE',  ( 5.000000000000000000, 8.660254037844385522, -125.1250000040967620 ) ) ;
#20085=CARTESIAN_POINT ( 'NONE',  ( 9.999999999999996447, -5.773502691896262640, -32.50000000409675494 ) ) ;
#20087=CARTESIAN_POINT ( 'NONE',  ( -4.999999999999996447, 8.660254037844387298, -117.3750000040967905 ) ) ;
#20088=AXIS2_PLACEMENT_3D ( 'NONE', #23021, #19977, #6409 ) ;
#20090=DIRECTION ( 'NONE',  ( -0.000000000000000000, -0.000000000000000000, -1.000000000000000000 ) ) ;
#20092=ORIENTED_EDGE ( 'NONE', *, *, #38191, .T. ) ;
#20099=CARTESIAN_POINT ( 'NONE',  ( 9.999999999999998224, 0.000000000000000000, -144.8750000040967905 ) ) ;
#20101=CARTESIAN_POINT ( 'NONE',  ( 0.000000000000000000, 0.000000000000000000, -169.9999999999999716 ) ) ;
#20102=ADVANCED_FACE ( 'NONE', ( #36091 ), #26381, .F. ) ;
#20106=CARTESIAN_POINT ( 'NONE',  ( -5.000000000000003553, -8.660254037844383745, -119.5000000000000000 ) ) ;
#20107=CARTESIAN_POINT ( 'NONE',  ( -10.81189881249999907, -6.242252689847864744, -121.9687500020483952 ) ) ;
#20108=CARTESIAN_POINT ( 'NONE',  ( 5.405949406249992428, -9.363379034771808662, -132.2812500020483810 ) ) ;
#20110=CARTESIAN_POINT ( 'NONE',  ( 5.405949406249992428, -9.363379034771808662, -136.5937500020483810 ) ) ;
#20111=EDGE_CURVE ( 'NONE', #28436, #41907, #8905, .T. ) ;
#20113=CARTESIAN_POINT ( 'NONE',  ( -9.999999999999998224, 1.224646799147353059E-15, -141.1250000040967905 ) ) ;
#20114=CARTESIAN_POINT ( 'NONE',  ( 9.999999999999998224, 0.000000000000000000, -153.5000000000000000 ) ) ;
#20115=CARTESIAN_POINT ( 'NONE',  ( 5.405949406249992428, -9.363379034771808662, -0.2812500020483721386 ) ) ;
#20120=CARTESIAN_POINT ( 'NONE',  ( -10.81189881249999907, -6.242252689847864744, -51.46875000204837391 ) ) ;
#20122=CARTESIAN_POINT ( 'NONE',  ( 7.644554776091147741E-16, 12.48450537969573659, -162.9687500020483810 ) ) ;
#20125=DIRECTION ( 'NONE',  ( -0.000000000000000000, -0.000000000000000000, -1.000000000000000000 ) ) ;
#20126=CARTESIAN_POINT ( 'NONE',  ( -9.999999999999998224, 5.773502691896259087, -82.37499999999998579 ) ) ;
#20128=CARTESIAN_POINT ( 'NONE',  ( 5.405949406249992428, -9.363379034771808662, -109.7812500020483810 ) ) ;
#20129=CARTESIAN_POINT ( 'NONE',  ( -5.000000000000003553, -8.660254037844383745, -130.3750000040967905 ) ) ;
#20130=CARTESIAN_POINT ( 'NONE',  ( 0.000000000000000000, 0.000000000000000000, -99.99999999999998579 ) ) ;
#20135=CARTESIAN_POINT ( 'NONE',  ( 5.405949406249999534, 9.363379034771803333, -55.28125000204836681 ) ) ;
#20142=EDGE_CURVE ( 'NONE', #40993, #37069, #8653, .T. ) ;
#20154=CYLINDRICAL_SURFACE ( 'NONE', #438, 24.99999999999999645 ) ;
#20157=CARTESIAN_POINT ( 'NONE',  ( -10.81189881249999729, 1.324075727343319199E-15, -147.5937500020483810 ) ) ;
#20158=CARTESIAN_POINT ( 'NONE',  ( -10.81189881249999729, 1.324075727343319199E-15, -164.0937500020484094 ) ) ;
#20160=DIRECTION ( 'NONE',  ( -0.000000000000000000, -0.000000000000000000, -1.000000000000000000 ) ) ;
#20162=CARTESIAN_POINT ( 'NONE',  ( -2.121150477449813534E-15, -11.54700538379251284, -177.8750000000000284 ) ) ;
#20164=CARTESIAN_POINT ( 'NONE',  ( 5.000000000000000000, 8.660254037844385522, -151.7500000000000000 ) ) ;
#20166=DIRECTION ( 'NONE',  ( -1.000000000000000000, 0.000000000000000000, 0.000000000000000000 ) ) ;
#20167=CARTESIAN_POINT ( 'NONE',  ( -10.81189881249999729, 6.242252689847871849, -183.7187500020484379 ) ) ;
#20171=CARTESIAN_POINT ( 'NONE',  ( -10.81189881249999729, 6.242252689847871849, -54.90625000204837391 ) ) ;
#20173=CARTESIAN_POINT ( 'NONE',  ( -9.999999999999998224, 1.224646799147353059E-15, -115.2499999999999858 ) ) ;
#20175=CARTESIAN_POINT ( 'NONE',  ( -5.405949406250003975, -9.363379034771801557, -134.0312500020484094 ) ) ;
#20176=CARTESIAN_POINT ( 'NONE',  ( 10.81189881249999551, -6.242252689847874514, -147.1562500020484094 ) ) ;
#20178=CARTESIAN_POINT ( 'NONE',  ( -2.121150477449813534E-15, -11.54700538379251284, -125.3749999999999858 ) ) ;
#20179=CARTESIAN_POINT ( 'NONE',  ( -10.81189881249999729, 6.242252689847871849, -81.71875000204838102 ) ) ;
#20182=CARTESIAN_POINT ( 'NONE',  ( 7.644554776091147741E-16, 12.48450537969573659, -182.4687500020484094 ) ) ;
#20185=CARTESIAN_POINT ( 'NONE',  ( 9.999999999999998224, 0.000000000000000000, -158.0000000000000000 ) ) ;
#20186=CARTESIAN_POINT ( 'NONE',  ( 5.405949406249992428, -9.363379034771808662, -75.28125000204838102 ) ) ;
#20188=ADVANCED_FACE ( 'NONE', ( #35091 ), #25171, .F. ) ;
#20189=CARTESIAN_POINT ( 'NONE',  ( -5.000000000000003553, -8.660254037844383745, -55.37500000409675494 ) ) ;
#20190=CARTESIAN_POINT ( 'NONE',  ( -5.405949406249996869, 9.363379034771805109, -8.343750002048345493 ) ) ;
#20191=CARTESIAN_POINT ( 'NONE',  ( -9.999999999999998224, 1.224646799147353059E-15, -138.1250000040967620 ) ) ;
#20193=CARTESIAN_POINT ( 'NONE',  ( 10.81189881249999551, -6.242252689847874514, -7.656250002048365921 ) ) ;
#20195=CARTESIAN_POINT ( 'NONE',  ( 4.999999999999992006, -8.660254037844389075, -148.1250000040967905 ) ) ;
#20209=CARTESIAN_POINT ( 'NONE',  ( -9.999999999999998224, 1.224646799147353059E-15, -47.74999999999998579 ) ) ;
#20212=( BOUNDED_CURVE ( )  B_SPLINE_CURVE ( 2, ( #38803, #6005, #8816, #5576, #31708, #12247, #2768 ),
 .UNSPECIFIED., .F., .F. ) 
 B_SPLINE_CURVE_WITH_KNOTS ( ( 3, 2, 2, 3 ),
 ( 0.3544776119402986980, 0.3557213930348260278, 0.3569651741293533576, 0.3582089552238806873 ),
 .UNSPECIFIED. ) 
 CURVE ( )  GEOMETRIC_REPRESENTATION_ITEM ( )  RATIONAL_B_SPLINE_CURVE ( ( 0.9999999999999820144, 0.8660254037844566932, 1.000000000000000000, 0.8660254037844387076, 1.000000000000000000, 0.8660254037844267172, 1.000000000000011990 ) ) 
 REPRESENTATION_ITEM ( '' )  );
#20215=CARTESIAN_POINT ( 'NONE',  ( -5.405949406250003975, -9.363379034771801557, -150.5312500020483810 ) ) ;
#20221=CARTESIAN_POINT ( 'NONE',  ( -2.293366432827344421E-15, -12.48450537969573659, -70.71875000204838102 ) ) ;
#20222=CARTESIAN_POINT ( 'NONE',  ( 10.81189881249999907, 6.242252689847868297, -77.90625000204836681 ) ) ;
#20224=CARTESIAN_POINT ( 'NONE',  ( 5.405949406249992428, -9.363379034771808662, -162.2812500020484094 ) ) ;
#20225=CARTESIAN_POINT ( 'NONE',  ( 5.405949406249992428, -9.363379034771808662, -172.7812500020484094 ) ) ;
#20227=CARTESIAN_POINT ( 'NONE',  ( 0.000000000000000000, 0.000000000000000000, -99.99999999999998579 ) ) ;
#20228=CARTESIAN_POINT ( 'NONE',  ( -9.999999999999479527, -5.773502691896549521, -145.5000000040967905 ) ) ;
#20229=CARTESIAN_POINT ( 'NONE',  ( 9.999999999999998224, 1.224646799147353059E-15, -99.99999999999998579 ) ) ;
#20230=CARTESIAN_POINT ( 'NONE',  ( 5.405949406249999534, 9.363379034771803333, -107.5937500020483810 ) ) ;
#20232=CARTESIAN_POINT ( 'NONE',  ( 10.81189881249999551, -6.242252689847874514, -4.656250002048361480 ) ) ;
#20235=CARTESIAN_POINT ( 'NONE',  ( 10.81189881249999729, 0.000000000000000000, -102.0312500020483952 ) ) ;
#20238=CARTESIAN_POINT ( 'NONE',  ( 5.000000000000000000, 8.660254037844385522, -74.12500000409677625 ) ) ;
#20240=CARTESIAN_POINT ( 'NONE',  ( -5.405949406249996869, 9.363379034771805109, -32.34375000204836681 ) ) ;
#20243=CARTESIAN_POINT ( 'NONE',  ( -5.405949406249996869, 9.363379034771805109, -35.53125000204837391 ) ) ;
#20246=CARTESIAN_POINT ( 'NONE',  ( 9.999999999999996447, -5.773502691896262640, -11.50000000409676026 ) ) ;
#20249=CARTESIAN_POINT ( 'NONE',  ( 9.999999999999998224, 0.000000000000000000, -155.3750000040967905 ) ) ;
#20253=ORIENTED_EDGE ( 'NONE', *, *, #19927, .T. ) ;
#20258=B_SPLINE_CURVE_WITH_KNOTS ( 'NONE', 3,
 ( #6328, #3086, #29415, #2878, #283, #23580, #29203, #42343, #68, #12774, #25967, #39118 ),
 .UNSPECIFIED., .F., .F.,
 ( 4, 2, 2, 2, 2, 4 ),
 ( 4.983255971813266780E-16, 0.002144051117877383752, 0.004288102235754269638, 0.005360127794692712798, 0.006432153353631154223, 0.008576204471508041410 ),
 .UNSPECIFIED. ) ;
#20264=CARTESIAN_POINT ( 'NONE',  ( -10.81189881249999907, -6.242252689847864744, -176.1562500020483810 ) ) ;
#20267=CARTESIAN_POINT ( 'NONE',  ( 5.405949406249992428, -9.363379034771808662, -90.09375000204838102 ) ) ;
#20269=CARTESIAN_POINT ( 'NONE',  ( 7.644554776091147741E-16, 12.48450537969573659, -98.65625000204838102 ) ) ;
#20271=CARTESIAN_POINT ( 'NONE',  ( -10.81189881249999729, 1.324075727343319199E-15, -113.0937500020483810 ) ) ;
#20274=CARTESIAN_POINT ( 'NONE',  ( -9.999999999999998224, 1.224646799147353059E-15, -105.1250000040967763 ) ) ;
#20276=CARTESIAN_POINT ( 'NONE',  ( -5.405949406250003975, -9.363379034771801557, -197.0312500020484094 ) ) ;
#20279=CARTESIAN_POINT ( 'NONE',  ( -2.121150477449813534E-15, -11.54700538379251284, -170.7500000040967620 ) ) ;
#20281=CARTESIAN_POINT ( 'NONE',  ( 10.81189881249999551, -6.242252689847874514, -20.96875000204837036 ) ) ;
#20282=CARTESIAN_POINT ( 'NONE',  ( -2.293366432827344421E-15, -12.48450537969573659, -130.7187500020483810 ) ) ;
#20284=CARTESIAN_POINT ( 'NONE',  ( 10.81189881249999907, 6.242252689847868297, -26.90625000204838813 ) ) ;
#20285=CARTESIAN_POINT ( 'NONE',  ( -4.999999999999996447, 8.660254037844387298, -102.0000000000000000 ) ) ;
#20286=CARTESIAN_POINT ( 'NONE',  ( 9.999999999999996447, -5.773502691896262640, -60.62499999999998579 ) ) ;
#20287=CARTESIAN_POINT ( 'NONE',  ( -5.405949406249996869, 9.363379034771805109, -131.5312500020484094 ) ) ;
#20291=CARTESIAN_POINT ( 'NONE',  ( -2.121150477449813534E-15, -11.54700538379251284, -110.7500000040967763 ) ) ;
#20292=CARTESIAN_POINT ( 'NONE',  ( 5.405949406249999534, 9.363379034771803333, -62.59375000204836681 ) ) ;
#20297=CARTESIAN_POINT ( 'NONE',  ( -2.121150477449813534E-15, -11.54700538379251284, -35.75000000409675494 ) ) ;
#20298=DIRECTION ( 'NONE',  ( -0.000000000000000000, -0.000000000000000000, -1.000000000000000000 ) ) ;
#20301=DIRECTION ( 'NONE',  ( -0.000000000000000000, -0.000000000000000000, -1.000000000000000000 ) ) ;
#20303=VERTEX_POINT ( 'NONE', #21911 ) ;
#20304=CARTESIAN_POINT ( 'NONE',  ( -9.999999999999998224, 0.000000000000000000, -99.99999999999998579 ) ) ;
#20307=CARTESIAN_POINT ( 'NONE',  ( -5.405949406250003975, -9.363379034771801557, -198.5312500020484094 ) ) ;
#20313=CARTESIAN_POINT ( 'NONE',  ( -10.81189881249999729, 1.324075727343319199E-15, -120.5937500020483952 ) ) ;
#20314=CARTESIAN_POINT ( 'NONE',  ( 10.81189881249999729, 0.000000000000000000, 0.1562499979516351889 ) ) ;
#20315=CARTESIAN_POINT ( 'NONE',  ( 10.81189881249999551, -6.242252689847874514, -126.1562500020483810 ) ) ;
#20317=CARTESIAN_POINT ( 'NONE',  ( -10.81189881249999729, 1.324075727343319199E-15, -141.5937500020483810 ) ) ;
#20320=CARTESIAN_POINT ( 'NONE',  ( 9.999999999999996447, -5.773502691896262640, -153.6250000000000284 ) ) ;
#20321=CARTESIAN_POINT ( 'NONE',  ( 5.000000000000000000, 8.660254037844385522, -19.74999999999996092 ) ) ;
#20325=CARTESIAN_POINT ( 'NONE',  ( 10.81189881249999907, 6.242252689847868297, -50.71875000204837391 ) ) ;
#20327=CARTESIAN_POINT ( 'NONE',  ( 7.644554776091147741E-16, 12.48450537969573659, -153.9687500020484094 ) ) ;
#20330=CARTESIAN_POINT ( 'NONE',  ( 10.28326034709391834, 3.150834530142504697, -180.0000000000000853 ) ) ;
#20332=CARTESIAN_POINT ( 'NONE',  ( -9.999999999999998224, 1.224646799147353059E-15, -82.24999999999998579 ) ) ;
#20334=( BOUNDED_CURVE ( )  B_SPLINE_CURVE ( 2, ( #6767, #36757, #3115, #9791, #22970, #13429, #36126 ),
 .UNSPECIFIED., .F., .F. ) 
 B_SPLINE_CURVE_WITH_KNOTS ( ( 3, 2, 2, 3 ),
 ( 0.1268656716417910224, 0.1281094527363183799, 0.1293532338308457652, 0.1305970149253731227 ),
 .UNSPECIFIED. ) 
 CURVE ( )  GEOMETRIC_REPRESENTATION_ITEM ( )  RATIONAL_B_SPLINE_CURVE ( ( 1.000000000000003109, 0.8660254037844358210, 1.000000000000000000, 0.8660254037844387076, 1.000000000000000000, 0.8660254037844387076, 1.000000000000000000 ) ) 
 REPRESENTATION_ITEM ( '' )  );
#20335=ORIENTED_EDGE ( 'NONE', *, *, #38191, .F. ) ;
#20336=CARTESIAN_POINT ( 'NONE',  ( 10.81189881249999551, -6.242252689847874514, -106.6562500020484094 ) ) ;
#20337=CARTESIAN_POINT ( 'NONE',  ( -4.999999999999996447, 8.660254037844387298, -135.3750000040967905 ) ) ;
#20341=CARTESIAN_POINT ( 'NONE',  ( -5.405949406250003975, -9.363379034771801557, -54.53125000204836681 ) ) ;
#20347=EDGE_CURVE ( 'NONE', #10534, #24567, #38742, .T. ) ;
#20355=ORIENTED_EDGE ( 'NONE', *, *, #23820, .T. ) ;
#20363=CARTESIAN_POINT ( 'NONE',  ( -5.405949406249996869, 9.363379034771805109, -150.8437500020483810 ) ) ;
#20364=CARTESIAN_POINT ( 'NONE',  ( 5.405949406249999534, 9.363379034771803333, -160.0937500020484094 ) ) ;
#20367=CARTESIAN_POINT ( 'NONE',  ( 9.999999999999996447, -5.773502691896262640, -180.6250000000000284 ) ) ;
#20369=CARTESIAN_POINT ( 'NONE',  ( 9.999999999999479527, 5.773502691896553074, -151.8749999999999716 ) ) ;
#20372=CARTESIAN_POINT ( 'NONE',  ( 10.81189881249999729, 0.000000000000000000, -187.3437500020483810 ) ) ;
#20375=CARTESIAN_POINT ( 'NONE',  ( -10.81189881249999729, 6.242252689847871849, -48.90625000204836681 ) ) ;
#20377=CARTESIAN_POINT ( 'NONE',  ( -4.999999999999996447, 8.660254037844387298, -109.4999999999999858 ) ) ;
#20379=CARTESIAN_POINT ( 'NONE',  ( 5.405949406249992428, -9.363379034771808662, -130.7812500020483810 ) ) ;
#20380=CARTESIAN_POINT ( 'NONE',  ( -2.293366432827344421E-15, -12.48450537969573659, -150.4062500020483810 ) ) ;
#20382=CARTESIAN_POINT ( 'NONE',  ( 10.81189881249999729, 0.000000000000000000, -82.34375000204836681 ) ) ;
#20385=CARTESIAN_POINT ( 'NONE',  ( -2.293366432827344421E-15, -12.48450537969573659, -183.2187500020484094 ) ) ;
#20389=CARTESIAN_POINT ( 'NONE',  ( 10.81189881249999551, -6.242252689847874514, -75.15625000204838102 ) ) ;
#20392=CARTESIAN_POINT ( 'NONE',  ( 9.999999999999996447, -5.773502691896262640, -53.50000000409677625 ) ) ;
#20393=CARTESIAN_POINT ( 'NONE',  ( 10.81189881249999729, 0.000000000000000000, -7.343750002048343717 ) ) ;
#20396=CARTESIAN_POINT ( 'NONE',  ( 5.405949406249992428, -9.363379034771808662, -3.281250002048374803 ) ) ;
#20400=AXIS2_PLACEMENT_3D ( 'NONE', #42079, #15532, #9080 ) ;
#20401=CYLINDRICAL_SURFACE ( 'NONE', #31159, 9.999999999999998224 ) ;
#20409=CARTESIAN_POINT ( 'NONE',  ( 9.999999999999998224, 0.000000000000000000, -153.5000000000000000 ) ) ;
#20418=CARTESIAN_POINT ( 'NONE',  ( 7.070501591499377789E-16, 11.54700538379251284, -48.12499999999997158 ) ) ;
#20425=DIRECTION ( 'NONE',  ( -0.000000000000000000, -0.000000000000000000, -1.000000000000000000 ) ) ;
#20428=CARTESIAN_POINT ( 'NONE',  ( 9.999999999999998224, 0.000000000000000000, -140.3750000040967905 ) ) ;
#20430=CARTESIAN_POINT ( 'NONE',  ( 9.999999999999872102, 5.773502691896329253, -161.2500000040967905 ) ) ;
#20433=CARTESIAN_POINT ( 'NONE',  ( -10.81189881249999729, 1.324075727343319199E-15, -72.59375000204838102 ) ) ;
#20434=CARTESIAN_POINT ( 'NONE',  ( -10.81189881249999729, 6.242252689847871849, -72.90625000204838102 ) ) ;
#20436=CARTESIAN_POINT ( 'NONE',  ( 10.81189881249999551, -6.242252689847874514, -157.6562500020484094 ) ) ;
#20437=CARTESIAN_POINT ( 'NONE',  ( 10.81189881249999907, 6.242252689847868297, -169.4062500020484094 ) ) ;
#20438=FACE_OUTER_BOUND ( 'NONE', #35603, .T. ) ;
#20439=FACE_OUTER_BOUND ( 'NONE', #1973, .T. ) ;
#20440=CARTESIAN_POINT ( 'NONE',  ( -10.81189881249999729, 6.242252689847871849, -108.7187500020483810 ) ) ;
#20443=CARTESIAN_POINT ( 'NONE',  ( 5.405949406249992428, -9.363379034771808662, -6.281250002048377468 ) ) ;
#20445=CARTESIAN_POINT ( 'NONE',  ( -2.293366432827344421E-15, -12.48450537969573659, -102.4062500020483952 ) ) ;
#20447=CARTESIAN_POINT ( 'NONE',  ( -9.999999999999998224, 1.224646799147353059E-15, -75.12500000409677625 ) ) ;
#20449=CARTESIAN_POINT ( 'NONE',  ( 10.81189881249999551, -6.242252689847874514, -34.46875000204835260 ) ) ;
#20452=CARTESIAN_POINT ( 'NONE',  ( -10.81189881249999729, 1.324075727343319199E-15, -26.28125000204836681 ) ) ;
#20455=CARTESIAN_POINT ( 'NONE',  ( -4.999999999999996447, 8.660254037844387298, -6.375000004096770034 ) ) ;
#20458=CARTESIAN_POINT ( 'NONE',  ( -9.999999999999998224, 1.224646799147353059E-15, -122.7500000000000000 ) ) ;
#20460=VERTEX_POINT ( 'NONE', #36711 ) ;
#20470=ORIENTED_EDGE ( 'NONE', *, *, #30448, .F. ) ;
#20473=( BOUNDED_CURVE ( )  B_SPLINE_CURVE ( 2, ( #39875, #206, #33216, #10308, #23496, #13740, #26930 ),
 .UNSPECIFIED., .F., .F. ) 
 B_SPLINE_CURVE_WITH_KNOTS ( ( 3, 2, 2, 3 ),
 ( 0.3208955223880597396, 0.3221393034825871804, 0.3233830845771145657, 0.3246268656716419510 ),
 .UNSPECIFIED. ) 
 CURVE ( )  GEOMETRIC_REPRESENTATION_ITEM ( )  RATIONAL_B_SPLINE_CURVE ( ( 0.9999999999999940048, 0.8660254037844447028, 1.000000000000000000, 0.8660254037844387076, 1.000000000000000000, 0.8660254037844207220, 1.000000000000017986 ) ) 
 REPRESENTATION_ITEM ( '' )  );
#20474=CARTESIAN_POINT ( 'NONE',  ( -10.81189881249999729, 1.324075727343319199E-15, -171.7812500020484094 ) ) ;
#20477=CARTESIAN_POINT ( 'NONE',  ( -10.81189881249999729, 6.242252689847871849, -96.71875000204838102 ) ) ;
#20479=CARTESIAN_POINT ( 'NONE',  ( -5.405949406249996869, 9.363379034771805109, -101.5312500020483952 ) ) ;
#20481=CARTESIAN_POINT ( 'NONE',  ( -5.405949406250003975, -9.363379034771801557, -108.3437500020483810 ) ) ;
#20484=CARTESIAN_POINT ( 'NONE',  ( 10.00000000000000000, 5.773502691896255534, -132.7500000040967905 ) ) ;
#20485=CARTESIAN_POINT ( 'NONE',  ( -10.81189881249999729, 1.324075727343319199E-15, -198.7812500020484094 ) ) ;
#20488=CARTESIAN_POINT ( 'NONE',  ( 5.000000000000000000, 8.660254037844385522, -173.1250000040968189 ) ) ;
#20490=CARTESIAN_POINT ( 'NONE',  ( 5.405949406249999534, 9.363379034771803333, -25.09375000204835970 ) ) ;
#20492=CARTESIAN_POINT ( 'NONE',  ( 10.81189881249999729, 0.000000000000000000, -133.3437500020484094 ) ) ;
#20494=CARTESIAN_POINT ( 'NONE',  ( -5.405949406249996869, 9.363379034771805109, -29.53125000204837036 ) ) ;
#20496=CARTESIAN_POINT ( 'NONE',  ( 9.999999999999996447, -5.773502691896262640, -57.62499999999998579 ) ) ;
#20497=CARTESIAN_POINT ( 'NONE',  ( 10.81189881249999729, 0.000000000000000000, -127.5312500020483952 ) ) ;
#20501=CARTESIAN_POINT ( 'NONE',  ( -9.999999999999998224, 5.773502691896259087, -102.2500000040967763 ) ) ;
#20502=CARTESIAN_POINT ( 'NONE',  ( 7.070501591499376803E-16, 11.54700538379251284, -101.0000000040967905 ) ) ;
#20503=CARTESIAN_POINT ( 'NONE',  ( -10.81189881249999729, 1.324075727343319199E-15, -54.59375000204835970 ) ) ;
#20508=DIRECTION ( 'NONE',  ( -0.000000000000000000, -0.000000000000000000, -1.000000000000000000 ) ) ;
#20509=CARTESIAN_POINT ( 'NONE',  ( -9.999999999999998224, 5.773502691896259087, -39.25000000409676204 ) ) ;
#20510=CARTESIAN_POINT ( 'NONE',  ( 7.070501591499376803E-16, 11.54700538379251284, -152.0000000040967905 ) ) ;
#20512=DIRECTION ( 'NONE',  ( -0.000000000000000000, -0.000000000000000000, -1.000000000000000000 ) ) ;
#20514=ORIENTED_EDGE ( 'NONE', *, *, #5893, .T. ) ;
#20518=CARTESIAN_POINT ( 'NONE',  ( 5.405949406249999534, 9.363379034771803333, -196.2812500020484094 ) ) ;
#20524=CARTESIAN_POINT ( 'NONE',  ( 5.405949406249999534, 9.363379034771803333, -118.0937500020483810 ) ) ;
#20525=CARTESIAN_POINT ( 'NONE',  ( 5.000000000000000000, 8.660254037844385522, -194.1250000040967905 ) ) ;
#20526=CARTESIAN_POINT ( 'NONE',  ( -5.405949406249996869, 9.363379034771805109, -128.5312500020484094 ) ) ;
#20528=CARTESIAN_POINT ( 'NONE',  ( -5.405949406249996869, 9.363379034771805109, -126.8437500020483952 ) ) ;
#20529=EDGE_CURVE ( 'NONE', #22548, #14748, #25794, .T. ) ;
#20532=CARTESIAN_POINT ( 'NONE',  ( 9.999999999999998224, 0.000000000000000000, -155.0000000000000000 ) ) ;
#20533=CARTESIAN_POINT ( 'NONE',  ( 9.999999999999998224, 0.000000000000000000, -18.49999999999996092 ) ) ;
#20536=CARTESIAN_POINT ( 'NONE',  ( 9.999999999999998224, 0.000000000000000000, -170.0000000000000000 ) ) ;
#20538=CARTESIAN_POINT ( 'NONE',  ( -10.81189881249999729, 6.242252689847871849, -44.21875000204836681 ) ) ;
#20540=CARTESIAN_POINT ( 'NONE',  ( -2.293366432827344421E-15, -12.48450537969573659, -150.2187500020483810 ) ) ;
#20544=CARTESIAN_POINT ( 'NONE',  ( 0.6533489177094430334, 10.23204748536553588, -179.9999999999998863 ) ) ;
#20545=CARTESIAN_POINT ( 'NONE',  ( -9.999999999999998224, 5.773502691896259087, -85.37499999999997158 ) ) ;
#20547=ORIENTED_EDGE ( 'NONE', *, *, #30982, .F. ) ;
#20548=CARTESIAN_POINT ( 'NONE',  ( -10.81189881249999729, -6.242252689847864744, -111.6562500020483952 ) ) ;
#20549=CARTESIAN_POINT ( 'NONE',  ( 7.070501591499377789E-16, 11.54700538379251284, -128.0000000040967620 ) ) ;
#20553=CARTESIAN_POINT ( 'NONE',  ( -5.405949406249996869, 9.363379034771805109, -55.03125000204836681 ) ) ;
#20560=CARTESIAN_POINT ( 'NONE',  ( 9.999999999999548805, 5.773502691896514882, -177.3749999999999716 ) ) ;
#20570=CARTESIAN_POINT ( 'NONE',  ( 0.000000000000000000, 0.000000000000000000, -99.99999999999998579 ) ) ;
#20573=CARTESIAN_POINT ( 'NONE',  ( 10.81189881249999551, -6.242252689847874514, -140.9687500020483810 ) ) ;
#20575=CARTESIAN_POINT ( 'NONE',  ( 5.405949406249999534, 9.363379034771803333, -158.5937500020483810 ) ) ;
#20578=CARTESIAN_POINT ( 'NONE',  ( -5.000000000000003553, -8.660254037844383745, -176.5000000000000000 ) ) ;
#20582=CARTESIAN_POINT ( 'NONE',  ( 10.00000000000025402, -5.773502691896113426, -124.0000000040967620 ) ) ;
#20584=CARTESIAN_POINT ( 'NONE',  ( -10.81189881249999729, 1.324075727343319199E-15, -180.5937500020484094 ) ) ;
#20588=CARTESIAN_POINT ( 'NONE',  ( -10.81189881249999907, -6.242252689847864744, -53.15625000204837391 ) ) ;
#20590=CARTESIAN_POINT ( 'NONE',  ( 4.999999999999992006, -8.660254037844389075, -108.7499999999999858 ) ) ;
#20592=CARTESIAN_POINT ( 'NONE',  ( 5.405949406249999534, 9.363379034771803333, -131.7812500020483810 ) ) ;
#20593=CARTESIAN_POINT ( 'NONE',  ( -9.999999999999998224, 5.773502691896259087, -157.7500000040967905 ) ) ;
#20594=CARTESIAN_POINT ( 'NONE',  ( -10.81189881249999729, 6.242252689847871849, -150.9062500020484094 ) ) ;
#20595=AXIS2_PLACEMENT_3D ( 'NONE', #27351, #40486, #7716 ) ;
#20597=CARTESIAN_POINT ( 'NONE',  ( 5.405949406249992428, -9.363379034771808662, -81.09375000204838102 ) ) ;
#20600=CARTESIAN_POINT ( 'NONE',  ( -10.81189881249999907, -6.242252689847864744, -178.9687500020484094 ) ) ;
#20604=CARTESIAN_POINT ( 'NONE',  ( -10.81189881249999907, -6.242252689847864744, -72.65625000204836681 ) ) ;
#20606=CARTESIAN_POINT ( 'NONE',  ( 10.00000000000000000, 5.773502691896255534, -48.75000000409676204 ) ) ;
#20608=CARTESIAN_POINT ( 'NONE',  ( -10.81189881249999907, -6.242252689847864744, -6.468750002048357040 ) ) ;
#20611=CARTESIAN_POINT ( 'NONE',  ( -5.405949406249996869, 9.363379034771805109, -4.031250002048375691 ) ) ;
#20613=CARTESIAN_POINT ( 'NONE',  ( -2.121150477449813534E-15, -11.54700538379251284, -148.2500000040968189 ) ) ;
#20617=ORIENTED_EDGE ( 'NONE', *, *, #42299, .F. ) ;
#20627=CARTESIAN_POINT ( 'NONE',  ( -10.00000000000000000, -5.773502691896251982, -43.12499999999997158 ) ) ;
#20629=CARTESIAN_POINT ( 'NONE',  ( -10.81189881249999729, 1.324075727343319199E-15, -164.0937500020484094 ) ) ;
#20630=CARTESIAN_POINT ( 'NONE',  ( 9.999999999999998224, 0.000000000000000000, -119.0000000000000000 ) ) ;
#20641=CARTESIAN_POINT ( 'NONE',  ( 5.405949406249999534, 9.363379034771803333, -71.59375000204836681 ) ) ;
#20643=CARTESIAN_POINT ( 'NONE',  ( 10.81189881249999729, 0.000000000000000000, -78.03125000204838102 ) ) ;
#20646=CARTESIAN_POINT ( 'NONE',  ( -5.405949406249996869, 9.363379034771805109, -158.5312500020484094 ) ) ;
#20647=CARTESIAN_POINT ( 'NONE',  ( -5.405949406249996869, 9.363379034771805109, -172.0312500020484094 ) ) ;
#20648=CARTESIAN_POINT ( 'NONE',  ( -5.405949406249996869, 9.363379034771805109, 0.6562499979516356330 ) ) ;
#20650=CARTESIAN_POINT ( 'NONE',  ( -10.81189881249999907, -6.242252689847864744, -108.4687500020483810 ) ) ;
#20652=CARTESIAN_POINT ( 'NONE',  ( -10.81189881249999729, 6.242252689847871849, -6.906250002048365033 ) ) ;
#20656=CARTESIAN_POINT ( 'NONE',  ( 5.405949406249992428, -9.363379034771808662, -103.7812500020483810 ) ) ;
#20658=CARTESIAN_POINT ( 'NONE',  ( -9.999999999999998224, 5.773502691896259087, -78.25000000409677625 ) ) ;
#20660=CARTESIAN_POINT ( 'NONE',  ( -5.405949406250003975, -9.363379034771801557, -33.34375000204836681 ) ) ;
#20663=CARTESIAN_POINT ( 'NONE',  ( 10.81189881249999729, 0.000000000000000000, -28.53125000204837036 ) ) ;
#20666=EDGE_CURVE ( 'NONE', #38366, #27040, #7368, .T. ) ;
#20667=CARTESIAN_POINT ( 'NONE',  ( -9.999999999999998224, 5.773502691896259087, -6.250000004096755823 ) ) ;
#20671=LINE ( 'NONE', #17423, #38570 ) ;
#20673=ORIENTED_EDGE ( 'NONE', *, *, #40453, .F. ) ;
#20683=CARTESIAN_POINT ( 'NONE',  ( -9.999999999999998224, 1.224646799147353059E-15, -136.2499999999999716 ) ) ;
#20684=EDGE_CURVE ( 'NONE', #9826, #6419, #10007, .T. ) ;
#20686=CARTESIAN_POINT ( 'NONE',  ( 10.81189881249999907, 6.242252689847868297, -173.9062500020484094 ) ) ;
#20688=VECTOR ( 'NONE', #39469, 1000.000000000000000 ) ;
#20690=CARTESIAN_POINT ( 'NONE',  ( -5.405949406249996869, 9.363379034771805109, -95.34375000204838102 ) ) ;
#20691=DIRECTION ( 'NONE',  ( 0.000000000000000000, 0.000000000000000000, -1.000000000000000000 ) ) ;
#20692=CARTESIAN_POINT ( 'NONE',  ( 10.81189881249999729, 0.000000000000000000, -102.0312500020483952 ) ) ;
#20694=CARTESIAN_POINT ( 'NONE',  ( 5.405949406249999534, 9.363379034771803333, -109.0937500020483810 ) ) ;
#20698=CARTESIAN_POINT ( 'NONE',  ( 10.81189881249999907, 6.242252689847868297, -196.4062500020484379 ) ) ;
#20701=CARTESIAN_POINT ( 'NONE',  ( -5.000000000000003553, -8.660254037844383745, -173.8750000040968189 ) ) ;
#20703=CARTESIAN_POINT ( 'NONE',  ( 5.405949406249999534, 9.363379034771803333, -19.09375000204835260 ) ) ;
#20705=CARTESIAN_POINT ( 'NONE',  ( -10.81189881249999729, 1.324075727343319199E-15, -132.5937500020483810 ) ) ;
#20707=CARTESIAN_POINT ( 'NONE',  ( 7.644554776091147741E-16, 12.48450537969573659, -28.15625000204838102 ) ) ;
#20709=CARTESIAN_POINT ( 'NONE',  ( -9.999999999999998224, 1.224646799147353059E-15, -152.7500000000000000 ) ) ;
#20710=CARTESIAN_POINT ( 'NONE',  ( 9.999999999999996447, -5.773502691896262640, -62.12499999999998579 ) ) ;
#20711=CARTESIAN_POINT ( 'NONE',  ( -10.81189881249999907, -6.242252689847864744, -120.6562500020483810 ) ) ;
#20714=CARTESIAN_POINT ( 'NONE',  ( -4.999999999999996447, 8.660254037844387298, -100.8750000040967905 ) ) ;
#20716=CARTESIAN_POINT ( 'NONE',  ( -10.81189881249999729, 1.324075727343319199E-15, -56.09375000204835970 ) ) ;
#20723=CARTESIAN_POINT ( 'NONE',  ( 10.00000000000000000, 5.773502691896255534, -27.75000000409677625 ) ) ;
#20733=CARTESIAN_POINT ( 'NONE',  ( 0.000000000000000000, 0.000000000000000000, -99.99999999999998579 ) ) ;
#20736=CARTESIAN_POINT ( 'NONE',  ( -10.81189881249999907, -6.242252689847864744, -194.1562500020484094 ) ) ;
#20742=CARTESIAN_POINT ( 'NONE',  ( -10.81189881249999729, 6.242252689847871849, -117.7187500020483952 ) ) ;
#20743=CARTESIAN_POINT ( 'NONE',  ( -10.00000000000000000, -5.773502691896251982, -198.0000000040968189 ) ) ;
#20744=CARTESIAN_POINT ( 'NONE',  ( -10.81189881249999729, 6.242252689847871849, -128.4062500020484094 ) ) ;
#20747=CARTESIAN_POINT ( 'NONE',  ( 10.81189881249999729, 0.000000000000000000, -128.8437500020484094 ) ) ;
#20750=CARTESIAN_POINT ( 'NONE',  ( -9.999999999999998224, 1.224646799147353059E-15, -154.2500000000000000 ) ) ;
#20751=CARTESIAN_POINT ( 'NONE',  ( 7.070501591499377789E-16, 11.54700538379251284, -21.12499999999997513 ) ) ;
#20756=CARTESIAN_POINT ( 'NONE',  ( 5.405949406249992428, -9.363379034771808662, -42.09375000204837391 ) ) ;
#20758=CARTESIAN_POINT ( 'NONE',  ( 10.81189881249999907, 6.242252689847868297, -154.2187500020483810 ) ) ;
#20762=CARTESIAN_POINT ( 'NONE',  ( -9.999999999999998224, 5.773502691896259087, -80.87499999999998579 ) ) ;
#20765=CARTESIAN_POINT ( 'NONE',  ( -6.058704384512919816, 8.986510772356837151, -100.0161565621822319 ) ) ;
#20766=CARTESIAN_POINT ( 'NONE',  ( 9.999999999999998224, 0.000000000000000000, -123.8750000040967905 ) ) ;
#20768=ADVANCED_FACE ( 'NONE', ( #14234 ), #17484, .F. ) ;
#20770=CARTESIAN_POINT ( 'NONE',  ( -9.999999999999998224, 0.000000000000000000, -99.99999999999998579 ) ) ;
#20771=CARTESIAN_POINT ( 'NONE',  ( 5.405949406249999534, 9.363379034771803333, -52.28125000204835970 ) ) ;
#20776=CARTESIAN_POINT ( 'NONE',  ( -9.999999999999998224, 1.224646799147353059E-15, -163.6250000040967905 ) ) ;
#20777=ORIENTED_EDGE ( 'NONE', *, *, #30448, .T. ) ;
#20778=ADVANCED_FACE ( 'NONE', ( #18134 ), #40571, .F. ) ;
#20789=( BOUNDED_CURVE ( )  B_SPLINE_CURVE ( 2, ( #18918, #26454, #32101, #22371, #2534, #16287, #19329 ),
 .UNSPECIFIED., .F., .F. ) 
 B_SPLINE_CURVE_WITH_KNOTS ( ( 3, 2, 2, 3 ),
 ( 0.1716417910447761430, 0.1728855721393035005, 0.1741293532338308858, 0.1753731343283582433 ),
 .UNSPECIFIED. ) 
 CURVE ( )  GEOMETRIC_REPRESENTATION_ITEM ( )  RATIONAL_B_SPLINE_CURVE ( ( 0.9999999999999970024, 0.8660254037844417052, 1.000000000000000000, 0.8660254037844387076, 1.000000000000000000, 0.8660254037844357100, 1.000000000000003109 ) ) 
 REPRESENTATION_ITEM ( '' )  );
#20791=CARTESIAN_POINT ( 'NONE',  ( -10.81189881249999729, 6.242252689847871849, -141.7187500020483810 ) ) ;
#20792=CARTESIAN_POINT ( 'NONE',  ( 7.644554776091147741E-16, 12.48450537969573659, -152.4687500020484094 ) ) ;
#20795=CARTESIAN_POINT ( 'NONE',  ( 10.00000000000000000, 5.773502691896255534, -183.3750000000000000 ) ) ;
#20800=CARTESIAN_POINT ( 'NONE',  ( -5.405949406249996869, 9.363379034771805109, -177.8437500020483810 ) ) ;
#20803=CARTESIAN_POINT ( 'NONE',  ( -10.00000000000076916, 5.773502691895813221, -115.3749999999999716 ) ) ;
#20804=CARTESIAN_POINT ( 'NONE',  ( -10.81189881249999907, -6.242252689847864744, -56.15625000204838102 ) ) ;
#20806=CARTESIAN_POINT ( 'NONE',  ( 9.999999999999998224, 0.000000000000000000, -106.9999999999999858 ) ) ;
#20807=CIRCLE ( 'NONE', #27048, 31.99999999999997158 ) ;
#20808=EDGE_CURVE ( 'NONE', #40108, #31308, #30677, .T. ) ;
#20810=CARTESIAN_POINT ( 'NONE',  ( 10.81189881249999729, 6.242252689847867408, -131.9062500020483810 ) ) ;
#20811=CARTESIAN_POINT ( 'NONE',  ( -9.999999999999998224, 5.773502691896259087, -148.7500000040967905 ) ) ;
#20812=CARTESIAN_POINT ( 'NONE',  ( 10.81189881249999729, 0.000000000000000000, -148.5312500020483810 ) ) ;
#20816=CARTESIAN_POINT ( 'NONE',  ( 5.405949406249992428, -9.363379034771808662, -178.5937500020484094 ) ) ;
#20820=CARTESIAN_POINT ( 'NONE',  ( 5.405949406249999534, 9.363379034771803333, -77.78125000204838102 ) ) ;
#20822=CARTESIAN_POINT ( 'NONE',  ( 5.000000000000000000, 8.660254037844385522, -56.12500000409676204 ) ) ;
#20823=CARTESIAN_POINT ( 'NONE',  ( -10.81189881249999729, 6.242252689847871849, -9.718750002048361480 ) ) ;
#20827=CARTESIAN_POINT ( 'NONE',  ( 5.405949406249999534, 9.363379034771803333, -4.281250002048375691 ) ) ;
#20829=CARTESIAN_POINT ( 'NONE',  ( 9.999999999999742428, 5.773502691896404748, -138.7500000040967905 ) ) ;
#20846=CARTESIAN_POINT ( 'NONE',  ( 9.999999999999998224, 0.000000000000000000, -45.49999999999998579 ) ) ;
#20848=CARTESIAN_POINT ( 'NONE',  ( -5.405949406249996869, 9.363379034771805109, -165.8437500020484094 ) ) ;
#20849=CARTESIAN_POINT ( 'NONE',  ( 10.81189881249999729, 6.242252689847867408, -175.2187500020484094 ) ) ;
#20850=LINE ( 'NONE', #31012, #13609 ) ;
#20851=DIRECTION ( 'NONE',  ( -0.000000000000000000, -0.000000000000000000, -1.000000000000000000 ) ) ;
#20852=CARTESIAN_POINT ( 'NONE',  ( 9.999999999999742428, 5.773502691896404748, -126.3749999999999858 ) ) ;
#20853=CARTESIAN_POINT ( 'NONE',  ( -4.999999999999996447, 8.660254037844387298, -199.5000000000000000 ) ) ;
#20858=CARTESIAN_POINT ( 'NONE',  ( -2.293366432827344421E-15, -12.48450537969573659, -69.21875000204839523 ) ) ;
#20859=CARTESIAN_POINT ( 'NONE',  ( -5.405949406250003975, -9.363379034771801557, -77.03125000204838102 ) ) ;
#20861=CARTESIAN_POINT ( 'NONE',  ( 10.00000000000000000, 5.773502691896255534, -135.3750000000000000 ) ) ;
#20862=CARTESIAN_POINT ( 'NONE',  ( 5.405949406249992428, -9.363379034771808662, -160.7812500020484094 ) ) ;
#20863=CARTESIAN_POINT ( 'NONE',  ( 10.81189881249999551, -6.242252689847874514, -174.1562500020484094 ) ) ;
#20866=CARTESIAN_POINT ( 'NONE',  ( 7.644554776091147741E-16, 12.48450537969573659, -105.9687500020483668 ) ) ;
#20869=CARTESIAN_POINT ( 'NONE',  ( 10.81189881249999907, 6.242252689847868297, -1.406250002048359260 ) ) ;
#20871=CARTESIAN_POINT ( 'NONE',  ( 5.405949406249999534, 9.363379034771803333, -98.78125000204839523 ) ) ;
#20873=CARTESIAN_POINT ( 'NONE',  ( 9.999999999999996447, -5.773502691896262640, -76.00000000409677625 ) ) ;
#20875=CARTESIAN_POINT ( 'NONE',  ( 7.644554776091147741E-16, 12.48450537969573659, -32.46875000204835260 ) ) ;
#20876=VERTEX_POINT ( 'NONE', #40998 ) ;
#20878=CARTESIAN_POINT ( 'NONE',  ( 5.405949406249999534, 9.363379034771803333, -29.78125000204837036 ) ) ;
#20880=CARTESIAN_POINT ( 'NONE',  ( 4.999999999999992006, -8.660254037844389075, -118.1250000040967905 ) ) ;
#20881=CARTESIAN_POINT ( 'NONE',  ( -4.999999999999996447, 8.660254037844387298, -0.3750000040967649273 ) ) ;
#20884=DIRECTION ( 'NONE',  ( -0.000000000000000000, -0.000000000000000000, -1.000000000000000000 ) ) ;
#20896=CARTESIAN_POINT ( 'NONE',  ( -10.00000000000051337, 5.773502691895962435, -113.8749999999999858 ) ) ;
#20898=CARTESIAN_POINT ( 'NONE',  ( -10.81189881249999729, 6.242252689847871849, -173.4062500020483810 ) ) ;
#20899=CARTESIAN_POINT ( 'NONE',  ( 9.999999999999998224, 0.000000000000000000, -110.3750000040967763 ) ) ;
#20900=ADVANCED_FACE ( 'NONE', ( #34133 ), #37785, .F. ) ;
#20902=CARTESIAN_POINT ( 'NONE',  ( 7.644554776091147741E-16, 12.48450537969573659, -90.96875000204838102 ) ) ;
#20904=CARTESIAN_POINT ( 'NONE',  ( 10.81189881249999729, 0.000000000000000000, -199.3437500020484094 ) ) ;
#20905=CARTESIAN_POINT ( 'NONE',  ( 7.644554776091147741E-16, 12.48450537969573659, -97.15625000204839523 ) ) ;
#20907=CARTESIAN_POINT ( 'NONE',  ( 7.644554776091147741E-16, 12.48450537969573659, -105.9687500020483668 ) ) ;
#20910=CARTESIAN_POINT ( 'NONE',  ( -10.81189881249999729, 1.324075727343319199E-15, -179.2812500020484094 ) ) ;
#20911=CARTESIAN_POINT ( 'NONE',  ( -10.81189881249999907, -6.242252689847864744, -195.6562500020484094 ) ) ;
#20914=CARTESIAN_POINT ( 'NONE',  ( -4.999999999999996447, 8.660254037844387298, -172.8750000040968189 ) ) ;
#20916=CARTESIAN_POINT ( 'NONE',  ( -10.81189881249999729, 1.324075727343319199E-15, -18.59375000204835260 ) ) ;
#20918=CARTESIAN_POINT ( 'NONE',  ( -2.293366432827344421E-15, -12.48450537969573659, -132.2187500020483810 ) ) ;
#20920=CARTESIAN_POINT ( 'NONE',  ( -5.405949406250003975, -9.363379034771801557, -26.03125000204836681 ) ) ;
#20922=ADVANCED_FACE ( 'NONE', ( #8448 ), #1325, .F. ) ;
#20923=CARTESIAN_POINT ( 'NONE',  ( -10.00000000000025580, 5.773502691896109873, -101.8750000000000000 ) ) ;
#20924=CARTESIAN_POINT ( 'NONE',  ( 9.999999999999998224, 0.000000000000000000, -60.49999999999997158 ) ) ;
#20925=CARTESIAN_POINT ( 'NONE',  ( -10.81189881249999729, 1.324075727343319199E-15, -123.7812500020483952 ) ) ;
#20928=CARTESIAN_POINT ( 'NONE',  ( -9.999999999999479527, -5.773502691896549521, -145.1250000000000000 ) ) ;
#20929=CARTESIAN_POINT ( 'NONE',  ( -9.999999999999998224, 5.773502691896259087, -99.25000000409677625 ) ) ;
#20930=CARTESIAN_POINT ( 'NONE',  ( -9.999999999999998224, 1.224646799147353059E-15, -151.6250000040967905 ) ) ;
#20932=CARTESIAN_POINT ( 'NONE',  ( -5.405949406250003975, -9.363379034771801557, -55.84375000204835970 ) ) ;
#20939=CARTESIAN_POINT ( 'NONE',  ( 4.999999999999992006, -8.660254037844389075, -25.12500000409675849 ) ) ;
#20945=ORIENTED_EDGE ( 'NONE', *, *, #39140, .T. ) ;
#20947=ADVANCED_FACE ( 'NONE', ( #8014 ), #33919, .F. ) ;
#20949=EDGE_LOOP ( 'NONE', ( #36400, #13631, #34541, #2725 ) ) ;
#20953=CARTESIAN_POINT ( 'NONE',  ( 5.405949406249992428, -9.363379034771808662, -196.7812500020484094 ) ) ;
#20959=CARTESIAN_POINT ( 'NONE',  ( 5.405949406249992428, -9.363379034771808662, -117.0937500020483810 ) ) ;
#20960=CARTESIAN_POINT ( 'NONE',  ( -5.000000000000003553, -8.660254037844383745, -196.3750000040967905 ) ) ;
#20961=CARTESIAN_POINT ( 'NONE',  ( 10.81189881249999907, 6.242252689847868297, -122.9062500020484094 ) ) ;
#20963=CARTESIAN_POINT ( 'NONE',  ( -10.81189881249999729, 6.242252689847871849, -134.2187500020483810 ) ) ;
#20966=CARTESIAN_POINT ( 'NONE',  ( 5.000000000000000000, 8.660254037844385522, -157.7500000000000000 ) ) ;
#20967=CARTESIAN_POINT ( 'NONE',  ( -10.00000000000000000, -5.773502691896251982, -23.62499999999997868 ) ) ;
#20972=CARTESIAN_POINT ( 'NONE',  ( -10.81189881249999729, 1.324075727343319199E-15, -45.59375000204838102 ) ) ;
#20973=CARTESIAN_POINT ( 'NONE',  ( 10.00000000000076916, -5.773502691895816774, -110.5000000040967763 ) ) ;
#20974=CARTESIAN_POINT ( 'NONE',  ( -10.81189881249999729, 6.242252689847871849, -156.7187500020483810 ) ) ;
#20978=CARTESIAN_POINT ( 'NONE',  ( -9.999999999999998224, 1.224646799147353059E-15, -86.74999999999998579 ) ) ;
#20980=EDGE_LOOP ( 'NONE', ( #18453, #31809, #32746, #10165 ) ) ;
#20982=CARTESIAN_POINT ( 'NONE',  ( 7.644554776091147741E-16, 12.48450537969573659, -106.1562500020483810 ) ) ;
#20983=CARTESIAN_POINT ( 'NONE',  ( 9.999999999999998224, 0.000000000000000000, -120.8750000040967905 ) ) ;
#20987=CARTESIAN_POINT ( 'NONE',  ( -10.81189881249999907, -6.242252689847864744, -42.65625000204836681 ) ) ;
#20992=CARTESIAN_POINT ( 'NONE',  ( 7.070501591499376803E-16, 11.54700538379251284, -165.5000000040967905 ) ) ;
#20994=CARTESIAN_POINT ( 'NONE',  ( -9.999999999999998224, 0.000000000000000000, -99.99999999999998579 ) ) ;
#20995=ORIENTED_EDGE ( 'NONE', *, *, #7249, .T. ) ;
#20996=ORIENTED_EDGE ( 'NONE', *, *, #12691, .F. ) ;
#21008=CARTESIAN_POINT ( 'NONE',  ( 5.405949406249999534, 9.363379034771803333, -145.0937500020483810 ) ) ;
#21009=CARTESIAN_POINT ( 'NONE',  ( -10.81189881249999729, 1.324075727343319199E-15, -150.7812500020483810 ) ) ;
#21010=CARTESIAN_POINT ( 'NONE',  ( 10.81189881249999551, -6.242252689847874514, -151.4687500020484094 ) ) ;
#21011=DIRECTION ( 'NONE',  ( -1.000000000000000000, 0.000000000000000000, 0.000000000000000000 ) ) ;
#21012=CARTESIAN_POINT ( 'NONE',  ( 5.000000000000000000, 8.660254037844385522, -180.2500000000000284 ) ) ;
#21014=CARTESIAN_POINT ( 'NONE',  ( -1.470112319795894296, 10.71737856626141827, -100.0000000000000142 ) ) ;
#21017=CARTESIAN_POINT ( 'NONE',  ( 10.81189881249999907, 6.242252689847868297, -181.2187500020484094 ) ) ;
#21020=CARTESIAN_POINT ( 'NONE',  ( 5.405949406249999534, 9.363379034771803333, -44.78125000204838102 ) ) ;
#21022=CARTESIAN_POINT ( 'NONE',  ( -2.121150477449813534E-15, -11.54700538379251284, -110.3749999999999858 ) ) ;
#21024=AXIS2_PLACEMENT_3D ( 'NONE', #15242, #1894, #28222 ) ;
#21025=CARTESIAN_POINT ( 'NONE',  ( 10.81189881249999729, 6.242252689847867408, -128.9062500020483810 ) ) ;
#21026=CARTESIAN_POINT ( 'NONE',  ( 9.999999999999996447, -5.773502691896262640, -145.0000000040967905 ) ) ;
#21027=CARTESIAN_POINT ( 'NONE',  ( 9.999999999999998224, 0.000000000000000000, -167.0000000000000000 ) ) ;
#21031=CARTESIAN_POINT ( 'NONE',  ( -10.81189881249999729, 1.324075727343319199E-15, -170.0937500020484094 ) ) ;
#21034=CARTESIAN_POINT ( 'NONE',  ( 0.000000000000000000, 0.000000000000000000, -99.99999999999998579 ) ) ;
#21035=CARTESIAN_POINT ( 'NONE',  ( -10.81189881249999729, 1.324075727343319199E-15, -77.28125000204838102 ) ) ;
#21037=CARTESIAN_POINT ( 'NONE',  ( 4.999999999999992006, -8.660254037844389075, -50.62500000409675494 ) ) ;
#21038=CARTESIAN_POINT ( 'NONE',  ( -10.81189881249999907, -6.242252689847864744, -10.96875000204835970 ) ) ;
#21041=DIRECTION ( 'NONE',  ( -0.000000000000000000, -0.000000000000000000, -1.000000000000000000 ) ) ;
#21051=( BOUNDED_CURVE ( )  B_SPLINE_CURVE ( 2, ( #32869, #12567, #39119, #35687, #32453, #6956, #20113 ),
 .UNSPECIFIED., .F., .F. ) 
 B_SPLINE_CURVE_WITH_KNOTS ( ( 3, 2, 2, 3 ),
 ( 0.2835820895522389029, 0.2848258706467662882, 0.2860696517412936180, 0.2873134328358210032 ),
 .UNSPECIFIED. ) 
 CURVE ( )  GEOMETRIC_REPRESENTATION_ITEM ( )  RATIONAL_B_SPLINE_CURVE ( ( 0.9999999999999880096, 0.8660254037844506980, 1.000000000000000000, 0.8660254037844387076, 1.000000000000000000, 0.8660254037844267172, 1.000000000000011990 ) ) 
 REPRESENTATION_ITEM ( '' )  );
#21058=CARTESIAN_POINT ( 'NONE',  ( -10.00000000000000000, -5.773502691896251982, -44.62499999999997158 ) ) ;
#21060=CARTESIAN_POINT ( 'NONE',  ( 5.405949406249992428, -9.363379034771808662, -162.0937500020484094 ) ) ;
#21062=CARTESIAN_POINT ( 'NONE',  ( -9.999999999999483080, -5.773502691897144601, -100.1249999999999574 ) ) ;
#21063=DIRECTION ( 'NONE',  ( -0.000000000000000000, -0.000000000000000000, -1.000000000000000000 ) ) ;
#21064=CARTESIAN_POINT ( 'NONE',  ( -9.999999999999998224, 1.224646799147353059E-15, -103.6250000040967763 ) ) ;
#21071=CARTESIAN_POINT ( 'NONE',  ( 7.644554776091147741E-16, 12.48450537969573659, -60.96875000204838102 ) ) ;
#21073=CARTESIAN_POINT ( 'NONE',  ( 10.81189881249999551, -6.242252689847874514, -64.65625000204839523 ) ) ;
#21075=CARTESIAN_POINT ( 'NONE',  ( 7.070501591499377789E-16, 11.54700538379251284, -130.6250000000000000 ) ) ;
#21076=VECTOR ( 'NONE', #37454, 1000.000000000000000 ) ;
#21077=CARTESIAN_POINT ( 'NONE',  ( 10.81189881249999551, -6.242252689847874514, -147.1562500020484379 ) ) ;
#21078=CARTESIAN_POINT ( 'NONE',  ( 10.81189881249999907, 6.242252689847868297, -163.4062500020484094 ) ) ;
#21079=CARTESIAN_POINT ( 'NONE',  ( -5.000000000000003553, -8.660254037844383745, -145.3750000040967905 ) ) ;
#21081=CARTESIAN_POINT ( 'NONE',  ( 10.81189881249999551, -6.242252689847874514, -95.96875000204838102 ) ) ;
#21084=CARTESIAN_POINT ( 'NONE',  ( -10.81189881249999729, 1.324075727343319199E-15, -0.7812500020483725827 ) ) ;
#21086=CARTESIAN_POINT ( 'NONE',  ( 4.162302680423837664, -9.761226838701102082, -180.0000000000000284 ) ) ;
#21087=CARTESIAN_POINT ( 'NONE',  ( -2.293366432827344421E-15, -12.48450537969573659, -97.90625000204839523 ) ) ;
#21089=CARTESIAN_POINT ( 'NONE',  ( -10.00000000000000000, -5.773502691896251982, -78.00000000409677625 ) ) ;
#21090=CARTESIAN_POINT ( 'NONE',  ( -4.999999999999996447, 8.660254037844387298, -135.0000000000000000 ) ) ;
#21091=CARTESIAN_POINT ( 'NONE',  ( -10.81189881249999729, 1.324075727343319199E-15, -35.09375000204836681 ) ) ;
#21094=CARTESIAN_POINT ( 'NONE',  ( 7.644554776091147741E-16, 12.48450537969573659, -29.65625000204835615 ) ) ;
#21097=CARTESIAN_POINT ( 'NONE',  ( -4.999999999999996447, 8.660254037844387298, -4.875000004096769146 ) ) ;
#21099=( BOUNDED_CURVE ( )  B_SPLINE_CURVE ( 2, ( #33946, #24232, #37383, #7826, #36950, #20973, #17081 ),
 .UNSPECIFIED., .F., .F. ) 
 B_SPLINE_CURVE_WITH_KNOTS ( ( 3, 2, 2, 3 ),
 ( 0.4365671641791046276, 0.4378109452736320129, 0.4390547263681593981, 0.4402985074626867279 ),
 .UNSPECIFIED. ) 
 CURVE ( )  GEOMETRIC_REPRESENTATION_ITEM ( )  RATIONAL_B_SPLINE_CURVE ( ( 0.9999999999999820144, 0.8660254037844566932, 1.000000000000000000, 0.8660254037844387076, 1.000000000000000000, 0.8660254037844207220, 1.000000000000017986 ) ) 
 REPRESENTATION_ITEM ( '' )  );
#21105=ORIENTED_EDGE ( 'NONE', *, *, #4603, .T. ) ;
#21113=CARTESIAN_POINT ( 'NONE',  ( 10.81189881249999551, -6.242252689847874514, -160.6562500020484379 ) ) ;
#21116=CARTESIAN_POINT ( 'NONE',  ( -10.81189881249999729, 1.324075727343319199E-15, -90.59375000204838102 ) ) ;
#21118=CARTESIAN_POINT ( 'NONE',  ( 10.81189881249999729, 0.000000000000000000, -197.8437500020484094 ) ) ;
#21119=CARTESIAN_POINT ( 'NONE',  ( 10.81189881249999551, -6.242252689847874514, -99.15625000204838102 ) ) ;
#21121=CARTESIAN_POINT ( 'NONE',  ( -10.81189881249999729, 6.242252689847871849, -105.7187500020483668 ) ) ;
#21125=CARTESIAN_POINT ( 'NONE',  ( 9.999999999999998224, 0.000000000000000000, -0.4999999999999726885 ) ) ;
#21127=CARTESIAN_POINT ( 'NONE',  ( -9.999999999999998224, 5.773502691896259087, -171.2500000040967905 ) ) ;
#21129=CARTESIAN_POINT ( 'NONE',  ( 10.81189881249999729, 0.000000000000000000, -22.34375000204835615 ) ) ;
#21131=CARTESIAN_POINT ( 'NONE',  ( -10.81189881249999729, 1.324075727343319199E-15, -131.0937500020483810 ) ) ;
#21134=CARTESIAN_POINT ( 'NONE',  ( 10.81189881249999907, 6.242252689847868297, -29.90625000204835970 ) ) ;
#21137=EDGE_CURVE ( 'NONE', #34823, #6210, #39762, .T. ) ;
#21138=CARTESIAN_POINT ( 'NONE',  ( -9.999999999999998224, 5.773502691896259087, -49.37499999999997868 ) ) ;
#21139=CARTESIAN_POINT ( 'NONE',  ( -2.293366432827344421E-15, -12.48450537969573659, -124.9062500020483810 ) ) ;
#21142=CARTESIAN_POINT ( 'NONE',  ( -9.999999999999998224, 5.773502691896259087, -97.75000000409677625 ) ) ;
#21143=LINE ( 'NONE', #8211, #40146 ) ;
#21145=CARTESIAN_POINT ( 'NONE',  ( 5.405949406249992428, -9.363379034771808662, -60.09375000204835970 ) ) ;
#21150=DIRECTION ( 'NONE',  ( -0.000000000000000000, -0.000000000000000000, -1.000000000000000000 ) ) ;
#21151=CARTESIAN_POINT ( 'NONE',  ( -5.000000000000003553, -8.660254037844383745, -31.37500000409676559 ) ) ;
#21163=CARTESIAN_POINT ( 'NONE',  ( 10.81189881249999551, -6.242252689847874514, -196.6562500020484379 ) ) ;
#21169=CARTESIAN_POINT ( 'NONE',  ( 10.81189881249999907, 6.242252689847868297, -115.2187500020483810 ) ) ;
#21170=CARTESIAN_POINT ( 'NONE',  ( 10.00000000000000000, 5.773502691896255534, -194.2500000040968189 ) ) ;
#21171=CARTESIAN_POINT ( 'NONE',  ( -10.81189881249999907, -6.242252689847864744, -120.6562500020483810 ) ) ;
#21173=CARTESIAN_POINT ( 'NONE',  ( 10.81189881249999729, 6.242252689847867408, -128.7187500020483810 ) ) ;
#21174=CARTESIAN_POINT ( 'NONE',  ( 9.999999999999998224, 0.000000000000000000, -165.8750000040967905 ) ) ;
#21176=CARTESIAN_POINT ( 'NONE',  ( 9.999999999999996447, -5.773502691896262640, -146.1250000000000000 ) ) ;
#21177=CARTESIAN_POINT ( 'NONE',  ( 7.070501591499377789E-16, 11.54700538379251284, -22.62499999999997868 ) ) ;
#21180=CARTESIAN_POINT ( 'NONE',  ( -5.000000000000003553, -8.660254037844383745, -158.8750000040967905 ) ) ;
#21182=CARTESIAN_POINT ( 'NONE',  ( -10.81189881249999729, 1.324075727343319199E-15, -44.09375000204837391 ) ) ;
#21184=CARTESIAN_POINT ( 'NONE',  ( 5.405949406249992428, -9.363379034771808662, -154.5937500020483810 ) ) ;
#21185=EDGE_CURVE ( 'NONE', #17257, #19459, #25698, .T. ) ;
#21190=CARTESIAN_POINT ( 'NONE',  ( 5.000000000000000000, 8.660254037844385522, -76.74999999999998579 ) ) ;
#21194=CARTESIAN_POINT ( 'NONE',  ( 10.81189881249999729, 6.242252689847867408, -104.9062500020483952 ) ) ;
#21195=CARTESIAN_POINT ( 'NONE',  ( -4.999999999999996447, 8.660254037844387298, -123.3750000040967905 ) ) ;
#21200=CARTESIAN_POINT ( 'NONE',  ( 5.405949406249992428, -9.363379034771808662, -45.28125000204838102 ) ) ;
#21204=CARTESIAN_POINT ( 'NONE',  ( 7.070501591499376803E-16, 11.54700538379251284, -109.6249999999999858 ) ) ;
#21205=ORIENTED_EDGE ( 'NONE', *, *, #34924, .F. ) ;
#21209=VERTEX_POINT ( 'NONE', #12294 ) ;
#21216=CARTESIAN_POINT ( 'NONE',  ( -10.00000000000038547, 5.773502691896036154, -153.2500000040967905 ) ) ;
#21221=CARTESIAN_POINT ( 'NONE',  ( -10.81189881249999729, 6.242252689847871849, -143.2187500020484094 ) ) ;
#21222=CARTESIAN_POINT ( 'NONE',  ( 10.81189881249999907, 6.242252689847868297, -145.4062500020484094 ) ) ;
#21223=CARTESIAN_POINT ( 'NONE',  ( -2.293366432827344421E-15, -12.48450537969573659, -151.7187500020483810 ) ) ;
#21225=( BOUNDED_CURVE ( )  B_SPLINE_CURVE ( 2, ( #40689, #20852, #34036, #24539, #37046, #11552, #40472 ),
 .UNSPECIFIED., .F., .F. ) 
 B_SPLINE_CURVE_WITH_KNOTS ( ( 3, 2, 2, 3 ),
 ( 0.3656716417910448325, 0.3669154228855722732, 0.3681592039800996030, 0.3694029850746270438 ),
 .UNSPECIFIED. ) 
 CURVE ( )  GEOMETRIC_REPRESENTATION_ITEM ( )  RATIONAL_B_SPLINE_CURVE ( ( 0.9999999999999940048, 0.8660254037844447028, 1.000000000000000000, 0.8660254037844387076, 1.000000000000000000, 0.8660254037844207220, 1.000000000000017986 ) ) 
 REPRESENTATION_ITEM ( '' )  );
#21227=CARTESIAN_POINT ( 'NONE',  ( -9.999999999999998224, 1.224646799147353059E-15, -167.7500000000000000 ) ) ;
#21231=CARTESIAN_POINT ( 'NONE',  ( -5.741579586894616227, -8.238110979333516326, -99.99999999999995737 ) ) ;
#21232=CARTESIAN_POINT ( 'NONE',  ( 5.405949406249999534, 9.363379034771803333, -176.5937500020484094 ) ) ;
#21236=CARTESIAN_POINT ( 'NONE',  ( -5.405949406249996869, 9.363379034771805109, -41.53125000204838102 ) ) ;
#21238=CARTESIAN_POINT ( 'NONE',  ( 5.000000000000000000, 8.660254037844385522, -105.2499999999999858 ) ) ;
#21241=CARTESIAN_POINT ( 'NONE',  ( 5.405949406249999534, 9.363379034771803333, -124.2812500020483952 ) ) ;
#21242=CARTESIAN_POINT ( 'NONE',  ( 5.000000000000000000, 8.660254037844385522, -152.1250000040967905 ) ) ;
#21246=CARTESIAN_POINT ( 'NONE',  ( -5.405949406250003975, -9.363379034771801557, -175.8437500020483810 ) ) ;
#21250=CARTESIAN_POINT ( 'NONE',  ( 5.405949406249999534, 9.363379034771803333, -71.78125000204838102 ) ) ;
#21252=CARTESIAN_POINT ( 'NONE',  ( -5.000000000000003553, -8.660254037844383745, -41.87500000409677625 ) ) ;
#21253=CARTESIAN_POINT ( 'NONE',  ( 5.405949406249992428, -9.363379034771808662, -4.593750002048368586 ) ) ;
#21258=CARTESIAN_POINT ( 'NONE',  ( -10.00000000000076916, 5.773502691895813221, -138.2500000040967905 ) ) ;
#21259=B_SPLINE_CURVE_WITH_KNOTS ( 'NONE', 3,
 ( #31179, #28366, #41505, #37198, #7646, #4406, #30747, #21014, #3458, #12149, #26550, #2669 ),
 .UNSPECIFIED., .F., .F.,
 ( 4, 2, 2, 2, 2, 4 ),
 ( 4.985610057939991272E-16, 0.002144051117877697737, 0.004288102235754896741, 0.005360127794693496026, 0.006432153353632096178, 0.008576204471509293881 ),
 .UNSPECIFIED. ) ;
#21263=CARTESIAN_POINT ( 'NONE',  ( -9.999999999999998224, 0.000000000000000000, -99.99999999999998579 ) ) ;
#21265=ORIENTED_EDGE ( 'NONE', *, *, #15138, .T. ) ;
#21275=CARTESIAN_POINT ( 'NONE',  ( -10.00000000000000000, -5.773502691896251982, -38.62499999999996447 ) ) ;
#21278=CARTESIAN_POINT ( 'NONE',  ( -5.405949406250003975, -9.363379034771801557, -166.8437500020484094 ) ) ;
#21280=DIRECTION ( 'NONE',  ( -1.000000000000000000, 0.000000000000000000, 0.000000000000000000 ) ) ;
#21287=CARTESIAN_POINT ( 'NONE',  ( -10.81189881249999729, 6.242252689847871849, -62.21875000204838102 ) ) ;
#21288=CARTESIAN_POINT ( 'NONE',  ( -2.293366432827344421E-15, -12.48450537969573659, -70.90625000204839523 ) ) ;
#21290=CARTESIAN_POINT ( 'NONE',  ( 9.999999999999998224, 0.000000000000000000, -129.5000000000000000 ) ) ;
#21291=CARTESIAN_POINT ( 'NONE',  ( -2.293366432827344421E-15, -12.48450537969573659, -148.9062500020484379 ) ) ;
#21292=CARTESIAN_POINT ( 'NONE',  ( 5.405949406249999534, 9.363379034771803333, -167.7812500020484094 ) ) ;
#21295=CARTESIAN_POINT ( 'NONE',  ( 10.81189881249999729, 0.000000000000000000, -97.34375000204838102 ) ) ;
#21298=CARTESIAN_POINT ( 'NONE',  ( 7.644554776091147741E-16, 12.48450537969573659, 0.3437499979516422943 ) ) ;
#21300=CYLINDRICAL_SURFACE ( 'NONE', #21024, 9.999999999999998224 ) ;
#21301=CARTESIAN_POINT ( 'NONE',  ( 7.644554776091147741E-16, 12.48450537969573659, -91.15625000204838102 ) ) ;
#21303=CARTESIAN_POINT ( 'NONE',  ( -9.999999999999998224, 1.224646799147353059E-15, -66.12500000409676204 ) ) ;
#21305=CARTESIAN_POINT ( 'NONE',  ( -5.405949406249996869, 9.363379034771805109, -26.34375000204835970 ) ) ;
#21306=ORIENTED_EDGE ( 'NONE', *, *, #6173, .T. ) ;
#21308=CARTESIAN_POINT ( 'NONE',  ( -2.293366432827344421E-15, -12.48450537969573659, -24.40625000204838102 ) ) ;
#21312=CARTESIAN_POINT ( 'NONE',  ( -9.999999999999998224, 1.224646799147353059E-15, -6.125000004096770034 ) ) ;
#21313=CARTESIAN_POINT ( 'NONE',  ( 9.999999999999998224, 0.000000000000000000, -152.3750000040967905 ) ) ;
#21319=VERTEX_POINT ( 'NONE', #38639 ) ;
#21327=CARTESIAN_POINT ( 'NONE',  ( -9.999999999999227285, -5.773502691896698735, -129.0000000040967620 ) ) ;
#21328=CARTESIAN_POINT ( 'NONE',  ( -9.999999999999998224, 1.224646799147353059E-15, -105.1250000040967763 ) ) ;
#21329=CARTESIAN_POINT ( 'NONE',  ( 5.405949406249999534, 9.363379034771803333, -163.2812500020484094 ) ) ;
#21332=CARTESIAN_POINT ( 'NONE',  ( 5.405949406249992428, -9.363379034771808662, -84.09375000204836681 ) ) ;
#21334=CARTESIAN_POINT ( 'NONE',  ( -10.81189881249999907, -6.242252689847864744, -193.9687500020484094 ) ) ;
#21335=CARTESIAN_POINT ( 'NONE',  ( 5.405949406249992428, -9.363379034771808662, -91.78125000204838102 ) ) ;
#21339=CARTESIAN_POINT ( 'NONE',  ( -5.405949406249996869, 9.363379034771805109, -178.0312500020483810 ) ) ;
#21340=CARTESIAN_POINT ( 'NONE',  ( -10.81189881249999907, -6.242252689847864744, -188.1562500020484094 ) ) ;
#21342=VECTOR ( 'NONE', #7677, 1000.000000000000000 ) ;
#21344=CARTESIAN_POINT ( 'NONE',  ( 7.070501591499377789E-16, 11.54700538379251284, -162.5000000040967905 ) ) ;
#21346=CARTESIAN_POINT ( 'NONE',  ( 10.81189881249999551, -6.242252689847874514, -10.46875000204835793 ) ) ;
#21347=DIRECTION ( 'NONE',  ( -1.000000000000000000, 0.000000000000000000, 0.000000000000000000 ) ) ;
#21348=CARTESIAN_POINT ( 'NONE',  ( 5.405949406249992428, -9.363379034771808662, -123.0937500020483952 ) ) ;
#21350=CARTESIAN_POINT ( 'NONE',  ( -10.81189881249999729, 6.242252689847871849, -23.40625000204837747 ) ) ;
#21353=CARTESIAN_POINT ( 'NONE',  ( 7.070501591499377789E-16, 11.54700538379251284, -52.62499999999997868 ) ) ;
#21354=CARTESIAN_POINT ( 'NONE',  ( -10.81189881249999729, 6.242252689847871849, -125.4062500020483810 ) ) ;
#21357=( BOUNDED_CURVE ( )  B_SPLINE_CURVE ( 2, ( #14074, #37412, #8067, #24045, #23831, #21216, #7854 ),
 .UNSPECIFIED., .F., .F. ) 
 B_SPLINE_CURVE_WITH_KNOTS ( ( 3, 2, 2, 3 ),
 ( 0.2238805970149254365, 0.2251243781094527940, 0.2263681592039801793, 0.2276119402985075368 ),
 .UNSPECIFIED. ) 
 CURVE ( )  GEOMETRIC_REPRESENTATION_ITEM ( )  RATIONAL_B_SPLINE_CURVE ( ( 0.9999999999999940048, 0.8660254037844447028, 1.000000000000000000, 0.8660254037844387076, 1.000000000000000000, 0.8660254037844297148, 1.000000000000008882 ) ) 
 REPRESENTATION_ITEM ( '' )  );
#21359=CARTESIAN_POINT ( 'NONE',  ( -9.999999999999998224, 1.224646799147353059E-15, -99.12500000409677625 ) ) ;
#21362=CARTESIAN_POINT ( 'NONE',  ( -10.81189881249999729, 6.242252689847871849, -47.21875000204836681 ) ) ;
#21368=CARTESIAN_POINT ( 'NONE',  ( -4.999999999999996447, 8.660254037844387298, -31.87500000409676559 ) ) ;
#21379=DIRECTION ( 'NONE',  ( -0.000000000000000000, -0.000000000000000000, -1.000000000000000000 ) ) ;
#21382=CARTESIAN_POINT ( 'NONE',  ( -10.81189881249999907, -6.242252689847864744, -185.1562500020484094 ) ) ;
#21387=CARTESIAN_POINT ( 'NONE',  ( -5.405949406249996869, 9.363379034771805109, -110.3437500020483810 ) ) ;
#21389=CARTESIAN_POINT ( 'NONE',  ( 5.405949406249992428, -9.363379034771808662, -112.7812500020483952 ) ) ;
#21391=CARTESIAN_POINT ( 'NONE',  ( -5.405949406249996869, 9.363379034771805109, -128.3437500020484094 ) ) ;
#21394=CARTESIAN_POINT ( 'NONE',  ( 9.999999999999998224, 0.000000000000000000, -146.0000000000000000 ) ) ;
#21395=CARTESIAN_POINT ( 'NONE',  ( 9.999999999999996447, -5.773502691896262640, -9.624999999999968026 ) ) ;
#21398=CARTESIAN_POINT ( 'NONE',  ( -10.00000000000000000, -5.773502691896252870, -170.6249999999999716 ) ) ;
#21400=CARTESIAN_POINT ( 'NONE',  ( 7.644554776091147741E-16, 12.48450537969573659, -42.96875000204835970 ) ) ;
#21401=CARTESIAN_POINT ( 'NONE',  ( -10.81189881249999907, -6.242252689847864744, -144.4687500020484094 ) ) ;
#21404=CARTESIAN_POINT ( 'NONE',  ( 5.000000000000000000, 8.660254037844385522, -72.24999999999998579 ) ) ;
#21407=CARTESIAN_POINT ( 'NONE',  ( -5.405949406250003975, -9.363379034771801557, -104.0312500020483810 ) ) ;
#21408=CARTESIAN_POINT ( 'NONE',  ( -4.999999999999996447, 8.660254037844387298, -126.3750000040967905 ) ) ;
#21410=CARTESIAN_POINT ( 'NONE',  ( -2.293366432827344421E-15, -12.48450537969573659, -79.71875000204838102 ) ) ;
#21413=VECTOR ( 'NONE', #12853, 1000.000000000000000 ) ;
#21415=CARTESIAN_POINT ( 'NONE',  ( 5.405949406249992428, -9.363379034771808662, -42.28125000204838102 ) ) ;
#21416=CARTESIAN_POINT ( 'NONE',  ( -2.121150477449813534E-15, -11.54700538379251284, -137.3750000000000000 ) ) ;
#21420=CARTESIAN_POINT ( 'NONE',  ( -9.999999999999868550, 5.773502691896333694, -176.8750000000000000 ) ) ;
#21424=ADVANCED_FACE ( 'NONE', ( #13765 ), #3236, .F. ) ;
#21425=VERTEX_POINT ( 'NONE', #7107 ) ;
#21435=CARTESIAN_POINT ( 'NONE',  ( -10.81189881249999729, 1.324075727343319199E-15, -140.0937500020483810 ) ) ;
#21436=CARTESIAN_POINT ( 'NONE',  ( -10.81189881249999907, -6.242252689847864744, -144.6562500020484094 ) ) ;
#21437=CARTESIAN_POINT ( 'NONE',  ( -10.81189881249999729, 1.324075727343319199E-15, -158.0937500020483810 ) ) ;
#21440=CARTESIAN_POINT ( 'NONE',  ( -5.000000000000003553, -8.660254037844383745, -170.5000000000000000 ) ) ;
#21444=CARTESIAN_POINT ( 'NONE',  ( -10.37936602110037931, 1.593253728262159941, -99.99999999999994316 ) ) ;
#21445=CARTESIAN_POINT ( 'NONE',  ( 7.644554776091147741E-16, 12.48450537969573659, -176.4687500020483810 ) ) ;
#21450=CARTESIAN_POINT ( 'NONE',  ( 10.81189881249999551, -6.242252689847874514, -40.65625000204835970 ) ) ;
#21452=CARTESIAN_POINT ( 'NONE',  ( -9.999999999999998224, 5.773502691896259087, -98.87499999999998579 ) ) ;
#21454=CARTESIAN_POINT ( 'NONE',  ( 10.81189881249999551, -6.242252689847874514, -126.1562500020483810 ) ) ;
#21455=CARTESIAN_POINT ( 'NONE',  ( -5.000000000000003553, -8.660254037844383745, -149.8750000040967905 ) ) ;
#21459=CARTESIAN_POINT ( 'NONE',  ( -10.81189881249999729, 6.242252689847871849, -173.2187500020483810 ) ) ;
#21461=ADVANCED_FACE ( 'NONE', ( #33239 ), #20044, .F. ) ;
#21462=CARTESIAN_POINT ( 'NONE',  ( -9.999999999999998224, 1.224646799147353059E-15, -121.6250000040967905 ) ) ;
#21463=CARTESIAN_POINT ( 'NONE',  ( 10.81189881249999729, 0.000000000000000000, -69.03125000204838102 ) ) ;
#21466=CARTESIAN_POINT ( 'NONE',  ( 10.00000000000000000, 5.773502691896255534, -41.25000000409676204 ) ) ;
#21467=CARTESIAN_POINT ( 'NONE',  ( 10.81189881249999729, 0.000000000000000000, -2.843750002048367698 ) ) ;
#21471=CARTESIAN_POINT ( 'NONE',  ( -5.000000000000003553, -8.660254037844383745, -106.3750000040967763 ) ) ;
#21476=( BOUNDED_CURVE ( )  B_SPLINE_CURVE ( 2, ( #422, #33853, #9898, #23073, #30194, #20030, #630 ),
 .UNSPECIFIED., .F., .F. ) 
 B_SPLINE_CURVE_WITH_KNOTS ( ( 3, 2, 2, 3 ),
 ( 0.2985074626865671932, 0.2997512437810946340, 0.3009950248756220192, 0.3022388059701494045 ),
 .UNSPECIFIED. ) 
 CURVE ( )  GEOMETRIC_REPRESENTATION_ITEM ( )  RATIONAL_B_SPLINE_CURVE ( ( 0.9999999999999940048, 0.8660254037844447028, 1.000000000000000000, 0.8660254037844387076, 1.000000000000000000, 0.8660254037844207220, 1.000000000000017986 ) ) 
 REPRESENTATION_ITEM ( '' )  );
#21480=ORIENTED_EDGE ( 'NONE', *, *, #8857, .F. ) ;
#21487=( BOUNDED_CURVE ( )  B_SPLINE_CURVE ( 2, ( #17253, #3475, #38, #19652, #13161, #19863, #26355 ),
 .UNSPECIFIED., .F., .F. ) 
 B_SPLINE_CURVE_WITH_KNOTS ( ( 3, 2, 2, 3 ),
 ( 0.3544776119402986980, 0.3557213930348260278, 0.3569651741293533576, 0.3582089552238806873 ),
 .UNSPECIFIED. ) 
 CURVE ( )  GEOMETRIC_REPRESENTATION_ITEM ( )  RATIONAL_B_SPLINE_CURVE ( ( 0.9999999999999820144, 0.8660254037844566932, 1.000000000000000000, 0.8660254037844387076, 1.000000000000000000, 0.8660254037844267172, 1.000000000000011990 ) ) 
 REPRESENTATION_ITEM ( '' )  );
#21494=CARTESIAN_POINT ( 'NONE',  ( -9.999999999999998224, 1.224646799147353059E-15, -38.74999999999997868 ) ) ;
#21497=CARTESIAN_POINT ( 'NONE',  ( 10.81189881249999729, 0.000000000000000000, -169.3437500020484094 ) ) ;
#21499=CARTESIAN_POINT ( 'NONE',  ( 5.405949406249999534, 9.363379034771803333, -175.0937500020484094 ) ) ;
#21502=CARTESIAN_POINT ( 'NONE',  ( -4.999999999999996447, 8.660254037844387298, -193.5000000000000000 ) ) ;
#21507=CARTESIAN_POINT ( 'NONE',  ( -5.405949406250003975, -9.363379034771801557, -58.84375000204835970 ) ) ;
#21508=CARTESIAN_POINT ( 'NONE',  ( 5.405949406249999534, 9.363379034771803333, -71.78125000204838102 ) ) ;
#21510=CARTESIAN_POINT ( 'NONE',  ( -9.999999999999998224, 1.224646799147353059E-15, -121.2500000000000000 ) ) ;
#21512=CARTESIAN_POINT ( 'NONE',  ( 5.405949406249999534, 9.363379034771803333, -149.7812500020483810 ) ) ;
#21513=CARTESIAN_POINT ( 'NONE',  ( -5.405949406249996869, 9.363379034771805109, -161.5312500020484094 ) ) ;
#21515=CARTESIAN_POINT ( 'NONE',  ( -4.999999999999996447, 8.660254037844387298, -159.3750000040967905 ) ) ;
#21516=CARTESIAN_POINT ( 'NONE',  ( 7.644554776091147741E-16, 12.48450537969573659, -98.46875000204839523 ) ) ;
#21517=ORIENTED_EDGE ( 'NONE', *, *, #37405, .T. ) ;
#21519=CARTESIAN_POINT ( 'NONE',  ( 5.405949406249992428, -9.363379034771808662, -196.5937500020484094 ) ) ;
#21521=CARTESIAN_POINT ( 'NONE',  ( -5.950676495627904572, -8.268445900970100126, -180.0000000000000000 ) ) ;
#21522=CARTESIAN_POINT ( 'NONE',  ( -10.81189881249999729, 6.242252689847871849, -89.40625000204838102 ) ) ;
#21524=CARTESIAN_POINT ( 'NONE',  ( 9.999999999999996447, -5.773502691896262640, -67.00000000409677625 ) ) ;
#21526=CARTESIAN_POINT ( 'NONE',  ( 5.405949406249992428, -9.363379034771808662, -25.59375000204835970 ) ) ;
#21529=CARTESIAN_POINT ( 'NONE',  ( -10.81189881249999907, -6.242252689847864744, -23.15625000204837747 ) ) ;
#21531=CARTESIAN_POINT ( 'NONE',  ( -2.121150477449813534E-15, -11.54700538379251284, -118.2500000040968189 ) ) ;
#21536=AXIS2_PLACEMENT_3D ( 'NONE', #18461, #11766, #32282 ) ;
#21538=CARTESIAN_POINT ( 'NONE',  ( 7.070501591499376803E-16, 11.54700538379251284, -120.1249999999999858 ) ) ;
#21546=VECTOR ( 'NONE', #30188, 1000.000000000000000 ) ;
#21549=CARTESIAN_POINT ( 'NONE',  ( -4.999999999999996447, 8.660254037844387298, -113.9999999999999858 ) ) ;
#21551=CARTESIAN_POINT ( 'NONE',  ( 10.81189881249999551, -6.242252689847874514, -163.6562500020484094 ) ) ;
#21555=CARTESIAN_POINT ( 'NONE',  ( 5.405949406249992428, -9.363379034771808662, -88.59375000204838102 ) ) ;
#21557=CARTESIAN_POINT ( 'NONE',  ( 5.405949406249992428, -9.363379034771808662, -190.5937500020484094 ) ) ;
#21558=CARTESIAN_POINT ( 'NONE',  ( -10.81189881249999729, 6.242252689847871849, -93.90625000204839523 ) ) ;
#21562=CARTESIAN_POINT ( 'NONE',  ( -5.405949406250003975, -9.363379034771801557, -173.0312500020484094 ) ) ;
#21563=CARTESIAN_POINT ( 'NONE',  ( 7.644554776091147741E-16, 12.48450537969573659, -188.6562500020484379 ) ) ;
#21565=CARTESIAN_POINT ( 'NONE',  ( 9.999999999999998224, 0.000000000000000000, -167.3750000040967905 ) ) ;
#21567=CARTESIAN_POINT ( 'NONE',  ( -5.405949406249996869, 9.363379034771805109, -17.34375000204835260 ) ) ;
#21569=CARTESIAN_POINT ( 'NONE',  ( 7.644554776091147741E-16, 12.48450537969573659, -120.9687500020483952 ) ) ;
#21571=CARTESIAN_POINT ( 'NONE',  ( -2.293366432827344421E-15, -12.48450537969573659, -18.40625000204837391 ) ) ;
#21575=CARTESIAN_POINT ( 'NONE',  ( -2.121150477449813534E-15, -11.54700538379251284, -53.37499999999997868 ) ) ;
#21576=CARTESIAN_POINT ( 'NONE',  ( -10.81189881249999729, 6.242252689847871849, -116.4062500020483810 ) ) ;
#21579=ORIENTED_EDGE ( 'NONE', *, *, #34123, .F. ) ;
#21580=CARTESIAN_POINT ( 'NONE',  ( 4.999999999999992006, -8.660254037844389075, -89.62500000409677625 ) ) ;
#21583=CARTESIAN_POINT ( 'NONE',  ( 10.81189881249999551, -6.242252689847874514, -53.96875000204837391 ) ) ;
#21589=CARTESIAN_POINT ( 'NONE',  ( 4.999999999999992006, -8.660254037844389075, -20.62500000409675494 ) ) ;
#21597=ORIENTED_EDGE ( 'NONE', *, *, #18843, .T. ) ;
#21602=EDGE_CURVE ( 'NONE', #13677, #23116, #19348, .T. ) ;
#21603=CARTESIAN_POINT ( 'NONE',  ( 7.644554776091147741E-16, 12.48450537969573659, -190.1562500020484094 ) ) ;
#21607=CARTESIAN_POINT ( 'NONE',  ( 5.405949406249992428, -9.363379034771808662, -112.5937500020483810 ) ) ;
#21609=CARTESIAN_POINT ( 'NONE',  ( 10.81189881249999551, -6.242252689847874514, -120.1562500020483810 ) ) ;
#21611=CARTESIAN_POINT ( 'NONE',  ( -5.405949406249996869, 9.363379034771805109, -122.3437500020483952 ) ) ;
#21614=CYLINDRICAL_SURFACE ( 'NONE', #13014, 9.999999999999998224 ) ;
#21615=CARTESIAN_POINT ( 'NONE',  ( -9.999999999999998224, 5.773502691896259087, -145.3750000000000000 ) ) ;
#21616=CARTESIAN_POINT ( 'NONE',  ( 10.00000000000000000, 5.773502691896255534, -12.37499999999996803 ) ) ;
#21619=CARTESIAN_POINT ( 'NONE',  ( -5.000000000000003553, -8.660254037844383745, -188.8750000040967905 ) ) ;
#21621=CARTESIAN_POINT ( 'NONE',  ( 7.644554776091147741E-16, 12.48450537969573659, -33.96875000204835260 ) ) ;
#21623=CARTESIAN_POINT ( 'NONE',  ( 10.81189881249999907, 6.242252689847868297, -149.7187500020483810 ) ) ;
#21625=ADVANCED_FACE ( 'NONE', ( #10964 ), #37660, .T. ) ;
#21626=CARTESIAN_POINT ( 'NONE',  ( 10.00000000000051159, -5.773502691895965988, -101.5000000040967763 ) ) ;
#21627=CARTESIAN_POINT ( 'NONE',  ( 7.070501591499377789E-16, 11.54700538379251284, -73.62499999999995737 ) ) ;
#21628=CARTESIAN_POINT ( 'NONE',  ( -5.405949406249996869, 9.363379034771805109, -143.5312500020483810 ) ) ;
#21630=ORIENTED_EDGE ( 'NONE', *, *, #37289, .F. ) ;
#21631=CARTESIAN_POINT ( 'NONE',  ( -10.81189881249999729, 6.242252689847871849, -105.9062500020483810 ) ) ;
#21632=CARTESIAN_POINT ( 'NONE',  ( 9.999999999999998224, 0.000000000000000000, -117.8750000040967905 ) ) ;
#21634=CARTESIAN_POINT ( 'NONE',  ( 10.81189881249999551, -6.242252689847874514, -77.96875000204838102 ) ) ;
#21636=CARTESIAN_POINT ( 'NONE',  ( 5.405949406249999534, 9.363379034771803333, -46.28125000204838813 ) ) ;
#21640=CARTESIAN_POINT ( 'NONE',  ( 4.999999999999992006, -8.660254037844389075, -164.6250000040967905 ) ) ;
#21644=ORIENTED_EDGE ( 'NONE', *, *, #26989, .F. ) ;
#21648=CARTESIAN_POINT ( 'NONE',  ( 4.999999999999992006, -8.660254037844389075, -130.1250000040967620 ) ) ;
#21652=CARTESIAN_POINT ( 'NONE',  ( 5.405949406249999534, 9.363379034771803333, -131.5937500020483810 ) ) ;
#21653=CARTESIAN_POINT ( 'NONE',  ( -10.81189881249999729, 6.242252689847871849, -138.9062500020484094 ) ) ;
#21654=CARTESIAN_POINT ( 'NONE',  ( -10.81189881249999729, -6.242252689847864744, -154.9687500020484094 ) ) ;
#21655=CARTESIAN_POINT ( 'NONE',  ( 7.070501591499376803E-16, 11.54700538379251284, -127.6249999999999858 ) ) ;
#21657=CARTESIAN_POINT ( 'NONE',  ( 9.999999999999996447, -5.773502691896262640, -173.1250000000000000 ) ) ;
#21662=CARTESIAN_POINT ( 'NONE',  ( -4.999999999999996447, 8.660254037844387298, -133.5000000000000000 ) ) ;
#21663=CARTESIAN_POINT ( 'NONE',  ( 10.81189881249999729, 0.000000000000000000, -172.3437500020484094 ) ) ;
#21666=CARTESIAN_POINT ( 'NONE',  ( -2.293366432827344421E-15, -12.48450537969573659, -48.40625000204838102 ) ) ;
#21668=CARTESIAN_POINT ( 'NONE',  ( -5.000000000000003553, -8.660254037844383745, -99.99999999999998579 ) ) ;
#21670=CARTESIAN_POINT ( 'NONE',  ( -10.81189881249999729, -6.242252689847864744, -125.1562500020483810 ) ) ;
#21671=CARTESIAN_POINT ( 'NONE',  ( -5.000000000000003553, -8.660254037844383745, -146.8750000040967905 ) ) ;
#21675=CARTESIAN_POINT ( 'NONE',  ( -10.81189881249999729, 6.242252689847871849, -170.2187500020483810 ) ) ;
#21677=EDGE_CURVE ( 'NONE', #27421, #31328, #23768, .T. ) ;
#21679=CARTESIAN_POINT ( 'NONE',  ( 9.999999999999998224, 0.000000000000000000, -155.0000000000000000 ) ) ;
#21681=CARTESIAN_POINT ( 'NONE',  ( -10.81189881249999907, -6.242252689847864744, -68.15625000204839523 ) ) ;
#21682=CARTESIAN_POINT ( 'NONE',  ( -9.999999999999998224, 1.224646799147353059E-15, -43.62500000409677625 ) ) ;
#21683=CARTESIAN_POINT ( 'NONE',  ( -2.293366432827344421E-15, -12.48450537969573659, -1.718750002048352377 ) ) ;
#21687=CARTESIAN_POINT ( 'NONE',  ( 7.070501591499376803E-16, 11.54700538379251284, -148.6250000000000000 ) ) ;
#21688=EDGE_LOOP ( 'NONE', ( #2813, #39943, #10374, #35405 ) ) ;
#21693=VERTEX_POINT ( 'NONE', #20683 ) ;
#21696=ORIENTED_EDGE ( 'NONE', *, *, #22141, .T. ) ;
#21697=ORIENTED_EDGE ( 'NONE', *, *, #4064, .T. ) ;
#21699=CARTESIAN_POINT ( 'NONE',  ( 0.000000000000000000, 0.000000000000000000, -99.99999999999998579 ) ) ;
#21703=CARTESIAN_POINT ( 'NONE',  ( 9.999999999999998224, 0.000000000000000000, -108.8750000040967763 ) ) ;
#21704=CARTESIAN_POINT ( 'NONE',  ( 9.999999999999996447, -5.773502691896262640, -35.12499999999996447 ) ) ;
#21707=CARTESIAN_POINT ( 'NONE',  ( 7.644554776091147741E-16, 12.48450537969573659, -153.9687500020484094 ) ) ;
#21710=VECTOR ( 'NONE', #17997, 1000.000000000000114 ) ;
#21711=FACE_OUTER_BOUND ( 'NONE', #18028, .T. ) ;
#21712=CARTESIAN_POINT ( 'NONE',  ( -10.00000000000000000, -5.773502691896251982, -191.6250000000000284 ) ) ;
#21714=CARTESIAN_POINT ( 'NONE',  ( -9.999999999999998224, 1.224646799147353059E-15, -140.7500000000000000 ) ) ;
#21717=CARTESIAN_POINT ( 'NONE',  ( 5.405949406249992428, -9.363379034771808662, -72.28125000204838102 ) ) ;
#21719=CARTESIAN_POINT ( 'NONE',  ( -4.999999999999996447, 8.660254037844387298, -123.0000000000000000 ) ) ;
#21720=CARTESIAN_POINT ( 'NONE',  ( 5.405949406249992428, -9.363379034771808662, -148.7812500020483810 ) ) ;
#21721=CARTESIAN_POINT ( 'NONE',  ( -10.81189881249999907, -6.242252689847864744, -167.1562500020483810 ) ) ;
#21722=LINE ( 'NONE', #15235, #18554 ) ;
#21724=CARTESIAN_POINT ( 'NONE',  ( 10.81189881249999729, 0.000000000000000000, -100.3437500020483810 ) ) ;
#21727=CARTESIAN_POINT ( 'NONE',  ( -5.405949406249996869, 9.363379034771805109, -194.3437500020484094 ) ) ;
#21729=EDGE_CURVE ( 'NONE', #39897, #30831, #580, .T. ) ;
#21730=CARTESIAN_POINT ( 'NONE',  ( 6.072958700806868393, -8.826036754033463438, -180.0000000000000853 ) ) ;
#21732=CARTESIAN_POINT ( 'NONE',  ( 5.405949406249992428, -9.363379034771808662, -93.28125000204838102 ) ) ;
#21737=CARTESIAN_POINT ( 'NONE',  ( 9.999999999999998224, 0.000000000000000000, -65.37500000409676204 ) ) ;
#21739=CARTESIAN_POINT ( 'NONE',  ( 10.81189881249999729, 0.000000000000000000, -29.84375000204836326 ) ) ;
#21741=EDGE_CURVE ( 'NONE', #5570, #36180, #8209, .T. ) ;
#21742=CARTESIAN_POINT ( 'NONE',  ( 5.405949406249999534, 9.363379034771803333, -19.28125000204835970 ) ) ;
#21744=CARTESIAN_POINT ( 'NONE',  ( 9.999999999999998224, 0.000000000000000000, -161.0000000000000000 ) ) ;
#21749=AXIS2_PLACEMENT_3D ( 'NONE', #29589, #6706, #3051 ) ;
#21752=VERTEX_POINT ( 'NONE', #22399 ) ;
#21753=CARTESIAN_POINT ( 'NONE',  ( -9.999999999999998224, 1.224646799147353059E-15, -115.6250000040967905 ) ) ;
#21759=EDGE_CURVE ( 'NONE', #34823, #24099, #2561, .T. ) ;
#21762=CARTESIAN_POINT ( 'NONE',  ( 9.600329599501245426, 4.034346693190136612, -99.99999999999994316 ) ) ;
#21763=CARTESIAN_POINT ( 'NONE',  ( 7.070501591499376803E-16, 11.54700538379251284, -105.5000000040967763 ) ) ;
#21764=CARTESIAN_POINT ( 'NONE',  ( 5.405949406249992428, -9.363379034771808662, -165.2812500020484094 ) ) ;
#21768=AXIS2_PLACEMENT_3D ( 'NONE', #1461, #824, #27570 ) ;
#21769=CARTESIAN_POINT ( 'NONE',  ( 5.405949406249992428, -9.363379034771808662, -87.09375000204836681 ) ) ;
#21771=CARTESIAN_POINT ( 'NONE',  ( 5.405949406249992428, -9.363379034771808662, -193.5937500020484094 ) ) ;
#21772=CARTESIAN_POINT ( 'NONE',  ( -5.405949406250003975, -9.363379034771801557, -95.03125000204838102 ) ) ;
#21776=CARTESIAN_POINT ( 'NONE',  ( 5.405949406249992428, -9.363379034771808662, -174.2812500020484094 ) ) ;
#21777=CARTESIAN_POINT ( 'NONE',  ( 7.644554776091147741E-16, 12.48450537969573659, -185.6562500020484094 ) ) ;
#21779=CARTESIAN_POINT ( 'NONE',  ( 5.000000000000000000, 8.660254037844385522, -161.1250000040967905 ) ) ;
#21781=CARTESIAN_POINT ( 'NONE',  ( 10.81189881249999729, 0.000000000000000000, -13.34375000204834905 ) ) ;
#21783=CARTESIAN_POINT ( 'NONE',  ( 5.405949406249999534, 9.363379034771803333, -121.0937500020483952 ) ) ;
#21785=CARTESIAN_POINT ( 'NONE',  ( -10.81189881249999729, 1.324075727343319199E-15, -23.28125000204836326 ) ) ;
#21788=CARTESIAN_POINT ( 'NONE',  ( -2.121150477449813534E-15, -11.54700538379251284, -51.87499999999997158 ) ) ;
#21789=CARTESIAN_POINT ( 'NONE',  ( 10.81189881249999907, 6.242252689847868297, -113.9062500020483952 ) ) ;
#21792=CARTESIAN_POINT ( 'NONE',  ( 9.999999999999998224, 0.000000000000000000, -90.87500000409677625 ) ) ;
#21795=CARTESIAN_POINT ( 'NONE',  ( -10.81189881249999729, 6.242252689847871849, -53.21875000204836681 ) ) ;
#21800=CARTESIAN_POINT ( 'NONE',  ( -4.999999999999996447, 8.660254037844387298, -16.87500000409675138 ) ) ;
#21806=VERTEX_POINT ( 'NONE', #38375 ) ;
#21811=ORIENTED_EDGE ( 'NONE', *, *, #34843, .F. ) ;
#21815=CARTESIAN_POINT ( 'NONE',  ( -10.81189881249999729, 1.324075727343319199E-15, -185.2812500020484094 ) ) ;
#21819=CARTESIAN_POINT ( 'NONE',  ( 7.644554776091147741E-16, 12.48450537969573659, -110.4687500020483668 ) ) ;
#21820=CARTESIAN_POINT ( 'NONE',  ( 9.999999999999998224, 0.000000000000000000, -149.3750000040967905 ) ) ;
#21821=CARTESIAN_POINT ( 'NONE',  ( -10.81189881249999907, -6.242252689847864744, -116.1562500020483952 ) ) ;
#21823=CARTESIAN_POINT ( 'NONE',  ( -10.81189881249999729, -6.242252689847864744, -123.4687500020483952 ) ) ;
#21825=CARTESIAN_POINT ( 'NONE',  ( 0.000000000000000000, 0.000000000000000000, -99.99999999999998579 ) ) ;
#21827=CARTESIAN_POINT ( 'NONE',  ( 9.999999999999996447, -5.773502691896262640, -149.1250000000000000 ) ) ;
#21828=CARTESIAN_POINT ( 'NONE',  ( -9.999999999999998224, 5.773502691896259087, -16.37499999999997158 ) ) ;
#21831=CARTESIAN_POINT ( 'NONE',  ( -9.999999999999998224, 1.224646799147353059E-15, -184.6250000040967905 ) ) ;
#21833=CARTESIAN_POINT ( 'NONE',  ( 7.644554776091147741E-16, 12.48450537969573659, -41.46875000204835970 ) ) ;
#21835=CARTESIAN_POINT ( 'NONE',  ( 10.81189881249999551, -6.242252689847874514, -149.9687500020483810 ) ) ;
#21838=CARTESIAN_POINT ( 'NONE',  ( -5.000000000000003553, -8.660254037844383745, -72.99999999999998579 ) ) ;
#21839=CARTESIAN_POINT ( 'NONE',  ( -10.81189881249999729, 6.242252689847871849, -141.9062500020484094 ) ) ;
#21841=ORIENTED_EDGE ( 'NONE', *, *, #15733, .T. ) ;
#21843=CARTESIAN_POINT ( 'NONE',  ( 9.999999999999996447, -5.773502691896262640, -119.5000000040967763 ) ) ;
#21845=CARTESIAN_POINT ( 'NONE',  ( -5.405949406250003975, -9.363379034771801557, -76.84375000204838102 ) ) ;
#21850=CARTESIAN_POINT ( 'NONE',  ( -10.81189881249999729, 6.242252689847871849, -41.40625000204836681 ) ) ;
#21859=EDGE_CURVE ( 'NONE', #36790, #41954, #28678, .T. ) ;
#21861=( BOUNDED_CURVE ( )  B_SPLINE_CURVE ( 2, ( #35787, #18730, #22829, #2351, #12660, #2138, #39010 ),
 .UNSPECIFIED., .F., .F. ) 
 B_SPLINE_CURVE_WITH_KNOTS ( ( 3, 2, 2, 3 ),
 ( 0.3731343283582090331, 0.3743781094527363629, 0.3756218905472638037, 0.3768656716417911334 ),
 .UNSPECIFIED. ) 
 CURVE ( )  GEOMETRIC_REPRESENTATION_ITEM ( )  RATIONAL_B_SPLINE_CURVE ( ( 0.9999999999999940048, 0.8660254037844447028, 1.000000000000000000, 0.8660254037844387076, 1.000000000000000000, 0.8660254037844267172, 1.000000000000011990 ) ) 
 REPRESENTATION_ITEM ( '' )  );
#21867=CARTESIAN_POINT ( 'NONE',  ( -10.00000000000012790, -5.773502691896177375, -176.6250000000000284 ) ) ;
#21868=CARTESIAN_POINT ( 'NONE',  ( 10.81189881249999729, 0.000000000000000000, -133.3437500020484094 ) ) ;
#21869=CARTESIAN_POINT ( 'NONE',  ( -10.81189881249999907, -6.242252689847864744, -140.1562500020484094 ) ) ;
#21870=CARTESIAN_POINT ( 'NONE',  ( -10.81189881249999729, 6.242252689847871849, -143.2187500020483810 ) ) ;
#21874=CARTESIAN_POINT ( 'NONE',  ( -9.999999999999998224, 1.224646799147353059E-15, -175.2500000000000284 ) ) ;
#21879=CARTESIAN_POINT ( 'NONE',  ( -10.81189881249999907, -6.242252689847864744, -166.9687500020484094 ) ) ;
#21883=CARTESIAN_POINT ( 'NONE',  ( -5.405949406249996869, 9.363379034771805109, -43.03125000204838102 ) ) ;
#21885=CARTESIAN_POINT ( 'NONE',  ( 9.999999999999998224, 0.000000000000000000, -100.9999999999999858 ) ) ;
#21887=CARTESIAN_POINT ( 'NONE',  ( 5.405949406249999534, 9.363379034771803333, -130.2812500020483810 ) ) ;
#21888=CARTESIAN_POINT ( 'NONE',  ( -9.999999999999998224, 5.773502691896259087, -142.7500000040967905 ) ) ;
#21892=CARTESIAN_POINT ( 'NONE',  ( 5.405949406249999534, 9.363379034771803333, -170.5937500020484094 ) ) ;
#21894=CARTESIAN_POINT ( 'NONE',  ( 4.999999999999992006, -8.660254037844389075, -155.2500000000000000 ) ) ;
#21895=CARTESIAN_POINT ( 'NONE',  ( 5.405949406249992428, -9.363379034771808662, -70.78125000204838102 ) ) ;
#21898=VECTOR ( 'NONE', #27556, 1000.000000000000000 ) ;
#21901=ORIENTED_EDGE ( 'NONE', *, *, #8538, .F. ) ;
#21904=CARTESIAN_POINT ( 'NONE',  ( 9.999999999999998224, 0.000000000000000000, -117.8750000040967905 ) ) ;
#21906=ORIENTED_EDGE ( 'NONE', *, *, #39107, .T. ) ;
#21907=CARTESIAN_POINT ( 'NONE',  ( -10.00000000000019362, -5.773502691896140959, -178.5000000040968189 ) ) ;
#21909=ORIENTED_EDGE ( 'NONE', *, *, #12806, .F. ) ;
#21911=CARTESIAN_POINT ( 'NONE',  ( -9.999999999999998224, 1.224646799147353059E-15, -122.7500000000000000 ) ) ;
#21917=CARTESIAN_POINT ( 'NONE',  ( -10.00000000000000000, -5.773502691896251982, -35.62499999999996447 ) ) ;
#21920=CARTESIAN_POINT ( 'NONE',  ( 7.644554776091147741E-16, 12.48450537969573659, -158.4687500020483810 ) ) ;
#21921=CARTESIAN_POINT ( 'NONE',  ( 10.81189881249999551, -6.242252689847874514, -167.9687500020483810 ) ) ;
#21923=CARTESIAN_POINT ( 'NONE',  ( 5.000000000000000000, 8.660254037844385522, -132.2499999999999716 ) ) ;
#21924=CARTESIAN_POINT ( 'NONE',  ( 10.00000000000000000, 5.773502691896255534, -198.3750000000000000 ) ) ;
#21927=VECTOR ( 'NONE', #11773, 1000.000000000000000 ) ;
#21931=CARTESIAN_POINT ( 'NONE',  ( 10.81189881249999729, 0.000000000000000000, -70.53125000204838102 ) ) ;
#21933=CARTESIAN_POINT ( 'NONE',  ( 5.000000000000000000, 8.660254037844385522, -124.7500000000000000 ) ) ;
#21934=ORIENTED_EDGE ( 'NONE', *, *, #5893, .F. ) ;
#21935=CARTESIAN_POINT ( 'NONE',  ( -10.81189881249999729, 1.324075727343319199E-15, -150.7812500020483810 ) ) ;
#21936=CARTESIAN_POINT ( 'NONE',  ( -10.81189881249999907, -6.242252689847864744, -162.6562500020483810 ) ) ;
#21939=CARTESIAN_POINT ( 'NONE',  ( 10.81189881249999907, 6.242252689847868297, -98.71875000204838102 ) ) ;
#21942=CARTESIAN_POINT ( 'NONE',  ( 10.81189881249999907, 6.242252689847868297, 0.09374999795164208616 ) ) ;
#21945=CARTESIAN_POINT ( 'NONE',  ( 4.999999999999992006, -8.660254037844389075, -144.7500000000000000 ) ) ;
#21946=CARTESIAN_POINT ( 'NONE',  ( -10.81189881249999907, -6.242252689847864744, -92.15625000204839523 ) ) ;
#21948=CARTESIAN_POINT ( 'NONE',  ( -4.999999999999996447, 8.660254037844387298, -67.87500000409677625 ) ) ;
#21950=CARTESIAN_POINT ( 'NONE',  ( 5.405949406249999534, 9.363379034771803333, -23.59375000204835970 ) ) ;
#21953=CARTESIAN_POINT ( 'NONE',  ( 5.405949406249992428, -9.363379034771808662, -16.78125000204835970 ) ) ;
#21963=ORIENTED_EDGE ( 'NONE', *, *, #31149, .F. ) ;
#21969=EDGE_CURVE ( 'NONE', #35880, #18233, #19581, .T. ) ;
#21970=EDGE_CURVE ( 'NONE', #36790, #1002, #5963, .T. ) ;
#21974=CARTESIAN_POINT ( 'NONE',  ( -5.405949406249996869, 9.363379034771805109, -161.5312500020484094 ) ) ;
#21976=CARTESIAN_POINT ( 'NONE',  ( 0.000000000000000000, 0.000000000000000000, -176.9999999999999432 ) ) ;
#21980=CARTESIAN_POINT ( 'NONE',  ( -2.293366432827344421E-15, -12.48450537969573659, -87.21875000204838102 ) ) ;
#21981=CARTESIAN_POINT ( 'NONE',  ( -10.81189881249999729, 6.242252689847871849, -192.7187500020483810 ) ) ;
#21982=CARTESIAN_POINT ( 'NONE',  ( -5.405949406250003975, -9.363379034771801557, -93.53125000204838102 ) ) ;
#21986=CARTESIAN_POINT ( 'NONE',  ( -5.000000000000003553, -8.660254037844383745, -151.0000000000000000 ) ) ;
#21987=CARTESIAN_POINT ( 'NONE',  ( -10.81189881249999729, 1.324075727343319199E-15, -177.7812500020484094 ) ) ;
#21988=CARTESIAN_POINT ( 'NONE',  ( 10.81189881249999729, 0.000000000000000000, -189.0312500020484094 ) ) ;
#21990=CARTESIAN_POINT ( 'NONE',  ( 10.00000000000000000, 5.773502691896255534, -165.7500000040967905 ) ) ;
#21992=CARTESIAN_POINT ( 'NONE',  ( 5.405949406249992428, -9.363379034771808662, -12.09375000204834727 ) ) ;
#21993=CARTESIAN_POINT ( 'NONE',  ( -9.999999999999998224, 1.224646799147353059E-15, -162.1250000040967905 ) ) ;
#21994=CARTESIAN_POINT ( 'NONE',  ( -10.81189881249999729, 6.242252689847871849, -123.7187500020483952 ) ) ;
#21996=CARTESIAN_POINT ( 'NONE',  ( -5.405949406250003975, -9.363379034771801557, -20.03125000204836326 ) ) ;
#21998=EDGE_CURVE ( 'NONE', #8116, #35398, #21225, .T. ) ;
#22001=CARTESIAN_POINT ( 'NONE',  ( -10.81189881249999907, -6.242252689847864744, -114.6562500020483952 ) ) ;
#22004=CARTESIAN_POINT ( 'NONE',  ( 9.999999999999998224, 0.000000000000000000, -95.37500000409677625 ) ) ;
#22007=CARTESIAN_POINT ( 'NONE',  ( -5.405949406249996869, 9.363379034771805109, -53.34375000204835970 ) ) ;
#22015=CARTESIAN_POINT ( 'NONE',  ( 4.999999999999992006, -8.660254037844389075, -19.12500000409675494 ) ) ;
#22019=ORIENTED_EDGE ( 'NONE', *, *, #25715, .F. ) ;
#22021=EDGE_CURVE ( 'NONE', #7904, #30038, #30320, .T. ) ;
#22022=CARTESIAN_POINT ( 'NONE',  ( 5.000000000000000000, 8.660254037844385522, -143.1250000040967905 ) ) ;
#22030=CARTESIAN_POINT ( 'NONE',  ( 9.999999999999998224, 1.224646799147353059E-15, -99.99999999999998579 ) ) ;
#22033=CARTESIAN_POINT ( 'NONE',  ( 10.81189881249999907, 6.242252689847868297, -191.9062500020484094 ) ) ;
#22035=CARTESIAN_POINT ( 'NONE',  ( -5.000000000000003553, -8.660254037844383745, -133.0000000000000000 ) ) ;
#22038=CARTESIAN_POINT ( 'NONE',  ( -2.293366432827344421E-15, -12.48450537969573659, -106.7187500020483668 ) ) ;
#22040=CARTESIAN_POINT ( 'NONE',  ( -10.81189881249999907, -6.242252689847864744, -119.1562500020484237 ) ) ;
#22042=CARTESIAN_POINT ( 'NONE',  ( -10.81189881249999729, -6.242252689847864744, -124.9687500020483810 ) ) ;
#22045=CARTESIAN_POINT ( 'NONE',  ( -9.999999999999998224, 1.224646799147353059E-15, -143.7500000000000000 ) ) ;
#22046=CARTESIAN_POINT ( 'NONE',  ( 4.999999999999992006, -8.660254037844389075, -15.74999999999995914 ) ) ;
#22049=CARTESIAN_POINT ( 'NONE',  ( 10.00000000000000000, 5.773502691896255534, -188.2500000040968189 ) ) ;
#22051=CARTESIAN_POINT ( 'NONE',  ( -5.405949406250003975, -9.363379034771801557, -39.34375000204837391 ) ) ;
#22053=CARTESIAN_POINT ( 'NONE',  ( -10.81189881249999729, 6.242252689847871849, -146.2187500020483810 ) ) ;
#22056=CARTESIAN_POINT ( 'NONE',  ( -9.999999999999998224, 1.224646799147353059E-15, -76.24999999999998579 ) ) ;
#22057=CARTESIAN_POINT ( 'NONE',  ( -10.81189881249999729, 6.242252689847871849, -137.4062500020484094 ) ) ;
#22062=CARTESIAN_POINT ( 'NONE',  ( 4.999999999999992006, -8.660254037844389075, -116.6250000040967905 ) ) ;
#22064=CARTESIAN_POINT ( 'NONE',  ( -2.293366432827344421E-15, -12.48450537969573659, -75.21875000204839523 ) ) ;
#22068=CARTESIAN_POINT ( 'NONE',  ( -10.81189881249999729, 6.242252689847871849, -36.90625000204835970 ) ) ;
#22071=VECTOR ( 'NONE', #3861, 1000.000000000000000 ) ;
#22075=ORIENTED_EDGE ( 'NONE', *, *, #22890, .T. ) ;
#22077=EDGE_LOOP ( 'NONE', ( #27259, #430, #6772, #38977 ) ) ;
#22086=CARTESIAN_POINT ( 'NONE',  ( -10.81189881249999729, 6.242252689847871849, -137.2187500020483810 ) ) ;
#22087=CARTESIAN_POINT ( 'NONE',  ( -2.293366432827344421E-15, -12.48450537969573659, -141.4062500020483810 ) ) ;
#22088=CARTESIAN_POINT ( 'NONE',  ( 0.000000000000000000, 0.000000000000000000, -99.99999999999998579 ) ) ;
#22089=CARTESIAN_POINT ( 'NONE',  ( 10.81189881249999551, -6.242252689847874514, -149.9687500020483810 ) ) ;
#22092=CARTESIAN_POINT ( 'NONE',  ( -9.999999999999998224, 1.224646799147353059E-15, -173.7500000000000284 ) ) ;
#22098=CARTESIAN_POINT ( 'NONE',  ( -9.187887513909968717, -4.550206982411138412, -99.99999999999997158 ) ) ;
#22099=CARTESIAN_POINT ( 'NONE',  ( -5.405949406250003975, -9.363379034771801557, -171.3437500020484094 ) ) ;
#22103=CARTESIAN_POINT ( 'NONE',  ( -2.293366432827344421E-15, -12.48450537969573659, -36.40625000204835970 ) ) ;
#22105=CARTESIAN_POINT ( 'NONE',  ( 5.000000000000000000, 8.660254037844385522, -97.74999999999998579 ) ) ;
#22106=EDGE_LOOP ( 'NONE', ( #27485, #38101, #37616, #32384 ) ) ;
#22107=CARTESIAN_POINT ( 'NONE',  ( -2.293366432827344421E-15, -12.48450537969573659, -121.9062500020483952 ) ) ;
#22108=CARTESIAN_POINT ( 'NONE',  ( -2.121150477449813534E-15, -11.54700538379251284, -140.7500000040967905 ) ) ;
#22113=CARTESIAN_POINT ( 'NONE',  ( 5.405949406249999534, 9.363379034771803333, -70.28125000204838102 ) ) ;
#22114=EDGE_CURVE ( 'NONE', #4599, #4329, #3625, .T. ) ;
#22126=CARTESIAN_POINT ( 'NONE',  ( -9.999999999999742428, -5.773502691896402084, -100.5000000040967905 ) ) ;
#22134=ORIENTED_EDGE ( 'NONE', *, *, #32284, .T. ) ;
#22135=CARTESIAN_POINT ( 'NONE',  ( -9.999999999999479527, -5.773502691896549521, -112.5000000040967478 ) ) ;
#22136=CARTESIAN_POINT ( 'NONE',  ( 5.000000000000000000, 8.660254037844385522, -33.24999999999997158 ) ) ;
#22139=CARTESIAN_POINT ( 'NONE',  ( 5.405949406249999534, 9.363379034771803333, -157.0937500020483810 ) ) ;
#22140=CARTESIAN_POINT ( 'NONE',  ( 7.644554776091147741E-16, 12.48450537969573659, -173.4687500020483810 ) ) ;
#22141=EDGE_CURVE ( 'NONE', #36280, #15509, #37495, .T. ) ;
#22143=CARTESIAN_POINT ( 'NONE',  ( 7.070501591499376803E-16, 11.54700538379251284, -132.1250000000000000 ) ) ;
#22144=CARTESIAN_POINT ( 'NONE',  ( -2.121150477449813534E-15, -11.54700538379251284, -194.3750000000000284 ) ) ;
#22149=CARTESIAN_POINT ( 'NONE',  ( 10.81189881249999551, -6.242252689847874514, -58.65625000204838813 ) ) ;
#22151=CARTESIAN_POINT ( 'NONE',  ( 9.999999999999996447, -5.773502691896262640, -120.6250000000000000 ) ) ;
#22154=CARTESIAN_POINT ( 'NONE',  ( 10.81189881249999729, 6.242252689847867408, -139.4062500020484094 ) ) ;
#22155=CARTESIAN_POINT ( 'NONE',  ( -10.81189881249999729, 1.324075727343319199E-15, -158.2812500020484094 ) ) ;
#22157=CARTESIAN_POINT ( 'NONE',  ( -9.999999999999998224, 1.224646799147353059E-15, -118.2500000000000000 ) ) ;
#22158=CARTESIAN_POINT ( 'NONE',  ( -10.81189881249999907, -6.242252689847864744, -91.96875000204838102 ) ) ;
#22159=ORIENTED_EDGE ( 'NONE', *, *, #20529, .F. ) ;
#22161=CARTESIAN_POINT ( 'NONE',  ( 10.81189881249999551, -6.242252689847874514, -0.1562500020483581498 ) ) ;
#22163=CARTESIAN_POINT ( 'NONE',  ( -5.000000000000003553, -8.660254037844383745, -169.3750000040967905 ) ) ;
#22165=CARTESIAN_POINT ( 'NONE',  ( 7.644554776091147741E-16, 12.48450537969573659, -89.65625000204839523 ) ) ;
#22167=CARTESIAN_POINT ( 'NONE',  ( -4.999999999999996447, 8.660254037844387298, -70.87500000409677625 ) ) ;
#22168=CARTESIAN_POINT ( 'NONE',  ( -9.999999999999998224, 0.000000000000000000, -99.99999999999998579 ) ) ;
#22169=CARTESIAN_POINT ( 'NONE',  ( -5.405949406250003975, -9.363379034771801557, -22.84375000204835615 ) ) ;
#22173=CARTESIAN_POINT ( 'NONE',  ( -5.405949406249996869, 9.363379034771805109, -22.03125000204836326 ) ) ;
#22189=DIRECTION ( 'NONE',  ( -0.000000000000000000, -0.000000000000000000, -1.000000000000000000 ) ) ;
#22190=CARTESIAN_POINT ( 'NONE',  ( 9.876501204336495476, -2.277692215602485692, -100.0000000000000142 ) ) ;
#22193=CARTESIAN_POINT ( 'NONE',  ( 5.405949406249999534, 9.363379034771803333, -155.7812500020484094 ) ) ;
#22198=CARTESIAN_POINT ( 'NONE',  ( -2.293366432827344421E-15, -12.48450537969573659, -82.71875000204838102 ) ) ;
#22199=CARTESIAN_POINT ( 'NONE',  ( -10.81189881249999729, 1.324075727343319199E-15, -89.28125000204838102 ) ) ;
#22203=CARTESIAN_POINT ( 'NONE',  ( -10.81189881249999729, 6.242252689847871849, -176.4062500020484094 ) ) ;
#22204=CARTESIAN_POINT ( 'NONE',  ( -10.81189881249999907, -6.242252689847864744, -191.1562500020484094 ) ) ;
#22206=CARTESIAN_POINT ( 'NONE',  ( -4.999999999999996447, 8.660254037844387298, -166.8750000040967905 ) ) ;
#22208=CARTESIAN_POINT ( 'NONE',  ( -10.81189881249999907, -6.242252689847864744, -10.96875000204835970 ) ) ;
#22209=CARTESIAN_POINT ( 'NONE',  ( 7.070501591499376803E-16, 11.54700538379251284, -162.5000000040967905 ) ) ;
#22210=CARTESIAN_POINT ( 'NONE',  ( 10.81189881249999551, -6.242252689847874514, -122.9687500020483810 ) ) ;
#22212=CARTESIAN_POINT ( 'NONE',  ( 5.405949406249999534, 9.363379034771803333, -22.28125000204836326 ) ) ;
#22214=LINE ( 'NONE', #12269, #19667 ) ;
#22215=CARTESIAN_POINT ( 'NONE',  ( -5.405949406249996869, 9.363379034771805109, -118.0312500020483952 ) ) ;
#22219=CARTESIAN_POINT ( 'NONE',  ( 7.070501591499377789E-16, 11.54700538379251284, -93.50000000409677625 ) ) ;
#22222=CARTESIAN_POINT ( 'NONE',  ( -5.405949406249996869, 9.363379034771805109, -48.84375000204838102 ) ) ;
#22228=CARTESIAN_POINT ( 'NONE',  ( -5.000000000000003553, -8.660254037844383745, -22.37500000409675494 ) ) ;
#22230=AXIS2_PLACEMENT_3D ( 'NONE', #14751, #5066, #18214 ) ;
#22242=CARTESIAN_POINT ( 'NONE',  ( -9.999999999999996447, 5.773502691896259975, -170.8750000000000000 ) ) ;
#22245=CARTESIAN_POINT ( 'NONE',  ( -10.81189881249999729, 1.324075727343319199E-15, -177.7812500020484094 ) ) ;
#22248=ADVANCED_FACE ( 'NONE', ( #393 ), #7705, .F. ) ;
#22250=CARTESIAN_POINT ( 'NONE',  ( 7.644554776091147741E-16, 12.48450537969573659, -108.9687500020483952 ) ) ;
#22252=CARTESIAN_POINT ( 'NONE',  ( 5.405949406249992428, -9.363379034771808662, -117.2812500020483952 ) ) ;
#22254=CARTESIAN_POINT ( 'NONE',  ( 7.644554776091147741E-16, 12.48450537969573659, -119.4687500020483668 ) ) ;
#22256=CARTESIAN_POINT ( 'NONE',  ( 5.000000000000000000, 8.660254037844385522, -157.7500000000000000 ) ) ;
#22257=CARTESIAN_POINT ( 'NONE',  ( 4.999999999999992006, -8.660254037844389075, -137.2499999999999716 ) ) ;
#22258=CARTESIAN_POINT ( 'NONE',  ( -9.999999999999998224, 1.224646799147353059E-15, -14.74999999999995737 ) ) ;
#22262=CARTESIAN_POINT ( 'NONE',  ( 5.000000000000000000, 8.660254037844385522, -189.6250000040967905 ) ) ;
#22264=CARTESIAN_POINT ( 'NONE',  ( -10.81189881249999729, 1.324075727343319199E-15, -41.09375000204837391 ) ) ;
#22265=CARTESIAN_POINT ( 'NONE',  ( 9.999999999999479527, 5.773502691896553074, -149.2500000040967905 ) ) ;
#22266=CARTESIAN_POINT ( 'NONE',  ( -2.293366432827344421E-15, -12.48450537969573659, -148.7187500020484094 ) ) ;
#22269=CARTESIAN_POINT ( 'NONE',  ( 9.999999999999998224, 0.000000000000000000, -66.49999999999997158 ) ) ;
#22270=CARTESIAN_POINT ( 'NONE',  ( -5.405949406249996869, 9.363379034771805109, -139.0312500020484094 ) ) ;
#22274=CARTESIAN_POINT ( 'NONE',  ( -4.999999999999996447, 8.660254037844387298, -112.8750000040967763 ) ) ;
#22276=CARTESIAN_POINT ( 'NONE',  ( 7.644554776091147741E-16, 12.48450537969573659, -71.46875000204835260 ) ) ;
#22282=CARTESIAN_POINT ( 'NONE',  ( -5.405949406250003975, -9.363379034771801557, -36.53125000204837391 ) ) ;
#22283=EDGE_CURVE ( 'NONE', #1789, #22578, #830, .T. ) ;
#22288=CARTESIAN_POINT ( 'NONE',  ( -9.999999999999998224, 1.224646799147353059E-15, -165.1250000040967905 ) ) ;
#22294=CARTESIAN_POINT ( 'NONE',  ( -10.00000000000019185, -5.773502691896140071, -177.0000000040967620 ) ) ;
#22301=CARTESIAN_POINT ( 'NONE',  ( 10.81189881249999907, 6.242252689847868297, -137.7187500020484094 ) ) ;
#22302=CARTESIAN_POINT ( 'NONE',  ( 5.405949406249999534, 9.363379034771803333, -139.2812500020483810 ) ) ;
#22304=CARTESIAN_POINT ( 'NONE',  ( 10.81189881249999729, 6.242252689847867408, -143.7187500020484094 ) ) ;
#22305=DIRECTION ( 'NONE',  ( -0.000000000000000000, -0.000000000000000000, -1.000000000000000000 ) ) ;
#22306=CARTESIAN_POINT ( 'NONE',  ( 5.000000000000000000, 8.660254037844385522, -163.7500000000000000 ) ) ;
#22308=CARTESIAN_POINT ( 'NONE',  ( 9.999999999999998224, 0.000000000000000000, -153.8750000040967905 ) ) ;
#22310=CARTESIAN_POINT ( 'NONE',  ( -5.405949406249996869, 9.363379034771805109, -63.84375000204836681 ) ) ;
#22312=CARTESIAN_POINT ( 'NONE',  ( -5.405949406250003975, -9.363379034771801557, -169.8437500020484094 ) ) ;
#22316=CARTESIAN_POINT ( 'NONE',  ( -10.81189881249999729, 6.242252689847871849, -38.40625000204835970 ) ) ;
#22318=CARTESIAN_POINT ( 'NONE',  ( -4.999999999999996447, 8.660254037844387298, -97.49999999999998579 ) ) ;
#22320=CARTESIAN_POINT ( 'NONE',  ( 10.81189881249999729, 0.000000000000000000, -117.0312500020483952 ) ) ;
#22321=CARTESIAN_POINT ( 'NONE',  ( -9.999999999999998224, 5.773502691896259087, -138.2500000040967905 ) ) ;
#22322=CARTESIAN_POINT ( 'NONE',  ( -9.999999999999998224, 1.224646799147353059E-15, -145.6250000040967905 ) ) ;
#22325=CARTESIAN_POINT ( 'NONE',  ( 9.999999999999998224, 0.000000000000000000, -159.5000000000000000 ) ) ;
#22326=CARTESIAN_POINT ( 'NONE',  ( -2.293366432827344421E-15, -12.48450537969573659, -63.40625000204838813 ) ) ;
#22338=CARTESIAN_POINT ( 'NONE',  ( 4.999999999999992006, -8.660254037844389075, -100.1250000040967905 ) ) ;
#22345=ORIENTED_EDGE ( 'NONE', *, *, #29898, .F. ) ;
#22346=CYLINDRICAL_SURFACE ( 'NONE', #21536, 9.999999999999998224 ) ;
#22347=CARTESIAN_POINT ( 'NONE',  ( 10.00000000000000000, 5.773502691896255534, -31.87499999999995737 ) ) ;
#22350=CARTESIAN_POINT ( 'NONE',  ( -10.81189881249999729, 6.242252689847871849, -155.2187500020483810 ) ) ;
#22351=CARTESIAN_POINT ( 'NONE',  ( 10.81189881249999551, -6.242252689847874514, -170.9687500020483810 ) ) ;
#22354=CARTESIAN_POINT ( 'NONE',  ( -9.999999999999998224, 5.773502691896259087, -196.3750000000000568 ) ) ;
#22359=CARTESIAN_POINT ( 'NONE',  ( -5.405949406249996869, 9.363379034771805109, -59.53125000204836681 ) ) ;
#22361=CARTESIAN_POINT ( 'NONE',  ( -5.000000000000003553, -8.660254037844383745, -119.5000000000000000 ) ) ;
#22363=CARTESIAN_POINT ( 'NONE',  ( -10.81189881249999729, -6.242252689847864744, -143.1562500020484094 ) ) ;
#22364=CARTESIAN_POINT ( 'NONE',  ( -10.81189881249999729, 1.324075727343319199E-15, -155.2812500020484094 ) ) ;
#22366=CARTESIAN_POINT ( 'NONE',  ( 5.405949406249992428, -9.363379034771808662, -88.59375000204838102 ) ) ;
#22367=ORIENTED_EDGE ( 'NONE', *, *, #36507, .T. ) ;
#22369=CARTESIAN_POINT ( 'NONE',  ( -2.293366432827344421E-15, -12.48450537969573659, -186.2187500020484094 ) ) ;
#22371=CARTESIAN_POINT ( 'NONE',  ( 7.070501591499376803E-16, 11.54700538379251284, -165.1250000000000000 ) ) ;
#22373=CARTESIAN_POINT ( 'NONE',  ( 10.81189881249999729, 0.000000000000000000, -82.53125000204838102 ) ) ;
#22375=( BOUNDED_CURVE ( )  B_SPLINE_CURVE ( 2, ( #2136, #41600, #15476, #18728, #18943, #9228, #25437 ),
 .UNSPECIFIED., .F., .F. ) 
 B_SPLINE_CURVE_WITH_KNOTS ( ( 3, 2, 2, 3 ),
 ( 0.1305970149253731227, 0.1318407960199005080, 0.1330845771144278378, 0.1343283582089551953 ),
 .UNSPECIFIED. ) 
 CURVE ( )  GEOMETRIC_REPRESENTATION_ITEM ( )  RATIONAL_B_SPLINE_CURVE ( ( 1.000000000000000000, 0.8660254037844387076, 1.000000000000000000, 0.8660254037844387076, 1.000000000000000000, 0.8660254037844417052, 0.9999999999999970024 ) ) 
 REPRESENTATION_ITEM ( '' )  );
#22376=CARTESIAN_POINT ( 'NONE',  ( 5.000000000000000000, 8.660254037844385522, -59.12500000409676204 ) ) ;
#22377=CARTESIAN_POINT ( 'NONE',  ( 9.999999999999998224, 0.000000000000000000, -158.3750000040967905 ) ) ;
#22378=CARTESIAN_POINT ( 'NONE',  ( -2.293366432827344421E-15, -12.48450537969573659, -15.21875000204836326 ) ) ;
#22381=CARTESIAN_POINT ( 'NONE',  ( 10.81189881249999551, -6.242252689847874514, -18.15625000204837391 ) ) ;
#22391=ORIENTED_EDGE ( 'NONE', *, *, #8821, .F. ) ;
#22399=CARTESIAN_POINT ( 'NONE',  ( 9.999999999999998224, 0.000000000000000000, -138.8750000040968189 ) ) ;
#22401=CARTESIAN_POINT ( 'NONE',  ( 10.81189881249999551, -6.242252689847874514, -159.1562500020484094 ) ) ;
#22407=CARTESIAN_POINT ( 'NONE',  ( -5.405949406250003975, -9.363379034771801557, -78.34375000204838102 ) ) ;
#22408=CARTESIAN_POINT ( 'NONE',  ( -5.405949406250003975, -9.363379034771801557, -83.03125000204838102 ) ) ;
#22411=CARTESIAN_POINT ( 'NONE',  ( -2.293366432827344421E-15, -12.48450537969573659, -163.9062500020483810 ) ) ;
#22412=CARTESIAN_POINT ( 'NONE',  ( -2.293366432827344421E-15, -12.48450537969573659, -178.9062500020484379 ) ) ;
#22414=CARTESIAN_POINT ( 'NONE',  ( 10.00000000000000000, 5.773502691896255534, -153.7500000040967905 ) ) ;
#22416=CARTESIAN_POINT ( 'NONE',  ( -10.81189881249999907, -6.242252689847864744, -3.468750002048353931 ) ) ;
#22418=CARTESIAN_POINT ( 'NONE',  ( 10.81189881249999551, -6.242252689847874514, -110.9687500020483810 ) ) ;
#22420=CARTESIAN_POINT ( 'NONE',  ( -10.81189881249999729, 6.242252689847871849, -12.90625000204836859 ) ) ;
#22423=CARTESIAN_POINT ( 'NONE',  ( -5.405949406250003975, -9.363379034771801557, -111.5312500020483810 ) ) ;
#22425=ORIENTED_EDGE ( 'NONE', *, *, #3654, .T. ) ;
#22426=CARTESIAN_POINT ( 'NONE',  ( 10.00000000000000000, 5.773502691896255534, -93.75000000409677625 ) ) ;
#22428=CARTESIAN_POINT ( 'NONE',  ( 10.81189881249999729, 0.000000000000000000, -43.34375000204837391 ) ) ;
#22433=CARTESIAN_POINT ( 'NONE',  ( 9.999999999999996447, -5.773502691896262640, -20.50000000409676915 ) ) ;
#22436=ORIENTED_EDGE ( 'NONE', *, *, #1201, .F. ) ;
#22437=CARTESIAN_POINT ( 'NONE',  ( -5.000000000000003553, -8.660254037844383745, -152.5000000000000000 ) ) ;
#22445=AXIS2_PLACEMENT_3D ( 'NONE', #25744, #15148, #2649 ) ;
#22446=( BOUNDED_CURVE ( )  B_SPLINE_CURVE ( 2, ( #30525, #17531, #10851, #11488, #24902, #40406, #8279 ),
 .UNSPECIFIED., .F., .F. ) 
 B_SPLINE_CURVE_WITH_KNOTS ( ( 3, 2, 2, 3 ),
 ( 0.4776119402985076756, 0.4788557213930350054, 0.4800995024875623352, 0.4813432835820896649 ),
 .UNSPECIFIED. ) 
 CURVE ( )  GEOMETRIC_REPRESENTATION_ITEM ( )  RATIONAL_B_SPLINE_CURVE ( ( 0.9999999999999761302, 0.8660254037844625774, 1.000000000000000000, 0.8660254037844387076, 1.000000000000000000, 0.8660254037844267172, 1.000000000000011990 ) ) 
 REPRESENTATION_ITEM ( '' )  );
#22450=CARTESIAN_POINT ( 'NONE',  ( 10.81189881249999907, 6.242252689847868297, -179.9062500020484094 ) ) ;
#22452=CARTESIAN_POINT ( 'NONE',  ( 9.999999999999998224, 0.000000000000000000, -132.5000000000000000 ) ) ;
#22455=CARTESIAN_POINT ( 'NONE',  ( -10.81189881249999729, 1.324075727343319199E-15, -99.59375000204838102 ) ) ;
#22457=CARTESIAN_POINT ( 'NONE',  ( 10.81189881249999907, 6.242252689847868297, -112.4062500020483952 ) ) ;
#22459=CARTESIAN_POINT ( 'NONE',  ( -2.293366432827344421E-15, -12.48450537969573659, -118.7187500020483668 ) ) ;
#22462=CARTESIAN_POINT ( 'NONE',  ( 4.999999999999992006, -8.660254037844389075, -135.7499999999999716 ) ) ;
#22463=CARTESIAN_POINT ( 'NONE',  ( -2.121150477449813534E-15, -11.54700538379251284, -0.8749999999999591438 ) ) ;
#22466=CARTESIAN_POINT ( 'NONE',  ( 5.000000000000000000, 8.660254037844385522, -185.1250000040967905 ) ) ;
#22468=CARTESIAN_POINT ( 'NONE',  ( 5.405949406249992428, -9.363379034771808662, -34.59375000204836681 ) ) ;
#22469=CARTESIAN_POINT ( 'NONE',  ( 10.00000000000051159, -5.773502691895965988, -142.0000000040967905 ) ) ;
#22470=CARTESIAN_POINT ( 'NONE',  ( 5.405949406249999534, 9.363379034771803333, -140.5937500020483810 ) ) ;
#22474=CARTESIAN_POINT ( 'NONE',  ( -2.121150477449813534E-15, -11.54700538379251284, -68.37499999999998579 ) ) ;
#22475=CARTESIAN_POINT ( 'NONE',  ( -5.405949406250003975, -9.363379034771801557, -138.5312500020484094 ) ) ;
#22477=VERTEX_POINT ( 'NONE', #34470 ) ;
#22479=CARTESIAN_POINT ( 'NONE',  ( -5.000000000000003553, -8.660254037844383745, -115.3750000040967905 ) ) ;
#22481=CARTESIAN_POINT ( 'NONE',  ( 5.405949406249992428, -9.363379034771808662, -75.09375000204838102 ) ) ;
#22487=CARTESIAN_POINT ( 'NONE',  ( 5.000000000000000000, 8.660254037844385522, -42.62500000409677625 ) ) ;
#22488=CARTESIAN_POINT ( 'NONE',  ( -2.293366432827344421E-15, -12.48450537969573659, -33.40625000204835970 ) ) ;
#22492=CARTESIAN_POINT ( 'NONE',  ( -4.999999999999996447, 8.660254037844387298, -153.0000000000000000 ) ) ;
#22507=DIRECTION ( 'NONE',  ( 0.000000000000000000, 0.000000000000000000, -1.000000000000000000 ) ) ;
#22508=CARTESIAN_POINT ( 'NONE',  ( 5.405949406249992428, -9.363379034771808662, -129.0937500020483810 ) ) ;
#22509=CARTESIAN_POINT ( 'NONE',  ( -10.81189881249999729, 6.242252689847871849, -143.4062500020484094 ) ) ;
#22511=CARTESIAN_POINT ( 'NONE',  ( -5.405949406250003975, -9.363379034771801557, -147.3437500020483810 ) ) ;
#22515=CARTESIAN_POINT ( 'NONE',  ( -9.999999999999998224, 5.773502691896259087, -166.3749999999999716 ) ) ;
#22518=CARTESIAN_POINT ( 'NONE',  ( 7.644554776091147741E-16, 12.48450537969573659, -57.96875000204837391 ) ) ;
#22519=CYLINDRICAL_SURFACE ( 'NONE', #29567, 9.999999999999998224 ) ;
#22520=CARTESIAN_POINT ( 'NONE',  ( -10.81189881249999729, 1.324075727343319199E-15, -170.0937500020484094 ) ) ;
#22526=CARTESIAN_POINT ( 'NONE',  ( -4.999999999999996447, 8.660254037844387298, -91.49999999999998579 ) ) ;
#22528=CARTESIAN_POINT ( 'NONE',  ( 10.81189881249999551, -6.242252689847874514, -121.6562500020483952 ) ) ;
#22529=CARTESIAN_POINT ( 'NONE',  ( -9.999999999999998224, 1.224646799147353059E-15, -144.1250000040967905 ) ) ;
#22533=CARTESIAN_POINT ( 'NONE',  ( -9.999999999999998224, 1.224646799147353059E-15, -160.2500000000000000 ) ) ;
#22534=CARTESIAN_POINT ( 'NONE',  ( -5.405949406250003975, -9.363379034771801557, -60.53125000204836681 ) ) ;
#22537=EDGE_CURVE ( 'NONE', #28346, #17318, #14360, .T. ) ;
#22542=CARTESIAN_POINT ( 'NONE',  ( 9.999999999999998224, 1.224646799147353059E-15, -99.99999999999998579 ) ) ;
#22548=VERTEX_POINT ( 'NONE', #24765 ) ;
#22554=CARTESIAN_POINT ( 'NONE',  ( 10.00000000000000000, 5.773502691896255534, -28.87499999999998579 ) ) ;
#22557=CARTESIAN_POINT ( 'NONE',  ( 10.81189881249999551, -6.242252689847874514, -160.4687500020484094 ) ) ;
#22558=CARTESIAN_POINT ( 'NONE',  ( -10.81189881249999729, 6.242252689847871849, -167.2187500020484379 ) ) ;
#22560=CARTESIAN_POINT ( 'NONE',  ( -5.000000000000003553, -8.660254037844383745, -127.0000000000000000 ) ) ;
#22561=CARTESIAN_POINT ( 'NONE',  ( -9.999999999999998224, 5.773502691896259087, -188.8750000000000568 ) ) ;
#22565=DIRECTION ( 'NONE',  ( -1.000000000000000000, 0.000000000000000000, 0.000000000000000000 ) ) ;
#22567=CARTESIAN_POINT ( 'NONE',  ( -10.81189881249999907, -6.242252689847864744, -57.65625000204838102 ) ) ;
#22569=CARTESIAN_POINT ( 'NONE',  ( 5.000000000000000000, 8.660254037844385522, -117.2500000000000000 ) ) ;
#22571=CARTESIAN_POINT ( 'NONE',  ( -10.81189881249999729, 6.242252689847871849, -143.4062500020484094 ) ) ;
#22572=CARTESIAN_POINT ( 'NONE',  ( -10.81189881249999907, -6.242252689847864744, -155.1562500020484094 ) ) ;
#22575=CARTESIAN_POINT ( 'NONE',  ( 10.00000000000051159, -5.773502691895965988, -179.1250000000000000 ) ) ;
#22576=CARTESIAN_POINT ( 'NONE',  ( -10.81189881249999729, 6.242252689847871849, -89.21875000204836681 ) ) ;
#22578=VERTEX_POINT ( 'NONE', #21714 ) ;
#22580=CARTESIAN_POINT ( 'NONE',  ( -2.293366432827344421E-15, -12.48450537969573659, -192.2187500020484379 ) ) ;
#22582=CARTESIAN_POINT ( 'NONE',  ( -9.999999999999998224, 1.224646799147353059E-15, -117.1250000040967905 ) ) ;
#22585=CARTESIAN_POINT ( 'NONE',  ( 5.405949406249999534, 9.363379034771803333, -85.28125000204838102 ) ) ;
#22587=CARTESIAN_POINT ( 'NONE',  ( -9.999999999999998224, 1.224646799147353059E-15, -61.62500000409676204 ) ) ;
#22588=CARTESIAN_POINT ( 'NONE',  ( -10.81189881249999729, 1.324075727343319199E-15, -17.09375000204835260 ) ) ;
#22589=CARTESIAN_POINT ( 'NONE',  ( 9.999999999999479527, 5.773502691896553074, -100.8749999999999716 ) ) ;
#22591=CARTESIAN_POINT ( 'NONE',  ( -10.81189881249999729, 6.242252689847871849, -15.90625000204837036 ) ) ;
#22601=VERTEX_POINT ( 'NONE', #11776 ) ;
#22603=B_SPLINE_CURVE_WITH_KNOTS ( 'NONE', 3,
 ( #4689, #35124, #41576, #15453, #11792, #21730, #1465, #21086, #34488, #4910, #18058, #28440, #15023, #24995, #5548, #24780, #18489, #31253, #2111, #37925, #21521, #18700, #31896, #1680, #2324, #28651, #41782, #14808 ),
 .UNSPECIFIED., .F., .F.,
 ( 4, 2, 2, 2, 2, 2, 2, 2, 2, 2, 2, 2, 2, 4 ),
 ( 0.000000000000000000, 0.001286352574009830274, 0.002572705148019660548, 0.005145410296039321096, 0.006431762870049149636, 0.007718115444058978175, 0.009004468018068808449, 0.01029082059207863699, 0.01286352574009829233, 0.01543623088811794768, 0.01672258346212777622, 0.01800893603613760649, 0.01929528861014742983, 0.02058164118415726010 ),
 .UNSPECIFIED. ) ;
#22612=( BOUNDED_CURVE ( )  B_SPLINE_CURVE ( 2, ( #34508, #15679, #35142, #8805, #18508, #2341, #6209 ),
 .UNSPECIFIED., .F., .F. ) 
 B_SPLINE_CURVE_WITH_KNOTS ( ( 3, 2, 2, 3 ),
 ( 0.1417910447761193959, 0.1430348258706467535, 0.1442786069651741387, 0.1455223880597014963 ),
 .UNSPECIFIED. ) 
 CURVE ( )  GEOMETRIC_REPRESENTATION_ITEM ( )  RATIONAL_B_SPLINE_CURVE ( ( 1.000000000000000000, 0.8660254037844387076, 1.000000000000000000, 0.8660254037844387076, 1.000000000000000000, 0.8660254037844387076, 1.000000000000000000 ) ) 
 REPRESENTATION_ITEM ( '' )  );
#22615=CARTESIAN_POINT ( 'NONE',  ( -2.293366432827344421E-15, -12.48450537969573659, -157.9062500020483810 ) ) ;
#22621=CARTESIAN_POINT ( 'NONE',  ( 5.405949406249999534, 9.363379034771803333, -79.09375000204838102 ) ) ;
#22622=CARTESIAN_POINT ( 'NONE',  ( -5.405949406250003975, -9.363379034771801557, -87.53125000204838102 ) ) ;
#22624=( BOUNDED_CURVE ( )  B_SPLINE_CURVE ( 2, ( #29915, #13477, #26668, #26878, #40033, #7238, #12167 ),
 .UNSPECIFIED., .F., .F. ) 
 B_SPLINE_CURVE_WITH_KNOTS ( ( 3, 2, 2, 3 ),
 ( 0.1156716417910447492, 0.1169154228855721483, 0.1181592039800995753, 0.1194029850746269744 ),
 .UNSPECIFIED. ) 
 CURVE ( )  GEOMETRIC_REPRESENTATION_ITEM ( )  RATIONAL_B_SPLINE_CURVE ( ( 1.000000000000003109, 0.8660254037844358210, 1.000000000000000000, 0.8660254037844387076, 1.000000000000000000, 0.8660254037844267172, 1.000000000000011990 ) ) 
 REPRESENTATION_ITEM ( '' )  );
#22626=CARTESIAN_POINT ( 'NONE',  ( -10.81189881249999729, 1.324075727343319199E-15, -165.7812500020484094 ) ) ;
#22627=CARTESIAN_POINT ( 'NONE',  ( 10.81189881249999551, -6.242252689847874514, -180.1562500020484379 ) ) ;
#22628=EDGE_CURVE ( 'NONE', #20876, #342, #27558, .T. ) ;
#22629=CARTESIAN_POINT ( 'NONE',  ( 10.00000000000000000, 5.773502691896255534, -159.7500000040967905 ) ) ;
#22631=CARTESIAN_POINT ( 'NONE',  ( 5.405949406249992428, -9.363379034771808662, -9.093750002048345493 ) ) ;
#22633=CARTESIAN_POINT ( 'NONE',  ( 10.81189881249999907, 6.242252689847868297, -115.2187500020483810 ) ) ;
#22635=CARTESIAN_POINT ( 'NONE',  ( 5.405949406249999534, 9.363379034771803333, -14.78125000204835793 ) ) ;
#22637=DIRECTION ( 'NONE',  ( -0.000000000000000000, -0.000000000000000000, -1.000000000000000000 ) ) ;
#22638=CARTESIAN_POINT ( 'NONE',  ( -10.81189881249999907, -6.242252689847864744, -111.6562500020483952 ) ) ;
#22642=CARTESIAN_POINT ( 'NONE',  ( 9.999999999999996447, -5.773502691896262640, -82.00000000409676204 ) ) ;
#22643=DIRECTION ( 'NONE',  ( -0.000000000000000000, -0.000000000000000000, -1.000000000000000000 ) ) ;
#22644=CARTESIAN_POINT ( 'NONE',  ( 5.405949406249992428, -9.363379034771808662, -43.59375000204837391 ) ) ;
#22648=CARTESIAN_POINT ( 'NONE',  ( -10.00000000000000000, -5.773502691896251982, -12.00000000409676204 ) ) ;
#22650=DIRECTION ( 'NONE',  ( -1.000000000000000000, 0.000000000000000000, 0.000000000000000000 ) ) ;
#22662=CARTESIAN_POINT ( 'NONE',  ( 7.644554776091147741E-16, 12.48450537969573659, -178.1562500020484094 ) ) ;
#22663=FACE_OUTER_BOUND ( 'NONE', #4444, .T. ) ;
#22668=CARTESIAN_POINT ( 'NONE',  ( 7.644554776091147741E-16, 12.48450537969573659, -102.9687500020483952 ) ) ;
#22670=CARTESIAN_POINT ( 'NONE',  ( 5.405949406249999534, 9.363379034771803333, -112.2812500020483952 ) ) ;
#22672=CARTESIAN_POINT ( 'NONE',  ( 10.81189881249999551, -6.242252689847874514, -115.4687500020483810 ) ) ;
#22676=CARTESIAN_POINT ( 'NONE',  ( -9.999999999999998224, 5.773502691896259087, -136.3750000000000000 ) ) ;
#22677=CARTESIAN_POINT ( 'NONE',  ( -9.999999999999998224, 5.773502691896259087, -7.374999999999964473 ) ) ;
#22682=CARTESIAN_POINT ( 'NONE',  ( 9.999999999999996447, -5.773502691896262640, -176.5000000040968189 ) ) ;
#22684=CARTESIAN_POINT ( 'NONE',  ( -10.81189881249999729, 1.324075727343319199E-15, -30.59375000204836326 ) ) ;
#22685=CARTESIAN_POINT ( 'NONE',  ( -9.999999999999998224, 1.224646799147353059E-15, -106.2499999999999858 ) ) ;
#22686=CARTESIAN_POINT ( 'NONE',  ( 10.81189881249999907, 6.242252689847868297, -136.2187500020483810 ) ) ;
#22688=CARTESIAN_POINT ( 'NONE',  ( -10.00000000000076916, 5.773502691895813221, -110.8749999999999574 ) ) ;
#22689=CARTESIAN_POINT ( 'NONE',  ( -9.999999999999998224, 5.773502691896259087, -67.37499999999998579 ) ) ;
#22690=CARTESIAN_POINT ( 'NONE',  ( -5.405949406249996869, 9.363379034771805109, -128.5312500020484094 ) ) ;
#22692=ORIENTED_EDGE ( 'NONE', *, *, #12535, .F. ) ;
#22693=CARTESIAN_POINT ( 'NONE',  ( 9.999999999999998224, 0.000000000000000000, -114.8750000040967905 ) ) ;
#22694=CARTESIAN_POINT ( 'NONE',  ( 9.999999999999996447, -5.773502691896262640, -106.0000000040967763 ) ) ;
#22696=CARTESIAN_POINT ( 'NONE',  ( -5.405949406249996869, 9.363379034771805109, -68.34375000204836681 ) ) ;
#22702=CARTESIAN_POINT ( 'NONE',  ( 5.000000000000000000, 8.660254037844385522, -44.12500000409677625 ) ) ;
#22703=CARTESIAN_POINT ( 'NONE',  ( 7.644554776091147741E-16, 12.48450537969573659, -37.15625000204836681 ) ) ;
#22704=CARTESIAN_POINT ( 'NONE',  ( -9.999999999999998224, 1.224646799147353059E-15, -117.1250000040967905 ) ) ;
#22708=( BOUNDED_CURVE ( )  B_SPLINE_CURVE ( 2, ( #8031, #27023, #33513, #7384, #37374, #24007, #27665 ),
 .UNSPECIFIED., .F., .F. ) 
 B_SPLINE_CURVE_WITH_KNOTS ( ( 3, 2, 2, 3 ),
 ( 0.4402985074626867279, 0.4415422885572141132, 0.4427860696517414429, 0.4440298507462688282 ),
 .UNSPECIFIED. ) 
 CURVE ( )  GEOMETRIC_REPRESENTATION_ITEM ( )  RATIONAL_B_SPLINE_CURVE ( ( 0.9999999999999820144, 0.8660254037844566932, 1.000000000000000000, 0.8660254037844387076, 1.000000000000000000, 0.8660254037844207220, 1.000000000000017986 ) ) 
 REPRESENTATION_ITEM ( '' )  );
#22709=CARTESIAN_POINT ( 'NONE',  ( 9.999999999999479527, 5.773502691896553074, -150.7500000040967336 ) ) ;
#22718=LINE ( 'NONE', #12970, #37080 ) ;
#22721=DIRECTION ( 'NONE',  ( -0.000000000000000000, -0.000000000000000000, -1.000000000000000000 ) ) ;
#22722=CARTESIAN_POINT ( 'NONE',  ( -5.405949406249996869, 9.363379034771805109, -123.8437500020483952 ) ) ;
#22723=CARTESIAN_POINT ( 'NONE',  ( 10.81189881249999551, -6.242252689847874514, -129.1562500020483810 ) ) ;
#22725=CARTESIAN_POINT ( 'NONE',  ( 10.81189881249999729, 6.242252689847867408, -145.2187500020484094 ) ) ;
#22726=CARTESIAN_POINT ( 'NONE',  ( 9.999999999999998224, 0.000000000000000000, -179.0000000000000000 ) ) ;
#22728=CARTESIAN_POINT ( 'NONE',  ( -9.999999999999998224, 5.773502691896259087, -161.8750000000000000 ) ) ;
#22732=CARTESIAN_POINT ( 'NONE',  ( -5.405949406249996869, 9.363379034771805109, -50.34375000204835260 ) ) ;
#22734=CARTESIAN_POINT ( 'NONE',  ( -10.81189881249999907, -6.242252689847864744, -159.4687500020484094 ) ) ;
#22739=CARTESIAN_POINT ( 'NONE',  ( -9.999999999999998224, 5.773502691896259087, -89.87499999999998579 ) ) ;
#22741=CARTESIAN_POINT ( 'NONE',  ( -10.81189881249999729, -6.242252689847864744, -119.1562500020484237 ) ) ;
#22742=CARTESIAN_POINT ( 'NONE',  ( 5.000000000000000000, 8.660254037844385522, -137.1250000040967620 ) ) ;
#22743=DIRECTION ( 'NONE',  ( -0.000000000000000000, -0.000000000000000000, -1.000000000000000000 ) ) ;
#22746=CARTESIAN_POINT ( 'NONE',  ( 0.000000000000000000, 0.000000000000000000, -99.99999999999998579 ) ) ;
#22747=CARTESIAN_POINT ( 'NONE',  ( 10.81189881249999551, -6.242252689847874514, -63.15625000204838813 ) ) ;
#22755=ORIENTED_EDGE ( 'NONE', *, *, #40781, .T. ) ;
#22768=CARTESIAN_POINT ( 'NONE',  ( -2.121150477449813534E-15, -11.54700538379251284, -32.37499999999996447 ) ) ;
#22772=CARTESIAN_POINT ( 'NONE',  ( 5.405949406249992428, -9.363379034771808662, -151.5937500020483810 ) ) ;
#22773=CARTESIAN_POINT ( 'NONE',  ( -10.81189881249999729, -6.242252689847864744, -168.4687500020483526 ) ) ;
#22774=LINE ( 'NONE', #3560, #8854 ) ;
#22776=CARTESIAN_POINT ( 'NONE',  ( 10.00000000000000000, 5.773502691896255534, -186.3750000000000284 ) ) ;
#22781=CARTESIAN_POINT ( 'NONE',  ( 7.644554776091147741E-16, 12.48450537969573659, -188.4687500020484094 ) ) ;
#22784=CARTESIAN_POINT ( 'NONE',  ( -5.405949406250003975, -9.363379034771801557, -62.03125000204837391 ) ) ;
#22786=CARTESIAN_POINT ( 'NONE',  ( 10.00000000000000000, 5.773502691896255534, -118.8749999999999858 ) ) ;
#22788=CARTESIAN_POINT ( 'NONE',  ( -10.81189881249999729, 6.242252689847871849, -144.9062500020484094 ) ) ;
#22789=CARTESIAN_POINT ( 'NONE',  ( 5.405949406249999534, 9.363379034771803333, -158.7812500020484094 ) ) ;
#22792=CARTESIAN_POINT ( 'NONE',  ( -5.405949406250003975, -9.363379034771801557, -90.34375000204838102 ) ) ;
#22795=CARTESIAN_POINT ( 'NONE',  ( -2.293366432827344421E-15, -12.48450537969573659, -190.7187500020484094 ) ) ;
#22797=CARTESIAN_POINT ( 'NONE',  ( 4.999999999999992006, -8.660254037844389075, -169.1250000040967905 ) ) ;
#22798=CARTESIAN_POINT ( 'NONE',  ( 4.999999999999992006, -8.660254037844389075, -123.7500000000000000 ) ) ;
#22799=CARTESIAN_POINT ( 'NONE',  ( -10.81189881249999729, 1.324075727343319199E-15, -83.28125000204838102 ) ) ;
#22801=CARTESIAN_POINT ( 'NONE',  ( 10.00000000000000000, 5.773502691896255534, -62.25000000409676915 ) ) ;
#22802=CARTESIAN_POINT ( 'NONE',  ( -10.81189881249999907, -6.242252689847864744, -21.46875000204836681 ) ) ;
#22806=CARTESIAN_POINT ( 'NONE',  ( 10.81189881249999729, 0.000000000000000000, -13.53125000204835615 ) ) ;
#22819=LINE ( 'NONE', #33598, #665 ) ;
#22829=CARTESIAN_POINT ( 'NONE',  ( 5.000000000000000000, 8.660254037844385522, -124.7500000000000000 ) ) ;
#22830=CARTESIAN_POINT ( 'NONE',  ( 10.00000000000012790, 5.773502691896179151, -172.8750000000000000 ) ) ;
#22831=CARTESIAN_POINT ( 'NONE',  ( -10.81189881249999729, 6.242252689847871849, -155.4062500020483810 ) ) ;
#22833=CARTESIAN_POINT ( 'NONE',  ( 9.999999999999742428, 5.773502691896404748, -121.8750000000000142 ) ) ;
#22838=CARTESIAN_POINT ( 'NONE',  ( -10.81189881249999729, 1.324075727343319199E-15, -81.59375000204838102 ) ) ;
#22839=CARTESIAN_POINT ( 'NONE',  ( -5.405949406250003975, -9.363379034771801557, -86.03125000204838102 ) ) ;
#22842=CARTESIAN_POINT ( 'NONE',  ( 10.81189881249999729, 6.242252689847867408, -169.4062500020484094 ) ) ;
#22843=CARTESIAN_POINT ( 'NONE',  ( 5.405949406249992428, -9.363379034771808662, -177.2812500020484094 ) ) ;
#22844=CARTESIAN_POINT ( 'NONE',  ( 9.999999999999996447, -5.773502691896262640, -154.0000000040968189 ) ) ;
#22846=CARTESIAN_POINT ( 'NONE',  ( -10.81189881249999907, -6.242252689847864744, -4.968750002048355263 ) ) ;
#22847=CARTESIAN_POINT ( 'NONE',  ( -2.121150477449813534E-15, -11.54700538379251284, -156.8750000000000000 ) ) ;
#22848=CARTESIAN_POINT ( 'NONE',  ( 10.81189881249999729, 0.000000000000000000, -113.8437500020483810 ) ) ;
#22850=CARTESIAN_POINT ( 'NONE',  ( 5.405949406249999534, 9.363379034771803333, -16.28125000204835970 ) ) ;
#22852=CYLINDRICAL_SURFACE ( 'NONE', #40978, 9.999999999999998224 ) ;
#22853=CARTESIAN_POINT ( 'NONE',  ( -10.81189881249999729, 6.242252689847871849, -104.4062500020483810 ) ) ;
#22856=CARTESIAN_POINT ( 'NONE',  ( -2.121150477449813534E-15, -11.54700538379251284, -82.25000000409676204 ) ) ;
#22858=CARTESIAN_POINT ( 'NONE',  ( -10.81189881249999729, 6.242252689847871849, -38.21875000204835970 ) ) ;
#22862=CARTESIAN_POINT ( 'NONE',  ( -5.000000000000003553, -8.660254037844383745, -8.875000004096744277 ) ) ;
#22863=AXIS2_PLACEMENT_3D ( 'NONE', #11005, #21150, #37348 ) ;
#22868=CARTESIAN_POINT ( 'NONE',  ( -9.999999999999998224, 1.224646799147353059E-15, -142.2500000000000000 ) ) ;
#22869=ORIENTED_EDGE ( 'NONE', *, *, #34654, .T. ) ;
#22873=VECTOR ( 'NONE', #8450, 1000.000000000000000 ) ;
#22879=DIRECTION ( 'NONE',  ( 0.000000000000000000, 0.000000000000000000, -1.000000000000000000 ) ) ;
#22881=CARTESIAN_POINT ( 'NONE',  ( 5.405949406249992428, -9.363379034771808662, -181.7812500020483810 ) ) ;
#22885=CARTESIAN_POINT ( 'NONE',  ( 10.81189881249999907, 6.242252689847868297, -101.7187500020483810 ) ) ;
#22887=CARTESIAN_POINT ( 'NONE',  ( 10.81189881249999729, 0.000000000000000000, -112.5312500020483952 ) ) ;
#22889=CARTESIAN_POINT ( 'NONE',  ( -5.405949406249996869, 9.363379034771805109, -117.8437500020483810 ) ) ;
#22890=EDGE_CURVE ( 'NONE', #30244, #3006, #25904, .T. ) ;
#22895=CARTESIAN_POINT ( 'NONE',  ( -9.999999999999998224, 1.224646799147353059E-15, -142.2500000000000000 ) ) ;
#22896=CARTESIAN_POINT ( 'NONE',  ( 7.070501591499377789E-16, 11.54700538379251284, -3.124999999999961364 ) ) ;
#22900=CARTESIAN_POINT ( 'NONE',  ( -5.000000000000003553, -8.660254037844383745, -179.8750000040967905 ) ) ;
#22902=CARTESIAN_POINT ( 'NONE',  ( 7.644554776091147741E-16, 12.48450537969573659, -30.96875000204835260 ) ) ;
#22903=CARTESIAN_POINT ( 'NONE',  ( 9.999999999999998224, 0.000000000000000000, -176.0000000000000000 ) ) ;
#22904=CARTESIAN_POINT ( 'NONE',  ( -10.81189881249999729, 1.324075727343319199E-15, -137.0937500020483810 ) ) ;
#22907=CARTESIAN_POINT ( 'NONE',  ( -9.999999999999998224, 1.224646799147353059E-15, -68.74999999999997158 ) ) ;
#22908=CARTESIAN_POINT ( 'NONE',  ( -10.81189881249999907, -6.242252689847864744, -134.1562500020483810 ) ) ;
#22912=CARTESIAN_POINT ( 'NONE',  ( -5.000000000000003553, -8.660254037844383745, -110.8750000040967763 ) ) ;
#22913=CARTESIAN_POINT ( 'NONE',  ( 5.000000000000000000, 8.660254037844385522, -101.1250000040967905 ) ) ;
#22914=CARTESIAN_POINT ( 'NONE',  ( 10.81189881249999729, 0.000000000000000000, -64.34375000204836681 ) ) ;
#22920=LINE ( 'NONE', #38887, #19397 ) ;
#22921=CARTESIAN_POINT ( 'NONE',  ( -9.999999999999998224, 5.773502691896259087, -33.25000000409675494 ) ) ;
#22938=ADVANCED_FACE ( 'NONE', ( #29682 ), #17337, .F. ) ;
#22939=CARTESIAN_POINT ( 'NONE',  ( -5.405949406250003975, -9.363379034771801557, -123.3437500020483952 ) ) ;
#22940=CARTESIAN_POINT ( 'NONE',  ( -10.81189881249999729, 6.242252689847871849, -132.9062500020483810 ) ) ;
#22942=CARTESIAN_POINT ( 'NONE',  ( 5.405949406249999534, 9.363379034771803333, -134.5937500020483810 ) ) ;
#22943=CARTESIAN_POINT ( 'NONE',  ( -9.999999999999227285, -5.773502691896698735, -126.0000000040967478 ) ) ;
#22945=CARTESIAN_POINT ( 'NONE',  ( -2.121150477449813534E-15, -11.54700538379251284, -167.3750000000000000 ) ) ;
#22949=CARTESIAN_POINT ( 'NONE',  ( 5.405949406249999534, 9.363379034771803333, -53.59375000204835970 ) ) ;
#22950=DIRECTION ( 'NONE',  ( -0.000000000000000000, -0.000000000000000000, -1.000000000000000000 ) ) ;
#22951=CARTESIAN_POINT ( 'NONE',  ( -10.81189881249999729, 6.242252689847871849, -158.2187500020483810 ) ) ;
#22956=CARTESIAN_POINT ( 'NONE',  ( -9.999999999999998224, 5.773502691896259087, -94.37499999999998579 ) ) ;
#22958=CARTESIAN_POINT ( 'NONE',  ( -2.293366432827344421E-15, -12.48450537969573659, -117.4062500020483952 ) ) ;
#22959=CARTESIAN_POINT ( 'NONE',  ( 7.070501591499377789E-16, 11.54700538379251284, -132.5000000040967620 ) ) ;
#22965=CARTESIAN_POINT ( 'NONE',  ( -5.405949406250003975, -9.363379034771801557, -63.53125000204837391 ) ) ;
#22970=CARTESIAN_POINT ( 'NONE',  ( -4.999999999999996447, 8.660254037844387298, -174.0000000000000284 ) ) ;
#22974=ORIENTED_EDGE ( 'NONE', *, *, #6438, .T. ) ;
#22977=VERTEX_POINT ( 'NONE', #6581 ) ;
#22978=VERTEX_POINT ( 'NONE', #3564 ) ;
#22982=CARTESIAN_POINT ( 'NONE',  ( 10.00000000000076916, -5.773502691895816774, -112.0000000040967620 ) ) ;
#22983=CARTESIAN_POINT ( 'NONE',  ( 5.000000000000000000, 8.660254037844385522, -31.74999999999997158 ) ) ;
#22986=CARTESIAN_POINT ( 'NONE',  ( 10.81189881249999551, -6.242252689847874514, -148.4687500020484094 ) ) ;
#22987=CARTESIAN_POINT ( 'NONE',  ( 5.405949406249999534, 9.363379034771803333, -164.5937500020484094 ) ) ;
#22989=CARTESIAN_POINT ( 'NONE',  ( 4.999999999999992006, -8.660254037844389075, -191.2500000000000000 ) ) ;
#22995=CARTESIAN_POINT ( 'NONE',  ( -5.405949406249996869, 9.363379034771805109, -189.8437500020483810 ) ) ;
#22998=CARTESIAN_POINT ( 'NONE',  ( -5.405949406250003975, -9.363379034771801557, -59.03125000204836681 ) ) ;
#23000=CARTESIAN_POINT ( 'NONE',  ( 4.999999999999992006, -8.660254037844389075, -117.7500000000000000 ) ) ;
#23003=CARTESIAN_POINT ( 'NONE',  ( -2.293366432827344421E-15, -12.48450537969573659, -142.9062500020484094 ) ) ;
#23004=CARTESIAN_POINT ( 'NONE',  ( 10.81189881249999729, 0.000000000000000000, -154.5312500020484094 ) ) ;
#23007=CARTESIAN_POINT ( 'NONE',  ( -10.81189881249999729, 6.242252689847871849, -92.21875000204838102 ) ) ;
#23010=CARTESIAN_POINT ( 'NONE',  ( -5.405949406250003975, -9.363379034771801557, -192.3437500020484094 ) ) ;
#23012=CARTESIAN_POINT ( 'NONE',  ( -9.999999999999998224, 1.224646799147353059E-15, -169.6250000040967905 ) ) ;
#23014=CARTESIAN_POINT ( 'NONE',  ( 7.644554776091147741E-16, 12.48450537969573659, -88.15625000204838102 ) ) ;
#23016=CARTESIAN_POINT ( 'NONE',  ( -4.999999999999996447, 8.660254037844387298, -63.37500000409676204 ) ) ;
#23017=CARTESIAN_POINT ( 'NONE',  ( 5.405949406249999534, 9.363379034771803333, -16.09375000204835260 ) ) ;
#23020=CARTESIAN_POINT ( 'NONE',  ( 7.644554776091147741E-16, 12.48450537969573659, -8.656250002048365033 ) ) ;
#23021=CARTESIAN_POINT ( 'NONE',  ( 0.000000000000000000, 0.000000000000000000, -99.99999999999998579 ) ) ;
#23029=CARTESIAN_POINT ( 'NONE',  ( -2.121150477449813534E-15, -11.54700538379251284, -160.2500000040967620 ) ) ;
#23030=CARTESIAN_POINT ( 'NONE',  ( 10.00000000000038369, -5.773502691896038819, -153.6250000000000284 ) ) ;
#23031=ORIENTED_EDGE ( 'NONE', *, *, #22141, .F. ) ;
#23032=VERTEX_POINT ( 'NONE', #27285 ) ;
#23039=CARTESIAN_POINT ( 'NONE',  ( -5.405949406250003975, -9.363379034771801557, -153.5312500020484094 ) ) ;
#23046=CARTESIAN_POINT ( 'NONE',  ( 10.81189881249999907, 6.242252689847868297, -80.71875000204838102 ) ) ;
#23047=CARTESIAN_POINT ( 'NONE',  ( -10.81189881249999907, -6.242252689847864744, -86.15625000204836681 ) ) ;
#23049=EDGE_CURVE ( 'NONE', #17267, #34592, #10753, .T. ) ;
#23051=CARTESIAN_POINT ( 'NONE',  ( 5.405949406249999534, 9.363379034771803333, -164.7812500020484094 ) ) ;
#23052=CARTESIAN_POINT ( 'NONE',  ( -10.81189881249999729, 1.324075727343319199E-15, -180.7812500020484094 ) ) ;
#23054=CARTESIAN_POINT ( 'NONE',  ( 4.999999999999992006, -8.660254037844389075, -155.6250000040967905 ) ) ;
#23056=CARTESIAN_POINT ( 'NONE',  ( -5.405949406249996869, 9.363379034771805109, -3.843750002048368586 ) ) ;
#23058=CARTESIAN_POINT ( 'NONE',  ( -10.81189881249999729, 6.242252689847871849, -114.7187500020483810 ) ) ;
#23060=CARTESIAN_POINT ( 'NONE',  ( 10.81189881249999907, 6.242252689847868297, -14.90625000204837036 ) ) ;
#23064=CARTESIAN_POINT ( 'NONE',  ( -10.81189881249999729, 6.242252689847871849, -111.9062500020483810 ) ) ;
#23067=CARTESIAN_POINT ( 'NONE',  ( -5.000000000000003553, -8.660254037844383745, -80.87500000409677625 ) ) ;
#23069=CARTESIAN_POINT ( 'NONE',  ( -5.405949406249996869, 9.363379034771805109, -45.84375000204838102 ) ) ;
#23073=CARTESIAN_POINT ( 'NONE',  ( 7.070501591499376803E-16, 11.54700538379251284, -139.6250000000000000 ) ) ;
#23074=CARTESIAN_POINT ( 'NONE',  ( -9.999999999999998224, 5.773502691896259087, -12.25000000409676204 ) ) ;
#23078=EDGE_LOOP ( 'NONE', ( #22869, #3148 ) ) ;
#23080=VERTEX_POINT ( 'NONE', #8078 ) ;
#23085=ORIENTED_EDGE ( 'NONE', *, *, #24107, .F. ) ;
#23087=CARTESIAN_POINT ( 'NONE',  ( 0.000000000000000000, 0.000000000000000000, -169.9999999999999716 ) ) ;
#23088=CARTESIAN_POINT ( 'NONE',  ( -2.293366432827344421E-15, -12.48450537969573659, -178.9062500020484379 ) ) ;
#23092=CARTESIAN_POINT ( 'NONE',  ( -5.405949406250003975, -9.363379034771801557, -99.34375000204838102 ) ) ;
#23094=CARTESIAN_POINT ( 'NONE',  ( -2.293366432827344421E-15, -12.48450537969573659, -108.4062500020483810 ) ) ;
#23096=CARTESIAN_POINT ( 'NONE',  ( 10.81189881249999729, 0.000000000000000000, -115.3437500020483810 ) ) ;
#23098=AXIS2_PLACEMENT_3D ( 'NONE', #25255, #38400, #38611 ) ;
#23101=CARTESIAN_POINT ( 'NONE',  ( 10.00000000000000000, 5.773502691896255534, -142.8750000000000000 ) ) ;
#23102=CARTESIAN_POINT ( 'NONE',  ( 7.070501591499377789E-16, 11.54700538379251284, -6.124999999999964473 ) ) ;
#23105=CARTESIAN_POINT ( 'NONE',  ( -10.00000000000000000, -5.773502691896251982, -178.5000000040967905 ) ) ;
#23107=CARTESIAN_POINT ( 'NONE',  ( -10.81189881249999729, 1.324075727343319199E-15, -33.59375000204836681 ) ) ;
#23108=CARTESIAN_POINT ( 'NONE',  ( 10.00000000000051159, -5.773502691895965988, -105.6249999999999858 ) ) ;
#23109=CARTESIAN_POINT ( 'NONE',  ( 10.81189881249999907, 6.242252689847868297, -137.7187500020484094 ) ) ;
#23111=CARTESIAN_POINT ( 'NONE',  ( -10.81189881249999729, 6.242252689847871849, -39.90625000204836681 ) ) ;
#23113=CARTESIAN_POINT ( 'NONE',  ( 10.00000000000000000, 5.773502691896255534, -69.37499999999998579 ) ) ;
#23114=CARTESIAN_POINT ( 'NONE',  ( -5.405949406249996869, 9.363379034771805109, -130.0312500020484094 ) ) ;
#23116=VERTEX_POINT ( 'NONE', #11937 ) ;
#23117=CARTESIAN_POINT ( 'NONE',  ( 10.00000000000000000, 5.773502691896255534, -108.7500000040967905 ) ) ;
#23119=CARTESIAN_POINT ( 'NONE',  ( 10.81189881249999551, -6.242252689847874514, -68.96875000204839523 ) ) ;
#23122=ADVANCED_FACE ( 'NONE', ( #17545 ), #34204, .F. ) ;
#23126=CARTESIAN_POINT ( 'NONE',  ( -5.000000000000003553, -8.660254037844383745, -37.37500000409676915 ) ) ;
#23130=AXIS2_PLACEMENT_3D ( 'NONE', #1423, #14556, #30778 ) ;
#23142=CARTESIAN_POINT ( 'NONE',  ( 10.81189881249999907, 6.242252689847868297, -122.7187500020483810 ) ) ;
#23143=AXIS2_PLACEMENT_3D ( 'NONE', #20733, #14456, #34779 ) ;
#23144=CARTESIAN_POINT ( 'NONE',  ( 10.81189881249999907, 6.242252689847868297, -128.9062500020483810 ) ) ;
#23146=CARTESIAN_POINT ( 'NONE',  ( 10.81189881249999729, 0.000000000000000000, -140.8437500020483810 ) ) ;
#23147=CARTESIAN_POINT ( 'NONE',  ( 0.000000000000000000, 0.000000000000000000, -99.99999999999998579 ) ) ;
#23150=CARTESIAN_POINT ( 'NONE',  ( 9.999999999999998224, 0.000000000000000000, -162.5000000000000000 ) ) ;
#23154=CARTESIAN_POINT ( 'NONE',  ( 10.81189881249999551, -6.242252689847874514, -52.46875000204837391 ) ) ;
#23155=CARTESIAN_POINT ( 'NONE',  ( -5.405949406250003975, -9.363379034771801557, -159.3437500020484094 ) ) ;
#23158=CARTESIAN_POINT ( 'NONE',  ( 0.000000000000000000, 0.000000000000000000, -99.99999999999998579 ) ) ;
#23160=CARTESIAN_POINT ( 'NONE',  ( 9.999999999999996447, -5.773502691896262640, -92.12499999999998579 ) ) ;
#23162=CARTESIAN_POINT ( 'NONE',  ( -10.81189881249999729, 6.242252689847871849, -113.4062500020483952 ) ) ;
#23163=CARTESIAN_POINT ( 'NONE',  ( 4.999999999999992006, -8.660254037844389075, -128.6250000040967620 ) ) ;
#23167=CARTESIAN_POINT ( 'NONE',  ( 9.999999999999998224, 0.000000000000000000, -149.3750000040967905 ) ) ;
#23168=CARTESIAN_POINT ( 'NONE',  ( -2.293366432827344421E-15, -12.48450537969573659, -54.40625000204838102 ) ) ;
#23173=CARTESIAN_POINT ( 'NONE',  ( -9.999999999999996447, 5.773502691896259975, -171.2500000040967905 ) ) ;
#23174=ORIENTED_EDGE ( 'NONE', *, *, #4812, .F. ) ;
#23180=VERTEX_POINT ( 'NONE', #14300 ) ;
#23183=ORIENTED_EDGE ( 'NONE', *, *, #30657, .F. ) ;
#23188=CARTESIAN_POINT ( 'NONE',  ( 9.999999999999994671, -5.773502691896262640, -134.1250000000000000 ) ) ;
#23189=CARTESIAN_POINT ( 'NONE',  ( -4.999999999999996447, 8.660254037844387298, -25.49999999999996803 ) ) ;
#23192=CARTESIAN_POINT ( 'NONE',  ( -10.81189881249999729, 6.242252689847871849, -149.2187500020484379 ) ) ;
#23194=CARTESIAN_POINT ( 'NONE',  ( -10.81189881249999729, 1.324075727343319199E-15, -161.0937500020484094 ) ) ;
#23195=CARTESIAN_POINT ( 'NONE',  ( -9.999999999999998224, 0.000000000000000000, -99.99999999999998579 ) ) ;
#23196=CARTESIAN_POINT ( 'NONE',  ( 9.999999999998969713, 5.773502691896851502, -102.7500000040967620 ) ) ;
#23197=CARTESIAN_POINT ( 'NONE',  ( 4.999999999999992006, -8.660254037844389075, -186.7500000000000000 ) ) ;
#23202=CARTESIAN_POINT ( 'NONE',  ( 0.000000000000000000, 0.000000000000000000, -99.99999999999998579 ) ) ;
#23203=CARTESIAN_POINT ( 'NONE',  ( -2.293366432827344421E-15, -12.48450537969573659, -187.7187500020484094 ) ) ;
#23207=CARTESIAN_POINT ( 'NONE',  ( -10.81189881249999729, 1.324075727343319199E-15, -50.28125000204835970 ) ) ;
#23209=CARTESIAN_POINT ( 'NONE',  ( -9.999999999999998224, 1.224646799147353059E-15, -116.7499999999999858 ) ) ;
#23210=VERTEX_POINT ( 'NONE', #18199 ) ;
#23211=CARTESIAN_POINT ( 'NONE',  ( -10.81189881249999729, 6.242252689847871849, -131.4062500020483810 ) ) ;
#23213=CARTESIAN_POINT ( 'NONE',  ( 10.81189881249999907, 6.242252689847868297, -145.4062500020484094 ) ) ;
#23216=CARTESIAN_POINT ( 'NONE',  ( 7.644554776091147741E-16, 12.48450537969573659, -81.96875000204839523 ) ) ;
#23219=CARTESIAN_POINT ( 'NONE',  ( 10.81189881249999551, -6.242252689847874514, -187.4687500020484094 ) ) ;
#23222=CARTESIAN_POINT ( 'NONE',  ( -10.00000000000051337, 5.773502691895962435, -139.7500000040967905 ) ) ;
#23223=CARTESIAN_POINT ( 'NONE',  ( 10.81189881249999729, 0.000000000000000000, -84.03125000204838102 ) ) ;
#23225=CARTESIAN_POINT ( 'NONE',  ( -5.000000000000003553, -8.660254037844383745, -61.37500000409676204 ) ) ;
#23226=CARTESIAN_POINT ( 'NONE',  ( -5.405949406250003975, -9.363379034771801557, -21.34375000204835615 ) ) ;
#23229=CARTESIAN_POINT ( 'NONE',  ( 10.81189881249999729, 0.000000000000000000, -10.53125000204835260 ) ) ;
#23231=CARTESIAN_POINT ( 'NONE',  ( -9.999999999999998224, 1.224646799147353059E-15, -175.6250000040968189 ) ) ;
#23239=CARTESIAN_POINT ( 'NONE',  ( 10.81189881249999729, 0.000000000000000000, -101.8437500020483810 ) ) ;
#23241=EDGE_LOOP ( 'NONE', ( #39180, #41850, #28026, #34454 ) ) ;
#23246=CARTESIAN_POINT ( 'NONE',  ( 10.00000000000051159, -5.773502691895965988, -115.0000000040967905 ) ) ;
#23249=( BOUNDED_CURVE ( )  B_SPLINE_CURVE ( 2, ( #4142, #33717, #1340, #8030, #27663, #34364, #21174 ),
 .UNSPECIFIED., .F., .F. ) 
 B_SPLINE_CURVE_WITH_KNOTS ( ( 3, 2, 2, 3 ),
 ( 0.1604477611940298698, 0.1616915422885572551, 0.1629353233830845848, 0.1641791044776119424 ),
 .UNSPECIFIED. ) 
 CURVE ( )  GEOMETRIC_REPRESENTATION_ITEM ( )  RATIONAL_B_SPLINE_CURVE ( ( 0.9999999999999970024, 0.8660254037844417052, 1.000000000000000000, 0.8660254037844387076, 1.000000000000000000, 0.8660254037844387076, 1.000000000000000000 ) ) 
 REPRESENTATION_ITEM ( '' )  );
#23250=CARTESIAN_POINT ( 'NONE',  ( -24.99999999999999645, 0.000000000000000000, -103.0000000000000000 ) ) ;
#23251=CARTESIAN_POINT ( 'NONE',  ( 9.999999999999998224, 1.224646799147353059E-15, -99.99999999999998579 ) ) ;
#23252=CARTESIAN_POINT ( 'NONE',  ( -10.81189881249999729, 1.324075727343319199E-15, -149.2812500020483810 ) ) ;
#23258=CARTESIAN_POINT ( 'NONE',  ( -5.405949406250003975, -9.363379034771801557, -67.84375000204836681 ) ) ;
#23259=CARTESIAN_POINT ( 'NONE',  ( -10.81189881249999907, -6.242252689847864744, -81.65625000204839523 ) ) ;
#23262=DIRECTION ( 'NONE',  ( -0.000000000000000000, -0.000000000000000000, -1.000000000000000000 ) ) ;
#23263=CARTESIAN_POINT ( 'NONE',  ( 5.405949406249992428, -9.363379034771808662, -166.7812500020484094 ) ) ;
#23264=CARTESIAN_POINT ( 'NONE',  ( 5.405949406249992428, -9.363379034771808662, -181.7812500020483810 ) ) ;
#23266=CARTESIAN_POINT ( 'NONE',  ( -5.405949406250003975, -9.363379034771801557, -3.343750002048367698 ) ) ;
#23268=CARTESIAN_POINT ( 'NONE',  ( -10.81189881249999907, -6.242252689847864744, -114.4687500020483810 ) ) ;
#23270=CARTESIAN_POINT ( 'NONE',  ( 7.644554776091147741E-16, 12.48450537969573659, -11.65625000204836859 ) ) ;
#23273=CARTESIAN_POINT ( 'NONE',  ( -10.81189881249999729, 1.324075727343319199E-15, -108.7812500020483810 ) ) ;
#23276=CARTESIAN_POINT ( 'NONE',  ( 7.070501591499377789E-16, 11.54700538379251284, -86.00000000409676204 ) ) ;
#23277=CARTESIAN_POINT ( 'NONE',  ( -2.121150477449813534E-15, -11.54700538379251284, -140.7500000040967905 ) ) ;
#23278=CARTESIAN_POINT ( 'NONE',  ( -10.81189881249999729, 6.242252689847871849, -45.71875000204836681 ) ) ;
#23279=ORIENTED_EDGE ( 'NONE', *, *, #19372, .T. ) ;
#23283=CARTESIAN_POINT ( 'NONE',  ( -2.121150477449813534E-15, -11.54700538379251284, -14.75000000409676382 ) ) ;
#23287=ORIENTED_EDGE ( 'NONE', *, *, #26750, .T. ) ;
#23288=CARTESIAN_POINT ( 'NONE',  ( 9.999999999999998224, 1.224646799147353059E-15, -99.99999999999998579 ) ) ;
#23289=EDGE_CURVE ( 'NONE', #36923, #12994, #7866, .T. ) ;
#23292=ORIENTED_EDGE ( 'NONE', *, *, #19687, .T. ) ;
#23293=EDGE_CURVE ( 'NONE', #13652, #4202, #14522, .T. ) ;
#23302=CARTESIAN_POINT ( 'NONE',  ( 7.644554776091147741E-16, 12.48450537969573659, -170.6562500020484094 ) ) ;
#23304=EDGE_CURVE ( 'NONE', #2497, #5570, #21259, .T. ) ;
#23306=CARTESIAN_POINT ( 'NONE',  ( 7.644554776091147741E-16, 12.48450537969573659, -98.46875000204839523 ) ) ;
#23308=CARTESIAN_POINT ( 'NONE',  ( -10.81189881249999729, 1.324075727343319199E-15, -107.2812500020483810 ) ) ;
#23310=CARTESIAN_POINT ( 'NONE',  ( 7.644554776091147741E-16, 12.48450537969573659, -113.4687500020483668 ) ) ;
#23314=CARTESIAN_POINT ( 'NONE',  ( -10.00000000000000000, -5.773502691896251982, -130.1250000000000000 ) ) ;
#23315=CARTESIAN_POINT ( 'NONE',  ( 5.000000000000000000, 8.660254037844385522, -3.249999999999975131 ) ) ;
#23319=CARTESIAN_POINT ( 'NONE',  ( 9.999999999999998224, 0.000000000000000000, -177.8750000040967905 ) ) ;
#23321=CARTESIAN_POINT ( 'NONE',  ( -10.81189881249999729, 6.242252689847871849, -33.71875000204835260 ) ) ;
#23322=FACE_OUTER_BOUND ( 'NONE', #15945, .T. ) ;
#23323=CARTESIAN_POINT ( 'NONE',  ( -5.405949406250003975, -9.363379034771801557, -136.8437500020484094 ) ) ;
#23325=CARTESIAN_POINT ( 'NONE',  ( 7.644554776091147741E-16, 12.48450537969573659, -32.65625000204835970 ) ) ;
#23329=CARTESIAN_POINT ( 'NONE',  ( -9.999999999999998224, 5.773502691896259087, -59.87499999999998579 ) ) ;
#23330=CARTESIAN_POINT ( 'NONE',  ( 5.405949406249999534, 9.363379034771803333, -131.7812500020483810 ) ) ;
#23334=CARTESIAN_POINT ( 'NONE',  ( -2.121150477449813534E-15, -11.54700538379251284, -109.2500000040967763 ) ) ;
#23336=CARTESIAN_POINT ( 'NONE',  ( 10.81189881249999907, 6.242252689847868297, -65.71875000204838102 ) ) ;
#23337=ORIENTED_EDGE ( 'NONE', *, *, #26094, .F. ) ;
#23339=B_SPLINE_CURVE_WITH_KNOTS ( 'NONE', 3,
 ( #41062, #35056, #21231, #18418, #11507, #34842, #11939, #24709, #22098, #5054, #41928, #5266, #38067, #25131, #37855, #28152, #35272, #8508, #21444, #31608, #31392, #28368, #34628, #4835, #32036, #1826, #5484, #15385, #25343 ),
 .UNSPECIFIED., .F., .F.,
 ( 4, 2, 2, 2, 2, 2, 2, 2, 2, 2, 2, 2, 1, 2, 4 ),
 ( 0.000000000000000000, 0.001276655870610509703, 0.002553311741221020708, 0.005106623482442043151, 0.006383279353052552854, 0.007659935223663064292, 0.008936591094273573996, 0.01021324696488408630, 0.01148990283549459861, 0.01276655870610510918, 0.01531987044732613552, 0.01659652631793664609, 0.01787318218854715840, 0.01914983805915767071, 0.02042649392976818301 ),
 .UNSPECIFIED. ) ;
#23344=CARTESIAN_POINT ( 'NONE',  ( -9.999999999999998224, 5.773502691896259087, -36.25000000409675494 ) ) ;
#23349=EDGE_CURVE ( 'NONE', #28187, #39897, #18456, .T. ) ;
#23350=ORIENTED_EDGE ( 'NONE', *, *, #13460, .T. ) ;
#23357=CARTESIAN_POINT ( 'NONE',  ( 9.999999999999998224, 0.000000000000000000, -111.8750000040967763 ) ) ;
#23361=CARTESIAN_POINT ( 'NONE',  ( 4.999999999999992006, -8.660254037844389075, -116.2499999999999858 ) ) ;
#23362=CARTESIAN_POINT ( 'NONE',  ( -5.405949406250003975, -9.363379034771801557, -126.3437500020483952 ) ) ;
#23363=CARTESIAN_POINT ( 'NONE',  ( 7.644554776091147741E-16, 12.48450537969573659, -134.6562500020483810 ) ) ;
#23365=CARTESIAN_POINT ( 'NONE',  ( 10.81189881249999551, -6.242252689847874514, -137.9687500020483810 ) ) ;
#23367=CARTESIAN_POINT ( 'NONE',  ( 10.00000000000025402, -5.773502691896113426, -129.6250000000000000 ) ) ;
#23369=CARTESIAN_POINT ( 'NONE',  ( 4.999999999999992006, -8.660254037844389075, -156.7500000000000000 ) ) ;
#23373=CARTESIAN_POINT ( 'NONE',  ( 5.405949406249992428, -9.363379034771808662, -55.59375000204835970 ) ) ;
#23374=CARTESIAN_POINT ( 'NONE',  ( 4.999999999999992006, -8.660254037844389075, -141.7500000000000000 ) ) ;
#23375=CARTESIAN_POINT ( 'NONE',  ( 5.405949406249992428, -9.363379034771808662, -162.0937500020484094 ) ) ;
#23380=CARTESIAN_POINT ( 'NONE',  ( 9.999999999999998224, 0.000000000000000000, -90.49999999999998579 ) ) ;
#23381=( BOUNDED_CURVE ( )  B_SPLINE_CURVE ( 2, ( #37236, #33808, #10689, #11113, #24523, #14122, #10905 ),
 .UNSPECIFIED., .F., .F. ) 
 B_SPLINE_CURVE_WITH_KNOTS ( ( 3, 2, 2, 3 ),
 ( 0.3768656716417911334, 0.3781094527363185187, 0.3793532338308459040, 0.3805970149253732338 ),
 .UNSPECIFIED. ) 
 CURVE ( )  GEOMETRIC_REPRESENTATION_ITEM ( )  RATIONAL_B_SPLINE_CURVE ( ( 0.9999999999999880096, 0.8660254037844506980, 1.000000000000000000, 0.8660254037844387076, 1.000000000000000000, 0.8660254037844267172, 1.000000000000011990 ) ) 
 REPRESENTATION_ITEM ( '' )  );
#23383=CARTESIAN_POINT ( 'NONE',  ( -10.81189881249999729, -6.242252689847864744, -108.6562500020483952 ) ) ;
#23384=CARTESIAN_POINT ( 'NONE',  ( -5.000000000000003553, -8.660254037844383745, -131.8750000040967905 ) ) ;
#23385=FACE_OUTER_BOUND ( 'NONE', #34242, .T. ) ;
#23389=CARTESIAN_POINT ( 'NONE',  ( 5.405949406249992428, -9.363379034771808662, -49.78125000204838813 ) ) ;
#23406=EDGE_CURVE ( 'NONE', #39897, #23938, #19844, .T. ) ;
#23411=CARTESIAN_POINT ( 'NONE',  ( 10.81189881249999907, 6.242252689847868297, -148.2187500020484094 ) ) ;
#23412=CARTESIAN_POINT ( 'NONE',  ( 10.81189881249999729, 0.000000000000000000, -161.8437500020484094 ) ) ;
#23415=CARTESIAN_POINT ( 'NONE',  ( 9.999999999999998224, 0.000000000000000000, -185.0000000000000000 ) ) ;
#23418=CARTESIAN_POINT ( 'NONE',  ( 9.999999999999998224, 0.000000000000000000, -138.5000000000000000 ) ) ;
#23420=CARTESIAN_POINT ( 'NONE',  ( 5.405949406249992428, -9.363379034771808662, -186.0937500020483810 ) ) ;
#23423=CARTESIAN_POINT ( 'NONE',  ( -5.405949406249996869, 9.363379034771805109, -55.03125000204836681 ) ) ;
#23425=CARTESIAN_POINT ( 'NONE',  ( -4.999999999999996447, 8.660254037844387298, -115.4999999999999858 ) ) ;
#23428=CARTESIAN_POINT ( 'NONE',  ( -2.293366432827344421E-15, -12.48450537969573659, -130.9062500020483810 ) ) ;
#23429=CARTESIAN_POINT ( 'NONE',  ( 10.81189881249999729, 0.000000000000000000, -150.0312500020483810 ) ) ;
#23432=CARTESIAN_POINT ( 'NONE',  ( -5.405949406250003975, -9.363379034771801557, -84.34375000204836681 ) ) ;
#23435=CARTESIAN_POINT ( 'NONE',  ( 10.81189881249999551, -6.242252689847874514, -176.9687500020483810 ) ) ;
#23439=CARTESIAN_POINT ( 'NONE',  ( -10.81189881249999729, 1.324075727343319199E-15, -78.78125000204838102 ) ) ;
#23441=CARTESIAN_POINT ( 'NONE',  ( -9.999999999999998224, 5.773502691896259087, -52.75000000409676915 ) ) ;
#23442=CARTESIAN_POINT ( 'NONE',  ( -10.81189881249999729, 1.324075727343319199E-15, -9.593750002048345493 ) ) ;
#23443=CARTESIAN_POINT ( 'NONE',  ( -31.99999999999997158, 4.102566777143632196E-15, -180.0000000000000000 ) ) ;
#23445=CARTESIAN_POINT ( 'NONE',  ( 5.405949406249999534, 9.363379034771803333, -13.28125000204835615 ) ) ;
#23449=CARTESIAN_POINT ( 'NONE',  ( -2.121150477449813534E-15, -11.54700538379251284, -134.7500000040967905 ) ) ;
#23454=ORIENTED_EDGE ( 'NONE', *, *, #16169, .F. ) ;
#23456=CARTESIAN_POINT ( 'NONE',  ( -5.405949406250003975, -9.363379034771801557, -102.3437500020483810 ) ) ;
#23457=VERTEX_POINT ( 'NONE', #13358 ) ;
#23458=ORIENTED_EDGE ( 'NONE', *, *, #4281, .T. ) ;
#23464=CARTESIAN_POINT ( 'NONE',  ( -4.999999999999996447, 8.660254037844387298, -46.49999999999998579 ) ) ;
#23467=( BOUNDED_CURVE ( )  B_SPLINE_CURVE ( 2, ( #23766, #17053, #34342, #14014, #36708, #17689, #1104 ),
 .UNSPECIFIED., .F., .F. ) 
 B_SPLINE_CURVE_WITH_KNOTS ( ( 3, 2, 2, 3 ),
 ( 0.3432835820895522860, 0.3445273631840797268, 0.3457711442786070566, 0.3470149253731344974 ),
 .UNSPECIFIED. ) 
 CURVE ( )  GEOMETRIC_REPRESENTATION_ITEM ( )  RATIONAL_B_SPLINE_CURVE ( ( 0.9999999999999940048, 0.8660254037844447028, 1.000000000000000000, 0.8660254037844387076, 1.000000000000000000, 0.8660254037844207220, 1.000000000000017986 ) ) 
 REPRESENTATION_ITEM ( '' )  );
#23470=CARTESIAN_POINT ( 'NONE',  ( 5.405949406249999534, 9.363379034771803333, -146.7812500020483810 ) ) ;
#23474=CARTESIAN_POINT ( 'NONE',  ( -4.999999999999996447, 8.660254037844387298, -160.8750000040967905 ) ) ;
#23477=CARTESIAN_POINT ( 'NONE',  ( 7.644554776091147741E-16, 12.48450537969573659, -68.46875000204838102 ) ) ;
#23478=CARTESIAN_POINT ( 'NONE',  ( 10.81189881249999551, -6.242252689847874514, -73.65625000204836681 ) ) ;
#23480=CARTESIAN_POINT ( 'NONE',  ( 10.81189881249999729, 0.000000000000000000, -157.5312500020484094 ) ) ;
#23481=CARTESIAN_POINT ( 'NONE',  ( -10.81189881249999907, -6.242252689847864744, -173.1562500020484094 ) ) ;
#23483=CARTESIAN_POINT ( 'NONE',  ( -9.999999999999998224, 1.224646799147353059E-15, -114.1250000040967763 ) ) ;
#23484=CARTESIAN_POINT ( 'NONE',  ( 5.405949406249999534, 9.363379034771803333, 0.4062499979516354109 ) ) ;
#23485=CARTESIAN_POINT ( 'NONE',  ( -10.81189881249999729, 1.324075727343319199E-15, -107.0937500020483810 ) ) ;
#23486=EDGE_CURVE ( 'NONE', #16772, #27040, #5239, .T. ) ;
#23488=CARTESIAN_POINT ( 'NONE',  ( -5.405949406250003975, -9.363379034771801557, -5.031250002048376579 ) ) ;
#23492=CARTESIAN_POINT ( 'NONE',  ( -10.81189881249999729, 1.324075727343319199E-15, -99.78125000204839523 ) ) ;
#23494=VERTEX_POINT ( 'NONE', #22308 ) ;
#23495=CARTESIAN_POINT ( 'NONE',  ( -5.000000000000003553, -8.660254037844383745, -82.37500000409676204 ) ) ;
#23496=CARTESIAN_POINT ( 'NONE',  ( -4.999999999999996447, 8.660254037844387298, -133.8750000040967905 ) ) ;
#23497=CARTESIAN_POINT ( 'NONE',  ( 5.405949406249992428, -9.363379034771808662, -34.59375000204836681 ) ) ;
#23500=CARTESIAN_POINT ( 'NONE',  ( 5.405949406249999534, 9.363379034771803333, -40.28125000204838102 ) ) ;
#23503=CARTESIAN_POINT ( 'NONE',  ( 5.000000000000000000, 8.660254037844385522, -12.62500000409674783 ) ) ;
#23517=DIRECTION ( 'NONE',  ( -0.000000000000000000, -0.000000000000000000, -1.000000000000000000 ) ) ;
#23518=DIRECTION ( 'NONE',  ( -1.000000000000000000, 0.000000000000000000, 0.000000000000000000 ) ) ;
#23519=( BOUNDED_CURVE ( )  B_SPLINE_CURVE ( 2, ( #36068, #27847, #4747, #33905, #31310, #7786, #17893 ),
 .UNSPECIFIED., .F., .F. ) 
 B_SPLINE_CURVE_WITH_KNOTS ( ( 3, 2, 2, 3 ),
 ( 0.4291044776119404269, 0.4303482587064677567, 0.4315920398009951975, 0.4328358208955225273 ),
 .UNSPECIFIED. ) 
 CURVE ( )  GEOMETRIC_REPRESENTATION_ITEM ( )  RATIONAL_B_SPLINE_CURVE ( ( 0.9999999999999880096, 0.8660254037844506980, 1.000000000000000000, 0.8660254037844387076, 1.000000000000000000, 0.8660254037844207220, 1.000000000000017986 ) ) 
 REPRESENTATION_ITEM ( '' )  );
#23520=CARTESIAN_POINT ( 'NONE',  ( -5.405949406250003975, -9.363379034771801557, -170.0312500020484094 ) ) ;
#23523=CARTESIAN_POINT ( 'NONE',  ( -10.81189881249999907, -6.242252689847864744, -91.96875000204838102 ) ) ;
#23524=CARTESIAN_POINT ( 'NONE',  ( 0.000000000000000000, 0.000000000000000000, -103.0000000000000000 ) ) ;
#23525=CARTESIAN_POINT ( 'NONE',  ( -2.293366432827344421E-15, -12.48450537969573659, -97.90625000204839523 ) ) ;
#23527=CARTESIAN_POINT ( 'NONE',  ( -10.81189881249999729, -6.242252689847864744, -111.4687500020483810 ) ) ;
#23529=CARTESIAN_POINT ( 'NONE',  ( 9.999999999999998224, 0.000000000000000000, -126.8750000040967905 ) ) ;
#23530=CARTESIAN_POINT ( 'NONE',  ( -10.81189881249999729, 6.242252689847871849, -179.4062500020484094 ) ) ;
#23531=CARTESIAN_POINT ( 'NONE',  ( -10.81189881249999729, 6.242252689847871849, -195.9062500020484094 ) ) ;
#23534=CARTESIAN_POINT ( 'NONE',  ( 4.999999999999992006, -8.660254037844389075, -182.6250000040967905 ) ) ;
#23536=CARTESIAN_POINT ( 'NONE',  ( -5.405949406249996869, 9.363379034771805109, -26.34375000204835970 ) ) ;
#23538=CARTESIAN_POINT ( 'NONE',  ( 10.81189881249999729, 0.000000000000000000, -131.8437500020484094 ) ) ;
#23541=CARTESIAN_POINT ( 'NONE',  ( -10.81189881249999907, -6.242252689847864744, -39.65625000204836681 ) ) ;
#23544=CARTESIAN_POINT ( 'NONE',  ( -10.00000000000000000, -5.773502691896251982, -61.12499999999998579 ) ) ;
#23545=CARTESIAN_POINT ( 'NONE',  ( 7.644554776091147741E-16, 12.48450537969573659, -134.6562500020483810 ) ) ;
#23549=CARTESIAN_POINT ( 'NONE',  ( 5.000000000000000000, 8.660254037844385522, -110.1250000040967763 ) ) ;
#23551=CARTESIAN_POINT ( 'NONE',  ( -10.81189881249999907, -6.242252689847864744, -64.96875000204838102 ) ) ;
#23557=CARTESIAN_POINT ( 'NONE',  ( 7.070501591499377789E-16, 11.54700538379251284, -36.50000000409675494 ) ) ;
#23568=DIRECTION ( 'NONE',  ( -1.000000000000000000, 0.000000000000000000, 0.000000000000000000 ) ) ;
#23575=CARTESIAN_POINT ( 'NONE',  ( 10.81189881249999907, 6.242252689847868297, -121.2187500020483952 ) ) ;
#23576=CARTESIAN_POINT ( 'NONE',  ( 10.81189881249999551, -6.242252689847874514, 0.03124999795164895566 ) ) ;
#23577=CARTESIAN_POINT ( 'NONE',  ( -2.293366432827344421E-15, -12.48450537969573659, -123.4062500020484094 ) ) ;
#23579=CARTESIAN_POINT ( 'NONE',  ( 7.644554776091147741E-16, 12.48450537969573659, -140.4687500020483810 ) ) ;
#23580=CARTESIAN_POINT ( 'NONE',  ( 10.37090729747365714, -3.076925949860441545, -179.9999999999999432 ) ) ;
#23582=CARTESIAN_POINT ( 'NONE',  ( -5.000000000000003553, -8.660254037844383745, -152.5000000000000000 ) ) ;
#23584=AXIS2_PLACEMENT_3D ( 'NONE', #37451, #21041, #4648 ) ;
#23588=CARTESIAN_POINT ( 'NONE',  ( -2.293366432827344421E-15, -12.48450537969573659, -51.21875000204836681 ) ) ;
#23590=CARTESIAN_POINT ( 'NONE',  ( -5.405949406249996869, 9.363379034771805109, -159.8437500020484094 ) ) ;
#23596=CARTESIAN_POINT ( 'NONE',  ( -5.000000000000003553, -8.660254037844383745, -81.99999999999998579 ) ) ;
#23598=EDGE_CURVE ( 'NONE', #7415, #6469, #31463, .T. ) ;
#23600=CARTESIAN_POINT ( 'NONE',  ( 10.81189881249999729, 6.242252689847867408, -110.9062500020483952 ) ) ;
#23601=CARTESIAN_POINT ( 'NONE',  ( -9.999999999999998224, 1.224646799147353059E-15, -135.1250000040967620 ) ) ;
#23606=CARTESIAN_POINT ( 'NONE',  ( 5.405949406249992428, -9.363379034771808662, -55.78125000204836681 ) ) ;
#23611=CARTESIAN_POINT ( 'NONE',  ( 5.000000000000000000, 8.660254037844385522, -171.6250000040968189 ) ) ;
#23612=ORIENTED_EDGE ( 'NONE', *, *, #4064, .F. ) ;
#23628=CARTESIAN_POINT ( 'NONE',  ( -2.293366432827344421E-15, -12.48450537969573659, -148.7187500020484094 ) ) ;
#23630=CARTESIAN_POINT ( 'NONE',  ( 7.644554776091147741E-16, 12.48450537969573659, -159.9687500020484094 ) ) ;
#23632=DIRECTION ( 'NONE',  ( -0.000000000000000000, -0.000000000000000000, -1.000000000000000000 ) ) ;
#23633=CARTESIAN_POINT ( 'NONE',  ( 7.070501591499377789E-16, 11.54700538379251284, -177.1250000000000000 ) ) ;
#23638=CARTESIAN_POINT ( 'NONE',  ( 7.644554776091147741E-16, 12.48450537969573659, -182.4687500020484094 ) ) ;
#23641=CARTESIAN_POINT ( 'NONE',  ( -10.81189881249999729, 1.324075727343319199E-15, -54.78125000204836681 ) ) ;
#23643=CARTESIAN_POINT ( 'NONE',  ( -10.00000000000000000, -5.773502691896251982, -109.1249999999999858 ) ) ;
#23645=CARTESIAN_POINT ( 'NONE',  ( -5.405949406249996869, 9.363379034771805109, -131.5312500020484094 ) ) ;
#23646=CARTESIAN_POINT ( 'NONE',  ( 5.405949406249992428, -9.363379034771808662, -151.7812500020484094 ) ) ;
#23648=CARTESIAN_POINT ( 'NONE',  ( 10.81189881249999907, 6.242252689847868297, -79.21875000204838102 ) ) ;
#23649=ORIENTED_EDGE ( 'NONE', *, *, #37567, .F. ) ;
#23651=CARTESIAN_POINT ( 'NONE',  ( -5.405949406250003975, -9.363379034771801557, -183.3437500020483810 ) ) ;
#23654=CARTESIAN_POINT ( 'NONE',  ( 10.81189881249999729, 0.000000000000000000, -79.53125000204838102 ) ) ;
#23656=CARTESIAN_POINT ( 'NONE',  ( -2.121150477449813534E-15, -11.54700538379251284, -50.75000000409676915 ) ) ;
#23657=CARTESIAN_POINT ( 'NONE',  ( 5.405949406249999534, 9.363379034771803333, -13.09375000204834905 ) ) ;
#23660=EDGE_CURVE ( 'NONE', #21425, #5246, #33096, .T. ) ;
#23661=CARTESIAN_POINT ( 'NONE',  ( -10.81189881249999729, 6.242252689847871849, -3.906250002048361480 ) ) ;
#23663=CARTESIAN_POINT ( 'NONE',  ( 10.00000000000051159, -5.773502691895965988, -148.0000000040967905 ) ) ;
#23664=CARTESIAN_POINT ( 'NONE',  ( -9.999999999999998224, 0.000000000000000000, -99.99999999999998579 ) ) ;
#23665=CARTESIAN_POINT ( 'NONE',  ( 0.000000000000000000, 0.000000000000000000, -99.99999999999998579 ) ) ;
#23670=CARTESIAN_POINT ( 'NONE',  ( -10.81189881249999729, 1.324075727343319199E-15, -101.0937500020483810 ) ) ;
#23671=ORIENTED_EDGE ( 'NONE', *, *, #32387, .T. ) ;
#23677=CARTESIAN_POINT ( 'NONE',  ( -4.999999999999996447, 8.660254037844387298, -47.99999999999998579 ) ) ;
#23682=CARTESIAN_POINT ( 'NONE',  ( -2.293366432827344421E-15, -12.48450537969573659, -147.4062500020483810 ) ) ;
#23686=CARTESIAN_POINT ( 'NONE',  ( -9.999999999999998224, 1.224646799147353059E-15, -140.7500000000000000 ) ) ;
#23689=CARTESIAN_POINT ( 'NONE',  ( -10.81189881249999729, 6.242252689847871849, -68.21875000204838102 ) ) ;
#23690=CARTESIAN_POINT ( 'NONE',  ( 5.405949406249992428, -9.363379034771808662, -75.28125000204838102 ) ) ;
#23692=CARTESIAN_POINT ( 'NONE',  ( 5.405949406249999534, 9.363379034771803333, -155.7812500020484094 ) ) ;
#23693=CARTESIAN_POINT ( 'NONE',  ( -10.81189881249999907, -6.242252689847864744, -170.1562500020483810 ) ) ;
#23694=CARTESIAN_POINT ( 'NONE',  ( -9.999999999999998224, 0.000000000000000000, -99.99999999999998579 ) ) ;
#23695=LINE ( 'NONE', #7286, #6837 ) ;
#23697=CARTESIAN_POINT ( 'NONE',  ( -10.81189881249999729, 1.324075727343319199E-15, -102.5937500020483810 ) ) ;
#23699=CARTESIAN_POINT ( 'NONE',  ( -5.405949406249996869, 9.363379034771805109, -2.531250002048373915 ) ) ;
#23702=CARTESIAN_POINT ( 'NONE',  ( 5.405949406249992428, -9.363379034771808662, -102.2812500020483952 ) ) ;
#23704=CARTESIAN_POINT ( 'NONE',  ( 4.999999999999992006, -8.660254037844389075, -74.62500000409677625 ) ) ;
#23705=CARTESIAN_POINT ( 'NONE',  ( 10.81189881249999729, 0.000000000000000000, -35.84375000204836681 ) ) ;
#23708=CARTESIAN_POINT ( 'NONE',  ( 10.81189881249999551, -6.242252689847874514, -30.15625000204835615 ) ) ;
#23711=CARTESIAN_POINT ( 'NONE',  ( 5.000000000000000000, 8.660254037844385522, -5.125000004096769146 ) ) ;
#23715=ORIENTED_EDGE ( 'NONE', *, *, #1154, .T. ) ;
#23717=EDGE_LOOP ( 'NONE', ( #15365, #36226, #3870, #4708 ) ) ;
#23719=ORIENTED_EDGE ( 'NONE', *, *, #10587, .F. ) ;
#23728=CARTESIAN_POINT ( 'NONE',  ( -10.81189881249999729, 1.324075727343319199E-15, -168.7812500020484094 ) ) ;
#23731=CARTESIAN_POINT ( 'NONE',  ( -5.405949406250003975, -9.363379034771801557, -93.34375000204838102 ) ) ;
#23732=CARTESIAN_POINT ( 'NONE',  ( -10.81189881249999729, 1.324075727343319199E-15, -198.5937500020484094 ) ) ;
#23733=CARTESIAN_POINT ( 'NONE',  ( -10.81189881249999729, 1.324075727343319199E-15, -101.2812500020483952 ) ) ;
#23735=CARTESIAN_POINT ( 'NONE',  ( -2.293366432827344421E-15, -12.48450537969573659, -109.7187500020483668 ) ) ;
#23737=CARTESIAN_POINT ( 'NONE',  ( 9.999999999999998224, 0.000000000000000000, -104.3750000040967763 ) ) ;
#23738=CARTESIAN_POINT ( 'NONE',  ( 5.000000000000000000, 8.660254037844385522, -132.6250000040967620 ) ) ;
#23739=CARTESIAN_POINT ( 'NONE',  ( 10.81189881249999729, 0.000000000000000000, -198.0312500020484094 ) ) ;
#23742=CARTESIAN_POINT ( 'NONE',  ( -9.999999999999998224, 1.224646799147353059E-15, -172.6250000040968189 ) ) ;
#23744=CARTESIAN_POINT ( 'NONE',  ( -5.405949406250003975, -9.363379034771801557, -18.34375000204835260 ) ) ;
#23746=CARTESIAN_POINT ( 'NONE',  ( -5.405949406249996869, 9.363379034771805109, -132.8437500020484094 ) ) ;
#23748=CARTESIAN_POINT ( 'NONE',  ( 5.405949406249992428, -9.363379034771808662, -31.78125000204837391 ) ) ;
#23750=CARTESIAN_POINT ( 'NONE',  ( 10.00000000000000000, 5.773502691896255534, -60.37499999999997868 ) ) ;
#23751=CARTESIAN_POINT ( 'NONE',  ( 5.405949406249992428, -9.363379034771808662, -123.2812500020483952 ) ) ;
#23753=VERTEX_POINT ( 'NONE', #4729 ) ;
#23754=CARTESIAN_POINT ( 'NONE',  ( 9.999999999999998224, 0.000000000000000000, -176.3750000040967905 ) ) ;
#23755=CARTESIAN_POINT ( 'NONE',  ( -2.121150477449813534E-15, -11.54700538379251284, -100.2500000040967905 ) ) ;
#23757=CARTESIAN_POINT ( 'NONE',  ( 10.81189881249999729, 0.000000000000000000, -61.34375000204836681 ) ) ;
#23762=CARTESIAN_POINT ( 'NONE',  ( 9.999999999999998224, 0.000000000000000000, -39.87500000409676915 ) ) ;
#23766=CARTESIAN_POINT ( 'NONE',  ( 9.999999999999998224, 0.000000000000000000, -129.8750000040967905 ) ) ;
#23768=( BOUNDED_CURVE ( )  B_SPLINE_CURVE ( 2, ( #1709, #27816, #14834, #28034, #18301, #31059, #27384 ),
 .UNSPECIFIED., .F., .F. ) 
 B_SPLINE_CURVE_WITH_KNOTS ( ( 3, 2, 2, 3 ),
 ( 0.4514925373134329734, 0.4527363184079603031, 0.4539800995024877439, 0.4552238805970150737 ),
 .UNSPECIFIED. ) 
 CURVE ( )  GEOMETRIC_REPRESENTATION_ITEM ( )  RATIONAL_B_SPLINE_CURVE ( ( 0.9999999999999880096, 0.8660254037844506980, 1.000000000000000000, 0.8660254037844387076, 1.000000000000000000, 0.8660254037844207220, 1.000000000000017986 ) ) 
 REPRESENTATION_ITEM ( '' )  );
#23771=DIRECTION ( 'NONE',  ( -0.000000000000000000, -0.000000000000000000, -1.000000000000000000 ) ) ;
#23775=CARTESIAN_POINT ( 'NONE',  ( -10.81189881249999729, 1.324075727343319199E-15, -197.2812500020484094 ) ) ;
#23781=CARTESIAN_POINT ( 'NONE',  ( 7.644554776091147741E-16, 12.48450537969573659, -114.9687500020483668 ) ) ;
#23782=CARTESIAN_POINT ( 'NONE',  ( -2.121150477449813534E-15, -11.54700538379251284, -194.7500000040967905 ) ) ;
#23783=CARTESIAN_POINT ( 'NONE',  ( 10.81189881249999551, -6.242252689847874514, -124.6562500020483952 ) ) ;
#23785=CARTESIAN_POINT ( 'NONE',  ( -5.405949406250003975, -9.363379034771801557, -138.3437500020484094 ) ) ;
#23788=CARTESIAN_POINT ( 'NONE',  ( -10.00000000000000000, -5.773502691896251982, -157.1250000000000284 ) ) ;
#23789=CARTESIAN_POINT ( 'NONE',  ( -2.121150477449813534E-15, -11.54700538379251284, -18.87499999999997158 ) ) ;
#23794=CARTESIAN_POINT ( 'NONE',  ( 5.405949406249992428, -9.363379034771808662, -48.09375000204838102 ) ) ;
#23795=CARTESIAN_POINT ( 'NONE',  ( -2.121150477449813534E-15, -11.54700538379251284, -141.8750000000000000 ) ) ;
#23796=CARTESIAN_POINT ( 'NONE',  ( 10.81189881249999907, 6.242252689847868297, -157.2187500020483810 ) ) ;
#23799=CARTESIAN_POINT ( 'NONE',  ( -3.491915452972480960, 9.450838780596122035, -179.9999999999999147 ) ) ;
#23801=CARTESIAN_POINT ( 'NONE',  ( -4.999999999999996447, 8.660254037844387298, -83.99999999999997158 ) ) ;
#23804=CARTESIAN_POINT ( 'NONE',  ( 10.81189881249999729, 0.000000000000000000, -112.5312500020483952 ) ) ;
#23805=CARTESIAN_POINT ( 'NONE',  ( -10.00000000000000000, -5.773502691896251982, -129.0000000040967905 ) ) ;
#23809=CARTESIAN_POINT ( 'NONE',  ( 10.81189881249999551, -6.242252689847874514, -49.65625000204837391 ) ) ;
#23811=CARTESIAN_POINT ( 'NONE',  ( 10.00000000000025402, -5.773502691896113426, -135.6250000000000000 ) ) ;
#23820=EDGE_CURVE ( 'NONE', #36083, #2497, #41898, .T. ) ;
#23824=EDGE_CURVE ( 'NONE', #33328, #17480, #15164, .T. ) ;
#23831=CARTESIAN_POINT ( 'NONE',  ( -4.999999999999996447, 8.660254037844387298, -153.3750000040967905 ) ) ;
#23832=CARTESIAN_POINT ( 'NONE',  ( -9.999999999999806377, 5.773502691895924244, -179.8750000000000000 ) ) ;
#23836=( BOUNDED_CURVE ( )  B_SPLINE_CURVE ( 2, ( #18219, #1844, #8524, #28169, #41303, #37838, #27913 ),
 .UNSPECIFIED., .F., .F. ) 
 B_SPLINE_CURVE_WITH_KNOTS ( ( 3, 2, 2, 3 ),
 ( 0.1679104477611940427, 0.1691542288557214002, 0.1703980099502487855, 0.1716417910447761430 ),
 .UNSPECIFIED. ) 
 CURVE ( )  GEOMETRIC_REPRESENTATION_ITEM ( )  RATIONAL_B_SPLINE_CURVE ( ( 1.000000000000000000, 0.8660254037844387076, 1.000000000000000000, 0.8660254037844387076, 1.000000000000000000, 0.8660254037844357100, 1.000000000000003109 ) ) 
 REPRESENTATION_ITEM ( '' )  );
#23838=CARTESIAN_POINT ( 'NONE',  ( 7.644554776091147741E-16, 12.48450537969573659, -138.9687500020484094 ) ) ;
#23839=CARTESIAN_POINT ( 'NONE',  ( 10.81189881249999729, 6.242252689847867408, -161.7187500020483810 ) ) ;
#23842=CARTESIAN_POINT ( 'NONE',  ( 9.999999999999996447, -5.773502691896262640, -176.1250000000000000 ) ) ;
#23844=DIRECTION ( 'NONE',  ( -1.000000000000000000, 0.000000000000000000, 0.000000000000000000 ) ) ;
#23847=CARTESIAN_POINT ( 'NONE',  ( 7.644554776091147741E-16, 12.48450537969573659, -174.9687500020484094 ) ) ;
#23851=CARTESIAN_POINT ( 'NONE',  ( 5.405949406249992428, -9.363379034771808662, -49.78125000204838813 ) ) ;
#23853=CARTESIAN_POINT ( 'NONE',  ( 7.070501591499377789E-16, 11.54700538379251284, -111.1249999999999716 ) ) ;
#23855=CARTESIAN_POINT ( 'NONE',  ( -10.81189881249999729, 1.324075727343319199E-15, -137.2812500020483810 ) ) ;
#23856=CARTESIAN_POINT ( 'NONE',  ( -4.999999999999996447, 8.660254037844387298, -156.3750000040967905 ) ) ;
#23857=CARTESIAN_POINT ( 'NONE',  ( 10.81189881249999907, 6.242252689847868297, -146.9062500020484094 ) ) ;
#23860=CARTESIAN_POINT ( 'NONE',  ( 10.81189881249999551, -6.242252689847874514, -85.46875000204836681 ) ) ;
#23863=CARTESIAN_POINT ( 'NONE',  ( -10.81189881249999907, -6.242252689847864744, -181.9687500020484094 ) ) ;
#23867=CARTESIAN_POINT ( 'NONE',  ( 5.405949406249992428, -9.363379034771808662, -79.78125000204838102 ) ) ;
#23869=CARTESIAN_POINT ( 'NONE',  ( -2.121150477449813534E-15, -11.54700538379251284, -53.75000000409677625 ) ) ;
#23870=CARTESIAN_POINT ( 'NONE',  ( 7.644554776091147741E-16, 12.48450537969573659, -12.96875000204836503 ) ) ;
#23873=CARTESIAN_POINT ( 'NONE',  ( 7.644554776091147741E-16, 12.48450537969573659, -5.656250002048362369 ) ) ;
#23875=CARTESIAN_POINT ( 'NONE',  ( 9.999999999999998224, 0.000000000000000000, -135.8750000040967905 ) ) ;
#23877=CARTESIAN_POINT ( 'NONE',  ( -2.121150477449813534E-15, -11.54700538379251284, -103.2500000040967763 ) ) ;
#23884=ORIENTED_EDGE ( 'NONE', *, *, #42274, .T. ) ;
#23887=( BOUNDED_CURVE ( )  B_SPLINE_CURVE ( 2, ( #549, #4622, #26861, #969, #30328, #14086, #11294 ),
 .UNSPECIFIED., .F., .F. ) 
 B_SPLINE_CURVE_WITH_KNOTS ( ( 3, 2, 2, 3 ),
 ( 0.1492537313432835966, 0.1504975124378109819, 0.1517412935323383116, 0.1529850746268656692 ),
 .UNSPECIFIED. ) 
 CURVE ( )  GEOMETRIC_REPRESENTATION_ITEM ( )  RATIONAL_B_SPLINE_CURVE ( ( 0.9999999999999970024, 0.8660254037844417052, 1.000000000000000000, 0.8660254037844387076, 1.000000000000000000, 0.8660254037844387076, 1.000000000000000000 ) ) 
 REPRESENTATION_ITEM ( '' )  );
#23892=CARTESIAN_POINT ( 'NONE',  ( 9.999999999999996447, -5.773502691896262640, -44.12499999999997158 ) ) ;
#23895=CARTESIAN_POINT ( 'NONE',  ( -10.81189881249999907, -6.242252689847864744, -166.9687500020484094 ) ) ;
#23899=CYLINDRICAL_SURFACE ( 'NONE', #38470, 9.999999999999998224 ) ;
#23900=CARTESIAN_POINT ( 'NONE',  ( -9.999999999999998224, 1.224646799147353059E-15, -143.7500000000000000 ) ) ;
#23907=CARTESIAN_POINT ( 'NONE',  ( 7.644554776091147741E-16, 12.48450537969573659, -69.96875000204838102 ) ) ;
#23908=CARTESIAN_POINT ( 'NONE',  ( -5.405949406249996869, 9.363379034771805109, -80.53125000204838102 ) ) ;
#23910=CARTESIAN_POINT ( 'NONE',  ( 5.405949406249999534, 9.363379034771803333, -158.7812500020484094 ) ) ;
#23911=CARTESIAN_POINT ( 'NONE',  ( -5.405949406249996869, 9.363379034771805109, -169.0312500020484094 ) ) ;
#23912=CARTESIAN_POINT ( 'NONE',  ( -2.293366432827344421E-15, -12.48450537969573659, -0.2187500020483512386 ) ) ;
#23914=CARTESIAN_POINT ( 'NONE',  ( -10.81189881249999907, -6.242252689847864744, -102.4687500020483810 ) ) ;
#23917=CARTESIAN_POINT ( 'NONE',  ( -10.81189881249999729, 1.324075727343319199E-15, -6.781250002048377468 ) ) ;
#23920=CARTESIAN_POINT ( 'NONE',  ( 5.405949406249999534, 9.363379034771803333, -103.2812500020483952 ) ) ;
#23922=CARTESIAN_POINT ( 'NONE',  ( -4.999999999999996447, 8.660254037844387298, -75.37500000409677625 ) ) ;
#23923=CARTESIAN_POINT ( 'NONE',  ( 9.999999999999998224, 0.000000000000000000, -168.8750000040967905 ) ) ;
#23924=CARTESIAN_POINT ( 'NONE',  ( 10.81189881249999729, 0.000000000000000000, -32.84375000204836681 ) ) ;
#23925=ORIENTED_EDGE ( 'NONE', *, *, #19041, .F. ) ;
#23927=CARTESIAN_POINT ( 'NONE',  ( 10.81189881249999551, -6.242252689847874514, -27.15625000204838102 ) ) ;
#23930=CARTESIAN_POINT ( 'NONE',  ( -9.999999999999998224, 5.773502691896259087, -7.750000004096757600 ) ) ;
#23933=CARTESIAN_POINT ( 'NONE',  ( -5.000000000000003553, -8.660254037844383745, -155.8750000040967905 ) ) ;
#23936=CARTESIAN_POINT ( 'NONE',  ( 9.999999999999998224, 0.000000000000000000, -115.9999999999999858 ) ) ;
#23938=VERTEX_POINT ( 'NONE', #22693 ) ;
#23943=CARTESIAN_POINT ( 'NONE',  ( 7.070501591499376803E-16, 11.54700538379251284, -114.1249999999999858 ) ) ;
#23945=CARTESIAN_POINT ( 'NONE',  ( -5.405949406250003975, -9.363379034771801557, -174.5312500020484094 ) ) ;
#23949=CARTESIAN_POINT ( 'NONE',  ( 10.81189881249999551, -6.242252689847874514, -91.46875000204838102 ) ) ;
#23951=CARTESIAN_POINT ( 'NONE',  ( -5.405949406249996869, 9.363379034771805109, -100.0312500020483952 ) ) ;
#23953=CARTESIAN_POINT ( 'NONE',  ( -10.81189881249999729, 6.242252689847871849, -108.7187500020483810 ) ) ;
#23957=CARTESIAN_POINT ( 'NONE',  ( 10.81189881249999551, -6.242252689847874514, -196.6562500020484379 ) ) ;
#23960=CARTESIAN_POINT ( 'NONE',  ( 7.070501591499377789E-16, 11.54700538379251284, -168.5000000040967905 ) ) ;
#23962=CARTESIAN_POINT ( 'NONE',  ( -10.81189881249999907, -6.242252689847864744, -18.46875000204836681 ) ) ;
#23963=DIRECTION ( 'NONE',  ( -1.000000000000000000, 0.000000000000000000, 0.000000000000000000 ) ) ;
#23964=CARTESIAN_POINT ( 'NONE',  ( 10.81189881249999551, -6.242252689847874514, -128.9687500020483810 ) ) ;
#23966=CARTESIAN_POINT ( 'NONE',  ( 7.644554776091147741E-16, 12.48450537969573659, -29.65625000204835615 ) ) ;
#23967=CARTESIAN_POINT ( 'NONE',  ( -9.999999999999998224, 1.224646799147353059E-15, -101.7500000000000000 ) ) ;
#23968=CARTESIAN_POINT ( 'NONE',  ( 5.000000000000000000, 8.660254037844385522, -63.24999999999997158 ) ) ;
#23969=CARTESIAN_POINT ( 'NONE',  ( 5.405949406249992428, -9.363379034771808662, -126.2812500020483668 ) ) ;
#23971=EDGE_CURVE ( 'NONE', #39100, #41044, #27281, .T. ) ;
#23974=CARTESIAN_POINT ( 'NONE',  ( 4.999999999999992006, -8.660254037844389075, -101.6250000040967905 ) ) ;
#23976=CARTESIAN_POINT ( 'NONE',  ( -2.293366432827344421E-15, -12.48450537969573659, -57.21875000204836681 ) ) ;
#23979=CIRCLE ( 'NONE', #1235, 35.00000000000000711 ) ;
#23983=CARTESIAN_POINT ( 'NONE',  ( -10.00000000000000000, -5.773502691896251982, -25.50000000409677270 ) ) ;
#23988=ORIENTED_EDGE ( 'NONE', *, *, #31063, .F. ) ;
#23993=CARTESIAN_POINT ( 'NONE',  ( -10.81189881249999729, 6.242252689847871849, -194.4062500020484094 ) ) ;
#24001=CARTESIAN_POINT ( 'NONE',  ( -10.81189881249999729, 6.242252689847871849, -119.2187500020483810 ) ) ;
#24002=CARTESIAN_POINT ( 'NONE',  ( -9.999999999999998224, 5.773502691896259087, -192.2500000040968189 ) ) ;
#24003=CARTESIAN_POINT ( 'NONE',  ( 7.644554776091147741E-16, 12.48450537969573659, -121.1562500020483952 ) ) ;
#24005=CARTESIAN_POINT ( 'NONE',  ( 10.81189881249999551, -6.242252689847874514, -133.4687500020483810 ) ) ;
#24006=CARTESIAN_POINT ( 'NONE',  ( -24.99999999999999645, 0.000000000000000000, -169.9999999999999716 ) ) ;
#24007=CARTESIAN_POINT ( 'NONE',  ( -10.00000000000076916, 5.773502691895813221, -109.7500000040967620 ) ) ;
#24008=CARTESIAN_POINT ( 'NONE',  ( 4.999999999999992006, -8.660254037844389075, -158.2500000000000000 ) ) ;
#24009=CARTESIAN_POINT ( 'NONE',  ( -5.000000000000003553, -8.660254037844383745, -23.49999999999996447 ) ) ;
#24012=DIRECTION ( 'NONE',  ( -0.000000000000000000, -0.000000000000000000, -1.000000000000000000 ) ) ;
#24014=CARTESIAN_POINT ( 'NONE',  ( -10.81189881249999907, -6.242252689847864744, -45.46875000204835970 ) ) ;
#24016=CARTESIAN_POINT ( 'NONE',  ( 7.644554776091147741E-16, 12.48450537969573659, -152.4687500020483810 ) ) ;
#24020=CARTESIAN_POINT ( 'NONE',  ( -9.999999999999998224, 1.224646799147353059E-15, -80.74999999999998579 ) ) ;
#24024=CARTESIAN_POINT ( 'NONE',  ( -5.405949406249996869, 9.363379034771805109, -110.5312500020483810 ) ) ;
#24025=CARTESIAN_POINT ( 'NONE',  ( -2.121150477449813534E-15, -11.54700538379251284, -127.2500000040967905 ) ) ;
#24026=CARTESIAN_POINT ( 'NONE',  ( -9.999999999999998224, 1.224646799147353059E-15, -154.2500000000000000 ) ) ;
#24029=DIRECTION ( 'NONE',  ( -0.000000000000000000, -0.000000000000000000, -1.000000000000000000 ) ) ;
#24030=CARTESIAN_POINT ( 'NONE',  ( 7.644554776091147741E-16, 12.48450537969573659, -55.15625000204838102 ) ) ;
#24031=( BOUNDED_CURVE ( )  B_SPLINE_CURVE ( 2, ( #4766, #27648, #14235, #37572, #10800, #34563, #8015 ),
 .UNSPECIFIED., .F., .F. ) 
 B_SPLINE_CURVE_WITH_KNOTS ( ( 3, 2, 2, 3 ),
 ( 0.1194029850746269744, 0.1206467661691543042, 0.1218905472636816062, 0.1231343283582089221 ),
 .UNSPECIFIED. ) 
 CURVE ( )  GEOMETRIC_REPRESENTATION_ITEM ( )  RATIONAL_B_SPLINE_CURVE ( ( 0.9999999999999880096, 0.8660254037844506980, 1.000000000000000000, 0.8660254037844387076, 1.000000000000000000, 0.8660254037844417052, 0.9999999999999970024 ) ) 
 REPRESENTATION_ITEM ( '' )  );
#24035=CARTESIAN_POINT ( 'NONE',  ( 9.999999999999998224, 0.000000000000000000, -165.8750000040967905 ) ) ;
#24036=VECTOR ( 'NONE', #19525, 1000.000000000000000 ) ;
#24038=CARTESIAN_POINT ( 'NONE',  ( -4.999999999999996447, 8.660254037844387298, -177.0000000000000000 ) ) ;
#24039=ORIENTED_EDGE ( 'NONE', *, *, #1047, .F. ) ;
#24042=VERTEX_POINT ( 'NONE', #6296 ) ;
#24045=CARTESIAN_POINT ( 'NONE',  ( 7.070501591499376803E-16, 11.54700538379251284, -153.5000000040967905 ) ) ;
#24050=CARTESIAN_POINT ( 'NONE',  ( -5.405949406249996869, 9.363379034771805109, -138.8437500020484094 ) ) ;
#24051=CARTESIAN_POINT ( 'NONE',  ( 5.405949406249999534, 9.363379034771803333, -155.5937500020483810 ) ) ;
#24054=CARTESIAN_POINT ( 'NONE',  ( 7.070501591499377789E-16, 11.54700538379251284, -175.6250000000000000 ) ) ;
#24058=CARTESIAN_POINT ( 'NONE',  ( 4.999999999999992006, -8.660254037844389075, -124.1250000040967905 ) ) ;
#24059=CARTESIAN_POINT ( 'NONE',  ( 5.405949406249999534, 9.363379034771803333, -179.5937500020484094 ) ) ;
#24063=CARTESIAN_POINT ( 'NONE',  ( 5.000000000000000000, 8.660254037844385522, -115.7499999999999858 ) ) ;
#24064=CARTESIAN_POINT ( 'NONE',  ( -10.81189881249999907, -6.242252689847864744, -54.65625000204838102 ) ) ;
#24066=CARTESIAN_POINT ( 'NONE',  ( 4.999999999999992006, -8.660254037844389075, -107.2499999999999858 ) ) ;
#24067=ORIENTED_EDGE ( 'NONE', *, *, #269, .T. ) ;
#24068=CARTESIAN_POINT ( 'NONE',  ( 7.644554776091147741E-16, 12.48450537969573659, -136.1562500020484094 ) ) ;
#24069=CARTESIAN_POINT ( 'NONE',  ( 9.999999999999998224, 0.000000000000000000, -147.8750000040967905 ) ) ;
#24070=CARTESIAN_POINT ( 'NONE',  ( 10.81189881249999551, -6.242252689847874514, -145.6562500020484094 ) ) ;
#24071=VECTOR ( 'NONE', #33418, 1000.000000000000000 ) ;
#24075=CARTESIAN_POINT ( 'NONE',  ( 10.81189881249999551, -6.242252689847874514, -179.9687500020484094 ) ) ;
#24079=EDGE_CURVE ( 'NONE', #31861, #15525, #21487, .T. ) ;
#24080=CARTESIAN_POINT ( 'NONE',  ( -10.81189881249999729, 1.324075727343319199E-15, -74.28125000204838102 ) ) ;
#24082=CARTESIAN_POINT ( 'NONE',  ( -5.000000000000003553, -8.660254037844383745, -53.87500000409675494 ) ) ;
#24084=CARTESIAN_POINT ( 'NONE',  ( 10.81189881249999907, 6.242252689847868297, -10.21875000204835970 ) ) ;
#24087=CARTESIAN_POINT ( 'NONE',  ( -5.405949406249996869, 9.363379034771805109, -2.531250002048373915 ) ) ;
#24089=CARTESIAN_POINT ( 'NONE',  ( 5.000000000000000000, 8.660254037844385522, -138.6250000040967905 ) ) ;
#24090=LINE ( 'NONE', #31212, #21076 ) ;
#24099=VERTEX_POINT ( 'NONE', #23754 ) ;
#24106=CARTESIAN_POINT ( 'NONE',  ( -2.121150477449813534E-15, -11.54700538379251284, -42.87499999999997158 ) ) ;
#24107=EDGE_CURVE ( 'NONE', #39101, #41597, #15420, .T. ) ;
#24109=CARTESIAN_POINT ( 'NONE',  ( 7.644554776091147741E-16, 12.48450537969573659, -164.4687500020483810 ) ) ;
#24113=CARTESIAN_POINT ( 'NONE',  ( -9.999999999999998224, 1.224646799147353059E-15, -146.7500000000000000 ) ) ;
#24115=CARTESIAN_POINT ( 'NONE',  ( 10.00000000000000000, 5.773502691896255534, -199.8750000000000284 ) ) ;
#24120=CARTESIAN_POINT ( 'NONE',  ( 10.81189881249999729, 0.000000000000000000, -70.34375000204836681 ) ) ;
#24121=CARTESIAN_POINT ( 'NONE',  ( -5.405949406250003975, -9.363379034771801557, -80.03125000204838102 ) ) ;
#24123=CARTESIAN_POINT ( 'NONE',  ( 9.999999999999996447, -5.773502691896262640, -131.1250000000000000 ) ) ;
#24124=CARTESIAN_POINT ( 'NONE',  ( 5.405949406249992428, -9.363379034771808662, -156.2812500020484094 ) ) ;
#24125=CARTESIAN_POINT ( 'NONE',  ( -10.81189881249999729, 6.242252689847871849, -171.9062500020484094 ) ) ;
#24127=CARTESIAN_POINT ( 'NONE',  ( -10.81189881249999729, 6.242252689847871849, -105.7187500020483668 ) ) ;
#24130=CARTESIAN_POINT ( 'NONE',  ( -10.81189881249999907, -6.242252689847864744, -2.156250002048359704 ) ) ;
#24134=CARTESIAN_POINT ( 'NONE',  ( 10.81189881249999907, 6.242252689847868297, -97.40625000204839523 ) ) ;
#24137=CARTESIAN_POINT ( 'NONE',  ( -4.999999999999996447, 8.660254037844387298, -72.37500000409677625 ) ) ;
#24139=CARTESIAN_POINT ( 'NONE',  ( 10.81189881249999729, 0.000000000000000000, -37.34375000204836681 ) ) ;
#24143=EDGE_CURVE ( 'NONE', #25900, #5096, #19832, .T. ) ;
#24144=CARTESIAN_POINT ( 'NONE',  ( -10.81189881249999907, -6.242252689847864744, -32.15625000204835970 ) ) ;
#24147=CARTESIAN_POINT ( 'NONE',  ( 7.070501591499377789E-16, 11.54700538379251284, -8.000000004096758488 ) ) ;
#24162=CARTESIAN_POINT ( 'NONE',  ( -5.405949406249996869, 9.363379034771805109, -169.0312500020484094 ) ) ;
#24165=CARTESIAN_POINT ( 'NONE',  ( -10.81189881249999907, -6.242252689847864744, -96.46875000204838102 ) ) ;
#24168=CARTESIAN_POINT ( 'NONE',  ( 10.81189881249999551, -6.242252689847874514, -97.65625000204839523 ) ) ;
#24170=CARTESIAN_POINT ( 'NONE',  ( 7.644554776091147741E-16, 12.48450537969573659, -108.9687500020483668 ) ) ;
#24172=CARTESIAN_POINT ( 'NONE',  ( -10.00000000000076916, 5.773502691895813221, -107.8749999999999574 ) ) ;
#24173=CARTESIAN_POINT ( 'NONE',  ( 5.405949406249999534, 9.363379034771803333, -179.7812500020484094 ) ) ;
#24174=CARTESIAN_POINT ( 'NONE',  ( 9.999999999999996447, -5.773502691896262640, -0.6249999999999588107 ) ) ;
#24177=CARTESIAN_POINT ( 'NONE',  ( -9.999999999999998224, 5.773502691896259087, -175.7500000040967905 ) ) ;
#24179=CARTESIAN_POINT ( 'NONE',  ( -2.293366432827344421E-15, -12.48450537969573659, -19.71875000204837036 ) ) ;
#24181=CARTESIAN_POINT ( 'NONE',  ( -5.405949406250003975, -9.363379034771801557, -130.8437500020484094 ) ) ;
#24183=CARTESIAN_POINT ( 'NONE',  ( -10.81189881249999729, 6.242252689847871849, -26.40625000204838102 ) ) ;
#24186=CARTESIAN_POINT ( 'NONE',  ( -10.00000000000000000, -5.773502691896251982, -59.62500000000000000 ) ) ;
#24187=CARTESIAN_POINT ( 'NONE',  ( -5.405949406249996869, 9.363379034771805109, -127.0312500020483952 ) ) ;
#24191=CARTESIAN_POINT ( 'NONE',  ( 10.00000000000000000, 5.773502691896255534, -99.75000000409679046 ) ) ;
#24194=CARTESIAN_POINT ( 'NONE',  ( 5.405949406249992428, -9.363379034771808662, -61.59375000204836681 ) ) ;
#24200=CARTESIAN_POINT ( 'NONE',  ( -9.999999999999998224, 1.224646799147353059E-15, -28.62500000409676204 ) ) ;
#24208=EDGE_LOOP ( 'NONE', ( #3649, #22755, #39099, #10059 ) ) ;
#24217=CARTESIAN_POINT ( 'NONE',  ( 10.81189881249999551, -6.242252689847874514, -121.4687500020484094 ) ) ;
#24218=CARTESIAN_POINT ( 'NONE',  ( 5.000000000000000000, 8.660254037844385522, -198.6250000040967905 ) ) ;
#24219=CARTESIAN_POINT ( 'NONE',  ( 10.81189881249999551, -6.242252689847874514, -123.1562500020483952 ) ) ;
#24221=CARTESIAN_POINT ( 'NONE',  ( 5.405949406249992428, -9.363379034771808662, -130.5937500020483810 ) ) ;
#24224=CARTESIAN_POINT ( 'NONE',  ( 10.00000000000000000, 5.773502691896255534, -159.3750000000000000 ) ) ;
#24225=CARTESIAN_POINT ( 'NONE',  ( 9.999999999999996447, -5.773502691896262640, -17.12499999999997158 ) ) ;
#24231=CARTESIAN_POINT ( 'NONE',  ( 5.405949406249999534, 9.363379034771803333, -46.09375000204838102 ) ) ;
#24232=CARTESIAN_POINT ( 'NONE',  ( -9.999999999999227285, -5.773502691896698735, -111.0000000040967620 ) ) ;
#24233=CARTESIAN_POINT ( 'NONE',  ( -10.81189881249999729, 1.324075727343319199E-15, -150.5937500020483810 ) ) ;
#24237=CARTESIAN_POINT ( 'NONE',  ( 9.999999999999996447, -5.773502691896262640, -84.62499999999998579 ) ) ;
#24240=CARTESIAN_POINT ( 'NONE',  ( -5.405949406250003975, -9.363379034771801557, -105.5312500020483810 ) ) ;
#24241=CARTESIAN_POINT ( 'NONE',  ( -9.999999999999998224, 5.773502691896259087, -126.2500000040967763 ) ) ;
#24246=CARTESIAN_POINT ( 'NONE',  ( 10.81189881249999907, 6.242252689847868297, -40.40625000204836681 ) ) ;
#24248=CARTESIAN_POINT ( 'NONE',  ( 9.999999999999998224, 1.224646799147353059E-15, -99.99999999999998579 ) ) ;
#24254=ORIENTED_EDGE ( 'NONE', *, *, #29121, .T. ) ;
#24257=ORIENTED_EDGE ( 'NONE', *, *, #3826, .T. ) ;
#24266=CYLINDRICAL_SURFACE ( 'NONE', #10885, 9.999999999999998224 ) ;
#24271=CARTESIAN_POINT ( 'NONE',  ( 5.405949406249992428, -9.363379034771808662, -141.0937500020483810 ) ) ;
#24272=CARTESIAN_POINT ( 'NONE',  ( -10.81189881249999729, 6.242252689847871849, -153.7187500020483810 ) ) ;
#24275=CARTESIAN_POINT ( 'NONE',  ( -9.999999999999998224, 1.224646799147353059E-15, -121.2500000000000000 ) ) ;
#24276=CARTESIAN_POINT ( 'NONE',  ( 10.00000000000000000, 5.773502691896255534, -181.8750000000000000 ) ) ;
#24281=CARTESIAN_POINT ( 'NONE',  ( -5.405949406250003975, -9.363379034771801557, -174.3437500020484094 ) ) ;
#24284=FACE_OUTER_BOUND ( 'NONE', #16886, .T. ) ;
#24285=CARTESIAN_POINT ( 'NONE',  ( 10.81189881249999729, 0.000000000000000000, -45.03125000204838102 ) ) ;
#24287=CARTESIAN_POINT ( 'NONE',  ( -4.999999999999996447, 8.660254037844387298, -110.9999999999999858 ) ) ;
#24289=VERTEX_POINT ( 'NONE', #24996 ) ;
#24291=CARTESIAN_POINT ( 'NONE',  ( -5.405949406249996869, 9.363379034771805109, -122.5312500020483952 ) ) ;
#24292=CARTESIAN_POINT ( 'NONE',  ( 4.999999999999992006, -8.660254037844389075, -151.1250000040967905 ) ) ;
#24296=CARTESIAN_POINT ( 'NONE',  ( -10.81189881249999907, -6.242252689847864744, -177.4687500020484094 ) ) ;
#24299=FACE_OUTER_BOUND ( 'NONE', #36502, .T. ) ;
#24300=CARTESIAN_POINT ( 'NONE',  ( -5.405949406250003975, -9.363379034771801557, -72.53125000204838102 ) ) ;
#24302=CARTESIAN_POINT ( 'NONE',  ( -4.999999999999996447, 8.660254037844387298, -48.37500000409677625 ) ) ;
#24303=CARTESIAN_POINT ( 'NONE',  ( 10.81189881249999729, 0.000000000000000000, -8.843750002048345493 ) ) ;
#24307=CARTESIAN_POINT ( 'NONE',  ( -10.81189881249999729, 1.324075727343319199E-15, -2.281250002048373915 ) ) ;
#24308=CYLINDRICAL_SURFACE ( 'NONE', #23584, 9.999999999999998224 ) ;
#24310=FACE_OUTER_BOUND ( 'NONE', #41095, .T. ) ;
#24315=CYLINDRICAL_SURFACE ( 'NONE', #10312, 9.999999999999998224 ) ;
#24316=ORIENTED_EDGE ( 'NONE', *, *, #38837, .T. ) ;
#24323=EDGE_CURVE ( 'NONE', #36923, #18938, #18195, .T. ) ;
#24324=CARTESIAN_POINT ( 'NONE',  ( 10.00000000000000000, 5.773502691896255534, -40.87499999999997158 ) ) ;
#24327=EDGE_CURVE ( 'NONE', #34592, #9953, #38347, .T. ) ;
#24328=CARTESIAN_POINT ( 'NONE',  ( 5.405949406249992428, -9.363379034771808662, -165.0937500020484094 ) ) ;
#24329=CARTESIAN_POINT ( 'NONE',  ( -5.405949406249996869, 9.363379034771805109, -176.3437500020483810 ) ) ;
#24330=DIRECTION ( 'NONE',  ( -0.000000000000000000, -0.000000000000000000, -1.000000000000000000 ) ) ;
#24331=CARTESIAN_POINT ( 'NONE',  ( -9.999999999999998224, 0.000000000000000000, -99.99999999999998579 ) ) ;
#24332=AXIS2_PLACEMENT_3D ( 'NONE', #9000, #8791, #5553 ) ;
#24338=CARTESIAN_POINT ( 'NONE',  ( 10.81189881249999729, 0.000000000000000000, -61.34375000204836681 ) ) ;
#24339=CARTESIAN_POINT ( 'NONE',  ( 10.81189881249999551, -6.242252689847874514, -66.15625000204839523 ) ) ;
#24341=CARTESIAN_POINT ( 'NONE',  ( 9.999999999999998224, 0.000000000000000000, -132.5000000000000000 ) ) ;
#24342=CARTESIAN_POINT ( 'NONE',  ( 10.81189881249999729, 0.000000000000000000, -154.5312500020484094 ) ) ;
#24343=CARTESIAN_POINT ( 'NONE',  ( 5.405949406249999534, 9.363379034771803333, -169.2812500020484094 ) ) ;
#24346=CARTESIAN_POINT ( 'NONE',  ( -5.405949406250003975, -9.363379034771801557, -103.8437500020483810 ) ) ;
#24347=FACE_OUTER_BOUND ( 'NONE', #12808, .T. ) ;
#24349=CARTESIAN_POINT ( 'NONE',  ( -10.81189881249999729, 6.242252689847871849, -8.406250002048365033 ) ) ;
#24352=CARTESIAN_POINT ( 'NONE',  ( 5.405949406249992428, -9.363379034771808662, -99.28125000204839523 ) ) ;
#24354=CARTESIAN_POINT ( 'NONE',  ( 10.00000000000000000, 5.773502691896255534, -75.75000000409679046 ) ) ;
#24355=CARTESIAN_POINT ( 'NONE',  ( 9.999999999999998224, 0.000000000000000000, -135.5000000000000000 ) ) ;
#24356=CARTESIAN_POINT ( 'NONE',  ( -10.81189881249999907, -6.242252689847864744, -36.46875000204835260 ) ) ;
#24357=ORIENTED_EDGE ( 'NONE', *, *, #7506, .F. ) ;
#24359=CARTESIAN_POINT ( 'NONE',  ( 10.81189881249999729, 0.000000000000000000, -30.03125000204837036 ) ) ;
#24363=CARTESIAN_POINT ( 'NONE',  ( -2.121150477449813534E-15, -11.54700538379251284, -4.250000004096754047 ) ) ;
#24368=ORIENTED_EDGE ( 'NONE', *, *, #3752, .F. ) ;
#24369=DIRECTION ( 'NONE',  ( -0.000000000000000000, -0.000000000000000000, -1.000000000000000000 ) ) ;
#24377=EDGE_CURVE ( 'NONE', #28346, #7904, #3601, .T. ) ;
#24378=CARTESIAN_POINT ( 'NONE',  ( 5.344739998537471948, 9.251476015204525893, -99.99999999999995737 ) ) ;
#24381=CARTESIAN_POINT ( 'NONE',  ( -5.405949406250003975, -9.363379034771801557, -161.0312500020484094 ) ) ;
#24385=CARTESIAN_POINT ( 'NONE',  ( -5.405949406250003975, -9.363379034771801557, -91.84375000204838102 ) ) ;
#24387=CARTESIAN_POINT ( 'NONE',  ( 5.405949406249999534, 9.363379034771803333, -193.0937500020484094 ) ) ;
#24388=CARTESIAN_POINT ( 'NONE',  ( -10.81189881249999729, 1.324075727343319199E-15, -96.78125000204839523 ) ) ;
#24390=CARTESIAN_POINT ( 'NONE',  ( 5.405949406249992428, -9.363379034771808662, -109.5937500020483810 ) ) ;
#24392=CARTESIAN_POINT ( 'NONE',  ( 5.000000000000000000, 8.660254037844385522, -108.2499999999999858 ) ) ;
#24393=CARTESIAN_POINT ( 'NONE',  ( 7.644554776091147741E-16, 12.48450537969573659, -179.6562500020484094 ) ) ;
#24394=CARTESIAN_POINT ( 'NONE',  ( -10.81189881249999907, -6.242252689847864744, -194.1562500020484094 ) ) ;
#24396=CARTESIAN_POINT ( 'NONE',  ( 10.00000000000000000, 5.773502691896255534, -173.2500000040967905 ) ) ;
#24398=CARTESIAN_POINT ( 'NONE',  ( 5.405949406249999534, 9.363379034771803333, -20.59375000204835615 ) ) ;
#24400=CARTESIAN_POINT ( 'NONE',  ( -2.293366432827344421E-15, -12.48450537969573659, -133.7187500020483810 ) ) ;
#24402=CARTESIAN_POINT ( 'NONE',  ( -10.81189881249999907, -6.242252689847864744, -27.65625000204838457 ) ) ;
#24405=CARTESIAN_POINT ( 'NONE',  ( -10.00000000000000000, -5.773502691896251982, -52.12499999999997158 ) ) ;
#24406=CARTESIAN_POINT ( 'NONE',  ( 10.81189881249999907, 6.242252689847868297, -125.9062500020483810 ) ) ;
#24409=( BOUNDED_CURVE ( )  B_SPLINE_CURVE ( 2, ( #19682, #22943, #39538, #35891, #19473, #32658, #19261 ),
 .UNSPECIFIED., .F., .F. ) 
 B_SPLINE_CURVE_WITH_KNOTS ( ( 3, 2, 2, 3 ),
 ( 0.3619402985074628432, 0.3631840796019901729, 0.3644278606965175027, 0.3656716417910448325 ),
 .UNSPECIFIED. ) 
 CURVE ( )  GEOMETRIC_REPRESENTATION_ITEM ( )  RATIONAL_B_SPLINE_CURVE ( ( 0.9999999999999820144, 0.8660254037844566932, 1.000000000000000000, 0.8660254037844387076, 1.000000000000000000, 0.8660254037844327124, 1.000000000000005995 ) ) 
 REPRESENTATION_ITEM ( '' )  );
#24410=CARTESIAN_POINT ( 'NONE',  ( -5.000000000000003553, -8.660254037844383745, -98.87500000409677625 ) ) ;
#24413=CARTESIAN_POINT ( 'NONE',  ( -10.81189881249999729, 1.324075727343319199E-15, -60.59375000204836681 ) ) ;
#24419=DIRECTION ( 'NONE',  ( -1.000000000000000000, 0.000000000000000000, 0.000000000000000000 ) ) ;
#24420=CARTESIAN_POINT ( 'NONE',  ( 7.070501591499377789E-16, 11.54700538379251284, -24.50000000409676915 ) ) ;
#24431=CARTESIAN_POINT ( 'NONE',  ( -2.293366432827344421E-15, -12.48450537969573659, -198.4062500020484094 ) ) ;
#24437=CARTESIAN_POINT ( 'NONE',  ( -10.81189881249999729, 1.324075727343319199E-15, -117.5937500020483810 ) ) ;
#24438=CARTESIAN_POINT ( 'NONE',  ( 4.999999999999992006, -8.660254037844389075, -196.1250000040967905 ) ) ;
#24439=CARTESIAN_POINT ( 'NONE',  ( -5.405949406249996869, 9.363379034771805109, -121.0312500020483952 ) ) ;
#24441=CARTESIAN_POINT ( 'NONE',  ( 10.81189881249999551, -6.242252689847874514, -128.9687500020483810 ) ) ;
#24442=CARTESIAN_POINT ( 'NONE',  ( 10.00000000000000000, 5.773502691896255534, -150.3750000000000000 ) ) ;
#24443=CARTESIAN_POINT ( 'NONE',  ( 9.999999999999998224, 0.000000000000000000, -21.49999999999996447 ) ) ;
#24447=CARTESIAN_POINT ( 'NONE',  ( -9.999999999999998224, 1.224646799147353059E-15, -116.7499999999999858 ) ) ;
#24449=CARTESIAN_POINT ( 'NONE',  ( -10.81189881249999729, 6.242252689847871849, -47.21875000204836681 ) ) ;
#24450=CARTESIAN_POINT ( 'NONE',  ( -10.81189881249999729, 6.242252689847871849, -152.2187500020483526 ) ) ;
#24453=CARTESIAN_POINT ( 'NONE',  ( -4.637759744350153923, 8.887906374204987969, -179.9999999999999716 ) ) ;
#24454=CARTESIAN_POINT ( 'NONE',  ( 7.070501591499377789E-16, 11.54700538379251284, -79.62500000000000000 ) ) ;
#24457=CARTESIAN_POINT ( 'NONE',  ( 5.405949406249999534, 9.363379034771803333, -103.2812500020483952 ) ) ;
#24458=CARTESIAN_POINT ( 'NONE',  ( 9.999999999999998224, 0.000000000000000000, -125.3750000040967905 ) ) ;
#24459=DIRECTION ( 'NONE',  ( -1.000000000000000000, 0.000000000000000000, 0.000000000000000000 ) ) ;
#24462=CARTESIAN_POINT ( 'NONE',  ( -2.293366432827344421E-15, -12.48450537969573659, -46.90625000204837391 ) ) ;
#24463=CARTESIAN_POINT ( 'NONE',  ( 9.999999999999998224, 1.224646799147353059E-15, -99.99999999999998579 ) ) ;
#24467=VERTEX_POINT ( 'NONE', #38137 ) ;
#24469=ORIENTED_EDGE ( 'NONE', *, *, #21677, .F. ) ;
#24471=ORIENTED_EDGE ( 'NONE', *, *, #4603, .F. ) ;
#24476=CARTESIAN_POINT ( 'NONE',  ( -9.999999999999998224, 1.224646799147353059E-15, -133.2499999999999716 ) ) ;
#24480=CARTESIAN_POINT ( 'NONE',  ( -10.81189881249999729, 1.324075727343319199E-15, -143.0937500020483810 ) ) ;
#24481=CARTESIAN_POINT ( 'NONE',  ( -5.405949406249996869, 9.363379034771805109, -149.5312500020483810 ) ) ;
#24482=CARTESIAN_POINT ( 'NONE',  ( -2.293366432827344421E-15, -12.48450537969573659, -153.2187500020483810 ) ) ;
#24484=CARTESIAN_POINT ( 'NONE',  ( -9.999999999999479527, -5.773502691896549521, -139.5000000040967620 ) ) ;
#24485=CARTESIAN_POINT ( 'NONE',  ( 10.00000000000000000, 5.773502691896255534, -168.3750000000000000 ) ) ;
#24488=CARTESIAN_POINT ( 'NONE',  ( -9.999999999999479527, -5.773502691896549521, -124.5000000040967620 ) ) ;
#24489=CARTESIAN_POINT ( 'NONE',  ( -10.81189881249999729, 6.242252689847871849, -177.7187500020483810 ) ) ;
#24492=DIRECTION ( 'NONE',  ( -0.000000000000000000, -0.000000000000000000, -1.000000000000000000 ) ) ;
#24493=CARTESIAN_POINT ( 'NONE',  ( -5.405949406249996869, 9.363379034771805109, -46.03125000204838813 ) ) ;
#24495=CARTESIAN_POINT ( 'NONE',  ( -9.999999999999998224, 5.773502691896259087, -107.8749999999999858 ) ) ;
#24498=CARTESIAN_POINT ( 'NONE',  ( 5.405949406249992428, -9.363379034771808662, -124.7812500020483952 ) ) ;
#24499=CARTESIAN_POINT ( 'NONE',  ( -9.999999999999998224, 5.773502691896259087, -144.2500000040967905 ) ) ;
#24503=CARTESIAN_POINT ( 'NONE',  ( -2.293366432827344421E-15, -12.48450537969573659, -171.2187500020484094 ) ) ;
#24506=CARTESIAN_POINT ( 'NONE',  ( -10.81189881249999729, 6.242252689847871849, -71.40625000204839523 ) ) ;
#24509=CARTESIAN_POINT ( 'NONE',  ( -9.999999999999998224, 5.773502691896259087, -45.25000000409676915 ) ) ;
#24510=CARTESIAN_POINT ( 'NONE',  ( -10.81189881249999729, 1.324075727343319199E-15, -3.593750002048368142 ) ) ;
#24515=ORIENTED_EDGE ( 'NONE', *, *, #23598, .T. ) ;
#24523=CARTESIAN_POINT ( 'NONE',  ( 4.999999999999992006, -8.660254037844389075, -122.6250000040967905 ) ) ;
#24524=ORIENTED_EDGE ( 'NONE', *, *, #17760, .T. ) ;
#24525=AXIS2_PLACEMENT_3D ( 'NONE', #29188, #20090, #39938 ) ;
#24534=CARTESIAN_POINT ( 'NONE',  ( -4.999999999999996447, 8.660254037844387298, -32.99999999999997158 ) ) ;
#24536=CARTESIAN_POINT ( 'NONE',  ( 5.405949406249999534, 9.363379034771803333, -164.5937500020484094 ) ) ;
#24538=LINE ( 'NONE', #1442, #3323 ) ;
#24539=CARTESIAN_POINT ( 'NONE',  ( 7.070501591499376803E-16, 11.54700538379251284, -126.1249999999999858 ) ) ;
#24545=CARTESIAN_POINT ( 'NONE',  ( 5.405949406249992428, -9.363379034771808662, -58.59375000204835970 ) ) ;
#24547=CARTESIAN_POINT ( 'NONE',  ( -10.81189881249999729, 1.324075727343319199E-15, -65.28125000204838102 ) ) ;
#24549=CARTESIAN_POINT ( 'NONE',  ( 7.070501591499377789E-16, 11.54700538379251284, -133.6250000000000000 ) ) ;
#24550=VECTOR ( 'NONE', #6095, 1000.000000000000000 ) ;
#24551=CARTESIAN_POINT ( 'NONE',  ( 7.644554776091147741E-16, 12.48450537969573659, -151.1562500020484094 ) ) ;
#24552=CARTESIAN_POINT ( 'NONE',  ( -10.81189881249999729, 6.242252689847871849, -167.4062500020483810 ) ) ;
#24555=CARTESIAN_POINT ( 'NONE',  ( -5.405949406250003975, -9.363379034771801557, -100.8437500020483810 ) ) ;
#24558=CARTESIAN_POINT ( 'NONE',  ( -10.81189881249999729, 1.324075727343319199E-15, -192.5937500020484094 ) ) ;
#24562=CARTESIAN_POINT ( 'NONE',  ( 10.81189881249999729, 0.000000000000000000, -91.53125000204838102 ) ) ;
#24564=CARTESIAN_POINT ( 'NONE',  ( 9.999999999999996447, -5.773502691896262640, -74.50000000409677625 ) ) ;
#24566=CARTESIAN_POINT ( 'NONE',  ( -10.81189881249999729, 6.242252689847871849, -23.21875000204837036 ) ) ;
#24567=VERTEX_POINT ( 'NONE', #11793 ) ;
#24569=CARTESIAN_POINT ( 'NONE',  ( -5.405949406249996869, 9.363379034771805109, -31.03125000204837036 ) ) ;
#24570=EDGE_CURVE ( 'NONE', #17801, #8961, #37231, .T. ) ;
#24573=CARTESIAN_POINT ( 'NONE',  ( 10.00000000000000000, 5.773502691896255534, -6.750000004096756712 ) ) ;
#24582=VECTOR ( 'NONE', #31706, 1000.000000000000000 ) ;
#24587=DIRECTION ( 'NONE',  ( -0.000000000000000000, -0.000000000000000000, -1.000000000000000000 ) ) ;
#24590=CARTESIAN_POINT ( 'NONE',  ( -2.293366432827344421E-15, -12.48450537969573659, -165.4062500020483810 ) ) ;
#24592=CARTESIAN_POINT ( 'NONE',  ( -10.81189881249999729, 1.324075727343319199E-15, -86.09375000204836681 ) ) ;
#24594=CARTESIAN_POINT ( 'NONE',  ( 7.644554776091147741E-16, 12.48450537969573659, -194.4687500020484094 ) ) ;
#24595=CARTESIAN_POINT ( 'NONE',  ( 10.81189881249999907, 6.242252689847868297, -94.40625000204836681 ) ) ;
#24599=CARTESIAN_POINT ( 'NONE',  ( -5.405949406249996869, 9.363379034771805109, -170.5312500020484094 ) ) ;
#24600=CARTESIAN_POINT ( 'NONE',  ( 5.405949406249992428, -9.363379034771808662, -187.7812500020484094 ) ) ;
#24602=CARTESIAN_POINT ( 'NONE',  ( 4.999999999999992006, -8.660254037844389075, -161.6250000040967905 ) ) ;
#24604=CARTESIAN_POINT ( 'NONE',  ( 10.81189881249999907, 6.242252689847868297, -11.71875000204836148 ) ) ;
#24606=CARTESIAN_POINT ( 'NONE',  ( 7.644554776091147741E-16, 12.48450537969573659, -122.4687500020483952 ) ) ;
#24608=CARTESIAN_POINT ( 'NONE',  ( -10.81189881249999729, 6.242252689847871849, -30.90625000204835615 ) ) ;
#24612=CARTESIAN_POINT ( 'NONE',  ( 9.999999999999996447, -5.773502691896262640, -51.62499999999998579 ) ) ;
#24613=CARTESIAN_POINT ( 'NONE',  ( 7.644554776091147741E-16, 12.48450537969573659, -125.6562500020483810 ) ) ;
#24616=CARTESIAN_POINT ( 'NONE',  ( 7.070501591499377789E-16, 11.54700538379251284, -96.50000000409679046 ) ) ;
#24617=CARTESIAN_POINT ( 'NONE',  ( -9.999999999999742428, -5.773502691896402084, -151.5000000040967620 ) ) ;
#24620=CARTESIAN_POINT ( 'NONE',  ( 5.405949406249992428, -9.363379034771808662, -57.09375000204835970 ) ) ;
#24628=CARTESIAN_POINT ( 'NONE',  ( 9.999999999999996447, -5.773502691896262640, -29.50000000409674783 ) ) ;
#24634=CARTESIAN_POINT ( 'NONE',  ( -9.999999999999998224, 1.224646799147353059E-15, -142.6250000040967905 ) ) ;
#24645=CARTESIAN_POINT ( 'NONE',  ( -5.405949406249996869, 9.363379034771805109, -188.5312500020484094 ) ) ;
#24651=CARTESIAN_POINT ( 'NONE',  ( 5.405949406249992428, -9.363379034771808662, -109.5937500020483810 ) ) ;
#24653=CARTESIAN_POINT ( 'NONE',  ( -2.293366432827344421E-15, -12.48450537969573659, -114.4062500020483952 ) ) ;
#24655=CARTESIAN_POINT ( 'NONE',  ( 7.644554776091147741E-16, 12.48450537969573659, -132.9687500020483810 ) ) ;
#24658=FACE_OUTER_BOUND ( 'NONE', #39551, .T. ) ;
#24659=CARTESIAN_POINT ( 'NONE',  ( 10.00000000000000000, 5.773502691896255534, -147.3750000000000000 ) ) ;
#24660=CARTESIAN_POINT ( 'NONE',  ( -10.00000000000000000, -5.773502691896251982, -22.12499999999997868 ) ) ;
#24665=CARTESIAN_POINT ( 'NONE',  ( -10.81189881249999907, -6.242252689847864744, -46.96875000204835970 ) ) ;
#24667=CARTESIAN_POINT ( 'NONE',  ( -10.81189881249999729, 1.324075727343319199E-15, -158.0937500020483810 ) ) ;
#24669=CARTESIAN_POINT ( 'NONE',  ( 3.157157116567558486, 9.864526434127757426, -180.0000000000001137 ) ) ;
#24670=CARTESIAN_POINT ( 'NONE',  ( 9.999999999999998224, 0.000000000000000000, -73.99999999999998579 ) ) ;
#24673=CARTESIAN_POINT ( 'NONE',  ( 10.81189881249999729, 0.000000000000000000, -100.5312500020483952 ) ) ;
#24674=CARTESIAN_POINT ( 'NONE',  ( -9.999999999999998224, 5.773502691896259087, -121.7500000040967905 ) ) ;
#24675=CARTESIAN_POINT ( 'NONE',  ( -9.999999999999998224, 1.224646799147353059E-15, -124.2500000000000000 ) ) ;
#24676=CARTESIAN_POINT ( 'NONE',  ( 10.81189881249999729, 0.000000000000000000, -83.84375000204836681 ) ) ;
#24679=CARTESIAN_POINT ( 'NONE',  ( -5.405949406250003975, -9.363379034771801557, -42.53125000204838102 ) ) ;
#24680=EDGE_CURVE ( 'NONE', #6263, #15924, #16795, .T. ) ;
#24700=CARTESIAN_POINT ( 'NONE',  ( 10.81189881249999729, 0.000000000000000000, -142.3437500020483810 ) ) ;
#24701=CARTESIAN_POINT ( 'NONE',  ( 7.644554776091147741E-16, 12.48450537969573659, -146.6562500020484379 ) ) ;
#24702=CARTESIAN_POINT ( 'NONE',  ( -5.405949406250003975, -9.363379034771801557, -157.8437500020483810 ) ) ;
#24705=CARTESIAN_POINT ( 'NONE',  ( 4.999999999999992006, -8.660254037844389075, -174.7500000000000284 ) ) ;
#24709=CARTESIAN_POINT ( 'NONE',  ( -8.973374131346412597, -4.922417620657181914, -99.99999999999995737 ) ) ;
#24710=CARTESIAN_POINT ( 'NONE',  ( 7.644554776091147741E-16, 12.48450537969573659, -177.9687500020483810 ) ) ;
#24713=CARTESIAN_POINT ( 'NONE',  ( 9.999999999999998224, 0.000000000000000000, -134.0000000000000000 ) ) ;
#24714=CARTESIAN_POINT ( 'NONE',  ( 10.81189881249999907, 6.242252689847868297, -41.90625000204836681 ) ) ;
#24716=CARTESIAN_POINT ( 'NONE',  ( -9.999999999999998224, 5.773502691896259087, -101.8749999999999858 ) ) ;
#24717=ORIENTED_EDGE ( 'NONE', *, *, #28025, .F. ) ;
#24718=CARTESIAN_POINT ( 'NONE',  ( 10.81189881249999729, 0.000000000000000000, -126.0312500020483952 ) ) ;
#24719=CARTESIAN_POINT ( 'NONE',  ( -2.121150477449813534E-15, -11.54700538379251284, -149.7500000040968189 ) ) ;
#24722=VERTEX_POINT ( 'NONE', #37014 ) ;
#24723=CARTESIAN_POINT ( 'NONE',  ( -10.81189881249999729, 1.324075727343319199E-15, -176.0937500020484094 ) ) ;
#24728=CARTESIAN_POINT ( 'NONE',  ( -5.405949406249996869, 9.363379034771805109, -70.03125000204838102 ) ) ;
#24730=CARTESIAN_POINT ( 'NONE',  ( 10.00000000000000000, 5.773502691896255534, -42.75000000409676204 ) ) ;
#24731=CARTESIAN_POINT ( 'NONE',  ( -10.81189881249999729, 6.242252689847871849, -0.7187500020483517105 ) ) ;
#24732=LINE ( 'NONE', #14550, #17950 ) ;
#24743=CARTESIAN_POINT ( 'NONE',  ( 0.000000000000000000, 0.000000000000000000, 0.000000000000000000 ) ) ;
#24745=ORIENTED_EDGE ( 'NONE', *, *, #5686, .T. ) ;
#24753=CARTESIAN_POINT ( 'NONE',  ( 10.00000000000000000, 5.773502691896255534, -37.87499999999996447 ) ) ;
#24756=CARTESIAN_POINT ( 'NONE',  ( -5.405949406250003975, -9.363379034771801557, -168.3437500020484094 ) ) ;
#24758=CARTESIAN_POINT ( 'NONE',  ( -10.81189881249999729, -6.242252689847864744, -175.9687500020483526 ) ) ;
#24760=CARTESIAN_POINT ( 'NONE',  ( -5.000000000000003553, -8.660254037844383745, -167.8750000040967905 ) ) ;
#24762=CARTESIAN_POINT ( 'NONE',  ( 9.999999999999998224, 0.000000000000000000, -194.0000000000000000 ) ) ;
#24765=CARTESIAN_POINT ( 'NONE',  ( -9.999999999999998224, 1.224646799147353059E-15, -166.2500000000000000 ) ) ;
#24768=CARTESIAN_POINT ( 'NONE',  ( -10.81189881249999907, -6.242252689847864744, -58.96875000204838102 ) ) ;
#24769=CARTESIAN_POINT ( 'NONE',  ( -5.405949406250003975, -9.363379034771801557, -66.53125000204838102 ) ) ;
#24771=CARTESIAN_POINT ( 'NONE',  ( 9.999999999999996447, -5.773502691896262640, -134.1250000000000000 ) ) ;
#24772=CARTESIAN_POINT ( 'NONE',  ( -5.405949406249996869, 9.363379034771805109, -151.0312500020483810 ) ) ;
#24773=CARTESIAN_POINT ( 'NONE',  ( -5.405949406250003975, -9.363379034771801557, -167.0312500020484094 ) ) ;
#24775=CARTESIAN_POINT ( 'NONE',  ( 10.81189881249999907, 6.242252689847868297, -95.71875000204838102 ) ) ;
#24776=VERTEX_POINT ( 'NONE', #3795 ) ;
#24778=CARTESIAN_POINT ( 'NONE',  ( 7.644554776091147741E-16, 12.48450537969573659, -194.4687500020484094 ) ) ;
#24780=CARTESIAN_POINT ( 'NONE',  ( -1.306318075773550857, -10.33130266446697831, -180.0000000000000284 ) ) ;
#24781=CARTESIAN_POINT ( 'NONE',  ( 10.81189881249999551, -6.242252689847874514, -91.65625000204838102 ) ) ;
#24784=CARTESIAN_POINT ( 'NONE',  ( -2.121150477449813534E-15, -11.54700538379251284, -71.75000000409674783 ) ) ;
#24786=CARTESIAN_POINT ( 'NONE',  ( 10.81189881249999551, -6.242252689847874514, -29.96875000204834905 ) ) ;
#24789=CARTESIAN_POINT ( 'NONE',  ( -2.293366432827344421E-15, -12.48450537969573659, -22.90625000204837747 ) ) ;
#24801=ORIENTED_EDGE ( 'NONE', *, *, #25160, .T. ) ;
#24807=CYLINDRICAL_SURFACE ( 'NONE', #168, 9.999999999999998224 ) ;
#24810=DIRECTION ( 'NONE',  ( -0.000000000000000000, -0.000000000000000000, -1.000000000000000000 ) ) ;
#24811=CARTESIAN_POINT ( 'NONE',  ( -5.405949406249996869, 9.363379034771805109, -164.5312500020484094 ) ) ;
#24812=CARTESIAN_POINT ( 'NONE',  ( -9.999999999999998224, 1.224646799147353059E-15, -106.6250000040967763 ) ) ;
#24814=CARTESIAN_POINT ( 'NONE',  ( -5.405949406249996869, 9.363379034771805109, -81.84375000204838102 ) ) ;
#24816=CARTESIAN_POINT ( 'NONE',  ( -10.81189881249999729, 1.324075727343319199E-15, -191.0937500020484094 ) ) ;
#24817=CARTESIAN_POINT ( 'NONE',  ( 5.405949406249992428, -9.363379034771808662, -94.78125000204838102 ) ) ;
#24821=CARTESIAN_POINT ( 'NONE',  ( 10.81189881249999551, -6.242252689847874514, -174.1562500020484094 ) ) ;
#24822=CARTESIAN_POINT ( 'NONE',  ( 10.81189881249999907, 6.242252689847868297, -190.4062500020484094 ) ) ;
#24824=CARTESIAN_POINT ( 'NONE',  ( -2.121150477449813534E-15, -11.54700538379251284, -164.7500000040967620 ) ) ;
#24826=CARTESIAN_POINT ( 'NONE',  ( -5.405949406249996869, 9.363379034771805109, -9.843750002048345493 ) ) ;
#24828=CARTESIAN_POINT ( 'NONE',  ( -5.405949406249996869, 9.363379034771805109, -122.3437500020483952 ) ) ;
#24830=CARTESIAN_POINT ( 'NONE',  ( 10.81189881249999907, 6.242252689847868297, -22.40625000204838102 ) ) ;
#24833=CARTESIAN_POINT ( 'NONE',  ( -10.00000000000000000, -5.773502691896251982, -49.12499999999997158 ) ) ;
#24834=CARTESIAN_POINT ( 'NONE',  ( -5.405949406250003975, -9.363379034771801557, -116.0312500020483952 ) ) ;
#24837=CARTESIAN_POINT ( 'NONE',  ( 5.000000000000000000, 8.660254037844385522, -95.12500000409677625 ) ) ;
#24839=CARTESIAN_POINT ( 'NONE',  ( 10.81189881249999551, -6.242252689847874514, -46.46875000204836681 ) ) ;
#24845=CARTESIAN_POINT ( 'NONE',  ( -4.999999999999996447, 8.660254037844387298, -25.87500000409675849 ) ) ;
#24849=ORIENTED_EDGE ( 'NONE', *, *, #27172, .T. ) ;
#24856=CARTESIAN_POINT ( 'NONE',  ( -2.293366432827344421E-15, -12.48450537969573659, -189.4062500020484094 ) ) ;
#24861=ADVANCED_FACE ( 'NONE', ( #24299 ), #17356, .F. ) ;
#24863=CARTESIAN_POINT ( 'NONE',  ( -5.405949406249996869, 9.363379034771805109, -107.3437500020483810 ) ) ;
#24865=CARTESIAN_POINT ( 'NONE',  ( 10.81189881249999729, 0.000000000000000000, -117.0312500020483952 ) ) ;
#24867=CARTESIAN_POINT ( 'NONE',  ( 5.405949406249999534, 9.363379034771803333, -127.0937500020483668 ) ) ;
#24870=CARTESIAN_POINT ( 'NONE',  ( 5.000000000000000000, 8.660254037844385522, -147.2500000000000000 ) ) ;
#24871=CARTESIAN_POINT ( 'NONE',  ( -9.999999999999998224, 1.224646799147353059E-15, -11.74999999999995559 ) ) ;
#24874=CARTESIAN_POINT ( 'NONE',  ( -10.00000000000000000, -5.773502691896251982, -186.0000000040967905 ) ) ;
#24876=CARTESIAN_POINT ( 'NONE',  ( -10.81189881249999907, -6.242252689847864744, -34.96875000204835260 ) ) ;
#24877=CARTESIAN_POINT ( 'NONE',  ( -9.999999999999479527, -5.773502691896549521, -108.0000000040967478 ) ) ;
#24878=CARTESIAN_POINT ( 'NONE',  ( 7.644554776091147741E-16, 12.48450537969573659, -143.4687500020483810 ) ) ;
#24881=CARTESIAN_POINT ( 'NONE',  ( -9.999999999999998224, 5.773502691896259087, -71.87500000000000000 ) ) ;
#24882=CARTESIAN_POINT ( 'NONE',  ( 7.644554776091147741E-16, 12.48450537969573659, -140.6562500020484094 ) ) ;
#24885=CARTESIAN_POINT ( 'NONE',  ( 10.81189881249999551, -6.242252689847874514, -103.6562500020483810 ) ) ;
#24886=CARTESIAN_POINT ( 'NONE',  ( -9.999999999999998224, 5.773502691896259087, -124.7500000040967763 ) ) ;
#24887=CARTESIAN_POINT ( 'NONE',  ( 9.999999999999998224, 0.000000000000000000, -156.8750000040967905 ) ) ;
#24888=CARTESIAN_POINT ( 'NONE',  ( 10.81189881249999907, 6.242252689847868297, -76.21875000204836681 ) ) ;
#24892=CARTESIAN_POINT ( 'NONE',  ( 10.81189881249999729, 0.000000000000000000, -46.53125000204838813 ) ) ;
#24898=ORIENTED_EDGE ( 'NONE', *, *, #11302, .T. ) ;
#24902=CARTESIAN_POINT ( 'NONE',  ( -4.999999999999996447, 8.660254037844387298, -103.5000000000000000 ) ) ;
#24912=CARTESIAN_POINT ( 'NONE',  ( -5.405949406250003975, -9.363379034771801557, -130.8437500020484094 ) ) ;
#24913=CARTESIAN_POINT ( 'NONE',  ( -5.405949406249996869, 9.363379034771805109, -143.5312500020483810 ) ) ;
#24914=CARTESIAN_POINT ( 'NONE',  ( -10.81189881249999729, 6.242252689847871849, -156.7187500020483810 ) ) ;
#24915=EDGE_CURVE ( 'NONE', #41753, #17257, #38890, .T. ) ;
#24918=CARTESIAN_POINT ( 'NONE',  ( 10.00000000000000000, 5.773502691896255534, -171.3750000000000000 ) ) ;
#24919=EDGE_CURVE ( 'NONE', #28187, #17582, #27306, .T. ) ;
#24923=CARTESIAN_POINT ( 'NONE',  ( -5.000000000000003553, -8.660254037844383745, -149.5000000000000000 ) ) ;
#24924=CARTESIAN_POINT ( 'NONE',  ( 10.81189881249999551, -6.242252689847874514, -172.4687500020484094 ) ) ;
#24929=CARTESIAN_POINT ( 'NONE',  ( 10.81189881249999729, 0.000000000000000000, -43.53125000204838102 ) ) ;
#24931=CARTESIAN_POINT ( 'NONE',  ( -9.999999999999998224, 1.224646799147353059E-15, -97.24999999999998579 ) ) ;
#24933=CARTESIAN_POINT ( 'NONE',  ( 10.81189881249999729, 6.242252689847867408, -124.4062500020483810 ) ) ;
#24934=CARTESIAN_POINT ( 'NONE',  ( -9.999999999999998224, 5.773502691896259087, -150.2500000040968189 ) ) ;
#24935=CARTESIAN_POINT ( 'NONE',  ( -9.999999999999998224, 1.224646799147353059E-15, -167.7500000000000000 ) ) ;
#24938=CARTESIAN_POINT ( 'NONE',  ( 10.81189881249999551, -6.242252689847874514, -170.9687500020483810 ) ) ;
#24942=CARTESIAN_POINT ( 'NONE',  ( 10.81189881249999907, 6.242252689847868297, -70.40625000204839523 ) ) ;
#24944=CARTESIAN_POINT ( 'NONE',  ( -10.00000000000000000, -5.773502691896251982, -43.50000000409675494 ) ) ;
#24945=CARTESIAN_POINT ( 'NONE',  ( 10.81189881249999551, -6.242252689847874514, -1.468750002048352377 ) ) ;
#24951=CYLINDRICAL_SURFACE ( 'NONE', #4967, 9.999999999999998224 ) ;
#24956=ORIENTED_EDGE ( 'NONE', *, *, #3752, .T. ) ;
#24967=CARTESIAN_POINT ( 'NONE',  ( -9.999999999999998224, 1.224646799147353059E-15, -112.2499999999999858 ) ) ;
#24968=CARTESIAN_POINT ( 'NONE',  ( 9.999999999999998224, 0.000000000000000000, -36.49999999999997868 ) ) ;
#24971=CARTESIAN_POINT ( 'NONE',  ( 10.81189881249999907, 6.242252689847868297, -154.2187500020483810 ) ) ;
#24972=VECTOR ( 'NONE', #25837, 1000.000000000000000 ) ;
#24973=CARTESIAN_POINT ( 'NONE',  ( -5.405949406250003975, -9.363379034771801557, -175.8437500020483810 ) ) ;
#24976=CARTESIAN_POINT ( 'NONE',  ( 4.999999999999992006, -8.660254037844389075, -194.2500000000000000 ) ) ;
#24981=CARTESIAN_POINT ( 'NONE',  ( 7.644554776091147741E-16, 12.48450537969573659, -71.65625000204836681 ) ) ;
#24983=CARTESIAN_POINT ( 'NONE',  ( -9.999999999999998224, 1.224646799147353059E-15, -122.7500000000000000 ) ) ;
#24984=CARTESIAN_POINT ( 'NONE',  ( -5.405949406249996869, 9.363379034771805109, -146.5312500020483810 ) ) ;
#24985=CARTESIAN_POINT ( 'NONE',  ( -10.81189881249999729, 1.324075727343319199E-15, -162.7812500020484094 ) ) ;
#24987=ADVANCED_FACE ( 'NONE', ( #36800 ), #30130, .F. ) ;
#24989=CARTESIAN_POINT ( 'NONE',  ( -5.405949406249996869, 9.363379034771805109, -95.34375000204838102 ) ) ;
#24992=CARTESIAN_POINT ( 'NONE',  ( 10.81189881249999907, 6.242252689847868297, -194.7187500020484094 ) ) ;
#24994=( BOUNDED_CURVE ( )  B_SPLINE_CURVE ( 2, ( #4320, #17458, #30656, #14211, #37332, #18755, #5601 ),
 .UNSPECIFIED., .F., .F. ) 
 B_SPLINE_CURVE_WITH_KNOTS ( ( 3, 2, 2, 3 ),
 ( 0.2014925373134328901, 0.2027363184079602476, 0.2039800995024875774, 0.2052238805970149627 ),
 .UNSPECIFIED. ) 
 CURVE ( )  GEOMETRIC_REPRESENTATION_ITEM ( )  RATIONAL_B_SPLINE_CURVE ( ( 0.9999999999999940048, 0.8660254037844447028, 1.000000000000000000, 0.8660254037844387076, 1.000000000000000000, 0.8660254037844357100, 1.000000000000002887 ) ) 
 REPRESENTATION_ITEM ( '' )  );
#24995=CARTESIAN_POINT ( 'NONE',  ( 0.4008866336925647755, -10.45073322229274915, -180.0000000000001421 ) ) ;
#24996=CARTESIAN_POINT ( 'NONE',  ( -9.999999999999998224, 1.224646799147353059E-15, -108.1250000040967763 ) ) ;
#24997=CARTESIAN_POINT ( 'NONE',  ( 5.405949406249992428, -9.363379034771808662, -90.28125000204838102 ) ) ;
#24999=CARTESIAN_POINT ( 'NONE',  ( -9.999999999999998224, 5.773502691896259087, -70.75000000409677625 ) ) ;
#25001=CARTESIAN_POINT ( 'NONE',  ( 5.405949406249992428, -9.363379034771808662, -30.09375000204836326 ) ) ;
#25004=CARTESIAN_POINT ( 'NONE',  ( 10.81189881249999729, 0.000000000000000000, -21.03125000204836326 ) ) ;
#25021=CARTESIAN_POINT ( 'NONE',  ( 9.057408897214770604, 5.192877711771748395, -100.0000000000000000 ) ) ;
#25023=CARTESIAN_POINT ( 'NONE',  ( 10.81189881249999551, -6.242252689847874514, -162.1562500020484379 ) ) ;
#25026=CARTESIAN_POINT ( 'NONE',  ( 5.405949406249999534, 9.363379034771803333, -83.59375000204836681 ) ) ;
#25028=CARTESIAN_POINT ( 'NONE',  ( -10.81189881249999907, -6.242252689847864744, -196.9687500020484379 ) ) ;
#25029=CARTESIAN_POINT ( 'NONE',  ( -2.293366432827344421E-15, -12.48450537969573659, -96.40625000204839523 ) ) ;
#25034=CARTESIAN_POINT ( 'NONE',  ( 5.405949406249992428, -9.363379034771808662, -177.2812500020484094 ) ) ;
#25035=CARTESIAN_POINT ( 'NONE',  ( 10.81189881249999907, 6.242252689847868297, -185.9062500020484094 ) ) ;
#25037=CARTESIAN_POINT ( 'NONE',  ( -5.000000000000003553, -8.660254037844383745, -167.8750000040967905 ) ) ;
#25039=CARTESIAN_POINT ( 'NONE',  ( 10.81189881249999907, 6.242252689847868297, -14.71875000204836326 ) ) ;
#25041=CARTESIAN_POINT ( 'NONE',  ( 10.81189881249999729, 0.000000000000000000, -122.8437500020483952 ) ) ;
#25043=CARTESIAN_POINT ( 'NONE',  ( 5.405949406249999534, 9.363379034771803333, -19.28125000204835970 ) ) ;
#25046=CARTESIAN_POINT ( 'NONE',  ( -10.00000000000000000, -5.773502691896251982, -55.12499999999997868 ) ) ;
#25047=CARTESIAN_POINT ( 'NONE',  ( -5.405949406249996869, 9.363379034771805109, -116.5312500020483952 ) ) ;
#25049=ORIENTED_EDGE ( 'NONE', *, *, #38833, .T. ) ;
#25050=CARTESIAN_POINT ( 'NONE',  ( -4.999999999999996447, 8.660254037844387298, -90.37500000409677625 ) ) ;
#25053=CARTESIAN_POINT ( 'NONE',  ( -10.81189881249999729, 6.242252689847871849, -48.71875000204836681 ) ) ;
#25054=ORIENTED_EDGE ( 'NONE', *, *, #21859, .T. ) ;
#25058=CARTESIAN_POINT ( 'NONE',  ( 5.000000000000000000, 8.660254037844385522, -17.12500000409675138 ) ) ;
#25059=EDGE_CURVE ( 'NONE', #1756, #33113, #22624, .T. ) ;
#25068=ORIENTED_EDGE ( 'NONE', *, *, #19874, .F. ) ;
#25069=ORIENTED_EDGE ( 'NONE', *, *, #13251, .T. ) ;
#25072=CARTESIAN_POINT ( 'NONE',  ( 5.405949406249992428, -9.363379034771808662, -190.7812500020484094 ) ) ;
#25076=CARTESIAN_POINT ( 'NONE',  ( 10.81189881249999551, -6.242252689847874514, -109.4687500020483810 ) ) ;
#25078=CARTESIAN_POINT ( 'NONE',  ( -10.81189881249999729, 1.324075727343319199E-15, -116.2812500020483952 ) ) ;
#25080=CARTESIAN_POINT ( 'NONE',  ( 10.81189881249999729, 0.000000000000000000, -122.8437500020483952 ) ) ;
#25083=CARTESIAN_POINT ( 'NONE',  ( -9.999999999999998224, 5.773502691896259087, -148.3750000000000000 ) ) ;
#25084=CARTESIAN_POINT ( 'NONE',  ( -2.121150477449813534E-15, -11.54700538379251284, -14.37499999999997158 ) ) ;
#25087=CARTESIAN_POINT ( 'NONE',  ( -4.999999999999996447, 8.660254037844387298, -186.3750000040967905 ) ) ;
#25089=CARTESIAN_POINT ( 'NONE',  ( -5.405949406249996869, 9.363379034771805109, -39.84375000204837391 ) ) ;
#25091=CARTESIAN_POINT ( 'NONE',  ( -10.81189881249999729, 1.324075727343319199E-15, -143.0937500020483810 ) ) ;
#25093=CARTESIAN_POINT ( 'NONE',  ( -9.999999999999998224, 1.224646799147353059E-15, -148.2500000000000000 ) ) ;
#25094=CARTESIAN_POINT ( 'NONE',  ( -9.999999999999998224, 1.224646799147353059E-15, -74.74999999999998579 ) ) ;
#25095=CARTESIAN_POINT ( 'NONE',  ( 10.81189881249999551, -6.242252689847874514, -141.1562500020484094 ) ) ;
#25098=CARTESIAN_POINT ( 'NONE',  ( 5.405949406249992428, -9.363379034771808662, -100.7812500020483952 ) ) ;
#25099=CARTESIAN_POINT ( 'NONE',  ( 9.999999999999998224, 0.000000000000000000, -113.3750000040967763 ) ) ;
#25100=CARTESIAN_POINT ( 'NONE',  ( 10.00000000000025402, -5.773502691896113426, -140.1250000000000000 ) ) ;
#25101=CARTESIAN_POINT ( 'NONE',  ( 5.405949406249999534, 9.363379034771803333, -77.59375000204838102 ) ) ;
#25104=CARTESIAN_POINT ( 'NONE',  ( -10.81189881249999729, 1.324075727343319199E-15, -41.28125000204838102 ) ) ;
#25108=CARTESIAN_POINT ( 'NONE',  ( 7.070501591499376803E-16, 11.54700538379251284, -153.1250000000000000 ) ) ;
#25109=EDGE_CURVE ( 'NONE', #42437, #30972, #27041, .T. ) ;
#25112=ORIENTED_EDGE ( 'NONE', *, *, #29095, .F. ) ;
#25122=CARTESIAN_POINT ( 'NONE',  ( -5.405949406249996869, 9.363379034771805109, -135.8437500020484094 ) ) ;
#25123=CARTESIAN_POINT ( 'NONE',  ( -5.405949406250003975, -9.363379034771801557, -143.0312500020483810 ) ) ;
#25124=CARTESIAN_POINT ( 'NONE',  ( -2.293366432827344421E-15, -12.48450537969573659, -147.2187500020484094 ) ) ;
#25127=CARTESIAN_POINT ( 'NONE',  ( 9.999999999999996447, -5.773502691896262640, -174.6250000000000000 ) ) ;
#25131=CARTESIAN_POINT ( 'NONE',  ( -10.30115550912761968, -1.362735121981329067, -99.99999999999994316 ) ) ;
#25132=CARTESIAN_POINT ( 'NONE',  ( 5.405949406249999534, 9.363379034771803333, -167.5937500020484094 ) ) ;
#25136=CARTESIAN_POINT ( 'NONE',  ( 10.81189881249999907, 6.242252689847868297, -43.40625000204836681 ) ) ;
#25138=CARTESIAN_POINT ( 'NONE',  ( -2.121150477449813534E-15, -11.54700538379251284, -102.8749999999999858 ) ) ;
#25139=VERTEX_POINT ( 'NONE', #18220 ) ;
#25140=CARTESIAN_POINT ( 'NONE',  ( -5.405949406250003975, -9.363379034771801557, -123.5312500020483952 ) ) ;
#25141=CARTESIAN_POINT ( 'NONE',  ( 5.000000000000000000, 8.660254037844385522, -141.6250000040967905 ) ) ;
#25145=CARTESIAN_POINT ( 'NONE',  ( -10.81189881249999729, 1.324075727343319199E-15, -171.5937500020484094 ) ) ;
#25147=CARTESIAN_POINT ( 'NONE',  ( -2.121150477449813534E-15, -11.54700538379251284, -155.3750000000000000 ) ) ;
#25148=CARTESIAN_POINT ( 'NONE',  ( -5.405949406250003975, -9.363379034771801557, -65.03125000204838102 ) ) ;
#25149=CARTESIAN_POINT ( 'NONE',  ( 7.070501591499377789E-16, 11.54700538379251284, -41.00000000409676204 ) ) ;
#25155=VERTEX_POINT ( 'NONE', #11742 ) ;
#25160=EDGE_CURVE ( 'NONE', #7201, #41736, #38016, .T. ) ;
#25161=( BOUNDED_CURVE ( )  B_SPLINE_CURVE ( 2, ( #42217, #26261, #29496, #6613, #7045, #19979, #33168 ),
 .UNSPECIFIED., .F., .F. ) 
 B_SPLINE_CURVE_WITH_KNOTS ( ( 3, 2, 2, 3 ),
 ( 0.4179104477611941260, 0.4191542288557215112, 0.4203980099502488965, 0.4216417910447762818 ),
 .UNSPECIFIED. ) 
 CURVE ( )  GEOMETRIC_REPRESENTATION_ITEM ( )  RATIONAL_B_SPLINE_CURVE ( ( 0.9999999999999880096, 0.8660254037844506980, 1.000000000000000000, 0.8660254037844387076, 1.000000000000000000, 0.8660254037844207220, 1.000000000000017986 ) ) 
 REPRESENTATION_ITEM ( '' )  );
#25162=LINE ( 'NONE', #16997, #22071 ) ;
#25171=CYLINDRICAL_SURFACE ( 'NONE', #2489, 9.999999999999998224 ) ;
#25173=( BOUNDED_CURVE ( )  B_SPLINE_CURVE ( 2, ( #17042, #20077, #30242, #16826, #16397, #13163, #30025 ),
 .UNSPECIFIED., .F., .F. ) 
 B_SPLINE_CURVE_WITH_KNOTS ( ( 3, 2, 2, 3 ),
 ( 0.4589552238805971740, 0.4601990049751245593, 0.4614427860696518890, 0.4626865671641792743 ),
 .UNSPECIFIED. ) 
 CURVE ( )  GEOMETRIC_REPRESENTATION_ITEM ( )  RATIONAL_B_SPLINE_CURVE ( ( 0.9999999999999820144, 0.8660254037844566932, 1.000000000000000000, 0.8660254037844387076, 1.000000000000000000, 0.8660254037844207220, 1.000000000000017986 ) ) 
 REPRESENTATION_ITEM ( '' )  );
#25177=CARTESIAN_POINT ( 'NONE',  ( 5.000000000000000000, 8.660254037844385522, -39.24999999999997868 ) ) ;
#25181=CARTESIAN_POINT ( 'NONE',  ( 5.405949406249992428, -9.363379034771808662, -160.5937500020484094 ) ) ;
#25182=CARTESIAN_POINT ( 'NONE',  ( 7.644554776091147741E-16, 12.48450537969573659, -170.4687500020483810 ) ) ;
#25186=CARTESIAN_POINT ( 'NONE',  ( 10.00000000000000000, 5.773502691896255534, -196.8750000000000284 ) ) ;
#25191=CARTESIAN_POINT ( 'NONE',  ( 5.405949406249992428, -9.363379034771808662, -64.78125000204838102 ) ) ;
#25193=CARTESIAN_POINT ( 'NONE',  ( 5.000000000000000000, 8.660254037844385522, -120.2500000000000000 ) ) ;
#25195=CARTESIAN_POINT ( 'NONE',  ( -2.293366432827344421E-15, -12.48450537969573659, -153.4062500020483810 ) ) ;
#25196=CARTESIAN_POINT ( 'NONE',  ( 10.81189881249999729, 0.000000000000000000, -165.0312500020484094 ) ) ;
#25199=CARTESIAN_POINT ( 'NONE',  ( -10.81189881249999729, 1.324075727343319199E-15, -96.59375000204838102 ) ) ;
#25202=CARTESIAN_POINT ( 'NONE',  ( 10.81189881249999729, 0.000000000000000000, -0.03125000204837191653 ) ) ;
#25206=CARTESIAN_POINT ( 'NONE',  ( -10.81189881249999729, 1.324075727343319199E-15, -90.78125000204838102 ) ) ;
#25208=CARTESIAN_POINT ( 'NONE',  ( 9.999999999999998224, 0.000000000000000000, -69.87500000409677625 ) ) ;
#25210=CARTESIAN_POINT ( 'NONE',  ( 10.81189881249999907, 6.242252689847868297, -29.71875000204834549 ) ) ;
#25213=CARTESIAN_POINT ( 'NONE',  ( -10.81189881249999907, -6.242252689847864744, -17.15625000204837391 ) ) ;
#25217=CARTESIAN_POINT ( 'NONE',  ( 9.999999999999998224, 0.000000000000000000, 0.6249999959032359609 ) ) ;
#25229=AXIS2_PLACEMENT_3D ( 'NONE', #1543, #4765, #5199 ) ;
#25232=CARTESIAN_POINT ( 'NONE',  ( 5.405949406249999534, 9.363379034771803333, -164.7812500020484094 ) ) ;
#25234=CARTESIAN_POINT ( 'NONE',  ( -5.000000000000003553, -8.660254037844383745, -172.3750000040968189 ) ) ;
#25238=CARTESIAN_POINT ( 'NONE',  ( -5.405949406249996869, 9.363379034771805109, -86.34375000204836681 ) ) ;
#25239=CARTESIAN_POINT ( 'NONE',  ( -10.81189881249999729, 1.324075727343319199E-15, -194.0937500020484094 ) ) ;
#25240=CARTESIAN_POINT ( 'NONE',  ( 5.405949406249992428, -9.363379034771808662, -96.28125000204838102 ) ) ;
#25243=CARTESIAN_POINT ( 'NONE',  ( 4.999999999999992006, -8.660254037844389075, -150.7500000000000000 ) ) ;
#25244=CARTESIAN_POINT ( 'NONE',  ( -5.405949406249996869, 9.363379034771805109, -172.0312500020484094 ) ) ;
#25245=CARTESIAN_POINT ( 'NONE',  ( -10.81189881249999729, 6.242252689847871849, -191.4062500020484094 ) ) ;
#25247=CARTESIAN_POINT ( 'NONE',  ( 5.000000000000000000, 8.660254037844385522, -165.6250000040967905 ) ) ;
#25249=CARTESIAN_POINT ( 'NONE',  ( 10.81189881249999729, 0.000000000000000000, -11.84375000204834727 ) ) ;
#25251=CARTESIAN_POINT ( 'NONE',  ( -2.293366432827344421E-15, -12.48450537969573659, -123.2187500020483952 ) ) ;
#25253=CARTESIAN_POINT ( 'NONE',  ( 7.644554776091147741E-16, 12.48450537969573659, -22.15625000204837747 ) ) ;
#25255=CARTESIAN_POINT ( 'NONE',  ( 0.000000000000000000, 0.000000000000000000, -99.99999999999998579 ) ) ;
#25256=CARTESIAN_POINT ( 'NONE',  ( 10.81189881249999729, 0.000000000000000000, -114.0312500020483952 ) ) ;
#25259=CARTESIAN_POINT ( 'NONE',  ( -9.999999999999998224, 5.773502691896259087, -88.75000000409677625 ) ) ;
#25262=CARTESIAN_POINT ( 'NONE',  ( 10.81189881249999551, -6.242252689847874514, -49.46875000204836681 ) ) ;
#25267=CARTESIAN_POINT ( 'NONE',  ( 10.00000000000000000, 5.773502691896255534, -20.25000000409676915 ) ) ;
#25268=VECTOR ( 'NONE', #17602, 1000.000000000000000 ) ;
#25273=CARTESIAN_POINT ( 'NONE',  ( 9.999999999999479527, 5.773502691896553074, -143.2500000040967905 ) ) ;
#25279=ORIENTED_EDGE ( 'NONE', *, *, #3276, .T. ) ;
#25281=DIRECTION ( 'NONE',  ( -0.000000000000000000, -0.000000000000000000, -1.000000000000000000 ) ) ;
#25282=( BOUNDED_CURVE ( )  B_SPLINE_CURVE ( 2, ( #25460, #28700, #41827, #22847, #32771, #28907, #5809 ),
 .UNSPECIFIED., .F., .F. ) 
 B_SPLINE_CURVE_WITH_KNOTS ( ( 3, 2, 2, 3 ),
 ( 0.2126865671641791633, 0.2139303482587065208, 0.2151741293532339061, 0.2164179104477612636 ),
 .UNSPECIFIED. ) 
 CURVE ( )  GEOMETRIC_REPRESENTATION_ITEM ( )  RATIONAL_B_SPLINE_CURVE ( ( 0.9999999999999940048, 0.8660254037844447028, 1.000000000000000000, 0.8660254037844387076, 1.000000000000000000, 0.8660254037844297148, 1.000000000000008882 ) ) 
 REPRESENTATION_ITEM ( '' )  );
#25284=CARTESIAN_POINT ( 'NONE',  ( -5.405949406250003975, -9.363379034771801557, -189.5312500020484094 ) ) ;
#25287=CARTESIAN_POINT ( 'NONE',  ( -10.81189881249999907, -6.242252689847864744, -106.9687500020483668 ) ) ;
#25289=CARTESIAN_POINT ( 'NONE',  ( 10.81189881249999551, -6.242252689847874514, -114.1562500020483952 ) ) ;
#25291=CARTESIAN_POINT ( 'NONE',  ( 5.405949406249992428, -9.363379034771808662, -123.0937500020483952 ) ) ;
#25295=CARTESIAN_POINT ( 'NONE',  ( -9.999999999999998224, 5.773502691896259087, -143.8750000000000000 ) ) ;
#25296=CARTESIAN_POINT ( 'NONE',  ( -9.999999999999998224, 1.224646799147353059E-15, -13.24999999999995559 ) ) ;
#25299=CARTESIAN_POINT ( 'NONE',  ( -2.121150477449813534E-15, -11.54700538379251284, -188.7500000040967905 ) ) ;
#25301=CARTESIAN_POINT ( 'NONE',  ( -10.81189881249999907, -6.242252689847864744, -40.96875000204835260 ) ) ;
#25303=CARTESIAN_POINT ( 'NONE',  ( -5.405949406250003975, -9.363379034771801557, -148.8437500020483810 ) ) ;
#25306=CARTESIAN_POINT ( 'NONE',  ( -5.000000000000003553, -8.660254037844383745, -77.49999999999998579 ) ) ;
#25307=CARTESIAN_POINT ( 'NONE',  ( 10.81189881249999907, 6.242252689847868297, -143.9062500020484094 ) ) ;
#25309=ORIENTED_EDGE ( 'NONE', *, *, #18345, .T. ) ;
#25311=CARTESIAN_POINT ( 'NONE',  ( 9.999999999999998224, 0.000000000000000000, -114.8750000040967905 ) ) ;
#25312=CARTESIAN_POINT ( 'NONE',  ( 5.000000000000000000, 8.660254037844385522, -169.7500000000000000 ) ) ;
#25313=CARTESIAN_POINT ( 'NONE',  ( -10.81189881249999907, -6.242252689847864744, -75.46875000204836681 ) ) ;
#25317=CARTESIAN_POINT ( 'NONE',  ( 7.644554776091147741E-16, 12.48450537969573659, -35.65625000204835970 ) ) ;
#25322=CARTESIAN_POINT ( 'NONE',  ( 9.999999999999998224, 0.000000000000000000, -171.8750000040968189 ) ) ;
#25324=EDGE_CURVE ( 'NONE', #16951, #40108, #17055, .T. ) ;
#25328=FACE_OUTER_BOUND ( 'NONE', #42280, .T. ) ;
#25334=CARTESIAN_POINT ( 'NONE',  ( 0.000000000000000000, 0.000000000000000000, -169.9999999999999716 ) ) ;
#25335=CARTESIAN_POINT ( 'NONE',  ( 5.405949406249992428, -9.363379034771808662, -136.5937500020483810 ) ) ;
#25336=CARTESIAN_POINT ( 'NONE',  ( -2.293366432827344421E-15, -12.48450537969573659, -136.9062500020484094 ) ) ;
#25337=CARTESIAN_POINT ( 'NONE',  ( 10.81189881249999729, 0.000000000000000000, -149.8437500020483810 ) ) ;
#25339=CARTESIAN_POINT ( 'NONE',  ( -4.999999999999996447, 8.660254037844387298, -174.0000000000000284 ) ) ;
#25343=CARTESIAN_POINT ( 'NONE',  ( -6.652853726956784897, 8.522716305231336165, -100.0000000000000142 ) ) ;
#25345=CARTESIAN_POINT ( 'NONE',  ( 10.81189881249999907, 6.242252689847868297, -166.2187500020484094 ) ) ;
#25348=CARTESIAN_POINT ( 'NONE',  ( 9.999999999999998224, 0.000000000000000000, -173.0000000000000284 ) ) ;
#25349=CARTESIAN_POINT ( 'NONE',  ( -2.293366432827344421E-15, -12.48450537969573659, -39.40625000204836681 ) ) ;
#25351=CARTESIAN_POINT ( 'NONE',  ( 7.070501591499377789E-16, 11.54700538379251284, -100.6250000000000000 ) ) ;
#25353=CARTESIAN_POINT ( 'NONE',  ( -10.81189881249999729, 6.242252689847871849, -116.4062500020483952 ) ) ;
#25354=CARTESIAN_POINT ( 'NONE',  ( -9.999999999999998224, 5.773502691896259087, -139.7500000040967905 ) ) ;
#25359=CARTESIAN_POINT ( 'NONE',  ( -10.81189881249999729, 6.242252689847871849, -65.40625000204838102 ) ) ;
#25362=APPLICATION_CONTEXT ( 'configuration controlled 3d designs of mechanical parts and assemblies' ) ;
#25363=CARTESIAN_POINT ( 'NONE',  ( 4.999999999999992006, -8.660254037844389075, -162.7500000000000000 ) ) ;
#25365=ORIENTED_EDGE ( 'NONE', *, *, #28344, .F. ) ;
#25367=( BOUNDED_CURVE ( )  B_SPLINE_CURVE ( 2, ( #4382, #33744, #10837, #27473, #1149, #23811, #26830 ),
 .UNSPECIFIED., .F., .F. ) 
 B_SPLINE_CURVE_WITH_KNOTS ( ( 3, 2, 2, 3 ),
 ( 0.3171641791044778058, 0.3184079601990050801, 0.3196517412935324653, 0.3208955223880597396 ),
 .UNSPECIFIED. ) 
 CURVE ( )  GEOMETRIC_REPRESENTATION_ITEM ( )  RATIONAL_B_SPLINE_CURVE ( ( 0.9999999999999820144, 0.8660254037844566932, 1.000000000000000000, 0.8660254037844387076, 1.000000000000000000, 0.8660254037844327124, 1.000000000000005995 ) ) 
 REPRESENTATION_ITEM ( '' )  );
#25374=VERTEX_POINT ( 'NONE', #41944 ) ;
#25380=DIRECTION ( 'NONE',  ( 1.000000000000000000, 0.000000000000000000, 0.000000000000000000 ) ) ;
#25381=CARTESIAN_POINT ( 'NONE',  ( 7.070501591499377789E-16, 11.54700538379251284, -33.12499999999995737 ) ) ;
#25384=CARTESIAN_POINT ( 'NONE',  ( -5.405949406249996869, 9.363379034771805109, -158.3437500020483810 ) ) ;
#25385=CARTESIAN_POINT ( 'NONE',  ( 10.81189881249999729, 6.242252689847867408, -167.7187500020483526 ) ) ;
#25387=CARTESIAN_POINT ( 'NONE',  ( -9.999999999999998224, 1.224646799147353059E-15, -194.7500000000000000 ) ) ;
#25394=ADVANCED_FACE ( 'NONE', ( #18871 ), #13213, .F. ) ;
#25395=CARTESIAN_POINT ( 'NONE',  ( -5.405949406249996869, 9.363379034771805109, -61.03125000204837391 ) ) ;
#25397=CARTESIAN_POINT ( 'NONE',  ( 9.999999999999998224, 0.000000000000000000, -123.5000000000000000 ) ) ;
#25399=CARTESIAN_POINT ( 'NONE',  ( -10.81189881249999729, -6.242252689847864744, -147.6562500020483810 ) ) ;
#25400=CARTESIAN_POINT ( 'NONE',  ( -10.81189881249999907, -6.242252689847864744, -165.6562500020483810 ) ) ;
#25403=CARTESIAN_POINT ( 'NONE',  ( 10.81189881249999907, 6.242252689847868297, -101.7187500020483810 ) ) ;
#25404=ORIENTED_EDGE ( 'NONE', *, *, #8237, .T. ) ;
#25406=CARTESIAN_POINT ( 'NONE',  ( 10.81189881249999729, 0.000000000000000000, -193.3437500020484094 ) ) ;
#25409=CARTESIAN_POINT ( 'NONE',  ( 9.999999999999998224, 0.000000000000000000, -144.5000000000000000 ) ) ;
#25410=CARTESIAN_POINT ( 'NONE',  ( 10.81189881249999551, -6.242252689847874514, -88.65625000204838102 ) ) ;
#25413=CARTESIAN_POINT ( 'NONE',  ( -9.999999999999998224, 5.773502691896259087, -66.25000000409677625 ) ) ;
#25415=CARTESIAN_POINT ( 'NONE',  ( -10.81189881249999907, -6.242252689847864744, -25.96875000204837391 ) ) ;
#25418=CARTESIAN_POINT ( 'NONE',  ( 5.405949406249999534, 9.363379034771803333, -20.78125000204836326 ) ) ;
#25431=VECTOR ( 'NONE', #6911, 1000.000000000000000 ) ;
#25437=CARTESIAN_POINT ( 'NONE',  ( 9.999999999999998224, 0.000000000000000000, -173.0000000000000284 ) ) ;
#25440=DIRECTION ( 'NONE',  ( -1.000000000000000000, 0.000000000000000000, 0.000000000000000000 ) ) ;
#25441=CARTESIAN_POINT ( 'NONE',  ( -2.293366432827344421E-15, -12.48450537969573659, -153.4062500020483810 ) ) ;
#25443=CARTESIAN_POINT ( 'NONE',  ( -9.999999999999998224, 1.224646799147353059E-15, -172.6250000040968189 ) ) ;
#25447=CARTESIAN_POINT ( 'NONE',  ( 5.405949406249999534, 9.363379034771803333, -86.59375000204836681 ) ) ;
#25448=CARTESIAN_POINT ( 'NONE',  ( -10.81189881249999729, 1.324075727343319199E-15, -90.78125000204838102 ) ) ;
#25453=CARTESIAN_POINT ( 'NONE',  ( -5.405949406249996869, 9.363379034771805109, -173.5312500020484094 ) ) ;
#25454=CARTESIAN_POINT ( 'NONE',  ( -5.405949406250003975, -9.363379034771801557, -186.5312500020484094 ) ) ;
#25457=CARTESIAN_POINT ( 'NONE',  ( 4.999999999999992006, -8.660254037844389075, -163.1250000040967905 ) ) ;
#25459=CARTESIAN_POINT ( 'NONE',  ( -5.405949406249996869, 9.363379034771805109, -14.34375000204834905 ) ) ;
#25460=CARTESIAN_POINT ( 'NONE',  ( -9.999999999999998224, 1.224646799147353059E-15, -157.2500000000000000 ) ) ;
#25461=CARTESIAN_POINT ( 'NONE',  ( -10.81189881249999907, -6.242252689847864744, -118.9687500020483810 ) ) ;
#25463=CARTESIAN_POINT ( 'NONE',  ( 10.81189881249999551, -6.242252689847874514, -18.15625000204837391 ) ) ;
#25467=CARTESIAN_POINT ( 'NONE',  ( 5.405949406249999534, 9.363379034771803333, -119.7812500020483952 ) ) ;
#25469=ORIENTED_EDGE ( 'NONE', *, *, #23660, .F. ) ;
#25470=CARTESIAN_POINT ( 'NONE',  ( 9.999999999999996447, -5.773502691896262640, -95.50000000409677625 ) ) ;
#25473=CARTESIAN_POINT ( 'NONE',  ( 10.81189881249999729, 0.000000000000000000, -47.84375000204838102 ) ) ;
#25478=CARTESIAN_POINT ( 'NONE',  ( -5.000000000000003553, -8.660254037844383745, -23.87500000409675849 ) ) ;
#25482=ORIENTED_EDGE ( 'NONE', *, *, #11078, .F. ) ;
#25488=VERTEX_POINT ( 'NONE', #938 ) ;
#25490=( BOUNDED_CURVE ( )  B_SPLINE_CURVE ( 2, ( #34954, #12047, #21986, #37965, #25243, #1506, #31719 ),
 .UNSPECIFIED., .F., .F. ) 
 B_SPLINE_CURVE_WITH_KNOTS ( ( 3, 2, 2, 3 ),
 ( 0.2425373134328359381, 0.2437810945273632957, 0.2450248756218906532, 0.2462686567164180107 ),
 .UNSPECIFIED. ) 
 CURVE ( )  GEOMETRIC_REPRESENTATION_ITEM ( )  RATIONAL_B_SPLINE_CURVE ( ( 0.9999999999999880096, 0.8660254037844506980, 1.000000000000000000, 0.8660254037844387076, 1.000000000000000000, 0.8660254037844267172, 1.000000000000011990 ) ) 
 REPRESENTATION_ITEM ( '' )  );
#25492=CARTESIAN_POINT ( 'NONE',  ( 5.000000000000000000, 8.660254037844385522, -171.2500000000000000 ) ) ;
#25494=CARTESIAN_POINT ( 'NONE',  ( 5.405949406249992428, -9.363379034771808662, -186.2812500020484094 ) ) ;
#25498=CARTESIAN_POINT ( 'NONE',  ( 10.81189881249999907, 6.242252689847868297, -106.2187500020483668 ) ) ;
#25499=CARTESIAN_POINT ( 'NONE',  ( 4.999999999999992006, -8.660254037844389075, -149.6250000040967905 ) ) ;
#25500=CARTESIAN_POINT ( 'NONE',  ( -2.293366432827344421E-15, -12.48450537969573659, -117.4062500020483952 ) ) ;
#25502=CARTESIAN_POINT ( 'NONE',  ( 10.81189881249999551, -6.242252689847874514, -124.4687500020483952 ) ) ;
#25506=CARTESIAN_POINT ( 'NONE',  ( 7.070501591499377789E-16, 11.54700538379251284, -138.1250000000000000 ) ) ;
#25507=CARTESIAN_POINT ( 'NONE',  ( -10.00000000000000000, -5.773502691896251982, -11.62499999999996803 ) ) ;
#25510=CARTESIAN_POINT ( 'NONE',  ( -9.999999999999998224, 5.773502691896259087, -187.7500000040967905 ) ) ;
#25512=CARTESIAN_POINT ( 'NONE',  ( -5.405949406249996869, 9.363379034771805109, -36.84375000204836681 ) ) ;
#25513=CARTESIAN_POINT ( 'NONE',  ( 9.999999999999998224, 0.000000000000000000, -105.4999999999999858 ) ) ;
#25514=CARTESIAN_POINT ( 'NONE',  ( 10.81189881249999729, 0.000000000000000000, -145.3437500020483810 ) ) ;
#25516=CARTESIAN_POINT ( 'NONE',  ( 0.000000000000000000, 0.000000000000000000, -99.99999999999998579 ) ) ;
#25517=CARTESIAN_POINT ( 'NONE',  ( -2.121150477449813534E-15, -11.54700538379251284, -75.87500000000000000 ) ) ;
#25518=CARTESIAN_POINT ( 'NONE',  ( 5.405949406249999534, 9.363379034771803333, -139.2812500020483810 ) ) ;
#25521=CARTESIAN_POINT ( 'NONE',  ( 9.999999999999742428, 5.773502691896404748, -120.7500000040967905 ) ) ;
#25522=CARTESIAN_POINT ( 'NONE',  ( -10.00000000000000000, -5.773502691896251982, -117.0000000040967905 ) ) ;
#25524=CARTESIAN_POINT ( 'NONE',  ( -5.405949406250003975, -9.363379034771801557, -73.84375000204838102 ) ) ;
#25526=ADVANCED_FACE ( 'NONE', ( #27250 ), #37168, .F. ) ;
#25530=CARTESIAN_POINT ( 'NONE',  ( -10.81189881249999907, -6.242252689847864744, -39.65625000204836681 ) ) ;
#25535=CYLINDRICAL_SURFACE ( 'NONE', #22445, 9.999999999999998224 ) ;
#25537=( BOUNDED_CURVE ( )  B_SPLINE_CURVE ( 2, ( #509, #4151, #7392, #23795, #23374, #30499, #30280 ),
 .UNSPECIFIED., .F., .F. ) 
 B_SPLINE_CURVE_WITH_KNOTS ( ( 3, 2, 2, 3 ),
 ( 0.2873134328358210032, 0.2885572139303483885, 0.2898009950248757183, 0.2910447761194031036 ),
 .UNSPECIFIED. ) 
 CURVE ( )  GEOMETRIC_REPRESENTATION_ITEM ( )  RATIONAL_B_SPLINE_CURVE ( ( 0.9999999999999880096, 0.8660254037844506980, 1.000000000000000000, 0.8660254037844387076, 1.000000000000000000, 0.8660254037844267172, 1.000000000000011990 ) ) 
 REPRESENTATION_ITEM ( '' )  );
#25540=CARTESIAN_POINT ( 'NONE',  ( -2.121150477449813534E-15, -11.54700538379251284, -176.7500000040967620 ) ) ;
#25543=CARTESIAN_POINT ( 'NONE',  ( 10.00000000000025402, -5.773502691896113426, -130.0000000040967905 ) ) ;
#25547=CARTESIAN_POINT ( 'NONE',  ( 7.644554776091147741E-16, 12.48450537969573659, -135.9687500020483810 ) ) ;
#25548=CARTESIAN_POINT ( 'NONE',  ( 5.405949406249992428, -9.363379034771808662, -141.2812500020483810 ) ) ;
#25550=CARTESIAN_POINT ( 'NONE',  ( 5.405949406249992428, -9.363379034771808662, -145.5937500020483810 ) ) ;
#25552=CARTESIAN_POINT ( 'NONE',  ( -10.00000000000000000, -5.773502691896251982, -160.1250000000000284 ) ) ;
#25557=CARTESIAN_POINT ( 'NONE',  ( 10.81189881249999907, 6.242252689847868297, -61.21875000204836681 ) ) ;
#25558=CARTESIAN_POINT ( 'NONE',  ( 5.405949406249992428, -9.363379034771808662, -166.5937500020484094 ) ) ;
#25563=CARTESIAN_POINT ( 'NONE',  ( -5.405949406249996869, 9.363379034771805109, -35.53125000204837391 ) ) ;
#25565=CARTESIAN_POINT ( 'NONE',  ( 9.999999999999996447, -5.773502691896262640, -102.6249999999999858 ) ) ;
#25566=ORIENTED_EDGE ( 'NONE', *, *, #269, .F. ) ;
#25567=CARTESIAN_POINT ( 'NONE',  ( 5.405949406249992428, -9.363379034771808662, -120.2812500020483952 ) ) ;
#25568=CARTESIAN_POINT ( 'NONE',  ( -5.000000000000003553, -8.660254037844383745, -143.8750000040967905 ) ) ;
#25572=CARTESIAN_POINT ( 'NONE',  ( 5.405949406249999534, 9.363379034771803333, -64.28125000204836681 ) ) ;
#25573=CARTESIAN_POINT ( 'NONE',  ( 5.000000000000000000, 8.660254037844385522, -147.6250000040967905 ) ) ;
#25577=ADVANCED_FACE ( 'NONE', ( #30293 ), #30511, .F. ) ;
#25579=CARTESIAN_POINT ( 'NONE',  ( 10.00000000000012790, 5.773502691896179151, -173.2500000040967905 ) ) ;
#25584=CARTESIAN_POINT ( 'NONE',  ( -9.999999999999998224, 1.224646799147353059E-15, -100.6250000040967905 ) ) ;
#25592=CARTESIAN_POINT ( 'NONE',  ( -5.000000000000003553, -8.660254037844383745, -27.99999999999996803 ) ) ;
#25595=CARTESIAN_POINT ( 'NONE',  ( 10.81189881249999729, 0.000000000000000000, -158.8437500020483810 ) ) ;
#25596=CARTESIAN_POINT ( 'NONE',  ( 10.81189881249999551, -6.242252689847874514, -173.9687500020483810 ) ) ;
#25599=CARTESIAN_POINT ( 'NONE',  ( 4.999999999999992006, -8.660254037844389075, -195.7500000000000000 ) ) ;
#25604=CARTESIAN_POINT ( 'NONE',  ( 10.81189881249999907, 6.242252689847868297, -58.40625000204838102 ) ) ;
#25606=CARTESIAN_POINT ( 'NONE',  ( -9.999999999999998224, 1.224646799147353059E-15, -119.7500000000000000 ) ) ;
#25608=CARTESIAN_POINT ( 'NONE',  ( 10.81189881249999729, 0.000000000000000000, -141.0312500020483810 ) ) ;
#25609=CARTESIAN_POINT ( 'NONE',  ( 7.644554776091147741E-16, 12.48450537969573659, -157.1562500020484094 ) ) ;
#25612=FACE_OUTER_BOUND ( 'NONE', #3479, .T. ) ;
#25613=CARTESIAN_POINT ( 'NONE',  ( -5.405949406249996869, 9.363379034771805109, -86.34375000204836681 ) ) ;
#25616=CARTESIAN_POINT ( 'NONE',  ( 7.644554776091147741E-16, 12.48450537969573659, -191.4687500020484094 ) ) ;
#25621=CARTESIAN_POINT ( 'NONE',  ( -5.405949406249996869, 9.363379034771805109, -86.53125000204838102 ) ) ;
#25623=CARTESIAN_POINT ( 'NONE',  ( -9.999999999999998224, 5.773502691896259087, -69.25000000409677625 ) ) ;
#25625=CARTESIAN_POINT ( 'NONE',  ( -10.81189881249999907, -6.242252689847864744, -16.96875000204836681 ) ) ;
#25628=CARTESIAN_POINT ( 'NONE',  ( -2.293366432827344421E-15, -12.48450537969573659, -18.40625000204837391 ) ) ;
#25631=CARTESIAN_POINT ( 'NONE',  ( 9.999999999999998224, 0.000000000000000000, -170.0000000000000000 ) ) ;
#25640=VERTEX_POINT ( 'NONE', #23167 ) ;
#25641=VECTOR ( 'NONE', #7250, 1000.000000000000000 ) ;
#25645=( BOUNDED_CURVE ( )  B_SPLINE_CURVE ( 2, ( #37936, #8381, #18500, #21531, #20880, #34067, #8591 ),
 .UNSPECIFIED., .F., .F. ) 
 B_SPLINE_CURVE_WITH_KNOTS ( ( 3, 2, 2, 3 ),
 ( 0.3992537313432836799, 0.4004975124378110651, 0.4017412935323383949, 0.4029850746268657802 ),
 .UNSPECIFIED. ) 
 CURVE ( )  GEOMETRIC_REPRESENTATION_ITEM ( )  RATIONAL_B_SPLINE_CURVE ( ( 0.9999999999999880096, 0.8660254037844506980, 1.000000000000000000, 0.8660254037844387076, 1.000000000000000000, 0.8660254037844267172, 1.000000000000011990 ) ) 
 REPRESENTATION_ITEM ( '' )  );
#25648=CARTESIAN_POINT ( 'NONE',  ( -10.81189881249999729, 1.324075727343319199E-15, -155.2812500020484094 ) ) ;
#25650=AXIS2_PLACEMENT_3D ( 'NONE', #6859, #42461, #20011 ) ;
#25654=CARTESIAN_POINT ( 'NONE',  ( -10.81189881249999907, -6.242252689847864744, -76.96875000204836681 ) ) ;
#25655=CARTESIAN_POINT ( 'NONE',  ( -5.405949406249996869, 9.363379034771805109, -85.03125000204838102 ) ) ;
#25659=CARTESIAN_POINT ( 'NONE',  ( 10.81189881249999551, -6.242252689847874514, -165.1562500020483526 ) ) ;
#25660=CARTESIAN_POINT ( 'NONE',  ( -5.405949406249996869, 9.363379034771805109, -179.5312500020483810 ) ) ;
#25662=CARTESIAN_POINT ( 'NONE',  ( -9.999999999999998224, 1.224646799147353059E-15, -156.1250000040967905 ) ) ;
#25664=CARTESIAN_POINT ( 'NONE',  ( -5.405949406250003975, -9.363379034771801557, -1.843750002048366587 ) ) ;
#25666=CARTESIAN_POINT ( 'NONE',  ( -10.81189881249999907, -6.242252689847864744, -111.4687500020483810 ) ) ;
#25668=CARTESIAN_POINT ( 'NONE',  ( -10.81189881249999729, 1.324075727343319199E-15, -12.78125000204835615 ) ) ;
#25671=CARTESIAN_POINT ( 'NONE',  ( 7.644554776091147741E-16, 12.48450537969573659, -115.1562500020483952 ) ) ;
#25674=VECTOR ( 'NONE', #41381, 1000.000000000000000 ) ;
#25676=CARTESIAN_POINT ( 'NONE',  ( -9.999999999999998224, 1.224646799147353059E-15, -90.12500000409677625 ) ) ;
#25678=CARTESIAN_POINT ( 'NONE',  ( -5.405949406250003975, -9.363379034771801557, -51.34375000204835260 ) ) ;
#25683=CARTESIAN_POINT ( 'NONE',  ( -9.999999999999998224, 5.773502691896259087, -22.75000000409677270 ) ) ;
#25688=CARTESIAN_POINT ( 'NONE',  ( 10.00000000000051159, -5.773502691895965988, -152.1250000000000000 ) ) ;
#25698=LINE ( 'NONE', #22030, #42445 ) ;
#25702=CARTESIAN_POINT ( 'NONE',  ( -10.81189881249999729, 6.242252689847871849, -183.9062500020484094 ) ) ;
#25706=CARTESIAN_POINT ( 'NONE',  ( -10.81189881249999729, 6.242252689847871849, -98.21875000204838102 ) ) ;
#25708=CARTESIAN_POINT ( 'NONE',  ( 10.81189881249999907, 6.242252689847868297, -107.9062500020483668 ) ) ;
#25710=CARTESIAN_POINT ( 'NONE',  ( -10.81189881249999729, 1.324075727343319199E-15, -123.5937500020483952 ) ) ;
#25713=CARTESIAN_POINT ( 'NONE',  ( -2.121150477449813534E-15, -11.54700538379251284, -138.8750000000000000 ) ) ;
#25714=CARTESIAN_POINT ( 'NONE',  ( 9.999999999999996447, -5.773502691896262640, -14.12499999999997158 ) ) ;
#25715=EDGE_CURVE ( 'NONE', #41597, #34758, #7186, .T. ) ;
#25718=CARTESIAN_POINT ( 'NONE',  ( 9.999999999999998224, 0.000000000000000000, -185.3750000040967905 ) ) ;
#25720=CARTESIAN_POINT ( 'NONE',  ( -5.405949406249996869, 9.363379034771805109, -38.34375000204837391 ) ) ;
#25722=CARTESIAN_POINT ( 'NONE',  ( 10.81189881249999551, -6.242252689847874514, -137.9687500020483810 ) ) ;
#25725=CARTESIAN_POINT ( 'NONE',  ( 5.000000000000000000, 8.660254037844385522, -69.24999999999997158 ) ) ;
#25726=CARTESIAN_POINT ( 'NONE',  ( -10.81189881249999729, 1.324075727343319199E-15, -137.2812500020483810 ) ) ;
#25730=CARTESIAN_POINT ( 'NONE',  ( 9.999999999999996447, -5.773502691896262640, -118.0000000040967905 ) ) ;
#25732=CARTESIAN_POINT ( 'NONE',  ( 10.81189881249999907, 6.242252689847868297, -70.21875000204838102 ) ) ;
#25738=CARTESIAN_POINT ( 'NONE',  ( 5.405949406249992428, -9.363379034771808662, -34.78125000204837391 ) ) ;
#25742=CARTESIAN_POINT ( 'NONE',  ( -9.999999999999998224, 1.224646799147353059E-15, -152.7500000000000000 ) ) ;
#25744=CARTESIAN_POINT ( 'NONE',  ( 0.000000000000000000, 0.000000000000000000, -99.99999999999998579 ) ) ;
#25746=EDGE_LOOP ( 'NONE', ( #31758, #41572, #1484, #34777 ) ) ;
#25748=CARTESIAN_POINT ( 'NONE',  ( 10.00000000000044764, -5.773502691896004180, -176.5000000040967905 ) ) ;
#25756=CARTESIAN_POINT ( 'NONE',  ( 5.405949406249999534, 9.363379034771803333, -130.0937500020483810 ) ) ;
#25757=CARTESIAN_POINT ( 'NONE',  ( 5.405949406249992428, -9.363379034771808662, -144.2812500020483810 ) ) ;
#25759=CARTESIAN_POINT ( 'NONE',  ( -5.405949406250003975, -9.363379034771801557, -142.8437500020483810 ) ) ;
#25762=CARTESIAN_POINT ( 'NONE',  ( -2.121150477449813534E-15, -11.54700538379251284, -159.8750000000000000 ) ) ;
#25765=CARTESIAN_POINT ( 'NONE',  ( 10.81189881249999729, 0.000000000000000000, -58.34375000204835970 ) ) ;
#25766=LINE ( 'NONE', #16015, #41261 ) ;
#25767=CARTESIAN_POINT ( 'NONE',  ( 10.81189881249999907, 6.242252689847868297, -173.7187500020484094 ) ) ;
#25770=DIRECTION ( 'NONE',  ( -1.000000000000000000, 0.000000000000000000, 0.000000000000000000 ) ) ;
#25772=CARTESIAN_POINT ( 'NONE',  ( 9.999999999999996447, -5.773502691896262640, -95.12499999999998579 ) ) ;
#25774=CARTESIAN_POINT ( 'NONE',  ( 7.644554776091147741E-16, 12.48450537969573659, -115.1562500020483952 ) ) ;
#25775=CARTESIAN_POINT ( 'NONE',  ( 4.999999999999992006, -8.660254037844389075, -137.6250000040967620 ) ) ;
#25776=CARTESIAN_POINT ( 'NONE',  ( 9.999999999999998224, 0.000000000000000000, -159.5000000000000000 ) ) ;
#25779=CARTESIAN_POINT ( 'NONE',  ( -5.000000000000003553, -8.660254037844383745, -160.0000000000000000 ) ) ;
#25780=CARTESIAN_POINT ( 'NONE',  ( -10.81189881249999729, 6.242252689847871849, -59.40625000204838813 ) ) ;
#25788=EDGE_LOOP ( 'NONE', ( #34668, #34778, #35653, #5146 ) ) ;
#25791=ORIENTED_EDGE ( 'NONE', *, *, #9853, .T. ) ;
#25792=ORIENTED_EDGE ( 'NONE', *, *, #2500, .F. ) ;
#25794=LINE ( 'NONE', #20304, #14144 ) ;
#25797=EDGE_LOOP ( 'NONE', ( #3024, #19965, #35461, #13328 ) ) ;
#25799=CARTESIAN_POINT ( 'NONE',  ( -10.00000000000000000, -5.773502691896251982, -28.12499999999998579 ) ) ;
#25802=CARTESIAN_POINT ( 'NONE',  ( 10.81189881249999907, 6.242252689847868297, -155.7187500020483810 ) ) ;
#25803=CARTESIAN_POINT ( 'NONE',  ( 7.644554776091147741E-16, 12.48450537969573659, -168.9687500020483810 ) ) ;
#25806=CARTESIAN_POINT ( 'NONE',  ( 7.070501591499377789E-16, 11.54700538379251284, -186.1250000000000000 ) ) ;
#25812=CARTESIAN_POINT ( 'NONE',  ( -5.405949406249996869, 9.363379034771805109, -64.03125000204836681 ) ) ;
#25814=CARTESIAN_POINT ( 'NONE',  ( -10.00000000000000000, -5.773502691896251982, -113.6249999999999858 ) ) ;
#25817=CARTESIAN_POINT ( 'NONE',  ( 10.81189881249999551, -6.242252689847874514, -139.6562500020484094 ) ) ;
#25818=CARTESIAN_POINT ( 'NONE',  ( 7.644554776091147741E-16, 12.48450537969573659, -154.1562500020484094 ) ) ;
#25820=CARTESIAN_POINT ( 'NONE',  ( 9.999999999999479527, 5.773502691896553074, -105.3749999999999716 ) ) ;
#25821=CARTESIAN_POINT ( 'NONE',  ( -10.81189881249999729, 1.324075727343319199E-15, -92.09375000204838102 ) ) ;
#25824=CARTESIAN_POINT ( 'NONE',  ( -10.81189881249999729, 1.324075727343319199E-15, -189.5937500020483810 ) ) ;
#25828=CARTESIAN_POINT ( 'NONE',  ( 5.405949406249992428, -9.363379034771808662, -85.78125000204838102 ) ) ;
#25830=CARTESIAN_POINT ( 'NONE',  ( 10.00000000000000000, 5.773502691896255534, -59.25000000409677625 ) ) ;
#25831=CARTESIAN_POINT ( 'NONE',  ( 5.405949406249992428, -9.363379034771808662, -16.59375000204835260 ) ) ;
#25834=CARTESIAN_POINT ( 'NONE',  ( 5.405949406249992428, -9.363379034771808662, -12.28125000204835438 ) ) ;
#25837=DIRECTION ( 'NONE',  ( -0.000000000000000000, -0.000000000000000000, -1.000000000000000000 ) ) ;
#25847=EDGE_CURVE ( 'NONE', #5096, #1917, #16039, .T. ) ;
#25853=DIRECTION ( 'NONE',  ( -0.000000000000000000, -0.000000000000000000, -1.000000000000000000 ) ) ;
#25854=CARTESIAN_POINT ( 'NONE',  ( 8.393774332151281214, 6.297795101496888925, -99.99999999999998579 ) ) ;
#25856=CARTESIAN_POINT ( 'NONE',  ( 0.000000000000000000, 0.000000000000000000, -99.99999999999998579 ) ) ;
#25857=CARTESIAN_POINT ( 'NONE',  ( 7.644554776091147741E-16, 12.48450537969573659, -158.6562500020484094 ) ) ;
#25863=CARTESIAN_POINT ( 'NONE',  ( 5.405949406249992428, -9.363379034771808662, -79.59375000204838102 ) ) ;
#25865=CARTESIAN_POINT ( 'NONE',  ( 7.644554776091147741E-16, 12.48450537969573659, -80.65625000204839523 ) ) ;
#25868=CARTESIAN_POINT ( 'NONE',  ( -5.405949406250003975, -9.363379034771801557, -168.5312500020484094 ) ) ;
#25869=CARTESIAN_POINT ( 'NONE',  ( 10.81189881249999729, 0.000000000000000000, -181.5312500020483810 ) ) ;
#25870=CARTESIAN_POINT ( 'NONE',  ( 10.00000000000000000, 5.773502691896255534, -152.2500000040967620 ) ) ;
#25872=CARTESIAN_POINT ( 'NONE',  ( -10.81189881249999729, 1.324075727343319199E-15, -8.093750002048343717 ) ) ;
#25873=CARTESIAN_POINT ( 'NONE',  ( 9.999999999999998224, 0.000000000000000000, -162.5000000000000000 ) ) ;
#25874=CARTESIAN_POINT ( 'NONE',  ( -5.405949406249996869, 9.363379034771805109, -113.3437500020483810 ) ) ;
#25877=CARTESIAN_POINT ( 'NONE',  ( -5.405949406249996869, 9.363379034771805109, -11.53125000204835438 ) ) ;
#25879=CARTESIAN_POINT ( 'NONE',  ( -2.121150477449813534E-15, -11.54700538379251284, -170.7500000040968189 ) ) ;
#25880=CARTESIAN_POINT ( 'NONE',  ( 10.81189881249999729, 0.000000000000000000, -106.5312500020483810 ) ) ;
#25884=CARTESIAN_POINT ( 'NONE',  ( -10.00000000000000000, -5.773502691896251982, -82.50000000409677625 ) ) ;
#25885=CARTESIAN_POINT ( 'NONE',  ( -10.81189881249999729, 1.324075727343319199E-15, -42.59375000204837391 ) ) ;
#25889=CARTESIAN_POINT ( 'NONE',  ( -2.121150477449813534E-15, -11.54700538379251284, -20.75000000409676915 ) ) ;
#25895=( BOUNDED_CURVE ( )  B_SPLINE_CURVE ( 2, ( #18930, #39201, #41587, #12019, #5988, #38565, #32324 ),
 .UNSPECIFIED., .F., .F. ) 
 B_SPLINE_CURVE_WITH_KNOTS ( ( 3, 2, 2, 3 ),
 ( 0.3059701492537313383, 0.3072139303482587791, 0.3084577114427861644, 0.3097014925373136052 ),
 .UNSPECIFIED. ) 
 CURVE ( )  GEOMETRIC_REPRESENTATION_ITEM ( )  RATIONAL_B_SPLINE_CURVE ( ( 1.000000000000000000, 0.8660254037844387076, 1.000000000000000000, 0.8660254037844387076, 1.000000000000000000, 0.8660254037844207220, 1.000000000000017986 ) ) 
 REPRESENTATION_ITEM ( '' )  );
#25899=ORIENTED_EDGE ( 'NONE', *, *, #35462, .T. ) ;
#25900=VERTEX_POINT ( 'NONE', #5030 ) ;
#25904=( BOUNDED_CURVE ( )  B_SPLINE_CURVE ( 2, ( #23418, #36359, #13879, #36781, #33136, #40218, #13247 ),
 .UNSPECIFIED., .F., .F. ) 
 B_SPLINE_CURVE_WITH_KNOTS ( ( 3, 2, 2, 3 ),
 ( 0.3059701492537313383, 0.3072139303482587791, 0.3084577114427861644, 0.3097014925373136052 ),
 .UNSPECIFIED. ) 
 CURVE ( )  GEOMETRIC_REPRESENTATION_ITEM ( )  RATIONAL_B_SPLINE_CURVE ( ( 1.000000000000000000, 0.8660254037844387076, 1.000000000000000000, 0.8660254037844387076, 1.000000000000000000, 0.8660254037844207220, 1.000000000000017986 ) ) 
 REPRESENTATION_ITEM ( '' )  );
#25905=CARTESIAN_POINT ( 'NONE',  ( 5.405949406249992428, -9.363379034771808662, -183.2812500020484094 ) ) ;
#25909=CARTESIAN_POINT ( 'NONE',  ( -2.293366432827344421E-15, -12.48450537969573659, -100.7187500020483952 ) ) ;
#25911=CARTESIAN_POINT ( 'NONE',  ( -10.81189881249999729, 6.242252689847871849, -105.9062500020483810 ) ) ;
#25913=CARTESIAN_POINT ( 'NONE',  ( 7.644554776091147741E-16, 12.48450537969573659, -110.4687500020483668 ) ) ;
#25916=CARTESIAN_POINT ( 'NONE',  ( 9.999999999999998224, 0.000000000000000000, -143.0000000000000000 ) ) ;
#25917=CARTESIAN_POINT ( 'NONE',  ( -9.999999999999998224, 1.224646799147353059E-15, -5.749999999999976907 ) ) ;
#25921=CARTESIAN_POINT ( 'NONE',  ( -2.121150477449813534E-15, -11.54700538379251284, -176.7500000040967620 ) ) ;
#25923=CARTESIAN_POINT ( 'NONE',  ( 5.405949406249999534, 9.363379034771803333, -32.59375000204836681 ) ) ;
#25925=CARTESIAN_POINT ( 'NONE',  ( 5.405949406249999534, 9.363379034771803333, -134.5937500020483810 ) ) ;
#25931=CARTESIAN_POINT ( 'NONE',  ( 10.00000000000000000, 5.773502691896255534, -66.37499999999998579 ) ) ;
#25932=CARTESIAN_POINT ( 'NONE',  ( -10.81189881249999907, -6.242252689847864744, -135.6562500020484094 ) ) ;
#25935=CARTESIAN_POINT ( 'NONE',  ( -4.999999999999996447, 8.660254037844387298, -120.3750000040967905 ) ) ;
#25936=CARTESIAN_POINT ( 'NONE',  ( 9.999999999999996447, -5.773502691896262640, -104.5000000040967763 ) ) ;
#25938=CARTESIAN_POINT ( 'NONE',  ( 10.81189881249999551, -6.242252689847874514, -64.46875000204838102 ) ) ;
#25944=CARTESIAN_POINT ( 'NONE',  ( -9.999999999999998224, 1.224646799147353059E-15, -45.12500000409677625 ) ) ;
#25945=CARTESIAN_POINT ( 'NONE',  ( -10.81189881249999729, 6.242252689847871849, -32.40625000204835970 ) ) ;
#25956=CARTESIAN_POINT ( 'NONE',  ( 10.00000000000102318, -5.773502691895667560, -104.1249999999999432 ) ) ;
#25963=CARTESIAN_POINT ( 'NONE',  ( 10.81189881249999729, 0.000000000000000000, -124.3437500020483952 ) ) ;
#25964=CARTESIAN_POINT ( 'NONE',  ( -10.81189881249999729, 1.324075727343319199E-15, -131.2812500020483810 ) ) ;
#25966=CARTESIAN_POINT ( 'NONE',  ( -10.81189881249999729, -6.242252689847864744, -147.4687500020484094 ) ) ;
#25967=CARTESIAN_POINT ( 'NONE',  ( 9.046166897582494926, -5.964473731795716382, -179.9999999999999716 ) ) ;
#25969=CARTESIAN_POINT ( 'NONE',  ( 9.999999999999996447, -5.773502691896262640, -162.6250000000000284 ) ) ;
#25970=CARTESIAN_POINT ( 'NONE',  ( 10.81189881249999907, 6.242252689847868297, 0.09374999795164208616 ) ) ;
#25973=CARTESIAN_POINT ( 'NONE',  ( 5.405949406249999534, 9.363379034771803333, -52.09375000204835260 ) ) ;
#25974=FACE_OUTER_BOUND ( 'NONE', #37565, .T. ) ;
#25975=CARTESIAN_POINT ( 'NONE',  ( 5.405949406249999534, 9.363379034771803333, -158.5937500020483810 ) ) ;
#25978=CYLINDRICAL_SURFACE ( 'NONE', #1372, 9.999999999999998224 ) ;
#25980=CARTESIAN_POINT ( 'NONE',  ( 4.999999999999992006, -8.660254037844389075, -93.74999999999998579 ) ) ;
#25982=ORIENTED_EDGE ( 'NONE', *, *, #18927, .F. ) ;
#25983=CARTESIAN_POINT ( 'NONE',  ( -10.81189881249999729, 1.324075727343319199E-15, -117.7812500020483952 ) ) ;
#25984=CARTESIAN_POINT ( 'NONE',  ( -2.121150477449813534E-15, -11.54700538379251284, -137.7500000040967905 ) ) ;
#25991=CARTESIAN_POINT ( 'NONE',  ( -10.81189881249999729, 1.324075727343319199E-15, -59.28125000204836681 ) ) ;
#25998=VERTEX_POINT ( 'NONE', #32007 ) ;
#26001=ORIENTED_EDGE ( 'NONE', *, *, #34409, .F. ) ;
#26010=CARTESIAN_POINT ( 'NONE',  ( 7.070501591499377789E-16, 11.54700538379251284, -31.62499999999995737 ) ) ;
#26013=CARTESIAN_POINT ( 'NONE',  ( 7.644554776091147741E-16, 12.48450537969573659, -149.4687500020484094 ) ) ;
#26014=CARTESIAN_POINT ( 'NONE',  ( 10.81189881249999729, 0.000000000000000000, -172.3437500020484094 ) ) ;
#26017=CARTESIAN_POINT ( 'NONE',  ( 5.000000000000000000, 8.660254037844385522, -190.7500000000000000 ) ) ;
#26021=DIRECTION ( 'NONE',  ( -0.000000000000000000, -0.000000000000000000, -1.000000000000000000 ) ) ;
#26022=CARTESIAN_POINT ( 'NONE',  ( -5.405949406250003975, -9.363379034771801557, -186.3437500020483810 ) ) ;
#26024=CARTESIAN_POINT ( 'NONE',  ( -10.81189881249999729, 6.242252689847871849, -57.90625000204838813 ) ) ;
#26026=CARTESIAN_POINT ( 'NONE',  ( 4.999999999999992006, -8.660254037844389075, -116.2499999999999858 ) ) ;
#26027=( BOUNDED_CURVE ( )  B_SPLINE_CURVE ( 2, ( #27600, #10381, #37306, #5153, #18304, #11394, #34081 ),
 .UNSPECIFIED., .F., .F. ) 
 B_SPLINE_CURVE_WITH_KNOTS ( ( 3, 2, 2, 3 ),
 ( 0.2089552238805970630, 0.2101990049751244205, 0.2114427860696518058, 0.2126865671641791633 ),
 .UNSPECIFIED. ) 
 CURVE ( )  GEOMETRIC_REPRESENTATION_ITEM ( )  RATIONAL_B_SPLINE_CURVE ( ( 0.9999999999999940048, 0.8660254037844447028, 1.000000000000000000, 0.8660254037844387076, 1.000000000000000000, 0.8660254037844327124, 1.000000000000005995 ) ) 
 REPRESENTATION_ITEM ( '' )  );
#26029=CARTESIAN_POINT ( 'NONE',  ( -5.405949406249996869, 9.363379034771805109, -145.0312500020483810 ) ) ;
#26030=CARTESIAN_POINT ( 'NONE',  ( -5.405949406250003975, -9.363379034771801557, -159.5312500020484094 ) ) ;
#26033=CARTESIAN_POINT ( 'NONE',  ( -10.81189881249999729, 6.242252689847871849, -87.71875000204838102 ) ) ;
#26034=VECTOR ( 'NONE', #38380, 1000.000000000000000 ) ;
#26037=CARTESIAN_POINT ( 'NONE',  ( -5.405949406249996869, 9.363379034771805109, -189.8437500020483810 ) ) ;
#26039=CARTESIAN_POINT ( 'NONE',  ( -2.121150477449813534E-15, -11.54700538379251284, -169.2500000040968189 ) ) ;
#26041=CARTESIAN_POINT ( 'NONE',  ( -5.405949406249996869, 9.363379034771805109, -88.03125000204838102 ) ) ;
#26043=CARTESIAN_POINT ( 'NONE',  ( -4.999999999999996447, 8.660254037844387298, -57.37500000409676204 ) ) ;
#26044=CARTESIAN_POINT ( 'NONE',  ( 7.644554776091147741E-16, 12.48450537969573659, -20.46875000204837036 ) ) ;
#26048=CARTESIAN_POINT ( 'NONE',  ( 10.81189881249999907, 6.242252689847868297, -13.40625000204837036 ) ) ;
#26054=CARTESIAN_POINT ( 'NONE',  ( 9.999999999999998224, 0.000000000000000000, -114.4999999999999858 ) ) ;
#26060=EDGE_CURVE ( 'NONE', #12598, #12994, #320, .T. ) ;
#26070=CARTESIAN_POINT ( 'NONE',  ( 10.81189881249999551, -6.242252689847874514, -157.6562500020484094 ) ) ;
#26076=CARTESIAN_POINT ( 'NONE',  ( -10.81189881249999729, 1.324075727343319199E-15, -80.09375000204838102 ) ) ;
#26077=CARTESIAN_POINT ( 'NONE',  ( 5.405949406249999534, 9.363379034771803333, -82.28125000204838102 ) ) ;
#26080=CARTESIAN_POINT ( 'NONE',  ( -5.405949406250003975, -9.363379034771801557, -164.0312500020484094 ) ) ;
#26081=CARTESIAN_POINT ( 'NONE',  ( 7.644554776091147741E-16, 12.48450537969573659, -181.1562500020484094 ) ) ;
#26082=CARTESIAN_POINT ( 'NONE',  ( 4.999999999999992006, -8.660254037844389075, -157.1250000040967905 ) ) ;
#26083=FACE_OUTER_BOUND ( 'NONE', #11174, .T. ) ;
#26084=CARTESIAN_POINT ( 'NONE',  ( 10.81189881249999907, 6.242252689847868297, -7.218750002048357040 ) ) ;
#26086=CARTESIAN_POINT ( 'NONE',  ( 7.644554776091147741E-16, 12.48450537969573659, -116.4687500020483952 ) ) ;
#26088=CARTESIAN_POINT ( 'NONE',  ( 7.644554776091147741E-16, 12.48450537969573659, -14.65625000204837214 ) ) ;
#26090=CARTESIAN_POINT ( 'NONE',  ( 4.999999999999992006, -8.660254037844389075, -170.6250000040968189 ) ) ;
#26091=CARTESIAN_POINT ( 'NONE',  ( 5.405949406249999534, 9.363379034771803333, -106.2812500020483810 ) ) ;
#26094=EDGE_CURVE ( 'NONE', #1002, #31616, #22920, .T. ) ;
#26095=CARTESIAN_POINT ( 'NONE',  ( 4.999999999999992006, -8.660254037844389075, -85.12500000409677625 ) ) ;
#26096=CARTESIAN_POINT ( 'NONE',  ( 9.999999999999998224, 1.224646799147353059E-15, -99.99999999999998579 ) ) ;
#26097=CARTESIAN_POINT ( 'NONE',  ( 5.405949406249999534, 9.363379034771803333, -41.59375000204837391 ) ) ;
#26101=CARTESIAN_POINT ( 'NONE',  ( -9.999999999999998224, 5.773502691896259087, -15.25000000409676382 ) ) ;
#26106=EDGE_CURVE ( 'NONE', #36911, #17741, #39996, .T. ) ;
#26113=CARTESIAN_POINT ( 'NONE',  ( 10.81189881249999907, 6.242252689847868297, -178.4062500020484094 ) ) ;
#26117=AXIS2_PLACEMENT_3D ( 'NONE', #13991, #459, #3896 ) ;
#26118=CARTESIAN_POINT ( 'NONE',  ( -10.81189881249999729, 1.324075727343319199E-15, -105.5937500020483810 ) ) ;
#26120=CARTESIAN_POINT ( 'NONE',  ( 5.405949406249999534, 9.363379034771803333, -107.7812500020483810 ) ) ;
#26122=CARTESIAN_POINT ( 'NONE',  ( 10.81189881249999729, 6.242252689847867408, -113.7187500020483952 ) ) ;
#26125=CARTESIAN_POINT ( 'NONE',  ( 9.999999999999996447, -5.773502691896262640, -138.6250000000000000 ) ) ;
#26126=CARTESIAN_POINT ( 'NONE',  ( 9.999999999999998224, 0.000000000000000000, -3.499999999999975131 ) ) ;
#26128=AXIS2_PLACEMENT_3D ( 'NONE', #39947, #11232, #30477 ) ;
#26131=CARTESIAN_POINT ( 'NONE',  ( 9.999999999999996447, -5.773502691896262640, -182.5000000040968189 ) ) ;
#26133=CARTESIAN_POINT ( 'NONE',  ( -10.81189881249999729, 1.324075727343319199E-15, -26.09375000204835970 ) ) ;
#26134=CARTESIAN_POINT ( 'NONE',  ( 9.999999999999742428, 5.773502691896404748, -117.3749999999999716 ) ) ;
#26135=CARTESIAN_POINT ( 'NONE',  ( 10.81189881249999551, -6.242252689847874514, -136.4687500020483810 ) ) ;
#26138=CARTESIAN_POINT ( 'NONE',  ( -4.999999999999996447, 8.660254037844387298, -68.99999999999997158 ) ) ;
#26139=CARTESIAN_POINT ( 'NONE',  ( -5.405949406249996869, 9.363379034771805109, -136.0312500020484094 ) ) ;
#26143=CARTESIAN_POINT ( 'NONE',  ( -4.999999999999996447, 8.660254037844387298, -109.8750000040967763 ) ) ;
#26145=CARTESIAN_POINT ( 'NONE',  ( 10.81189881249999729, 0.000000000000000000, -67.34375000204836681 ) ) ;
#26146=ORIENTED_EDGE ( 'NONE', *, *, #5364, .F. ) ;
#26151=CARTESIAN_POINT ( 'NONE',  ( 9.999999999999998224, 0.000000000000000000, -33.87500000409676915 ) ) ;
#26152=CARTESIAN_POINT ( 'NONE',  ( 5.405949406249992428, -9.363379034771808662, -39.28125000204838102 ) ) ;
#26158=ORIENTED_EDGE ( 'NONE', *, *, #39645, .T. ) ;
#26160=ORIENTED_EDGE ( 'NONE', *, *, #26481, .T. ) ;
#26161=EDGE_CURVE ( 'NONE', #6469, #25139, #31213, .T. ) ;
#26168=CARTESIAN_POINT ( 'NONE',  ( -9.999999999999998224, 0.000000000000000000, -99.99999999999998579 ) ) ;
#26172=CARTESIAN_POINT ( 'NONE',  ( 7.644554776091147741E-16, 12.48450537969573659, -128.4687500020483810 ) ) ;
#26173=CARTESIAN_POINT ( 'NONE',  ( 10.81189881249999551, -6.242252689847874514, -132.1562500020484094 ) ) ;
#26175=CARTESIAN_POINT ( 'NONE',  ( -5.405949406250003975, -9.363379034771801557, -141.3437500020483810 ) ) ;
#26178=CARTESIAN_POINT ( 'NONE',  ( 9.999999999999998224, 0.000000000000000000, -159.5000000000000000 ) ) ;
#26179=CARTESIAN_POINT ( 'NONE',  ( 5.405949406249999534, 9.363379034771803333, 0.2187499979516283055 ) ) ;
#26182=CARTESIAN_POINT ( 'NONE',  ( -2.293366432827344421E-15, -12.48450537969573659, -55.71875000204837391 ) ) ;
#26183=CARTESIAN_POINT ( 'NONE',  ( -9.999999999999998224, 1.224646799147353059E-15, -175.2500000000000284 ) ) ;
#26184=CARTESIAN_POINT ( 'NONE',  ( 10.81189881249999729, 0.000000000000000000, -164.8437500020484094 ) ) ;
#26187=CYLINDRICAL_SURFACE ( 'NONE', #10693, 9.999999999999998224 ) ;
#26189=CARTESIAN_POINT ( 'NONE',  ( -10.00000000000000000, -5.773502691896251982, -88.12499999999998579 ) ) ;
#26191=CARTESIAN_POINT ( 'NONE',  ( -10.81189881249999729, -6.242252689847864744, -120.6562500020483810 ) ) ;
#26192=CARTESIAN_POINT ( 'NONE',  ( -9.999999999999998224, 1.224646799147353059E-15, -130.6250000040967620 ) ) ;
#26197=CARTESIAN_POINT ( 'NONE',  ( 10.81189881249999729, 0.000000000000000000, -63.03125000204837391 ) ) ;
#26210=ORIENTED_EDGE ( 'NONE', *, *, #27661, .T. ) ;
#26215=AXIS2_PLACEMENT_3D ( 'NONE', #11172, #24369, #37511 ) ;
#26219=CARTESIAN_POINT ( 'NONE',  ( 4.999999999999992006, -8.660254037844389075, -26.24999999999996803 ) ) ;
#26223=CARTESIAN_POINT ( 'NONE',  ( -5.405949406249996869, 9.363379034771805109, -149.3437500020483810 ) ) ;
#26224=CARTESIAN_POINT ( 'NONE',  ( -10.81189881249999729, 1.324075727343319199E-15, -165.5937500020484094 ) ) ;
#26227=CARTESIAN_POINT ( 'NONE',  ( 9.999999999999996447, -5.773502691896262640, -185.1250000000000284 ) ) ;
#26232=CARTESIAN_POINT ( 'NONE',  ( -5.405949406250003975, -9.363379034771801557, -189.3437500020483810 ) ) ;
#26234=( BOUNDED_CURVE ( )  B_SPLINE_CURVE ( 2, ( #38896, #9325, #18178, #14932, #41263, #8702, #28130 ),
 .UNSPECIFIED., .F., .F. ) 
 B_SPLINE_CURVE_WITH_KNOTS ( ( 3, 2, 2, 3 ),
 ( 0.3917910447761194792, 0.3930348258706468090, 0.3942786069651742498, 0.3955223880597015795 ),
 .UNSPECIFIED. ) 
 CURVE ( )  GEOMETRIC_REPRESENTATION_ITEM ( )  RATIONAL_B_SPLINE_CURVE ( ( 0.9999999999999940048, 0.8660254037844447028, 1.000000000000000000, 0.8660254037844387076, 1.000000000000000000, 0.8660254037844267172, 1.000000000000011990 ) ) 
 REPRESENTATION_ITEM ( '' )  );
#26235=CARTESIAN_POINT ( 'NONE',  ( -5.405949406250003975, -9.363379034771801557, -60.53125000204836681 ) ) ;
#26237=CARTESIAN_POINT ( 'NONE',  ( 10.00000000000000000, 5.773502691896255534, -112.8749999999999858 ) ) ;
#26238=ORIENTED_EDGE ( 'NONE', *, *, #1695, .T. ) ;
#26239=CARTESIAN_POINT ( 'NONE',  ( -10.81189881249999729, 1.324075727343319199E-15, -143.2812500020483810 ) ) ;
#26240=CARTESIAN_POINT ( 'NONE',  ( -5.405949406250003975, -9.363379034771801557, -155.0312500020484094 ) ) ;
#26244=CARTESIAN_POINT ( 'NONE',  ( -2.293366432827344421E-15, -12.48450537969573659, -88.71875000204838102 ) ) ;
#26247=CARTESIAN_POINT ( 'NONE',  ( 10.81189881249999551, -6.242252689847874514, -185.9687500020484094 ) ) ;
#26249=CARTESIAN_POINT ( 'NONE',  ( -5.000000000000003553, -8.660254037844383745, -116.8750000040967905 ) ) ;
#26250=CARTESIAN_POINT ( 'NONE',  ( 10.81189881249999551, -6.242252689847874514, -85.65625000204838102 ) ) ;
#26252=CARTESIAN_POINT ( 'NONE',  ( -9.999999999999998224, 1.224646799147353059E-15, -57.12500000409676204 ) ) ;
#26254=CARTESIAN_POINT ( 'NONE',  ( 5.405949406249992428, -9.363379034771808662, -19.59375000204835615 ) ) ;
#26258=CARTESIAN_POINT ( 'NONE',  ( -10.81189881249999729, 6.242252689847871849, -14.40625000204837036 ) ) ;
#26261=CARTESIAN_POINT ( 'NONE',  ( 9.999999999999479527, 5.773502691896553074, -114.7500000040967620 ) ) ;
#26268=CARTESIAN_POINT ( 'NONE',  ( 10.81189881249999729, 0.000000000000000000, -103.3437500020483668 ) ) ;
#26270=ORIENTED_EDGE ( 'NONE', *, *, #28598, .T. ) ;
#26280=FACE_OUTER_BOUND ( 'NONE', #8541, .T. ) ;
#26281=CARTESIAN_POINT ( 'NONE',  ( 5.405949406249992428, -9.363379034771808662, -156.2812500020484094 ) ) ;
#26289=CARTESIAN_POINT ( 'NONE',  ( -5.405949406249996869, 9.363379034771805109, -74.34375000204838102 ) ) ;
#26290=CARTESIAN_POINT ( 'NONE',  ( 5.405949406249999534, 9.363379034771803333, -85.28125000204838102 ) ) ;
#26294=CARTESIAN_POINT ( 'NONE',  ( -10.81189881249999729, 6.242252689847871849, -164.4062500020483810 ) ) ;
#26295=CARTESIAN_POINT ( 'NONE',  ( -10.81189881249999729, 1.324075727343319199E-15, -182.2812500020483810 ) ) ;
#26296=CARTESIAN_POINT ( 'NONE',  ( 5.000000000000000000, 8.660254037844385522, -159.6250000040967905 ) ) ;
#26298=CARTESIAN_POINT ( 'NONE',  ( -5.405949406250003975, -9.363379034771801557, -6.343750002048370362 ) ) ;
#26300=CARTESIAN_POINT ( 'NONE',  ( 10.81189881249999729, 0.000000000000000000, -112.3437500020483810 ) ) ;
#26302=CARTESIAN_POINT ( 'NONE',  ( 10.81189881249999551, -6.242252689847874514, -10.65625000204836859 ) ) ;
#26305=CARTESIAN_POINT ( 'NONE',  ( 10.81189881249999729, 0.000000000000000000, -105.0312500020483810 ) ) ;
#26308=CARTESIAN_POINT ( 'NONE',  ( 7.070501591499377789E-16, 11.54700538379251284, -83.00000000409677625 ) ) ;
#26310=CARTESIAN_POINT ( 'NONE',  ( -2.293366432827344421E-15, -12.48450537969573659, -40.71875000204835970 ) ) ;
#26314=CARTESIAN_POINT ( 'NONE',  ( -10.00000000000000000, -5.773502691896251982, -10.50000000409675849 ) ) ;
#26320=ORIENTED_EDGE ( 'NONE', *, *, #15086, .T. ) ;
#26325=ORIENTED_EDGE ( 'NONE', *, *, #25109, .F. ) ;
#26328=CARTESIAN_POINT ( 'NONE',  ( -10.81189881249999907, -6.242252689847864744, -182.1562500020483810 ) ) ;
#26332=CARTESIAN_POINT ( 'NONE',  ( 7.644554776091147741E-16, 12.48450537969573659, -101.4687500020483668 ) ) ;
#26333=CARTESIAN_POINT ( 'NONE',  ( 10.81189881249999551, -6.242252689847874514, -108.1562500020483810 ) ) ;
#26335=CARTESIAN_POINT ( 'NONE',  ( 10.81189881249999729, 0.000000000000000000, -118.3437500020483810 ) ) ;
#26339=CARTESIAN_POINT ( 'NONE',  ( -9.999999999999998224, 1.224646799147353059E-15, -139.2499999999999716 ) ) ;
#26340=CARTESIAN_POINT ( 'NONE',  ( 4.999999999999992006, -8.660254037844389075, -5.249999999999976907 ) ) ;
#26343=CARTESIAN_POINT ( 'NONE',  ( -5.000000000000003553, -8.660254037844383745, -181.3750000040967905 ) ) ;
#26345=CARTESIAN_POINT ( 'NONE',  ( -2.293366432827344421E-15, -12.48450537969573659, -28.71875000204834905 ) ) ;
#26346=CARTESIAN_POINT ( 'NONE',  ( -2.293366432827344421E-15, -12.48450537969573659, -139.7187500020483810 ) ) ;
#26348=CARTESIAN_POINT ( 'NONE',  ( 10.81189881249999907, 6.242252689847868297, -34.40625000204835970 ) ) ;
#26350=CARTESIAN_POINT ( 'NONE',  ( 9.999999999999996447, -5.773502691896262640, -71.12499999999998579 ) ) ;
#26351=CARTESIAN_POINT ( 'NONE',  ( 10.81189881249999729, 0.000000000000000000, -132.0312500020484094 ) ) ;
#26355=CARTESIAN_POINT ( 'NONE',  ( 9.999999999999998224, 0.000000000000000000, -128.0000000000000000 ) ) ;
#26356=CARTESIAN_POINT ( 'NONE',  ( 4.999999999999992006, -8.660254037844389075, -110.6250000040967763 ) ) ;
#26357=CARTESIAN_POINT ( 'NONE',  ( -9.999999999999998224, 1.224646799147353059E-15, -103.6250000040967763 ) ) ;
#26358=CARTESIAN_POINT ( 'NONE',  ( -5.405949406250003975, -9.363379034771801557, -64.84375000204836681 ) ) ;
#26365=CARTESIAN_POINT ( 'NONE',  ( 7.070501591499377789E-16, 11.54700538379251284, -35.00000000409675494 ) ) ;
#26371=ORIENTED_EDGE ( 'NONE', *, *, #18927, .T. ) ;
#26376=VECTOR ( 'NONE', #22743, 1000.000000000000000 ) ;
#26381=CYLINDRICAL_SURFACE ( 'NONE', #16210, 9.999999999999998224 ) ;
#26382=CARTESIAN_POINT ( 'NONE',  ( 10.81189881249999729, 0.000000000000000000, -128.8437500020484094 ) ) ;
#26383=CARTESIAN_POINT ( 'NONE',  ( 10.81189881249999729, 0.000000000000000000, -133.5312500020484094 ) ) ;
#26385=CARTESIAN_POINT ( 'NONE',  ( -10.81189881249999729, 6.242252689847871849, -141.7187500020483810 ) ) ;
#26386=CYLINDRICAL_SURFACE ( 'NONE', #27443, 9.999999999999998224 ) ;
#26388=CARTESIAN_POINT ( 'NONE',  ( 9.999999999999998224, 0.000000000000000000, -161.0000000000000000 ) ) ;
#26392=CARTESIAN_POINT ( 'NONE',  ( -5.405949406250003975, -9.363379034771801557, -54.34375000204835970 ) ) ;
#26393=CARTESIAN_POINT ( 'NONE',  ( -10.00000000000012790, -5.773502691896178263, -175.1250000000000284 ) ) ;
#26394=CARTESIAN_POINT ( 'NONE',  ( -10.81189881249999729, 1.324075727343319199E-15, -164.0937500020484094 ) ) ;
#26399=CARTESIAN_POINT ( 'NONE',  ( -9.999999999999998224, 5.773502691896259087, -91.37499999999998579 ) ) ;
#26402=CARTESIAN_POINT ( 'NONE',  ( 10.81189881249999729, 6.242252689847867408, -113.9062500020483952 ) ) ;
#26403=CARTESIAN_POINT ( 'NONE',  ( 9.999999999999996447, -5.773502691896262640, -130.0000000040967905 ) ) ;
#26404=CARTESIAN_POINT ( 'NONE',  ( 10.00000000000076916, -5.773502691895816774, -111.6249999999999716 ) ) ;
#26409=CARTESIAN_POINT ( 'NONE',  ( 7.644554776091147741E-16, 12.48450537969573659, -56.65625000204838813 ) ) ;
#26419=EDGE_LOOP ( 'NONE', ( #11487, #37297, #26627, #31483 ) ) ;
#26425=CARTESIAN_POINT ( 'NONE',  ( -9.999999999999998224, 5.773502691896259087, -25.37499999999998224 ) ) ;
#26428=CARTESIAN_POINT ( 'NONE',  ( 10.81189881249999907, 6.242252689847868297, -152.7187500020483810 ) ) ;
#26429=CARTESIAN_POINT ( 'NONE',  ( -5.405949406250003975, -9.363379034771801557, -165.3437500020484094 ) ) ;
#26430=CARTESIAN_POINT ( 'NONE',  ( 7.070501591499376803E-16, 11.54700538379251284, -107.0000000040967763 ) ) ;
#26431=CARTESIAN_POINT ( 'NONE',  ( 0.000000000000000000, 0.000000000000000000, -99.99999999999998579 ) ) ;
#26432=CARTESIAN_POINT ( 'NONE',  ( 7.070501591499377789E-16, 11.54700538379251284, -190.6250000000000000 ) ) ;
#26436=CYLINDRICAL_SURFACE ( 'NONE', #29547, 9.999999999999998224 ) ;
#26437=CARTESIAN_POINT ( 'NONE',  ( -10.81189881249999907, -6.242252689847864744, -187.9687500020484094 ) ) ;
#26440=CARTESIAN_POINT ( 'NONE',  ( -2.293366432827344421E-15, -12.48450537969573659, -49.90625000204838102 ) ) ;
#26442=CARTESIAN_POINT ( 'NONE',  ( 9.999999999999996447, -5.773502691896262640, -116.1250000000000000 ) ) ;
#26443=ORIENTED_EDGE ( 'NONE', *, *, #24570, .F. ) ;
#26444=CARTESIAN_POINT ( 'NONE',  ( 5.405949406249999534, 9.363379034771803333, -137.7812500020483810 ) ) ;
#26445=CARTESIAN_POINT ( 'NONE',  ( 10.81189881249999907, 6.242252689847868297, -158.9062500020483810 ) ) ;
#26448=CARTESIAN_POINT ( 'NONE',  ( -10.81189881249999907, -6.242252689847864744, -78.46875000204838102 ) ) ;
#26449=ORIENTED_EDGE ( 'NONE', *, *, #11181, .F. ) ;
#26451=CARTESIAN_POINT ( 'NONE',  ( 7.644554776091147741E-16, 12.48450537969573659, -185.4687500020483810 ) ) ;
#26454=CARTESIAN_POINT ( 'NONE',  ( 9.999999999999872102, 5.773502691896329253, -165.3750000000000000 ) ) ;
#26455=CARTESIAN_POINT ( 'NONE',  ( 9.999999999999479527, 5.773502691896553074, -140.2500000040967620 ) ) ;
#26456=EDGE_CURVE ( 'NONE', #21319, #23753, #19335, .T. ) ;
#26457=CARTESIAN_POINT ( 'NONE',  ( -10.81189881249999729, 6.242252689847871849, -81.90625000204838102 ) ) ;
#26460=CARTESIAN_POINT ( 'NONE',  ( -9.999999999999998224, 5.773502691896259087, -61.75000000409678336 ) ) ;
#26461=CARTESIAN_POINT ( 'NONE',  ( 10.81189881249999729, 0.000000000000000000, -16.34375000204835260 ) ) ;
#26464=CARTESIAN_POINT ( 'NONE',  ( -10.81189881249999729, 6.242252689847871849, -12.90625000204836859 ) ) ;
#26474=ADVANCED_FACE ( 'NONE', ( #6720 ), #33487, .F. ) ;
#26477=ORIENTED_EDGE ( 'NONE', *, *, #34924, .T. ) ;
#26481=EDGE_CURVE ( 'NONE', #24722, #270, #17047, .T. ) ;
#26489=CARTESIAN_POINT ( 'NONE',  ( 10.81189881249999729, 0.000000000000000000, -147.0312500020483810 ) ) ;
#26496=ADVANCED_FACE ( 'NONE', ( #40778 ), #11219, .F. ) ;
#26497=CARTESIAN_POINT ( 'NONE',  ( -10.81189881249999729, 6.242252689847871849, -74.21875000204836681 ) ) ;
#26498=CARTESIAN_POINT ( 'NONE',  ( 10.81189881249999729, 0.000000000000000000, -85.53125000204838102 ) ) ;
#26500=CARTESIAN_POINT ( 'NONE',  ( -5.405949406250003975, -9.363379034771801557, -162.5312500020484094 ) ) ;
#26501=CARTESIAN_POINT ( 'NONE',  ( -2.293366432827344421E-15, -12.48450537969573659, -183.4062500020483810 ) ) ;
#26502=CARTESIAN_POINT ( 'NONE',  ( -10.00000000000000000, -5.773502691896251982, -157.5000000040968189 ) ) ;
#26504=CARTESIAN_POINT ( 'NONE',  ( -2.293366432827344421E-15, -12.48450537969573659, -6.218750002048356151 ) ) ;
#26506=CARTESIAN_POINT ( 'NONE',  ( 5.405949406249992428, -9.363379034771808662, -115.5937500020483810 ) ) ;
#26508=CARTESIAN_POINT ( 'NONE',  ( -10.81189881249999729, 1.324075727343319199E-15, -15.78125000204835793 ) ) ;
#26510=FACE_OUTER_BOUND ( 'NONE', #7364, .T. ) ;
#26511=CARTESIAN_POINT ( 'NONE',  ( 5.405949406249992428, -9.363379034771808662, -109.7812500020483810 ) ) ;
#26515=CARTESIAN_POINT ( 'NONE',  ( 5.000000000000000000, 8.660254037844385522, -86.12500000409677625 ) ) ;
#26516=CARTESIAN_POINT ( 'NONE',  ( 7.070501591499376803E-16, 11.54700538379251284, -146.0000000040967905 ) ) ;
#26517=CARTESIAN_POINT ( 'NONE',  ( -10.81189881249999729, 6.242252689847871849, -39.71875000204835970 ) ) ;
#26522=CARTESIAN_POINT ( 'NONE',  ( 10.00000000000000000, 5.773502691896255534, -8.250000004096758488 ) ) ;
#26528=VERTEX_POINT ( 'NONE', #17473 ) ;
#26539=CARTESIAN_POINT ( 'NONE',  ( -10.81189881249999729, 1.324075727343319199E-15, -183.7812500020484094 ) ) ;
#26542=CARTESIAN_POINT ( 'NONE',  ( 10.81189881249999907, 6.242252689847868297, -98.71875000204838102 ) ) ;
#26544=CARTESIAN_POINT ( 'NONE',  ( 5.405949406249992428, -9.363379034771808662, -106.7812500020483810 ) ) ;
#26546=CARTESIAN_POINT ( 'NONE',  ( -2.293366432827344421E-15, -12.48450537969573659, -111.2187500020483668 ) ) ;
#26550=CARTESIAN_POINT ( 'NONE',  ( 0.6423023231492728247, 10.81644720607814314, -99.99999999999997158 ) ) ;
#26551=CARTESIAN_POINT ( 'NONE',  ( -2.121150477449813534E-15, -11.54700538379251284, -128.3750000000000000 ) ) ;
#26552=CARTESIAN_POINT ( 'NONE',  ( -4.999999999999996447, 8.660254037844387298, -5.999999999999977796 ) ) ;
#26555=CARTESIAN_POINT ( 'NONE',  ( -9.999999999999998224, 1.224646799147353059E-15, -181.6250000040967905 ) ) ;
#26557=CARTESIAN_POINT ( 'NONE',  ( 10.81189881249999729, 0.000000000000000000, -32.84375000204836681 ) ) ;
#26558=CARTESIAN_POINT ( 'NONE',  ( 9.999999999999998224, 1.224646799147353059E-15, -99.99999999999998579 ) ) ;
#26559=CARTESIAN_POINT ( 'NONE',  ( 10.81189881249999729, 0.000000000000000000, -137.8437500020484094 ) ) ;
#26561=CARTESIAN_POINT ( 'NONE',  ( 5.405949406249999534, 9.363379034771803333, -32.78125000204837391 ) ) ;
#26563=CARTESIAN_POINT ( 'NONE',  ( 5.000000000000000000, 8.660254037844385522, -60.24999999999997158 ) ) ;
#26564=CARTESIAN_POINT ( 'NONE',  ( 10.81189881249999907, 6.242252689847868297, -133.4062500020483810 ) ) ;
#26566=ORIENTED_EDGE ( 'NONE', *, *, #18720, .T. ) ;
#26568=CARTESIAN_POINT ( 'NONE',  ( 7.070501591499377789E-16, 11.54700538379251284, -111.5000000040967763 ) ) ;
#26569=CARTESIAN_POINT ( 'NONE',  ( 9.999999999999998224, 0.000000000000000000, -146.0000000000000000 ) ) ;
#26570=CARTESIAN_POINT ( 'NONE',  ( -10.81189881249999729, 6.242252689847871849, -65.21875000204838102 ) ) ;
#26571=ORIENTED_EDGE ( 'NONE', *, *, #8956, .F. ) ;
#26576=CARTESIAN_POINT ( 'NONE',  ( 9.999999999999996447, -5.773502691896262640, -34.00000000409675494 ) ) ;
#26579=CARTESIAN_POINT ( 'NONE',  ( -4.999999999999996447, 8.660254037844387298, -121.8750000040967905 ) ) ;
#26581=ORIENTED_EDGE ( 'NONE', *, *, #7526, .T. ) ;
#26582=ORIENTED_EDGE ( 'NONE', *, *, #21759, .T. ) ;
#26591=CARTESIAN_POINT ( 'NONE',  ( 7.644554776091147741E-16, 12.48450537969573659, -122.4687500020483952 ) ) ;
#26593=CARTESIAN_POINT ( 'NONE',  ( 10.81189881249999729, 0.000000000000000000, -136.5312500020484094 ) ) ;
#26595=CARTESIAN_POINT ( 'NONE',  ( -5.405949406249996869, 9.363379034771805109, -140.3437500020484094 ) ) ;
#26596=CARTESIAN_POINT ( 'NONE',  ( -9.999999999999998224, 1.224646799147353059E-15, -172.2500000000000000 ) ) ;
#26599=CARTESIAN_POINT ( 'NONE',  ( -2.121150477449813534E-15, -11.54700538379251284, -153.8750000000000000 ) ) ;
#26603=CARTESIAN_POINT ( 'NONE',  ( -10.81189881249999729, 1.324075727343319199E-15, -51.59375000204835260 ) ) ;
#26605=CARTESIAN_POINT ( 'NONE',  ( -2.293366432827344421E-15, -12.48450537969573659, -163.7187500020483810 ) ) ;
#26610=CARTESIAN_POINT ( 'NONE',  ( -9.999999999999998224, 0.000000000000000000, -99.99999999999998579 ) ) ;
#26612=CARTESIAN_POINT ( 'NONE',  ( 5.000000000000000000, 8.660254037844385522, -90.24999999999998579 ) ) ;
#26614=CARTESIAN_POINT ( 'NONE',  ( -5.405949406250003975, -9.363379034771801557, -110.0312500020483810 ) ) ;
#26615=CARTESIAN_POINT ( 'NONE',  ( -4.999999999999996447, 8.660254037844387298, -132.3750000040967905 ) ) ;
#26620=CARTESIAN_POINT ( 'NONE',  ( -10.81189881249999729, 1.324075727343319199E-15, -50.28125000204835970 ) ) ;
#26627=ORIENTED_EDGE ( 'NONE', *, *, #6321, .T. ) ;
#26638=ADVANCED_FACE ( 'NONE', ( #27854 ), #17683, .F. ) ;
#26642=CARTESIAN_POINT ( 'NONE',  ( -10.81189881249999907, -6.242252689847864744, -145.9687500020484094 ) ) ;
#26643=( BOUNDED_CURVE ( )  B_SPLINE_CURVE ( 2, ( #8057, #33747, #40612, #21204, #4808, #4168, #17313 ),
 .UNSPECIFIED., .F., .F. ) 
 B_SPLINE_CURVE_WITH_KNOTS ( ( 3, 2, 2, 3 ),
 ( 0.4477611940298508730, 0.4490049751243782028, 0.4502487562189055881, 0.4514925373134329734 ),
 .UNSPECIFIED. ) 
 CURVE ( )  GEOMETRIC_REPRESENTATION_ITEM ( )  RATIONAL_B_SPLINE_CURVE ( ( 0.9999999999999880096, 0.8660254037844506980, 1.000000000000000000, 0.8660254037844387076, 1.000000000000000000, 0.8660254037844267172, 1.000000000000011990 ) ) 
 REPRESENTATION_ITEM ( '' )  );
#26644=CARTESIAN_POINT ( 'NONE',  ( 10.81189881249999729, 6.242252689847867408, -163.2187500020483810 ) ) ;
#26646=CARTESIAN_POINT ( 'NONE',  ( -9.999999999999998224, 1.224646799147353059E-15, -184.2500000000000000 ) ) ;
#26650=FACE_OUTER_BOUND ( 'NONE', #12368, .T. ) ;
#26651=CARTESIAN_POINT ( 'NONE',  ( 10.81189881249999907, 6.242252689847868297, -187.2187500020484094 ) ) ;
#26654=CARTESIAN_POINT ( 'NONE',  ( 10.81189881249999729, 0.000000000000000000, -54.03125000204836681 ) ) ;
#26656=CARTESIAN_POINT ( 'NONE',  ( 10.00000000000000000, 5.773502691896255534, -117.3750000000000000 ) ) ;
#26658=CARTESIAN_POINT ( 'NONE',  ( -10.81189881249999729, -6.242252689847864744, -134.1562500020483810 ) ) ;
#26659=CARTESIAN_POINT ( 'NONE',  ( -5.405949406250003975, -9.363379034771801557, -147.5312500020483810 ) ) ;
#26661=CARTESIAN_POINT ( 'NONE',  ( -5.000000000000003553, -8.660254037844383745, -125.5000000000000000 ) ) ;
#26662=CARTESIAN_POINT ( 'NONE',  ( -10.81189881249999729, 6.242252689847871849, -83.21875000204838102 ) ) ;
#26665=CARTESIAN_POINT ( 'NONE',  ( 10.81189881249999907, 6.242252689847868297, -179.7187500020484094 ) ) ;
#26668=CARTESIAN_POINT ( 'NONE',  ( -5.000000000000003553, -8.660254037844383745, -175.3750000040967905 ) ) ;
#26669=CARTESIAN_POINT ( 'NONE',  ( 5.405949406249999534, 9.363379034771803333, -79.28125000204838102 ) ) ;
#26671=CARTESIAN_POINT ( 'NONE',  ( 7.070501591499377789E-16, 11.54700538379251284, -53.00000000409676915 ) ) ;
#26672=CARTESIAN_POINT ( 'NONE',  ( 5.405949406249992428, -9.363379034771808662, -12.09375000204834727 ) ) ;
#26673=CARTESIAN_POINT ( 'NONE',  ( 9.999999999999998224, 0.000000000000000000, -137.3750000040967905 ) ) ;
#26675=CARTESIAN_POINT ( 'NONE',  ( -2.293366432827344421E-15, -12.48450537969573659, -9.406250002048365033 ) ) ;
#26685=CARTESIAN_POINT ( 'NONE',  ( -2.121150477449813534E-15, -11.54700538379251284, -153.8749999999999716 ) ) ;
#26698=CARTESIAN_POINT ( 'NONE',  ( 10.81189881249999551, -6.242252689847874514, -151.6562500020484094 ) ) ;
#26701=CARTESIAN_POINT ( 'NONE',  ( 0.000000000000000000, 0.000000000000000000, -99.99999999999998579 ) ) ;
#26704=CARTESIAN_POINT ( 'NONE',  ( -5.405949406250003975, -9.363379034771801557, -72.34375000204836681 ) ) ;
#26705=CARTESIAN_POINT ( 'NONE',  ( -10.81189881249999729, 6.242252689847871849, -74.40625000204836681 ) ) ;
#26707=CARTESIAN_POINT ( 'NONE',  ( 9.999999999999998224, 0.000000000000000000, -115.9999999999999858 ) ) ;
#26708=CARTESIAN_POINT ( 'NONE',  ( -10.81189881249999729, -6.242252689847864744, -159.6562500020484094 ) ) ;
#26709=CARTESIAN_POINT ( 'NONE',  ( -5.405949406249996869, 9.363379034771805109, -173.5312500020484094 ) ) ;
#26711=CARTESIAN_POINT ( 'NONE',  ( 10.81189881249999551, -6.242252689847874514, -1.468750002048352377 ) ) ;
#26713=CARTESIAN_POINT ( 'NONE',  ( 10.81189881249999729, 0.000000000000000000, -103.3437500020483668 ) ) ;
#26715=CARTESIAN_POINT ( 'NONE',  ( 7.644554776091147741E-16, 12.48450537969573659, -5.656250002048362369 ) ) ;
#26718=CARTESIAN_POINT ( 'NONE',  ( -2.293366432827344421E-15, -12.48450537969573659, -108.4062500020483810 ) ) ;
#26721=CARTESIAN_POINT ( 'NONE',  ( 9.999999999999998224, 0.000000000000000000, -84.87500000409677625 ) ) ;
#26723=CARTESIAN_POINT ( 'NONE',  ( -2.293366432827344421E-15, -12.48450537969573659, -45.21875000204835970 ) ) ;
#26729=CARTESIAN_POINT ( 'NONE',  ( -2.121150477449813534E-15, -11.54700538379251284, -10.25000000409676026 ) ) ;
#26734=VECTOR ( 'NONE', #28037, 1000.000000000000000 ) ;
#26737=( BOUNDED_CURVE ( )  B_SPLINE_CURVE ( 2, ( #2331, #22589, #35766, #41362, #8587, #35344, #15460 ),
 .UNSPECIFIED., .F., .F. ) 
 B_SPLINE_CURVE_WITH_KNOTS ( ( 3, 2, 2, 3 ),
 ( 0.4925373134328359104, 0.4937810945273632957, 0.4950248756218906809, 0.4962686567164180107 ),
 .UNSPECIFIED. ) 
 CURVE ( )  GEOMETRIC_REPRESENTATION_ITEM ( )  RATIONAL_B_SPLINE_CURVE ( ( 0.9999999999999880096, 0.8660254037844506980, 1.000000000000000000, 0.8660254037844387076, 1.000000000000000000, 0.8660254037844267172, 1.000000000000011990 ) ) 
 REPRESENTATION_ITEM ( '' )  );
#26748=CARTESIAN_POINT ( 'NONE',  ( 10.81189881249999907, 6.242252689847868297, -172.4062500020484094 ) ) ;
#26750=EDGE_CURVE ( 'NONE', #32882, #25640, #2843, .T. ) ;
#26752=CARTESIAN_POINT ( 'NONE',  ( -10.81189881249999907, -6.242252689847864744, -90.46875000204836681 ) ) ;
#26754=CARTESIAN_POINT ( 'NONE',  ( -2.293366432827344421E-15, -12.48450537969573659, -99.40625000204839523 ) ) ;
#26756=CARTESIAN_POINT ( 'NONE',  ( 10.81189881249999729, 6.242252689847867408, -116.7187500020483810 ) ) ;
#26760=CARTESIAN_POINT ( 'NONE',  ( 10.81189881249999907, 6.242252689847868297, -197.9062500020484379 ) ) ;
#26763=CARTESIAN_POINT ( 'NONE',  ( 7.070501591499377789E-16, 11.54700538379251284, -179.0000000040967905 ) ) ;
#26765=CARTESIAN_POINT ( 'NONE',  ( 5.405949406249992428, -9.363379034771808662, -33.09375000204836681 ) ) ;
#26767=CARTESIAN_POINT ( 'NONE',  ( -5.405949406249996869, 9.363379034771805109, -126.8437500020483952 ) ) ;
#26769=CARTESIAN_POINT ( 'NONE',  ( -5.405949406249996869, 9.363379034771805109, -40.03125000204838102 ) ) ;
#26772=CARTESIAN_POINT ( 'NONE',  ( -4.999999999999996447, 8.660254037844387298, -56.99999999999996447 ) ) ;
#26773=CARTESIAN_POINT ( 'NONE',  ( -5.405949406250003975, -9.363379034771801557, -131.0312500020484094 ) ) ;
#26778=CARTESIAN_POINT ( 'NONE',  ( 9.999999999999998224, 0.000000000000000000, -105.8750000040967763 ) ) ;
#26779=CARTESIAN_POINT ( 'NONE',  ( -9.999999999999998224, 1.224646799147353059E-15, -146.7500000000000000 ) ) ;
#26780=CARTESIAN_POINT ( 'NONE',  ( -5.405949406249996869, 9.363379034771805109, -63.84375000204836681 ) ) ;
#26781=ORIENTED_EDGE ( 'NONE', *, *, #40656, .F. ) ;
#26784=CARTESIAN_POINT ( 'NONE',  ( -9.999999999999998224, 1.224646799147353059E-15, -124.6250000040967763 ) ) ;
#26785=CARTESIAN_POINT ( 'NONE',  ( 5.000000000000000000, 8.660254037844385522, -36.62500000409676915 ) ) ;
#26794=CARTESIAN_POINT ( 'NONE',  ( 9.999999999999998224, 1.224646799147353059E-15, -99.99999999999998579 ) ) ;
#26795=CARTESIAN_POINT ( 'NONE',  ( -2.121150477449813534E-15, -11.54700538379251284, -104.3749999999999858 ) ) ;
#26797=CARTESIAN_POINT ( 'NONE',  ( -5.405949406250003975, -9.363379034771801557, -194.0312500020484094 ) ) ;
#26803=CARTESIAN_POINT ( 'NONE',  ( -9.999999999999479527, -5.773502691896549521, -116.6249999999999574 ) ) ;
#26804=CARTESIAN_POINT ( 'NONE',  ( -5.405949406250003975, -9.363379034771801557, -121.8437500020483952 ) ) ;
#26805=CARTESIAN_POINT ( 'NONE',  ( 5.405949406249999534, 9.363379034771803333, 0.4062499979516354109 ) ) ;
#26806=CARTESIAN_POINT ( 'NONE',  ( -5.405949406249996869, 9.363379034771805109, -131.5312500020484094 ) ) ;
#26808=CARTESIAN_POINT ( 'NONE',  ( -5.405949406249996869, 9.363379034771805109, -138.8437500020484094 ) ) ;
#26811=CARTESIAN_POINT ( 'NONE',  ( -4.999999999999996447, 8.660254037844387298, -159.0000000000000000 ) ) ;
#26816=CARTESIAN_POINT ( 'NONE',  ( -5.405949406250003975, -9.363379034771801557, -52.84375000204835970 ) ) ;
#26818=CARTESIAN_POINT ( 'NONE',  ( -10.81189881249999729, 1.324075727343319199E-15, -161.0937500020484094 ) ) ;
#26821=CARTESIAN_POINT ( 'NONE',  ( -2.121150477449813534E-15, -11.54700538379251284, -86.37499999999997158 ) ) ;
#26823=VERTEX_POINT ( 'NONE', #18143 ) ;
#26824=CARTESIAN_POINT ( 'NONE',  ( -10.81189881249999729, 1.324075727343319199E-15, -113.2812500020483952 ) ) ;
#26825=CARTESIAN_POINT ( 'NONE',  ( 9.999999999999998224, 0.000000000000000000, -131.3750000040967905 ) ) ;
#26826=CARTESIAN_POINT ( 'NONE',  ( -9.999999999999998224, 1.224646799147353059E-15, -112.2499999999999858 ) ) ;
#26828=DIRECTION ( 'NONE',  ( -1.000000000000000000, 0.000000000000000000, 0.000000000000000000 ) ) ;
#26829=CARTESIAN_POINT ( 'NONE',  ( -10.81189881249999729, 6.242252689847871849, -48.90625000204836681 ) ) ;
#26830=CARTESIAN_POINT ( 'NONE',  ( 9.999999999999998224, 0.000000000000000000, -135.5000000000000000 ) ) ;
#26832=VECTOR ( 'NONE', #20425, 1000.000000000000000 ) ;
#26852=CARTESIAN_POINT ( 'NONE',  ( -10.81189881249999729, 1.324075727343319199E-15, -152.0937500020483810 ) ) ;
#26853=CARTESIAN_POINT ( 'NONE',  ( 10.81189881249999551, -6.242252689847874514, -160.4687500020484094 ) ) ;
#26854=CARTESIAN_POINT ( 'NONE',  ( -9.999999999999998224, 1.224646799147353059E-15, -106.6250000040967763 ) ) ;
#26856=CARTESIAN_POINT ( 'NONE',  ( 9.999999999999996447, -5.773502691896262640, -177.6250000000000000 ) ) ;
#26861=CARTESIAN_POINT ( 'NONE',  ( 5.000000000000000000, 8.660254037844385522, -168.6250000040967905 ) ) ;
#26862=CARTESIAN_POINT ( 'NONE',  ( 10.81189881249999729, 0.000000000000000000, -182.8437500020483810 ) ) ;
#26865=CARTESIAN_POINT ( 'NONE',  ( -10.81189881249999729, 6.242252689847871849, -50.40625000204837391 ) ) ;
#26867=CARTESIAN_POINT ( 'NONE',  ( -9.999999999999998224, 1.224646799147353059E-15, -104.7499999999999858 ) ) ;
#26869=CARTESIAN_POINT ( 'NONE',  ( -10.81189881249999729, 6.242252689847871849, -135.9062500020484094 ) ) ;
#26870=CARTESIAN_POINT ( 'NONE',  ( -2.293366432827344421E-15, -12.48450537969573659, -144.4062500020484094 ) ) ;
#26872=CARTESIAN_POINT ( 'NONE',  ( 10.81189881249999729, 0.000000000000000000, -79.34375000204838102 ) ) ;
#26875=CARTESIAN_POINT ( 'NONE',  ( 7.644554776091147741E-16, 12.48450537969573659, -177.9687500020483810 ) ) ;
#26877=CARTESIAN_POINT ( 'NONE',  ( -9.999999999999998224, 1.224646799147353059E-15, -110.7499999999999858 ) ) ;
#26878=CARTESIAN_POINT ( 'NONE',  ( -2.121150477449813534E-15, -11.54700538379251284, -175.2500000040968189 ) ) ;
#26879=CARTESIAN_POINT ( 'NONE',  ( 10.81189881249999907, 6.242252689847868297, -74.90625000204839523 ) ) ;
#26881=CARTESIAN_POINT ( 'NONE',  ( -4.999999999999996447, 8.660254037844387298, -55.87500000409676204 ) ) ;
#26882=CARTESIAN_POINT ( 'NONE',  ( 10.81189881249999551, -6.242252689847874514, -11.96875000204836326 ) ) ;
#26885=CARTESIAN_POINT ( 'NONE',  ( -10.81189881249999907, -6.242252689847864744, -8.156250002048365033 ) ) ;
#26886=CARTESIAN_POINT ( 'NONE',  ( 0.000000000000000000, 0.000000000000000000, -99.99999999999998579 ) ) ;
#26888=CARTESIAN_POINT ( 'NONE',  ( 9.999999999999479527, 5.773502691896553074, -177.7500000040967620 ) ) ;
#26892=VERTEX_POINT ( 'NONE', #31768 ) ;
#26893=CARTESIAN_POINT ( 'NONE',  ( 1.351487262974977233, 10.72709830801206543, -100.0000000000000000 ) ) ;
#26895=ORIENTED_EDGE ( 'NONE', *, *, #4394, .T. ) ;
#26896=( BOUNDED_CURVE ( )  B_SPLINE_CURVE ( 2, ( #8934, #27933, #24923, #12151, #11725, #2465, #15171 ),
 .UNSPECIFIED., .F., .F. ) 
 B_SPLINE_CURVE_WITH_KNOTS ( ( 3, 2, 2, 3 ),
 ( 0.2500000000000001110, 0.2512437810945274963, 0.2524875621890548261, 0.2537313432835822113 ),
 .UNSPECIFIED. ) 
 CURVE ( )  GEOMETRIC_REPRESENTATION_ITEM ( )  RATIONAL_B_SPLINE_CURVE ( ( 0.9999999999999880096, 0.8660254037844506980, 1.000000000000000000, 0.8660254037844387076, 1.000000000000000000, 0.8660254037844267172, 1.000000000000011990 ) ) 
 REPRESENTATION_ITEM ( '' )  );
#26900=CARTESIAN_POINT ( 'NONE',  ( -9.999999999999998224, 1.224646799147353059E-15, -115.6250000040967905 ) ) ;
#26901=CARTESIAN_POINT ( 'NONE',  ( -10.00000000000000000, -5.773502691896251982, -46.12499999999997158 ) ) ;
#26905=CARTESIAN_POINT ( 'NONE',  ( -9.999999999999996447, 5.773502691896259975, -172.3750000000000568 ) ) ;
#26906=CARTESIAN_POINT ( 'NONE',  ( 5.405949406249992428, -9.363379034771808662, -147.2812500020483810 ) ) ;
#26908=DIRECTION ( 'NONE',  ( -0.000000000000000000, -0.000000000000000000, -1.000000000000000000 ) ) ;
#26913=CARTESIAN_POINT ( 'NONE',  ( 10.81189881249999907, 6.242252689847868297, -71.71875000204836681 ) ) ;
#26914=CARTESIAN_POINT ( 'NONE',  ( -5.405949406249996869, 9.363379034771805109, -74.53125000204838102 ) ) ;
#26916=CARTESIAN_POINT ( 'NONE',  ( 7.644554776091147741E-16, 12.48450537969573659, -158.6562500020484094 ) ) ;
#26917=CARTESIAN_POINT ( 'NONE',  ( -5.405949406249996869, 9.363379034771805109, -170.5312500020484094 ) ) ;
#26921=CARTESIAN_POINT ( 'NONE',  ( 5.405949406249999534, 9.363379034771803333, -103.0937500020483810 ) ) ;
#26923=CARTESIAN_POINT ( 'NONE',  ( 5.405949406249992428, -9.363379034771808662, -3.281250002048374803 ) ) ;
#26927=CARTESIAN_POINT ( 'NONE',  ( 10.81189881249999907, 6.242252689847868297, -103.4062500020483952 ) ) ;
#26929=CARTESIAN_POINT ( 'NONE',  ( -9.999999999999998224, 5.773502691896259087, -73.75000000409676204 ) ) ;
#26930=CARTESIAN_POINT ( 'NONE',  ( -9.999999999999998224, 1.224646799147353059E-15, -133.6250000040967620 ) ) ;
#26931=CARTESIAN_POINT ( 'NONE',  ( -5.405949406250003975, -9.363379034771801557, -37.84375000204837391 ) ) ;
#26934=CARTESIAN_POINT ( 'NONE',  ( 5.405949406249992428, -9.363379034771808662, -27.28125000204836681 ) ) ;
#26938=CARTESIAN_POINT ( 'NONE',  ( 4.999999999999992006, -8.660254037844389075, -16.12500000409675138 ) ) ;
#26941=CARTESIAN_POINT ( 'NONE',  ( 5.000000000000000000, 8.660254037844385522, -123.2500000000000000 ) ) ;
#26943=ORIENTED_EDGE ( 'NONE', *, *, #6913, .T. ) ;
#26955=CARTESIAN_POINT ( 'NONE',  ( 7.644554776091147741E-16, 12.48450537969573659, -172.1562500020484094 ) ) ;
#26958=CARTESIAN_POINT ( 'NONE',  ( 7.644554776091147741E-16, 12.48450537969573659, -95.46875000204839523 ) ) ;
#26959=CARTESIAN_POINT ( 'NONE',  ( 10.81189881249999729, 0.000000000000000000, -99.03125000204839523 ) ) ;
#26961=CARTESIAN_POINT ( 'NONE',  ( -10.81189881249999729, 1.324075727343319199E-15, -105.5937500020483810 ) ) ;
#26964=CARTESIAN_POINT ( 'NONE',  ( -10.81189881249999729, -6.242252689847864744, -179.1562500020484094 ) ) ;
#26965=CARTESIAN_POINT ( 'NONE',  ( 10.81189881249999907, 6.242252689847868297, -194.9062500020484379 ) ) ;
#26968=CARTESIAN_POINT ( 'NONE',  ( -2.121150477449813534E-15, -11.54700538379251284, -175.2500000040968189 ) ) ;
#26970=CARTESIAN_POINT ( 'NONE',  ( -10.81189881249999729, 6.242252689847871849, -21.71875000204837036 ) ) ;
#26972=CARTESIAN_POINT ( 'NONE',  ( 10.81189881249999551, -6.242252689847874514, -127.4687500020483810 ) ) ;
#26974=CARTESIAN_POINT ( 'NONE',  ( 10.81189881249999729, 0.000000000000000000, -30.03125000204837036 ) ) ;
#26976=CARTESIAN_POINT ( 'NONE',  ( 7.070501591499377789E-16, 11.54700538379251284, -61.62499999999998579 ) ) ;
#26977=CARTESIAN_POINT ( 'NONE',  ( -5.405949406249996869, 9.363379034771805109, -124.0312500020483952 ) ) ;
#26979=ORIENTED_EDGE ( 'NONE', *, *, #42434, .F. ) ;
#26982=CARTESIAN_POINT ( 'NONE',  ( 5.000000000000000000, 8.660254037844385522, -98.12500000409677625 ) ) ;
#26984=CARTESIAN_POINT ( 'NONE',  ( -10.81189881249999729, 1.324075727343319199E-15, -62.09375000204836681 ) ) ;
#26985=ORIENTED_EDGE ( 'NONE', *, *, #9191, .T. ) ;
#26987=PRODUCT_DEFINITION_FORMATION_WITH_SPECIFIED_SOURCE ( 'ANY', '', #18390, .NOT_KNOWN. ) ;
#26989=EDGE_CURVE ( 'NONE', #30038, #39101, #36728, .T. ) ;
#26994=CARTESIAN_POINT ( 'NONE',  ( 9.999999999999998224, 0.000000000000000000, -36.87500000409676915 ) ) ;
#26997=CARTESIAN_POINT ( 'NONE',  ( 24.99999999999999645, 3.061616997868382648E-15, -99.99999999999998579 ) ) ;
#27001=CARTESIAN_POINT ( 'NONE',  ( -9.999999999999998224, 1.224646799147353059E-15, -105.1250000040967763 ) ) ;
#27010=CARTESIAN_POINT ( 'NONE',  ( -5.405949406249996869, 9.363379034771805109, -197.5312500020484094 ) ) ;
#27015=CARTESIAN_POINT ( 'NONE',  ( -9.999999999999998224, 1.224646799147353059E-15, -116.7499999999999858 ) ) ;
#27016=CARTESIAN_POINT ( 'NONE',  ( -5.405949406250003975, -9.363379034771801557, -118.8437500020483810 ) ) ;
#27017=CARTESIAN_POINT ( 'NONE',  ( 5.000000000000000000, 8.660254037844385522, -197.1250000040967905 ) ) ;
#27018=CARTESIAN_POINT ( 'NONE',  ( -2.293366432827344421E-15, -12.48450537969573659, -124.9062500020483810 ) ) ;
#27021=CARTESIAN_POINT ( 'NONE',  ( 10.81189881249999729, 0.000000000000000000, -137.8437500020484094 ) ) ;
#27023=CARTESIAN_POINT ( 'NONE',  ( 9.999999999999227285, 5.773502691896701400, -110.2500000040967478 ) ) ;
#27024=CARTESIAN_POINT ( 'NONE',  ( 9.999999999999996447, -5.773502691896262640, -156.6250000000000000 ) ) ;
#27025=CARTESIAN_POINT ( 'NONE',  ( -9.999999999999998224, 1.224646799147353059E-15, -23.74999999999996447 ) ) ;
#27031=CARTESIAN_POINT ( 'NONE',  ( 10.81189881249999729, 0.000000000000000000, -47.84375000204838102 ) ) ;
#27033=CARTESIAN_POINT ( 'NONE',  ( 10.81189881249999729, 0.000000000000000000, -151.3437500020483810 ) ) ;
#27038=CARTESIAN_POINT ( 'NONE',  ( -10.00000000000000000, -5.773502691896251982, -83.62499999999998579 ) ) ;
#27040=VERTEX_POINT ( 'NONE', #2822 ) ;
#27041=( BOUNDED_CURVE ( )  B_SPLINE_CURVE ( 2, ( #11957, #35074, #18436, #25147, #21894, #8949, #21679 ),
 .UNSPECIFIED., .F., .F. ) 
 B_SPLINE_CURVE_WITH_KNOTS ( ( 3, 2, 2, 3 ),
 ( 0.2201492537313433639, 0.2213930348258707215, 0.2226368159203980790, 0.2238805970149254365 ),
 .UNSPECIFIED. ) 
 CURVE ( )  GEOMETRIC_REPRESENTATION_ITEM ( )  RATIONAL_B_SPLINE_CURVE ( ( 0.9999999999999910072, 0.8660254037844477004, 1.000000000000000000, 0.8660254037844387076, 1.000000000000000000, 0.8660254037844327124, 1.000000000000005995 ) ) 
 REPRESENTATION_ITEM ( '' )  );
#27042=CARTESIAN_POINT ( 'NONE',  ( -2.293366432827344421E-15, -12.48450537969573659, -111.4062500020483952 ) ) ;
#27043=CARTESIAN_POINT ( 'NONE',  ( 7.070501591499377789E-16, 11.54700538379251284, -129.5000000040967620 ) ) ;
#27044=CARTESIAN_POINT ( 'NONE',  ( -9.999999999999998224, 1.224646799147353059E-15, -178.2500000000000284 ) ) ;
#27047=CARTESIAN_POINT ( 'NONE',  ( -5.405949406250003975, -9.363379034771801557, -48.53125000204838813 ) ) ;
#27048=AXIS2_PLACEMENT_3D ( 'NONE', #32547, #22189, #12448 ) ;
#27069=CARTESIAN_POINT ( 'NONE',  ( 10.81189881249999907, 6.242252689847868297, -139.2187500020484094 ) ) ;
#27070=CARTESIAN_POINT ( 'NONE',  ( -5.405949406249996869, 9.363379034771805109, -165.8437500020484094 ) ) ;
#27072=CARTESIAN_POINT ( 'NONE',  ( -5.000000000000003553, -8.660254037844383745, -139.3750000040968189 ) ) ;
#27073=CARTESIAN_POINT ( 'NONE',  ( -2.121150477449813534E-15, -11.54700538379251284, -179.3750000000000284 ) ) ;
#27077=CARTESIAN_POINT ( 'NONE',  ( 0.000000000000000000, 0.000000000000000000, -99.99999999999998579 ) ) ;
#27078=CARTESIAN_POINT ( 'NONE',  ( 5.405949406249992428, -9.363379034771808662, -175.5937500020484094 ) ) ;
#27081=CARTESIAN_POINT ( 'NONE',  ( -10.81189881249999907, -6.242252689847864744, -48.65625000204836681 ) ) ;
#27083=CARTESIAN_POINT ( 'NONE',  ( 4.999999999999992006, -8.660254037844389075, -104.2499999999999858 ) ) ;
#27084=ORIENTED_EDGE ( 'NONE', *, *, #20111, .T. ) ;
#27085=CARTESIAN_POINT ( 'NONE',  ( 10.81189881249999729, 6.242252689847867408, -136.4062500020484094 ) ) ;
#27086=CARTESIAN_POINT ( 'NONE',  ( -5.405949406250003975, -9.363379034771801557, -150.5312500020483810 ) ) ;
#27088=CARTESIAN_POINT ( 'NONE',  ( -10.81189881249999729, 1.324075727343319199E-15, -83.09375000204836681 ) ) ;
#27091=CARTESIAN_POINT ( 'NONE',  ( 10.81189881249999907, 6.242252689847868297, -178.2187500020483810 ) ) ;
#27093=CARTESIAN_POINT ( 'NONE',  ( -9.999999999999227285, -5.773502691896698735, -110.6249999999999574 ) ) ;
#27095=CARTESIAN_POINT ( 'NONE',  ( 7.644554776091147741E-16, 12.48450537969573659, -79.15625000204838102 ) ) ;
#27097=CARTESIAN_POINT ( 'NONE',  ( 9.999999999999998224, 0.000000000000000000, -51.87500000409675494 ) ) ;
#27098=CARTESIAN_POINT ( 'NONE',  ( 7.644554776091147741E-16, 12.48450537969573659, -6.968750002048357040 ) ) ;
#27101=CARTESIAN_POINT ( 'NONE',  ( 10.81189881249999551, -6.242252689847874514, -3.156250002048361036 ) ) ;
#27104=CARTESIAN_POINT ( 'NONE',  ( 10.00000000000102318, -5.773502691895667560, -103.0000000040967194 ) ) ;
#27105=CARTESIAN_POINT ( 'NONE',  ( 5.000000000000000000, 8.660254037844385522, -177.6250000040968189 ) ) ;
#27110=CARTESIAN_POINT ( 'NONE',  ( -9.999999999999612754, -5.773502691896474914, -154.1249999999999716 ) ) ;
#27112=( BOUNDED_CURVE ( )  B_SPLINE_CURVE ( 2, ( #10814, #30694, #15116, #12307, #8462, #11457, #41231 ),
 .UNSPECIFIED., .F., .F. ) 
 B_SPLINE_CURVE_WITH_KNOTS ( ( 3, 2, 2, 3 ),
 ( 0.09701492537313441411, 0.09825870646766173000, 0.09950248756218905977, 0.1007462686567163757 ),
 .UNSPECIFIED. ) 
 CURVE ( )  GEOMETRIC_REPRESENTATION_ITEM ( )  RATIONAL_B_SPLINE_CURVE ( ( 0.9999999999999910072, 0.8660254037844477004, 1.000000000000000000, 0.8660254037844387076, 1.000000000000000000, 0.8660254037844431485, 0.9999999999999955591 ) ) 
 REPRESENTATION_ITEM ( '' )  );
#27119=B_SPLINE_CURVE_WITH_KNOTS ( 'NONE', 3,
 ( #30707, #24453, #17085, #23799, #33950, #37599, #8043, #36954, #20544, #4583, #40181, #30503, #24669, #1353, #30918, #17512, #34377, #930, #14483, #1138, #33732, #27892, #14261, #27678, #37814, #20330, #14046, #7607, #10612 ),
 .UNSPECIFIED., .F., .F.,
 ( 4, 2, 2, 2, 2, 2, 2, 2, 2, 2, 2, 2, 1, 2, 4 ),
 ( 0.000000000000000000, 0.001276655870610494525, 0.002553311741220990350, 0.005106623482441982435, 0.006383279353052479128, 0.007659935223662975821, 0.008936591094273473382, 0.01021324696488396834, 0.01148990283549446330, 0.01276655870610495652, 0.01531987044732594644, 0.01659652631793644140, 0.01787318218854693636, 0.01914983805915743131, 0.02042649392976792627 ),
 .UNSPECIFIED. ) ;
#27120=CARTESIAN_POINT ( 'NONE',  ( -2.121150477449813534E-15, -11.54700538379251284, -45.87499999999997158 ) ) ;
#27125=CARTESIAN_POINT ( 'NONE',  ( 9.999999999999998224, 0.000000000000000000, -144.5000000000000000 ) ) ;
#27130=CARTESIAN_POINT ( 'NONE',  ( -5.405949406249996869, 9.363379034771805109, -66.84375000204836681 ) ) ;
#27131=CARTESIAN_POINT ( 'NONE',  ( -10.81189881249999729, 6.242252689847871849, -75.90625000204838102 ) ) ;
#27133=CARTESIAN_POINT ( 'NONE',  ( 10.81189881249999729, 0.000000000000000000, -156.0312500020484094 ) ) ;
#27134=CARTESIAN_POINT ( 'NONE',  ( 7.644554776091147741E-16, 12.48450537969573659, -175.1562500020484094 ) ) ;
#27135=CARTESIAN_POINT ( 'NONE',  ( 5.405949406249992428, -9.363379034771808662, -1.593750002048366365 ) ) ;
#27137=CARTESIAN_POINT ( 'NONE',  ( -5.405949406250003975, -9.363379034771801557, -109.8437500020483810 ) ) ;
#27138=CARTESIAN_POINT ( 'NONE',  ( 9.999999999999998224, 0.000000000000000000, -156.5000000000000000 ) ) ;
#27140=CARTESIAN_POINT ( 'NONE',  ( -10.81189881249999907, -6.242252689847864744, -3.656250002048361036 ) ) ;
#27143=CARTESIAN_POINT ( 'NONE',  ( -5.405949406250003975, -9.363379034771801557, -99.53125000204839523 ) ) ;
#27145=CARTESIAN_POINT ( 'NONE',  ( -9.999999999999998224, 1.224646799147353059E-15, -78.12500000409677625 ) ) ;
#27146=CARTESIAN_POINT ( 'NONE',  ( -4.999999999999996447, 8.660254037844387298, -118.5000000000000000 ) ) ;
#27147=CARTESIAN_POINT ( 'NONE',  ( 10.81189881249999907, 6.242252689847868297, -34.21875000204835260 ) ) ;
#27151=CARTESIAN_POINT ( 'NONE',  ( -10.81189881249999729, 6.242252689847871849, -26.40625000204838102 ) ) ;
#27153=CARTESIAN_POINT ( 'NONE',  ( -9.999999999999998224, 5.773502691896259087, -4.750000004096754935 ) ) ;
#27162=EDGE_LOOP ( 'NONE', ( #37619, #35507, #23279, #22391 ) ) ;
#27168=DIRECTION ( 'NONE',  ( -1.000000000000000000, 0.000000000000000000, 0.000000000000000000 ) ) ;
#27170=CARTESIAN_POINT ( 'NONE',  ( 10.81189881249999907, 6.242252689847868297, -175.4062500020484094 ) ) ;
#27172=EDGE_CURVE ( 'NONE', #38211, #31374, #38376, .T. ) ;
#27174=CARTESIAN_POINT ( 'NONE',  ( -2.293366432827344421E-15, -12.48450537969573659, -91.71875000204838102 ) ) ;
#27175=CARTESIAN_POINT ( 'NONE',  ( -4.999999999999996447, 8.660254037844387298, -106.4999999999999858 ) ) ;
#27176=CARTESIAN_POINT ( 'NONE',  ( -2.293366432827344421E-15, -12.48450537969573659, -103.9062500020483810 ) ) ;
#27178=CARTESIAN_POINT ( 'NONE',  ( -5.405949406249996869, 9.363379034771805109, -110.3437500020483810 ) ) ;
#27180=CARTESIAN_POINT ( 'NONE',  ( -4.999999999999996447, 8.660254037844387298, -107.9999999999999858 ) ) ;
#27181=CARTESIAN_POINT ( 'NONE',  ( 9.999999999999998224, 0.000000000000000000, -152.3750000040967905 ) ) ;
#27182=CARTESIAN_POINT ( 'NONE',  ( -2.293366432827344421E-15, -12.48450537969573659, -192.4062500020484094 ) ) ;
#27185=CARTESIAN_POINT ( 'NONE',  ( -4.999999999999996447, 8.660254037844387298, -169.8750000040967905 ) ) ;
#27187=CARTESIAN_POINT ( 'NONE',  ( 10.81189881249999729, 0.000000000000000000, -25.34375000204835970 ) ) ;
#27188=FACE_OUTER_BOUND ( 'NONE', #41189, .T. ) ;
#27189=CARTESIAN_POINT ( 'NONE',  ( 7.644554776091147741E-16, 12.48450537969573659, -131.4687500020483810 ) ) ;
#27191=CARTESIAN_POINT ( 'NONE',  ( -10.81189881249999729, 1.324075727343319199E-15, -30.78125000204837036 ) ) ;
#27193=CARTESIAN_POINT ( 'NONE',  ( 10.00000000000000000, 5.773502691896255534, -55.87499999999997158 ) ) ;
#27194=CARTESIAN_POINT ( 'NONE',  ( 10.81189881249999907, 6.242252689847868297, -121.4062500020483810 ) ) ;
#27198=CARTESIAN_POINT ( 'NONE',  ( -5.000000000000003553, -8.660254037844383745, -101.8750000040967905 ) ) ;
#27199=FACE_OUTER_BOUND ( 'NONE', #25797, .T. ) ;
#27200=CARTESIAN_POINT ( 'NONE',  ( -10.81189881249999907, -6.242252689847864744, -60.46875000204838102 ) ) ;
#27201=ORIENTED_EDGE ( 'NONE', *, *, #4394, .F. ) ;
#27205=CARTESIAN_POINT ( 'NONE',  ( 7.070501591499377789E-16, 11.54700538379251284, -26.00000000409677270 ) ) ;
#27206=CARTESIAN_POINT ( 'NONE',  ( 9.999999999999994671, -5.773502691896262640, -138.6250000000000000 ) ) ;
#27214=CARTESIAN_POINT ( 'NONE',  ( 5.405949406249992428, -9.363379034771808662, -195.2812500020484094 ) ) ;
#27218=EDGE_CURVE ( 'NONE', #27040, #27517, #32595, .T. ) ;
#27223=CARTESIAN_POINT ( 'NONE',  ( -10.81189881249999729, 1.324075727343319199E-15, -119.0937500020483810 ) ) ;
#27224=CARTESIAN_POINT ( 'NONE',  ( 7.070501591499377789E-16, 11.54700538379251284, -192.5000000040968189 ) ) ;
#27225=CARTESIAN_POINT ( 'NONE',  ( 10.81189881249999551, -6.242252689847874514, -127.6562500020483952 ) ) ;
#27227=CARTESIAN_POINT ( 'NONE',  ( -10.81189881249999729, -6.242252689847864744, -127.9687500020483810 ) ) ;
#27228=CARTESIAN_POINT ( 'NONE',  ( 9.999999999999742428, 5.773502691896404748, -163.8750000000000284 ) ) ;
#27230=CARTESIAN_POINT ( 'NONE',  ( -10.00000000000000000, -5.773502691896251982, -155.6249999999999716 ) ) ;
#27231=CARTESIAN_POINT ( 'NONE',  ( 4.999999999999992006, -8.660254037844389075, -23.24999999999996447 ) ) ;
#27234=LINE ( 'NONE', #30496, #11166 ) ;
#27236=CARTESIAN_POINT ( 'NONE',  ( 10.81189881249999551, -6.242252689847874514, -43.46875000204836681 ) ) ;
#27238=CARTESIAN_POINT ( 'NONE',  ( -5.405949406250003975, -9.363379034771801557, -153.3437500020483810 ) ) ;
#27243=CARTESIAN_POINT ( 'NONE',  ( 7.070501591499377789E-16, 11.54700538379251284, -81.12499999999997158 ) ) ;
#27245=ORIENTED_EDGE ( 'NONE', *, *, #1751, .F. ) ;
#27246=CARTESIAN_POINT ( 'NONE',  ( -10.81189881249999729, -6.242252689847864744, -107.1562500020483952 ) ) ;
#27247=CARTESIAN_POINT ( 'NONE',  ( 4.999999999999992006, -8.660254037844389075, -127.1250000040967620 ) ) ;
#27249=EDGE_CURVE ( 'NONE', #30972, #17641, #11642, .T. ) ;
#27250=FACE_OUTER_BOUND ( 'NONE', #29663, .T. ) ;
#27251=CARTESIAN_POINT ( 'NONE',  ( -10.81189881249999907, -6.242252689847864744, -56.15625000204838102 ) ) ;
#27258=CARTESIAN_POINT ( 'NONE',  ( 5.000000000000000000, 8.660254037844385522, -164.1250000040967905 ) ) ;
#27259=ORIENTED_EDGE ( 'NONE', *, *, #14202, .T. ) ;
#27260=ORIENTED_EDGE ( 'NONE', *, *, #29565, .T. ) ;
#27271=FACE_OUTER_BOUND ( 'NONE', #691, .T. ) ;
#27277=CARTESIAN_POINT ( 'NONE',  ( 10.81189881249999907, 6.242252689847868297, -145.2187500020484094 ) ) ;
#27278=CARTESIAN_POINT ( 'NONE',  ( -10.81189881249999729, -6.242252689847864744, -150.4687500020484094 ) ) ;
#27279=EDGE_CURVE ( 'NONE', #41954, #31616, #27694, .T. ) ;
#27281=( BOUNDED_CURVE ( )  B_SPLINE_CURVE ( 2, ( #32421, #25521, #15350, #28548, #25935, #38879, #39084 ),
 .UNSPECIFIED., .F., .F. ) 
 B_SPLINE_CURVE_WITH_KNOTS ( ( 3, 2, 2, 3 ),
 ( 0.3880597014925373789, 0.3893034825870647087, 0.3905472636815920939, 0.3917910447761194792 ),
 .UNSPECIFIED. ) 
 CURVE ( )  GEOMETRIC_REPRESENTATION_ITEM ( )  RATIONAL_B_SPLINE_CURVE ( ( 0.9999999999999940048, 0.8660254037844447028, 1.000000000000000000, 0.8660254037844387076, 1.000000000000000000, 0.8660254037844327124, 1.000000000000005995 ) ) 
 REPRESENTATION_ITEM ( '' )  );
#27282=CARTESIAN_POINT ( 'NONE',  ( 10.00000000000000000, 5.773502691896255534, -175.8750000000000000 ) ) ;
#27283=ADVANCED_FACE ( 'NONE', ( #7760 ), #8896, .T. ) ;
#27285=CARTESIAN_POINT ( 'NONE',  ( -9.999999999999998224, 1.224646799147353059E-15, -110.7499999999999858 ) ) ;
#27288=CARTESIAN_POINT ( 'NONE',  ( -10.81189881249999729, 6.242252689847871849, -180.7187500020483810 ) ) ;
#27292=CARTESIAN_POINT ( 'NONE',  ( 10.81189881249999729, 0.000000000000000000, -55.53125000204836681 ) ) ;
#27294=CARTESIAN_POINT ( 'NONE',  ( -9.999999999999998224, 5.773502691896259087, -104.8749999999999858 ) ) ;
#27296=( BOUNDED_CURVE ( )  B_SPLINE_CURVE ( 2, ( #27044, #519, #39979, #6975, #36327, #10410, #13634 ),
 .UNSPECIFIED., .F., .F. ) 
 B_SPLINE_CURVE_WITH_KNOTS ( ( 3, 2, 2, 3 ),
 ( 0.1082089552238805485, 0.1094527363184079616, 0.1106965174129353746, 0.1119402985074627876 ),
 .UNSPECIFIED. ) 
 CURVE ( )  GEOMETRIC_REPRESENTATION_ITEM ( )  RATIONAL_B_SPLINE_CURVE ( ( 1.000000000000004441, 0.8660254037844343777, 1.000000000000000000, 0.8660254037844387076, 1.000000000000000000, 0.8660254037844282715, 1.000000000000010436 ) ) 
 REPRESENTATION_ITEM ( '' )  );
#27297=CARTESIAN_POINT ( 'NONE',  ( 5.405949406249999534, 9.363379034771803333, -134.7812500020483810 ) ) ;
#27298=CARTESIAN_POINT ( 'NONE',  ( -10.00000000000000000, -5.773502691896251982, -150.0000000040967905 ) ) ;
#27299=CARTESIAN_POINT ( 'NONE',  ( -5.405949406249996869, 9.363379034771805109, -146.5312500020483810 ) ) ;
#27303=CARTESIAN_POINT ( 'NONE',  ( 5.405949406249992428, -9.363379034771808662, -183.0937500020483810 ) ) ;
#27306=LINE ( 'NONE', #11096, #17376 ) ;
#27307=CARTESIAN_POINT ( 'NONE',  ( -10.81189881249999729, 6.242252689847871849, -74.40625000204836681 ) ) ;
#27311=CARTESIAN_POINT ( 'NONE',  ( 7.070501591499377789E-16, 11.54700538379251284, -54.50000000409676915 ) ) ;
#27312=CARTESIAN_POINT ( 'NONE',  ( 7.644554776091147741E-16, 12.48450537969573659, -9.968750002048359704 ) ) ;
#27313=CARTESIAN_POINT ( 'NONE',  ( 9.999999999999998224, 0.000000000000000000, -105.4999999999999858 ) ) ;
#27315=CARTESIAN_POINT ( 'NONE',  ( 10.81189881249999907, 6.242252689847868297, -5.906250002048363257 ) ) ;
#27332=CARTESIAN_POINT ( 'NONE',  ( -9.999999999999998224, 1.224646799147353059E-15, -41.74999999999997868 ) ) ;
#27334=CARTESIAN_POINT ( 'NONE',  ( 10.81189881249999907, 6.242252689847868297, -163.2187500020483810 ) ) ;
#27337=CARTESIAN_POINT ( 'NONE',  ( 9.999999999999479527, 5.773502691896553074, -147.3750000000000000 ) ) ;
#27339=CARTESIAN_POINT ( 'NONE',  ( 5.000000000000000000, 8.660254037844385522, -199.7500000000000000 ) ) ;
#27344=CARTESIAN_POINT ( 'NONE',  ( 10.81189881249999551, -6.242252689847874514, -68.96875000204839523 ) ) ;
#27345=CARTESIAN_POINT ( 'NONE',  ( -10.81189881249999729, 6.242252689847871849, -78.90625000204838102 ) ) ;
#27347=CARTESIAN_POINT ( 'NONE',  ( -4.999999999999996447, 8.660254037844387298, -132.0000000000000000 ) ) ;
#27348=CARTESIAN_POINT ( 'NONE',  ( -10.81189881249999729, 6.242252689847871849, -156.9062500020483526 ) ) ;
#27349=CARTESIAN_POINT ( 'NONE',  ( -10.81189881249999729, 1.324075727343319199E-15, -171.7812500020484094 ) ) ;
#27351=CARTESIAN_POINT ( 'NONE',  ( 0.000000000000000000, 0.000000000000000000, -180.0000000000000000 ) ) ;
#27353=CARTESIAN_POINT ( 'NONE',  ( 10.81189881249999551, -6.242252689847874514, -109.4687500020483810 ) ) ;
#27356=CARTESIAN_POINT ( 'NONE',  ( 10.81189881249999907, 6.242252689847868297, -5.906250002048363257 ) ) ;
#27359=CARTESIAN_POINT ( 'NONE',  ( -2.293366432827344421E-15, -12.48450537969573659, -103.9062500020483810 ) ) ;
#27361=CARTESIAN_POINT ( 'NONE',  ( 9.999999999999998224, 0.000000000000000000, -77.37500000409677625 ) ) ;
#27363=CARTESIAN_POINT ( 'NONE',  ( -10.81189881249999729, 6.242252689847871849, -30.71875000204834905 ) ) ;
#27366=CARTESIAN_POINT ( 'NONE',  ( 10.81189881249999907, 6.242252689847868297, -29.90625000204835970 ) ) ;
#27370=CARTESIAN_POINT ( 'NONE',  ( 5.000000000000000000, 8.660254037844385522, -2.125000004096766482 ) ) ;
#27384=CARTESIAN_POINT ( 'NONE',  ( 9.999999999999998224, 0.000000000000000000, -108.4999999999999858 ) ) ;
#27386=CARTESIAN_POINT ( 'NONE',  ( 10.81189881249999729, 0.000000000000000000, -175.5312500020483810 ) ) ;
#27389=CARTESIAN_POINT ( 'NONE',  ( 10.81189881249999551, -6.242252689847874514, -92.96875000204838102 ) ) ;
#27391=CARTESIAN_POINT ( 'NONE',  ( -10.00000000000038547, 5.773502691896036154, -154.3749999999999716 ) ) ;
#27392=CARTESIAN_POINT ( 'NONE',  ( -10.81189881249999729, 1.324075727343319199E-15, -99.78125000204839523 ) ) ;
#27394=CARTESIAN_POINT ( 'NONE',  ( -10.81189881249999729, -6.242252689847864744, -106.9687500020483810 ) ) ;
#27396=ADVANCED_FACE ( 'NONE', ( #38789 ), #29089, .T. ) ;
#27397=CARTESIAN_POINT ( 'NONE',  ( 9.999999999999998224, 0.000000000000000000, -108.4999999999999858 ) ) ;
#27398=CARTESIAN_POINT ( 'NONE',  ( 7.070501591499376803E-16, 11.54700538379251284, -132.5000000040967905 ) ) ;
#27399=CARTESIAN_POINT ( 'NONE',  ( 5.405949406249992428, -9.363379034771808662, -198.2812500020484094 ) ) ;
#27402=CARTESIAN_POINT ( 'NONE',  ( -9.999999999999998224, 5.773502691896259087, -174.2500000040967905 ) ) ;
#27404=CARTESIAN_POINT ( 'NONE',  ( 10.81189881249999551, -6.242252689847874514, -17.96875000204836681 ) ) ;
#27406=CARTESIAN_POINT ( 'NONE',  ( -10.81189881249999729, 1.324075727343319199E-15, -129.5937500020483810 ) ) ;
#27408=CARTESIAN_POINT ( 'NONE',  ( -10.81189881249999729, 6.242252689847871849, -27.90625000204838102 ) ) ;
#27411=CARTESIAN_POINT ( 'NONE',  ( -5.000000000000003553, -8.660254037844383745, -60.99999999999997158 ) ) ;
#27412=CARTESIAN_POINT ( 'NONE',  ( 7.644554776091147741E-16, 12.48450537969573659, -124.1562500020483952 ) ) ;
#27414=VERTEX_POINT ( 'NONE', #25631 ) ;
#27416=CARTESIAN_POINT ( 'NONE',  ( -9.999999999999742428, -5.773502691896402084, -118.1249999999999858 ) ) ;
#27417=CARTESIAN_POINT ( 'NONE',  ( -4.999999999999996447, 8.660254037844387298, -103.8750000040967763 ) ) ;
#27420=CARTESIAN_POINT ( 'NONE',  ( 10.81189881249999551, -6.242252689847874514, -58.46875000204837391 ) ) ;
#27421=VERTEX_POINT ( 'NONE', #18285 ) ;
#27428=CARTESIAN_POINT ( 'NONE',  ( 10.00000000000000000, 5.773502691896255534, -29.25000000409675494 ) ) ;
#27434=ORIENTED_EDGE ( 'NONE', *, *, #34023, .F. ) ;
#27435=CARTESIAN_POINT ( 'NONE',  ( 0.000000000000000000, 0.000000000000000000, -99.99999999999998579 ) ) ;
#27438=CARTESIAN_POINT ( 'NONE',  ( 10.81189881249999729, 0.000000000000000000, -193.5312500020484094 ) ) ;
#27441=AXIS2_PLACEMENT_3D ( 'NONE', #3828, #33402, #3191 ) ;
#27443=AXIS2_PLACEMENT_3D ( 'NONE', #23147, #36310, #6742 ) ;
#27446=CARTESIAN_POINT ( 'NONE',  ( -5.405949406250003975, -9.363379034771801557, -117.3437500020483810 ) ) ;
#27447=CARTESIAN_POINT ( 'NONE',  ( 7.070501591499377789E-16, 11.54700538379251284, -195.5000000040968189 ) ) ;
#27448=CARTESIAN_POINT ( 'NONE',  ( -2.293366432827344421E-15, -12.48450537969573659, -127.9062500020483952 ) ) ;
#27450=CARTESIAN_POINT ( 'NONE',  ( 7.644554776091147741E-16, 12.48450537969573659, -126.9687500020483952 ) ) ;
#27453=CARTESIAN_POINT ( 'NONE',  ( -5.000000000000003553, -8.660254037844383745, -157.0000000000000000 ) ) ;
#27454=CARTESIAN_POINT ( 'NONE',  ( -9.999999999999998224, 1.224646799147353059E-15, -22.24999999999996447 ) ) ;
#27457=CARTESIAN_POINT ( 'NONE',  ( 4.999999999999992006, -8.660254037844389075, -158.6250000040967905 ) ) ;
#27459=CARTESIAN_POINT ( 'NONE',  ( 7.644554776091147741E-16, 12.48450537969573659, -45.96875000204836681 ) ) ;
#27461=CARTESIAN_POINT ( 'NONE',  ( -5.405949406250003975, -9.363379034771801557, -157.8437500020483810 ) ) ;
#27465=CARTESIAN_POINT ( 'NONE',  ( 10.00000000000000000, 5.773502691896255534, -82.87499999999997158 ) ) ;
#27467=EDGE_LOOP ( 'NONE', ( #35308, #33806, #9691, #30254 ) ) ;
#27468=CARTESIAN_POINT ( 'NONE',  ( 5.405949406249992428, -9.363379034771808662, -103.7812500020483810 ) ) ;
#27469=CARTESIAN_POINT ( 'NONE',  ( 5.000000000000000000, 8.660254037844385522, -120.6250000040967905 ) ) ;
#27472=CARTESIAN_POINT ( 'NONE',  ( -10.81189881249999729, 1.324075727343319199E-15, -53.28125000204836681 ) ) ;
#27473=CARTESIAN_POINT ( 'NONE',  ( -2.121150477449813534E-15, -11.54700538379251284, -135.8750000000000000 ) ) ;
#27485=ORIENTED_EDGE ( 'NONE', *, *, #23349, .T. ) ;
#27494=CARTESIAN_POINT ( 'NONE',  ( 10.81189881249999551, -6.242252689847874514, -137.9687500020483810 ) ) ;
#27495=CARTESIAN_POINT ( 'NONE',  ( 5.405949406249992428, -9.363379034771808662, -154.5937500020483810 ) ) ;
#27497=FACE_OUTER_BOUND ( 'NONE', #34546, .T. ) ;
#27498=CARTESIAN_POINT ( 'NONE',  ( 9.999999999999998224, 0.000000000000000000, -180.5000000000000000 ) ) ;
#27503=CARTESIAN_POINT ( 'NONE',  ( -10.81189881249999907, -6.242252689847864744, -178.9687500020484094 ) ) ;
#27505=AXIS2_PLACEMENT_3D ( 'NONE', #8552, #31868, #31433 ) ;
#27508=CARTESIAN_POINT ( 'NONE',  ( -5.405949406250003975, -9.363379034771801557, -44.03125000204838102 ) ) ;
#27510=CARTESIAN_POINT ( 'NONE',  ( -4.999999999999996447, 8.660254037844387298, -103.5000000000000000 ) ) ;
#27512=CARTESIAN_POINT ( 'NONE',  ( -2.293366432827344421E-15, -12.48450537969573659, -129.4062500020483810 ) ) ;
#27513=CARTESIAN_POINT ( 'NONE',  ( 4.999999999999992006, -8.660254037844389075, -148.1250000040967905 ) ) ;
#27514=CARTESIAN_POINT ( 'NONE',  ( 10.81189881249999729, 0.000000000000000000, -141.0312500020483810 ) ) ;
#27517=VERTEX_POINT ( 'NONE', #9429 ) ;
#27519=CARTESIAN_POINT ( 'NONE',  ( -5.405949406249996869, 9.363379034771805109, -177.8437500020483810 ) ) ;
#27521=CARTESIAN_POINT ( 'NONE',  ( -9.999999999999998224, 1.224646799147353059E-15, -158.7500000000000000 ) ) ;
#27522=CARTESIAN_POINT ( 'NONE',  ( -10.81189881249999729, 1.324075727343319199E-15, -72.78125000204838102 ) ) ;
#27524=CARTESIAN_POINT ( 'NONE',  ( 5.000000000000000000, 8.660254037844385522, -48.62500000409678336 ) ) ;
#27526=CARTESIAN_POINT ( 'NONE',  ( 10.81189881249999729, 0.000000000000000000, -11.84375000204834727 ) ) ;
#27528=CARTESIAN_POINT ( 'NONE',  ( -10.81189881249999907, -6.242252689847864744, -5.156250002048362369 ) ) ;
#27535=EDGE_CURVE ( 'NONE', #1789, #15268, #36392, .T. ) ;
#27539=FACE_OUTER_BOUND ( 'NONE', #4484, .T. ) ;
#27546=AXIS2_PLACEMENT_3D ( 'NONE', #29983, #20884, #1049 ) ;
#27549=CARTESIAN_POINT ( 'NONE',  ( -2.121150477449813534E-15, -11.54700538379251284, -41.37499999999996447 ) ) ;
#27551=CARTESIAN_POINT ( 'NONE',  ( -5.405949406250003975, -9.363379034771801557, -162.3437500020484094 ) ) ;
#27552=CARTESIAN_POINT ( 'NONE',  ( -10.81189881249999729, 6.242252689847871849, -177.7187500020484379 ) ) ;
#27556=DIRECTION ( 'NONE',  ( -0.000000000000000000, -0.000000000000000000, -1.000000000000000000 ) ) ;
#27558=LINE ( 'NONE', #8564, #12833 ) ;
#27561=CARTESIAN_POINT ( 'NONE',  ( -2.293366432827344421E-15, -12.48450537969573659, -72.21875000204835260 ) ) ;
#27562=CARTESIAN_POINT ( 'NONE',  ( 10.81189881249999729, 0.000000000000000000, -75.03125000204838102 ) ) ;
#27564=CARTESIAN_POINT ( 'NONE',  ( 10.00000000000000000, 5.773502691896255534, -133.8750000000000000 ) ) ;
#27565=CARTESIAN_POINT ( 'NONE',  ( -10.81189881249999729, 1.324075727343319199E-15, -158.2812500020484094 ) ) ;
#27566=CARTESIAN_POINT ( 'NONE',  ( 5.405949406249992428, -9.363379034771808662, -169.7812500020484094 ) ) ;
#27568=FACE_OUTER_BOUND ( 'NONE', #7053, .T. ) ;
#27569=CARTESIAN_POINT ( 'NONE',  ( 10.81189881249999907, 6.242252689847868297, -106.2187500020483668 ) ) ;
#27570=DIRECTION ( 'NONE',  ( -1.000000000000000000, 0.000000000000000000, 0.000000000000000000 ) ) ;
#27572=CARTESIAN_POINT ( 'NONE',  ( -5.405949406250003975, -9.363379034771801557, -2.031250002048373915 ) ) ;
#27575=CARTESIAN_POINT ( 'NONE',  ( -5.405949406249996869, 9.363379034771805109, -103.0312500020483952 ) ) ;
#27577=CARTESIAN_POINT ( 'NONE',  ( 10.00000000000000000, 5.773502691896255534, -78.75000000409679046 ) ) ;
#27579=CARTESIAN_POINT ( 'NONE',  ( -5.405949406249996869, 9.363379034771805109, -30.84375000204836326 ) ) ;
#27582=CARTESIAN_POINT ( 'NONE',  ( 5.405949406249992428, -9.363379034771808662, -25.78125000204836681 ) ) ;
#27585=CARTESIAN_POINT ( 'NONE',  ( 9.999999999999998224, 0.000000000000000000, -6.875000004096742501 ) ) ;
#27598=LINE ( 'NONE', #31058, #14614 ) ;
#27599=CARTESIAN_POINT ( 'NONE',  ( 1.351487262974977233, 10.72709830801206543, -100.0000000000000000 ) ) ;
#27600=CARTESIAN_POINT ( 'NONE',  ( 9.999999999999998224, 0.000000000000000000, -156.8750000040967905 ) ) ;
#27601=CARTESIAN_POINT ( 'NONE',  ( 10.81189881249999729, 0.000000000000000000, -171.0312500020484094 ) ) ;
#27605=CARTESIAN_POINT ( 'NONE',  ( -5.405949406249996869, 9.363379034771805109, -92.34375000204838102 ) ) ;
#27607=CARTESIAN_POINT ( 'NONE',  ( -5.405949406249996869, 9.363379034771805109, -198.8437500020484094 ) ) ;
#27608=CARTESIAN_POINT ( 'NONE',  ( -10.81189881249999729, 6.242252689847871849, -98.40625000204838102 ) ) ;
#27610=CARTESIAN_POINT ( 'NONE',  ( 10.81189881249999729, 6.242252689847867408, -106.2187500020483810 ) ) ;
#27613=CARTESIAN_POINT ( 'NONE',  ( 10.70731569305653252, 1.500182182591227154, -180.0000000000000284 ) ) ;
#27614=CARTESIAN_POINT ( 'NONE',  ( -5.405949406249996869, 9.363379034771805109, -196.0312500020484094 ) ) ;
#27616=CARTESIAN_POINT ( 'NONE',  ( 9.999999999999998224, 0.000000000000000000, -171.8750000040968189 ) ) ;
#27618=CARTESIAN_POINT ( 'NONE',  ( 5.405949406249992428, -9.363379034771808662, -22.59375000204835615 ) ) ;
#27619=CARTESIAN_POINT ( 'NONE',  ( 8.614196012144985204, -6.533971456632194474, -180.0000000000000000 ) ) ;
#27620=CARTESIAN_POINT ( 'NONE',  ( 7.644554776091147741E-16, 12.48450537969573659, -126.9687500020483668 ) ) ;
#27622=CARTESIAN_POINT ( 'NONE',  ( -10.81189881249999729, 1.324075727343319199E-15, -26.28125000204836681 ) ) ;
#27626=CARTESIAN_POINT ( 'NONE',  ( 7.070501591499377789E-16, 11.54700538379251284, -54.12499999999997868 ) ) ;
#27627=CARTESIAN_POINT ( 'NONE',  ( -10.81189881249999729, 1.324075727343319199E-15, -125.2812500020483668 ) ) ;
#27630=CARTESIAN_POINT ( 'NONE',  ( -9.999999999999998224, 1.224646799147353059E-15, -103.6250000040967763 ) ) ;
#27633=CARTESIAN_POINT ( 'NONE',  ( 10.81189881249999729, 0.000000000000000000, -56.84375000204835970 ) ) ;
#27634=ORIENTED_EDGE ( 'NONE', *, *, #11435, .F. ) ;
#27639=CARTESIAN_POINT ( 'NONE',  ( 9.999999999999996447, -5.773502691896262640, -26.50000000409677270 ) ) ;
#27648=CARTESIAN_POINT ( 'NONE',  ( 9.999999999999479527, 5.773502691896553074, -174.7500000040967905 ) ) ;
#27650=CARTESIAN_POINT ( 'NONE',  ( 5.405949406249992428, -9.363379034771808662, -193.7812500020484094 ) ) ;
#27656=CARTESIAN_POINT ( 'NONE',  ( 10.81189881249999729, 0.000000000000000000, -115.3437500020483810 ) ) ;
#27657=CARTESIAN_POINT ( 'NONE',  ( -9.999999999999998224, 1.224646799147353059E-15, -196.6250000040967905 ) ) ;
#27658=CARTESIAN_POINT ( 'NONE',  ( -5.405949406250003975, -9.363379034771801557, -122.0312500020483952 ) ) ;
#27660=CARTESIAN_POINT ( 'NONE',  ( 10.81189881249999729, 6.242252689847867408, -133.2187500020483810 ) ) ;
#27661=EDGE_CURVE ( 'NONE', #35515, #7848, #39615, .T. ) ;
#27663=CARTESIAN_POINT ( 'NONE',  ( 4.999999999999992006, -8.660254037844389075, -166.1250000040967905 ) ) ;
#27664=( BOUNDED_CURVE ( )  B_SPLINE_CURVE ( 2, ( #37039, #800, #17380, #40681, #17168, #30580, #27977 ),
 .UNSPECIFIED., .F., .F. ) 
 B_SPLINE_CURVE_WITH_KNOTS ( ( 3, 2, 2, 3 ),
 ( 0.3843283582089552786, 0.3855721393034826638, 0.3868159203980099936, 0.3880597014925373789 ),
 .UNSPECIFIED. ) 
 CURVE ( )  GEOMETRIC_REPRESENTATION_ITEM ( )  RATIONAL_B_SPLINE_CURVE ( ( 0.9999999999999940048, 0.8660254037844447028, 1.000000000000000000, 0.8660254037844387076, 1.000000000000000000, 0.8660254037844327124, 1.000000000000005995 ) ) 
 REPRESENTATION_ITEM ( '' )  );
#27665=CARTESIAN_POINT ( 'NONE',  ( -9.999999999999998224, 1.224646799147353059E-15, -109.6250000040967763 ) ) ;
#27666=CARTESIAN_POINT ( 'NONE',  ( -9.999999999999998224, 1.224646799147353059E-15, -145.2500000000000000 ) ) ;
#27667=CARTESIAN_POINT ( 'NONE',  ( -9.999999999999998224, 5.773502691896259087, -23.87499999999998224 ) ) ;
#27673=CARTESIAN_POINT ( 'NONE',  ( -5.405949406249996869, 9.363379034771805109, -47.34375000204838102 ) ) ;
#27674=CARTESIAN_POINT ( 'NONE',  ( -9.999999999999872102, -5.773502691896326589, -163.5000000040967620 ) ) ;
#27675=CARTESIAN_POINT ( 'NONE',  ( -5.405949406249996869, 9.363379034771805109, -152.3437500020483810 ) ) ;
#27678=CARTESIAN_POINT ( 'NONE',  ( 9.602216827598432758, 4.693292424609470714, -179.9999999999999432 ) ) ;
#27679=CARTESIAN_POINT ( 'NONE',  ( -5.000000000000003553, -8.660254037844383745, -84.99999999999997158 ) ) ;
#27682=CARTESIAN_POINT ( 'NONE',  ( -10.81189881249999729, -6.242252689847864744, -105.6562500020483952 ) ) ;
#27683=CARTESIAN_POINT ( 'NONE',  ( -10.00000000000000000, -5.773502691896251982, -124.5000000040967620 ) ) ;
#27684=CARTESIAN_POINT ( 'NONE',  ( 10.00000000000025402, -5.773502691896113426, -154.0000000040967905 ) ) ;
#27687=CARTESIAN_POINT ( 'NONE',  ( -5.405949406249996869, 9.363379034771805109, -47.53125000204838813 ) ) ;
#27692=CARTESIAN_POINT ( 'NONE',  ( -9.999999999999998224, 1.224646799147353059E-15, -176.7500000000000284 ) ) ;
#27694=CIRCLE ( 'NONE', #7021, 24.99999999999999645 ) ;
#27698=VERTEX_POINT ( 'NONE', #3379 ) ;
#27708=CARTESIAN_POINT ( 'NONE',  ( -5.405949406250003975, -9.363379034771801557, -142.8437500020483810 ) ) ;
#27709=CARTESIAN_POINT ( 'NONE',  ( -10.81189881249999729, 6.242252689847871849, -149.4062500020484094 ) ) ;
#27710=CARTESIAN_POINT ( 'NONE',  ( 10.81189881249999729, 6.242252689847867408, -157.2187500020483810 ) ) ;
#27712=CARTESIAN_POINT ( 'NONE',  ( 9.999999999999998224, 0.000000000000000000, -138.8750000040968189 ) ) ;
#27713=CARTESIAN_POINT ( 'NONE',  ( -4.999999999999996447, 8.660254037844387298, -180.0000000000000000 ) ) ;
#27718=EDGE_CURVE ( 'NONE', #23938, #16772, #25161, .T. ) ;
#27719=CARTESIAN_POINT ( 'NONE',  ( -5.405949406249996869, 9.363379034771805109, -179.3437500020483810 ) ) ;
#27723=CARTESIAN_POINT ( 'NONE',  ( -5.405949406250003975, -9.363379034771801557, -47.03125000204838813 ) ) ;
#27725=CARTESIAN_POINT ( 'NONE',  ( -5.000000000000003553, -8.660254037844383745, -105.9999999999999858 ) ) ;
#27727=CARTESIAN_POINT ( 'NONE',  ( 5.405949406249999534, 9.363379034771803333, -127.2812500020483810 ) ) ;
#27728=CARTESIAN_POINT ( 'NONE',  ( -9.999999999999998224, 5.773502691896259087, -147.2500000040967905 ) ) ;
#27733=CARTESIAN_POINT ( 'NONE',  ( 10.81189881249999729, 0.000000000000000000, -172.3437500020484094 ) ) ;
#27735=CARTESIAN_POINT ( 'NONE',  ( -9.999999999999998224, 1.224646799147353059E-15, -163.6250000040967905 ) ) ;
#27737=CARTESIAN_POINT ( 'NONE',  ( -5.405949406250003975, -9.363379034771801557, -68.03125000204838102 ) ) ;
#27739=CARTESIAN_POINT ( 'NONE',  ( 5.000000000000000000, 8.660254037844385522, -45.62500000409677625 ) ) ;
#27740=CARTESIAN_POINT ( 'NONE',  ( 7.644554776091147741E-16, 12.48450537969573659, -2.468750002048353043 ) ) ;
#27760=CARTESIAN_POINT ( 'NONE',  ( 9.999999999999996447, -5.773502691896262640, -47.12499999999997868 ) ) ;
#27762=CARTESIAN_POINT ( 'NONE',  ( -5.405949406249996869, 9.363379034771805109, -162.8437500020484094 ) ) ;
#27763=CARTESIAN_POINT ( 'NONE',  ( 5.405949406249992428, -9.363379034771808662, -178.5937500020484094 ) ) ;
#27766=DIRECTION ( 'NONE',  ( 1.000000000000000000, 0.000000000000000000, 0.000000000000000000 ) ) ;
#27773=CARTESIAN_POINT ( 'NONE',  ( 5.405949406249999534, 9.363379034771803333, -59.59375000204835970 ) ) ;
#27775=CARTESIAN_POINT ( 'NONE',  ( 10.81189881249999729, 0.000000000000000000, -69.03125000204838102 ) ) ;
#27777=CARTESIAN_POINT ( 'NONE',  ( -10.00000000000000000, -5.773502691896251982, -134.6250000000000000 ) ) ;
#27779=CARTESIAN_POINT ( 'NONE',  ( -10.81189881249999729, 6.242252689847871849, -153.9062500020483810 ) ) ;
#27780=CARTESIAN_POINT ( 'NONE',  ( 5.405949406249992428, -9.363379034771808662, -168.2812500020484094 ) ) ;
#27783=CARTESIAN_POINT ( 'NONE',  ( -10.81189881249999729, 6.242252689847871849, -98.21875000204838102 ) ) ;
#27784=LINE ( 'NONE', #14373, #3172 ) ;
#27786=CARTESIAN_POINT ( 'NONE',  ( -5.405949406249996869, 9.363379034771805109, 0.4687499979516285276 ) ) ;
#27788=CARTESIAN_POINT ( 'NONE',  ( 9.999999999999998224, 0.000000000000000000, -132.8750000040967905 ) ) ;
#27790=CARTESIAN_POINT ( 'NONE',  ( -10.81189881249999729, 6.242252689847871849, -101.4062500020483952 ) ) ;
#27793=CARTESIAN_POINT ( 'NONE',  ( -9.999999999999998224, 5.773502691896259087, -75.25000000409677625 ) ) ;
#27795=CARTESIAN_POINT ( 'NONE',  ( 10.81189881249999729, 0.000000000000000000, -22.34375000204835615 ) ) ;
#27798=CARTESIAN_POINT ( 'NONE',  ( -2.293366432827344421E-15, -12.48450537969573659, -31.90625000204835970 ) ) ;
#27801=CARTESIAN_POINT ( 'NONE',  ( 10.00000000000000000, 5.773502691896255534, -2.250000004096752715 ) ) ;
#27816=CARTESIAN_POINT ( 'NONE',  ( -9.999999999999479527, -5.773502691896549521, -109.1249999999999716 ) ) ;
#27818=CARTESIAN_POINT ( 'NONE',  ( 10.81189881249999551, -6.242252689847874514, -166.6562500020484094 ) ) ;
#27819=CARTESIAN_POINT ( 'NONE',  ( 1.351487262974977233, 10.72709830801206543, -100.0000000000000000 ) ) ;
#27821=CARTESIAN_POINT ( 'NONE',  ( -10.81189881249999907, -6.242252689847864744, -87.46875000204838102 ) ) ;
#27823=CARTESIAN_POINT ( 'NONE',  ( 10.81189881249999551, -6.242252689847874514, -193.4687500020484094 ) ) ;
#27824=CARTESIAN_POINT ( 'NONE',  ( 10.81189881249999551, -6.242252689847874514, -88.65625000204838102 ) ) ;
#27826=CARTESIAN_POINT ( 'NONE',  ( -5.405949406250003975, -9.363379034771801557, -105.3437500020483810 ) ) ;
#27828=EDGE_CURVE ( 'NONE', #18233, #36337, #41124, .T. ) ;
#27830=CARTESIAN_POINT ( 'NONE',  ( 10.81189881249999729, 6.242252689847867408, -170.9062500020484094 ) ) ;
#27831=CARTESIAN_POINT ( 'NONE',  ( 10.81189881249999551, -6.242252689847874514, -184.6562500020484094 ) ) ;
#27833=CARTESIAN_POINT ( 'NONE',  ( 7.070501591499377789E-16, 11.54700538379251284, -173.0000000040967905 ) ) ;
#27835=CARTESIAN_POINT ( 'NONE',  ( 5.405949406249992428, -9.363379034771808662, -19.59375000204835615 ) ) ;
#27837=CARTESIAN_POINT ( 'NONE',  ( 5.405949406249999534, 9.363379034771803333, -124.0937500020483952 ) ) ;
#27839=CARTESIAN_POINT ( 'NONE',  ( 7.644554776091147741E-16, 12.48450537969573659, -25.15625000204837747 ) ) ;
#27842=CARTESIAN_POINT ( 'NONE',  ( 4.999999999999992006, -8.660254037844389075, -48.74999999999998579 ) ) ;
#27843=CARTESIAN_POINT ( 'NONE',  ( 5.405949406249999534, 9.363379034771803333, -122.7812500020483952 ) ) ;
#27846=CARTESIAN_POINT ( 'NONE',  ( 5.000000000000000000, 8.660254037844385522, -102.6250000040967905 ) ) ;
#27847=CARTESIAN_POINT ( 'NONE',  ( -9.999999999999479527, -5.773502691896549521, -113.6249999999999716 ) ) ;
#27849=CARTESIAN_POINT ( 'NONE',  ( -10.81189881249999729, 1.324075727343319199E-15, -57.59375000204835970 ) ) ;
#27854=FACE_OUTER_BOUND ( 'NONE', #28724, .T. ) ;
#27855=CARTESIAN_POINT ( 'NONE',  ( 4.999999999999992006, -8.660254037844389075, -29.62500000409676204 ) ) ;
#27867=CARTESIAN_POINT ( 'NONE',  ( -5.405949406250003975, -9.363379034771801557, -191.0312500020484094 ) ) ;
#27874=CARTESIAN_POINT ( 'NONE',  ( 5.405949406249992428, -9.363379034771808662, -121.5937500020483952 ) ) ;
#27876=CARTESIAN_POINT ( 'NONE',  ( -10.81189881249999729, 6.242252689847871849, -125.4062500020483810 ) ) ;
#27878=CARTESIAN_POINT ( 'NONE',  ( 10.81189881249999729, 0.000000000000000000, -133.3437500020484094 ) ) ;
#27881=CARTESIAN_POINT ( 'NONE',  ( -5.000000000000003553, -8.660254037844383745, -148.0000000000000000 ) ) ;
#27882=CARTESIAN_POINT ( 'NONE',  ( 4.999999999999992006, -8.660254037844389075, -20.24999999999996092 ) ) ;
#27887=CARTESIAN_POINT ( 'NONE',  ( 10.81189881249999551, -6.242252689847874514, -41.96875000204836681 ) ) ;
#27889=CARTESIAN_POINT ( 'NONE',  ( -2.293366432827344421E-15, -12.48450537969573659, -156.2187500020483810 ) ) ;
#27892=CARTESIAN_POINT ( 'NONE',  ( 8.928897960546947843, 5.779144828205879492, -179.9999999999999716 ) ) ;
#27893=CARTESIAN_POINT ( 'NONE',  ( 5.000000000000000000, 8.660254037844385522, -73.74999999999998579 ) ) ;
#27896=CARTESIAN_POINT ( 'NONE',  ( -5.405949406250003975, -9.363379034771801557, -101.0312500020483952 ) ) ;
#27897=CARTESIAN_POINT ( 'NONE',  ( 9.999999999999998224, 0.000000000000000000, -126.8750000040967905 ) ) ;
#27898=CARTESIAN_POINT ( 'NONE',  ( 4.999999999999992006, -8.660254037844389075, -143.6250000040967905 ) ) ;
#27899=CARTESIAN_POINT ( 'NONE',  ( 5.405949406249999534, 9.363379034771803333, -83.59375000204836681 ) ) ;
#27902=CARTESIAN_POINT ( 'NONE',  ( 5.405949406249992428, -9.363379034771808662, -43.78125000204838102 ) ) ;
#27907=ADVANCED_BREP_SHAPE_REPRESENTATION ( '', ( #28380, #39998 ), #29026 ) ;
#27913=CARTESIAN_POINT ( 'NONE',  ( 9.999999999999998224, 0.000000000000000000, -165.5000000000000000 ) ) ;
#27922=CARTESIAN_POINT ( 'NONE',  ( 7.644554776091147741E-16, 12.48450537969573659, -140.4687500020483810 ) ) ;
#27924=CARTESIAN_POINT ( 'NONE',  ( -2.293366432827344421E-15, -12.48450537969573659, -148.9062500020483810 ) ) ;
#27925=CARTESIAN_POINT ( 'NONE',  ( 10.81189881249999729, 6.242252689847867408, -152.7187500020483810 ) ) ;
#27927=( BOUNDED_CURVE ( )  B_SPLINE_CURVE ( 2, ( #624, #20024, #12900, #26516, #19809, #13110, #40088 ),
 .UNSPECIFIED., .F., .F. ) 
 B_SPLINE_CURVE_WITH_KNOTS ( ( 3, 2, 2, 3 ),
 ( 0.2611940298507463565, 0.2624378109452737418, 0.2636815920398011270, 0.2649253731343284568 ),
 .UNSPECIFIED. ) 
 CURVE ( )  GEOMETRIC_REPRESENTATION_ITEM ( )  RATIONAL_B_SPLINE_CURVE ( ( 0.9999999999999880096, 0.8660254037844506980, 1.000000000000000000, 0.8660254037844387076, 1.000000000000000000, 0.8660254037844267172, 1.000000000000011990 ) ) 
 REPRESENTATION_ITEM ( '' )  );
#27929=CARTESIAN_POINT ( 'NONE',  ( 9.999999999999996447, -5.773502691896262640, -168.6250000000000000 ) ) ;
#27933=CARTESIAN_POINT ( 'NONE',  ( -9.999999999999479527, -5.773502691896549521, -149.6249999999999716 ) ) ;
#27934=CARTESIAN_POINT ( 'NONE',  ( -10.81189881249999907, -6.242252689847864744, -180.4687500020484094 ) ) ;
#27937=CARTESIAN_POINT ( 'NONE',  ( 0.000000000000000000, 0.000000000000000000, -99.99999999999998579 ) ) ;
#27938=CARTESIAN_POINT ( 'NONE',  ( 5.405949406249992428, -9.363379034771808662, -42.28125000204838102 ) ) ;
#27940=CARTESIAN_POINT ( 'NONE',  ( -9.999999999999998224, 1.224646799147353059E-15, -95.74999999999998579 ) ) ;
#27941=EDGE_CURVE ( 'NONE', #28436, #41419, #33801, .T. ) ;
#27944=CARTESIAN_POINT ( 'NONE',  ( 7.644554776091147741E-16, 12.48450537969573659, -124.1562500020483810 ) ) ;
#27945=CARTESIAN_POINT ( 'NONE',  ( 5.000000000000000000, 8.660254037844385522, -149.1250000040967905 ) ) ;
#27949=CARTESIAN_POINT ( 'NONE',  ( -5.405949406250003975, -9.363379034771801557, -174.3437500020484094 ) ) ;
#27951=DIRECTION ( 'NONE',  ( -0.000000000000000000, -0.000000000000000000, -1.000000000000000000 ) ) ;
#27953=CARTESIAN_POINT ( 'NONE',  ( -5.405949406250003975, -9.363379034771801557, -71.03125000204838102 ) ) ;
#27955=CARTESIAN_POINT ( 'NONE',  ( 9.999999999999998224, 0.000000000000000000, -45.87500000409677625 ) ) ;
#27956=CARTESIAN_POINT ( 'NONE',  ( 5.405949406249999534, 9.363379034771803333, -1.093750002048365921 ) ) ;
#27966=ORIENTED_EDGE ( 'NONE', *, *, #24327, .F. ) ;
#27969=DIRECTION ( 'NONE',  ( -0.000000000000000000, -0.000000000000000000, -1.000000000000000000 ) ) ;
#27977=CARTESIAN_POINT ( 'NONE',  ( 9.999999999999998224, 0.000000000000000000, -122.0000000000000000 ) ) ;
#27978=CARTESIAN_POINT ( 'NONE',  ( 7.070501591499377789E-16, 11.54700538379251284, -36.12499999999996447 ) ) ;
#27980=CARTESIAN_POINT ( 'NONE',  ( 5.405949406249992428, -9.363379034771808662, -166.5937500020484094 ) ) ;
#27981=CARTESIAN_POINT ( 'NONE',  ( 10.81189881249999551, -3.636584649182867057, -179.9165719629227169 ) ) ;
#27985=CARTESIAN_POINT ( 'NONE',  ( -2.121150477449813534E-15, -11.54700538379251284, -197.3750000000000284 ) ) ;
#27990=CARTESIAN_POINT ( 'NONE',  ( -10.81189881249999729, 1.324075727343319199E-15, -62.09375000204836681 ) ) ;
#27992=CARTESIAN_POINT ( 'NONE',  ( -10.81189881249999729, 6.242252689847871849, -68.40625000204839523 ) ) ;
#27994=CARTESIAN_POINT ( 'NONE',  ( -2.121150477449813534E-15, -11.54700538379251284, -134.3750000000000000 ) ) ;
#27995=CARTESIAN_POINT ( 'NONE',  ( -2.293366432827344421E-15, -12.48450537969573659, -150.4062500020484379 ) ) ;
#27996=CARTESIAN_POINT ( 'NONE',  ( 5.405949406249992428, -9.363379034771808662, -166.7812500020484094 ) ) ;
#27999=CARTESIAN_POINT ( 'NONE',  ( 7.644554776091147741E-16, 12.48450537969573659, -96.96875000204838102 ) ) ;
#28002=CARTESIAN_POINT ( 'NONE',  ( -2.293366432827344421E-15, -12.48450537969573659, -0.4062500020483583718 ) ) ;
#28006=CARTESIAN_POINT ( 'NONE',  ( 10.81189881249999729, 0.000000000000000000, -90.03125000204838102 ) ) ;
#28009=CARTESIAN_POINT ( 'NONE',  ( 4.999999999999992006, -8.660254037844389075, -71.62500000409677625 ) ) ;
#28011=CARTESIAN_POINT ( 'NONE',  ( -10.81189881249999729, 6.242252689847871849, -26.21875000204837391 ) ) ;
#28014=CARTESIAN_POINT ( 'NONE',  ( -5.405949406250003975, -9.363379034771801557, -18.53125000204835970 ) ) ;
#28017=CARTESIAN_POINT ( 'NONE',  ( -2.121150477449813534E-15, -11.54700538379251284, 0.2499999959032495056 ) ) ;
#28025=EDGE_CURVE ( 'NONE', #40993, #41044, #7897, .T. ) ;
#28026=ORIENTED_EDGE ( 'NONE', *, *, #8053, .F. ) ;
#28027=ADVANCED_FACE ( 'NONE', ( #24310 ), #20401, .F. ) ;
#28034=CARTESIAN_POINT ( 'NONE',  ( -2.121150477449813534E-15, -11.54700538379251284, -108.8749999999999858 ) ) ;
#28036=CARTESIAN_POINT ( 'NONE',  ( -10.81189881249999729, 6.242252689847871849, -167.4062500020483810 ) ) ;
#28037=DIRECTION ( 'NONE',  ( -0.000000000000000000, -0.000000000000000000, -1.000000000000000000 ) ) ;
#28040=CARTESIAN_POINT ( 'NONE',  ( -5.405949406250003975, -9.363379034771801557, -87.34375000204836681 ) ) ;
#28042=CARTESIAN_POINT ( 'NONE',  ( 5.405949406249999534, 9.363379034771803333, -191.5937500020484094 ) ) ;
#28043=CARTESIAN_POINT ( 'NONE',  ( 7.644554776091147741E-16, 12.48450537969573659, -94.15625000204839523 ) ) ;
#28048=CARTESIAN_POINT ( 'NONE',  ( 5.405949406249999534, 9.363379034771803333, -173.7812500020484094 ) ) ;
#28049=CARTESIAN_POINT ( 'NONE',  ( 10.81189881249999729, 0.000000000000000000, -192.0312500020484094 ) ) ;
#28051=CARTESIAN_POINT ( 'NONE',  ( 10.00000000000000000, 5.773502691896255534, -164.2500000040967905 ) ) ;
#28053=CARTESIAN_POINT ( 'NONE',  ( -5.405949406249996869, 9.363379034771805109, -15.84375000204835082 ) ) ;
#28054=FACE_OUTER_BOUND ( 'NONE', #41434, .T. ) ;
#28055=CARTESIAN_POINT ( 'NONE',  ( 7.644554776091147741E-16, 12.48450537969573659, -125.4687500020483952 ) ) ;
#28057=CARTESIAN_POINT ( 'NONE',  ( -10.81189881249999729, 6.242252689847871849, -18.90625000204837391 ) ) ;
#28060=CARTESIAN_POINT ( 'NONE',  ( -9.999999999999998224, 1.224646799147353059E-15, -53.74999999999996447 ) ) ;
#28061=CARTESIAN_POINT ( 'NONE',  ( 7.644554776091147741E-16, 12.48450537969573659, -113.6562500020483952 ) ) ;
#28063=ORIENTED_EDGE ( 'NONE', *, *, #4849, .F. ) ;
#28064=CARTESIAN_POINT ( 'NONE',  ( 10.00000000000000000, 5.773502691896255534, -90.75000000409677625 ) ) ;
#28067=CARTESIAN_POINT ( 'NONE',  ( -2.293366432827344421E-15, -12.48450537969573659, -49.71875000204836681 ) ) ;
#28074=CARTESIAN_POINT ( 'NONE',  ( -5.000000000000003553, -8.660254037844383745, -28.37500000409676204 ) ) ;
#28075=DIRECTION ( 'NONE',  ( -0.000000000000000000, -0.000000000000000000, -1.000000000000000000 ) ) ;
#28086=ORIENTED_EDGE ( 'NONE', *, *, #37948, .F. ) ;
#28089=CYLINDRICAL_SURFACE ( 'NONE', #11823, 9.999999999999998224 ) ;
#28091=CARTESIAN_POINT ( 'NONE',  ( 10.81189881249999729, 0.000000000000000000, -187.5312500020484094 ) ) ;
#28097=CARTESIAN_POINT ( 'NONE',  ( -10.81189881249999729, 1.324075727343319199E-15, -108.5937500020483810 ) ) ;
#28099=CARTESIAN_POINT ( 'NONE',  ( -10.81189881249999729, 1.324075727343319199E-15, -119.2812500020483952 ) ) ;
#28101=CARTESIAN_POINT ( 'NONE',  ( -5.405949406249996869, 9.363379034771805109, -129.8437500020484094 ) ) ;
#28104=CARTESIAN_POINT ( 'NONE',  ( 9.999999999999996447, -5.773502691896262640, -150.6250000000000000 ) ) ;
#28105=CARTESIAN_POINT ( 'NONE',  ( -4.999999999999996447, 8.660254037844387298, -10.49999999999995381 ) ) ;
#28108=CARTESIAN_POINT ( 'NONE',  ( -9.999999999999998224, 1.224646799147353059E-15, -187.6250000040967905 ) ) ;
#28111=CARTESIAN_POINT ( 'NONE',  ( 10.81189881249999551, -6.242252689847874514, -34.46875000204835260 ) ) ;
#28113=CARTESIAN_POINT ( 'NONE',  ( 10.81189881249999907, 6.242252689847868297, -143.7187500020483810 ) ) ;
#28116=CARTESIAN_POINT ( 'NONE',  ( -10.00000000000000000, -5.773502691896251982, -79.12499999999998579 ) ) ;
#28119=CARTESIAN_POINT ( 'NONE',  ( -5.405949406249996869, 9.363379034771805109, -100.0312500020483952 ) ) ;
#28120=CARTESIAN_POINT ( 'NONE',  ( -2.121150477449813534E-15, -11.54700538379251284, -125.7500000040967763 ) ) ;
#28122=CARTESIAN_POINT ( 'NONE',  ( -10.81189881249999729, 1.324075727343319199E-15, -74.09375000204838102 ) ) ;
#28125=CARTESIAN_POINT ( 'NONE',  ( -5.405949406249996869, 9.363379034771805109, -41.53125000204838102 ) ) ;
#28126=CARTESIAN_POINT ( 'NONE',  ( 9.999999999999998224, 0.000000000000000000, -150.5000000000000000 ) ) ;
#28129=CARTESIAN_POINT ( 'NONE',  ( 5.000000000000000000, 8.660254037844385522, -165.6250000040967905 ) ) ;
#28130=CARTESIAN_POINT ( 'NONE',  ( 9.999999999999998224, 0.000000000000000000, -120.5000000000000000 ) ) ;
#28140=ADVANCED_FACE ( 'NONE', ( #18656 ), #24951, .F. ) ;
#28144=CARTESIAN_POINT ( 'NONE',  ( 5.405949406249992428, -9.363379034771808662, -135.0937500020483810 ) ) ;
#28145=CARTESIAN_POINT ( 'NONE',  ( -2.293366432827344421E-15, -12.48450537969573659, -138.4062500020483810 ) ) ;
#28146=CARTESIAN_POINT ( 'NONE',  ( 5.405949406249999534, 9.363379034771803333, -152.5937500020483810 ) ) ;
#28147=CARTESIAN_POINT ( 'NONE',  ( -10.00000000000076916, 5.773502691895813221, -127.3749999999999858 ) ) ;
#28148=CARTESIAN_POINT ( 'NONE',  ( 9.999999999999998224, 0.000000000000000000, -170.0000000000000000 ) ) ;
#28152=CARTESIAN_POINT ( 'NONE',  ( -10.43766569794794208, -0.1000697250298307195, -99.99999999999998579 ) ) ;
#28153=CARTESIAN_POINT ( 'NONE',  ( 5.405949406249999534, 9.363379034771803333, -172.0937500020484094 ) ) ;
#28157=CARTESIAN_POINT ( 'NONE',  ( 10.81189881249999907, 6.242252689847868297, -47.90625000204837391 ) ) ;
#28159=CARTESIAN_POINT ( 'NONE',  ( -2.121150477449813534E-15, -11.54700538379251284, -98.37500000000000000 ) ) ;
#28160=ORIENTED_EDGE ( 'NONE', *, *, #24079, .F. ) ;
#28161=CARTESIAN_POINT ( 'NONE',  ( -5.405949406249996869, 9.363379034771805109, -125.5312500020483952 ) ) ;
#28162=CARTESIAN_POINT ( 'NONE',  ( -9.999999999999998224, 1.224646799147353059E-15, -151.6250000040967905 ) ) ;
#28166=CARTESIAN_POINT ( 'NONE',  ( -5.405949406249996869, 9.363379034771805109, -176.3437500020483810 ) ) ;
#28169=CARTESIAN_POINT ( 'NONE',  ( -2.121150477449813534E-15, -11.54700538379251284, -165.8750000000000000 ) ) ;
#28171=CARTESIAN_POINT ( 'NONE',  ( -10.81189881249999729, 6.242252689847871849, -68.40625000204839523 ) ) ;
#28172=CARTESIAN_POINT ( 'NONE',  ( -5.000000000000003553, -8.660254037844383745, -40.37500000409677625 ) ) ;
#28173=CARTESIAN_POINT ( 'NONE',  ( 5.405949406249992428, -9.363379034771808662, -6.093750002048370362 ) ) ;
#28187=VERTEX_POINT ( 'NONE', #5083 ) ;
#28192=( BOUNDED_CURVE ( )  B_SPLINE_CURVE ( 2, ( #24355, #31258, #37497, #14813, #21090, #10731, #34278 ),
 .UNSPECIFIED., .F., .F. ) 
 B_SPLINE_CURVE_WITH_KNOTS ( ( 3, 2, 2, 3 ),
 ( 0.3208955223880597396, 0.3221393034825871804, 0.3233830845771145657, 0.3246268656716419510 ),
 .UNSPECIFIED. ) 
 CURVE ( )  GEOMETRIC_REPRESENTATION_ITEM ( )  RATIONAL_B_SPLINE_CURVE ( ( 0.9999999999999940048, 0.8660254037844447028, 1.000000000000000000, 0.8660254037844387076, 1.000000000000000000, 0.8660254037844207220, 1.000000000000017986 ) ) 
 REPRESENTATION_ITEM ( '' )  );
#28195=CARTESIAN_POINT ( 'NONE',  ( -4.999999999999996447, 8.660254037844387298, -112.4999999999999858 ) ) ;
#28196=CARTESIAN_POINT ( 'NONE',  ( 4.999999999999992006, -8.660254037844389075, -39.74999999999997868 ) ) ;
#28199=CARTESIAN_POINT ( 'NONE',  ( 10.81189881249999729, 0.000000000000000000, -154.3437500020483810 ) ) ;
#28203=CARTESIAN_POINT ( 'NONE',  ( 9.999999999999996447, -5.773502691896262640, -197.1250000000000284 ) ) ;
#28208=CARTESIAN_POINT ( 'NONE',  ( -5.405949406250003975, -9.363379034771801557, -65.03125000204838102 ) ) ;
#28210=CARTESIAN_POINT ( 'NONE',  ( 10.00000000000000000, 5.773502691896255534, -124.8750000000000000 ) ) ;
#28213=CARTESIAN_POINT ( 'NONE',  ( -10.81189881249999729, -6.242252689847864744, -152.1562500020484094 ) ) ;
#28214=CARTESIAN_POINT ( 'NONE',  ( -10.81189881249999729, 1.324075727343319199E-15, -165.7812500020484094 ) ) ;
#28216=CARTESIAN_POINT ( 'NONE',  ( 9.999999999999998224, 0.000000000000000000, -159.8750000040967905 ) ) ;
#28217=CARTESIAN_POINT ( 'NONE',  ( 7.644554776091147741E-16, 12.48450537969573659, -101.4687500020483668 ) ) ;
#28218=VERTEX_POINT ( 'NONE', #28397 ) ;
#28220=CARTESIAN_POINT ( 'NONE',  ( 10.81189881249999729, 0.000000000000000000, -196.3437500020484094 ) ) ;
#28222=DIRECTION ( 'NONE',  ( -1.000000000000000000, 0.000000000000000000, 0.000000000000000000 ) ) ;
#28224=CARTESIAN_POINT ( 'NONE',  ( 10.81189881249999729, 0.000000000000000000, -93.03125000204838102 ) ) ;
#28226=CARTESIAN_POINT ( 'NONE',  ( -9.999999999999998224, 1.224646799147353059E-15, -64.62500000409676204 ) ) ;
#28228=CARTESIAN_POINT ( 'NONE',  ( 10.81189881249999551, -6.242252689847874514, -23.96875000204837391 ) ) ;
#28230=CARTESIAN_POINT ( 'NONE',  ( 5.405949406249992428, -9.363379034771808662, -21.28125000204836326 ) ) ;
#28239=ORIENTED_EDGE ( 'NONE', *, *, #34162, .F. ) ;
#28247=CARTESIAN_POINT ( 'NONE',  ( -9.999999999999998224, 0.000000000000000000, -99.99999999999998579 ) ) ;
#28248=CARTESIAN_POINT ( 'NONE',  ( 10.19523493519047719, 1.536126885025608235, -100.0000000000000142 ) ) ;
#28250=CARTESIAN_POINT ( 'NONE',  ( -10.81189881249999729, 6.242252689847871849, -162.9062500020484094 ) ) ;
#28254=CARTESIAN_POINT ( 'NONE',  ( -10.81189881249999729, 1.324075727343319199E-15, -87.59375000204836681 ) ) ;
#28256=CARTESIAN_POINT ( 'NONE',  ( 10.81189881249999729, 0.000000000000000000, -190.3437500020484094 ) ) ;
#28257=CARTESIAN_POINT ( 'NONE',  ( 7.644554776091147741E-16, 12.48450537969573659, -91.15625000204838102 ) ) ;
#28261=CARTESIAN_POINT ( 'NONE',  ( -10.81189881249999729, 6.242252689847871849, -177.9062500020484094 ) ) ;
#28262=CARTESIAN_POINT ( 'NONE',  ( -10.81189881249999907, -6.242252689847864744, -186.6562500020484094 ) ) ;
#28265=CARTESIAN_POINT ( 'NONE',  ( -10.00000000000000000, -5.773502691896251982, -162.0000000040967620 ) ) ;
#28267=CARTESIAN_POINT ( 'NONE',  ( -10.81189881249999729, 1.324075727343319199E-15, -15.59375000204835082 ) ) ;
#28269=CARTESIAN_POINT ( 'NONE',  ( -10.81189881249999907, -6.242252689847864744, -120.4687500020483810 ) ) ;
#28272=CARTESIAN_POINT ( 'NONE',  ( -5.405949406250003975, -9.363379034771801557, -17.03125000204835970 ) ) ;
#28275=CARTESIAN_POINT ( 'NONE',  ( 5.000000000000000000, 8.660254037844385522, -51.24999999999996447 ) ) ;
#28276=CARTESIAN_POINT ( 'NONE',  ( 5.405949406249999534, 9.363379034771803333, -118.2812500020483952 ) ) ;
#28279=CARTESIAN_POINT ( 'NONE',  ( 9.999999999999998224, 0.000000000000000000, -93.87500000409677625 ) ) ;
#28281=CARTESIAN_POINT ( 'NONE',  ( 5.405949406249992428, -9.363379034771808662, -51.09375000204835260 ) ) ;
#28282=ORIENTED_EDGE ( 'NONE', *, *, #18180, .T. ) ;
#28286=CARTESIAN_POINT ( 'NONE',  ( 5.000000000000000000, 8.660254037844385522, -21.62500000409675494 ) ) ;
#28291=ORIENTED_EDGE ( 'NONE', *, *, #39523, .F. ) ;
#28296=ORIENTED_EDGE ( 'NONE', *, *, #37809, .T. ) ;
#28301=CARTESIAN_POINT ( 'NONE',  ( 10.81189881249999907, 6.242252689847868297, -185.9062500020484094 ) ) ;
#28305=CARTESIAN_POINT ( 'NONE',  ( 5.405949406249992428, -9.363379034771808662, -108.0937500020483810 ) ) ;
#28306=CARTESIAN_POINT ( 'NONE',  ( -5.000000000000003553, -8.660254037844383745, -149.8750000040967905 ) ) ;
#28307=CARTESIAN_POINT ( 'NONE',  ( 10.81189881249999729, 0.000000000000000000, -120.0312500020483952 ) ) ;
#28309=CARTESIAN_POINT ( 'NONE',  ( 7.644554776091147741E-16, 12.48450537969573659, -122.4687500020483952 ) ) ;
#28312=CARTESIAN_POINT ( 'NONE',  ( 7.070501591499377789E-16, 11.54700538379251284, -150.1250000000000000 ) ) ;
#28313=CARTESIAN_POINT ( 'NONE',  ( 4.999999999999992006, -8.660254037844389075, -14.24999999999995737 ) ) ;
#28316=CARTESIAN_POINT ( 'NONE',  ( 5.000000000000000000, 8.660254037844385522, -186.6250000040967905 ) ) ;
#28318=CARTESIAN_POINT ( 'NONE',  ( 10.81189881249999907, 6.242252689847868297, -41.71875000204835970 ) ) ;
#28319=CARTESIAN_POINT ( 'NONE',  ( -9.999999999999998224, 1.224646799147353059E-15, -108.1250000040967763 ) ) ;
#28320=CARTESIAN_POINT ( 'NONE',  ( -10.81189881249999907, -6.242252689847864744, -145.9687500020484094 ) ) ;
#28325=CARTESIAN_POINT ( 'NONE',  ( -2.121150477449813534E-15, -11.54700538379251284, -72.87499999999995737 ) ) ;
#28326=CARTESIAN_POINT ( 'NONE',  ( 10.81189881249999729, 0.000000000000000000, -139.5312500020484094 ) ) ;
#28329=ORIENTED_EDGE ( 'NONE', *, *, #13251, .F. ) ;
#28330=CARTESIAN_POINT ( 'NONE',  ( 7.644554776091147741E-16, 12.48450537969573659, -103.1562500020483952 ) ) ;
#28331=CARTESIAN_POINT ( 'NONE',  ( 10.00000000000000000, 5.773502691896255534, -113.2500000040967905 ) ) ;
#28332=CARTESIAN_POINT ( 'NONE',  ( -5.000000000000003553, -8.660254037844383745, -140.5000000000000000 ) ) ;
#28333=CARTESIAN_POINT ( 'NONE',  ( -10.81189881249999729, 1.324075727343319199E-15, -77.09375000204838102 ) ) ;
#28339=CARTESIAN_POINT ( 'NONE',  ( 7.644554776091147741E-16, 12.48450537969573659, -43.15625000204837391 ) ) ;
#28343=CARTESIAN_POINT ( 'NONE',  ( -2.121150477449813534E-15, -11.54700538379251284, -164.7500000040968189 ) ) ;
#28344=EDGE_CURVE ( 'NONE', #32304, #19459, #33972, .T. ) ;
#28346=VERTEX_POINT ( 'NONE', #41018 ) ;
#28350=AXIS2_PLACEMENT_3D ( 'NONE', #31626, #8525, #2059 ) ;
#28354=CARTESIAN_POINT ( 'NONE',  ( 9.999999999999998224, 0.000000000000000000, -129.8750000040967905 ) ) ;
#28358=CARTESIAN_POINT ( 'NONE',  ( -9.999999999999998224, 1.224646799147353059E-15, -163.2500000000000000 ) ) ;
#28359=CARTESIAN_POINT ( 'NONE',  ( 10.81189881249999729, 0.000000000000000000, -136.3437500020484094 ) ) ;
#28360=CARTESIAN_POINT ( 'NONE',  ( -10.81189881249999907, -6.242252689847864744, -143.1562500020484094 ) ) ;
#28361=CARTESIAN_POINT ( 'NONE',  ( -2.293366432827344421E-15, -12.48450537969573659, -144.2187500020484094 ) ) ;
#28364=CARTESIAN_POINT ( 'NONE',  ( 5.000000000000000000, 8.660254037844385522, -168.2500000000000000 ) ) ;
#28366=CARTESIAN_POINT ( 'NONE',  ( -6.089403866005159038, 8.962546680094892082, -99.99999999999998579 ) ) ;
#28368=CARTESIAN_POINT ( 'NONE',  ( -9.469335213649141991, 4.843080047529867649, -100.0000000000000142 ) ) ;
#28369=CARTESIAN_POINT ( 'NONE',  ( 10.81189881249999907, 6.242252689847868297, -167.7187500020483810 ) ) ;
#28373=CARTESIAN_POINT ( 'NONE',  ( -5.405949406250003975, -9.363379034771801557, -45.53125000204838102 ) ) ;
#28375=CARTESIAN_POINT ( 'NONE',  ( -5.000000000000003553, -8.660254037844383745, -103.0000000000000000 ) ) ;
#28376=ORIENTED_EDGE ( 'NONE', *, *, #8538, .T. ) ;
#28377=CARTESIAN_POINT ( 'NONE',  ( -5.405949406250003975, -9.363379034771801557, -126.5312500020483952 ) ) ;
#28378=CARTESIAN_POINT ( 'NONE',  ( 10.00000000000000000, 5.773502691896255534, -140.2500000040967905 ) ) ;
#28380=MANIFOLD_SOLID_BREP ( 'Cavity2', #9445 ) ;
#28383=CARTESIAN_POINT ( 'NONE',  ( 5.405949406249992428, -9.363379034771808662, -174.0937500020484094 ) ) ;
#28387=CARTESIAN_POINT ( 'NONE',  ( 5.405949406249999534, 9.363379034771803333, -65.78125000204838102 ) ) ;
#28389=CARTESIAN_POINT ( 'NONE',  ( -9.999999999999998224, 1.224646799147353059E-15, -48.12500000409677625 ) ) ;
#28390=CARTESIAN_POINT ( 'NONE',  ( -4.999999999999996447, 8.660254037844387298, -147.3750000040967905 ) ) ;
#28393=EDGE_CURVE ( 'NONE', #32933, #31697, #27234, .T. ) ;
#28396=ORIENTED_EDGE ( 'NONE', *, *, #37394, .T. ) ;
#28397=CARTESIAN_POINT ( 'NONE',  ( -9.999999999999998224, 1.224646799147353059E-15, -156.1250000040967905 ) ) ;
#28398=( BOUNDED_CURVE ( )  B_SPLINE_CURVE ( 2, ( #32950, #10054, #369, #23449, #17156, #19980, #3380 ),
 .UNSPECIFIED., .F., .F. ) 
 B_SPLINE_CURVE_WITH_KNOTS ( ( 3, 2, 2, 3 ),
 ( 0.3171641791044778058, 0.3184079601990050801, 0.3196517412935324653, 0.3208955223880597396 ),
 .UNSPECIFIED. ) 
 CURVE ( )  GEOMETRIC_REPRESENTATION_ITEM ( )  RATIONAL_B_SPLINE_CURVE ( ( 0.9999999999999820144, 0.8660254037844566932, 1.000000000000000000, 0.8660254037844387076, 1.000000000000000000, 0.8660254037844327124, 1.000000000000005995 ) ) 
 REPRESENTATION_ITEM ( '' )  );
#28413=CARTESIAN_POINT ( 'NONE',  ( 4.999999999999992006, -8.660254037844389075, -35.24999999999997868 ) ) ;
#28416=CARTESIAN_POINT ( 'NONE',  ( -2.293366432827344421E-15, -12.48450537969573659, -154.7187500020483810 ) ) ;
#28418=CARTESIAN_POINT ( 'NONE',  ( -5.405949406250003975, -9.363379034771801557, -178.8437500020483810 ) ) ;
#28420=CARTESIAN_POINT ( 'NONE',  ( 4.999999999999992006, -8.660254037844389075, -126.7499999999999716 ) ) ;
#28421=CARTESIAN_POINT ( 'NONE',  ( -4.999999999999996447, 8.660254037844387298, -196.5000000000000000 ) ) ;
#28426=CARTESIAN_POINT ( 'NONE',  ( 5.405949406249999534, 9.363379034771803333, -67.28125000204838102 ) ) ;
#28428=CARTESIAN_POINT ( 'NONE',  ( -2.121150477449813534E-15, -11.54700538379251284, -122.3750000000000142 ) ) ;
#28430=CARTESIAN_POINT ( 'NONE',  ( 10.81189881249999729, 6.242252689847867408, -151.4062500020484094 ) ) ;
#28431=CARTESIAN_POINT ( 'NONE',  ( -5.405949406249996869, 9.363379034771805109, -163.0312500020484094 ) ) ;
#28433=CARTESIAN_POINT ( 'NONE',  ( 0.000000000000000000, 0.000000000000000000, -99.99999999999998579 ) ) ;
#28435=CARTESIAN_POINT ( 'NONE',  ( -10.81189881249999729, 1.324075727343319199E-15, -99.59375000204838102 ) ) ;
#28436=VERTEX_POINT ( 'NONE', #24447 ) ;
#28438=CARTESIAN_POINT ( 'NONE',  ( 5.405949406249992428, -9.363379034771808662, -193.5937500020484094 ) ) ;
#28440=CARTESIAN_POINT ( 'NONE',  ( 1.680766644672218924, -10.37565344158061542, -180.0000000000000284 ) ) ;
#28441=CARTESIAN_POINT ( 'NONE',  ( -9.999999999999998224, 1.224646799147353059E-15, -124.2500000000000000 ) ) ;
#28442=CARTESIAN_POINT ( 'NONE',  ( -10.81189881249999907, -6.242252689847864744, -90.65625000204836681 ) ) ;
#28445=CARTESIAN_POINT ( 'NONE',  ( -10.00000000000000000, -5.773502691896251982, -69.00000000409677625 ) ) ;
#28447=CARTESIAN_POINT ( 'NONE',  ( -5.405949406249996869, 9.363379034771805109, -29.34375000204836326 ) ) ;
#28451=CARTESIAN_POINT ( 'NONE',  ( 10.81189881249999551, -6.242252689847874514, -22.65625000204837747 ) ) ;
#28463=ORIENTED_EDGE ( 'NONE', *, *, #11687, .F. ) ;
#28471=CARTESIAN_POINT ( 'NONE',  ( 9.617269083703753552, -3.087026286776204831, -100.0000000000000142 ) ) ;
#28473=CARTESIAN_POINT ( 'NONE',  ( -5.405949406250003975, -9.363379034771801557, -167.0312500020484094 ) ) ;
#28477=CARTESIAN_POINT ( 'NONE',  ( 7.644554776091147741E-16, 12.48450537969573659, -86.46875000204838102 ) ) ;
#28478=CARTESIAN_POINT ( 'NONE',  ( -5.405949406249996869, 9.363379034771805109, -197.3437500020484094 ) ) ;
#28479=CARTESIAN_POINT ( 'NONE',  ( 10.81189881249999551, -6.242252689847874514, -93.15625000204838102 ) ) ;
#28482=CARTESIAN_POINT ( 'NONE',  ( 10.81189881249999729, 6.242252689847867408, -175.4062500020484094 ) ) ;
#28483=CARTESIAN_POINT ( 'NONE',  ( 7.644554776091147741E-16, 12.48450537969573659, -191.6562500020484094 ) ) ;
#28485=CARTESIAN_POINT ( 'NONE',  ( -5.000000000000003553, -8.660254037844383745, -160.3750000040967905 ) ) ;
#28487=CARTESIAN_POINT ( 'NONE',  ( -5.405949406250003975, -9.363379034771801557, -16.84375000204835260 ) ) ;
#28489=CARTESIAN_POINT ( 'NONE',  ( -5.405949406249996869, 9.363379034771805109, -120.8437500020483952 ) ) ;
#28491=CARTESIAN_POINT ( 'NONE',  ( -5.405949406249996869, 9.363379034771805109, -20.53125000204836326 ) ) ;
#28493=CYLINDRICAL_SURFACE ( 'NONE', #23098, 9.999999999999998224 ) ;
#28494=CARTESIAN_POINT ( 'NONE',  ( -5.000000000000003553, -8.660254037844383745, -54.99999999999996447 ) ) ;
#28495=CARTESIAN_POINT ( 'NONE',  ( -5.405949406250003975, -9.363379034771801557, -114.5312500020483952 ) ) ;
#28497=ORIENTED_EDGE ( 'NONE', *, *, #30302, .T. ) ;
#28498=ADVANCED_FACE ( 'NONE', ( #11035 ), #10819, .F. ) ;
#28499=CARTESIAN_POINT ( 'NONE',  ( -9.999999999999998224, 1.224646799147353059E-15, -94.62500000409677625 ) ) ;
#28500=CARTESIAN_POINT ( 'NONE',  ( 9.999999999999998224, 0.000000000000000000, -100.9999999999999858 ) ) ;
#28502=CARTESIAN_POINT ( 'NONE',  ( -10.81189881249999729, 6.242252689847871849, -51.71875000204836681 ) ) ;
#28507=CARTESIAN_POINT ( 'NONE',  ( 9.999999999999996447, -5.773502691896262640, -22.00000000409677270 ) ) ;
#28512=ORIENTED_EDGE ( 'NONE', *, *, #8183, .F. ) ;
#28516=EDGE_CURVE ( 'NONE', #9539, #27414, #69, .T. ) ;
#28517=VERTEX_POINT ( 'NONE', #1566 ) ;
#28518=VERTEX_POINT ( 'NONE', #14038 ) ;
#28523=CARTESIAN_POINT ( 'NONE',  ( 10.81189881249999551, -6.242252689847874514, -184.6562500020484094 ) ) ;
#28526=CARTESIAN_POINT ( 'NONE',  ( 7.644554776091147741E-16, 12.48450537969573659, -113.4687500020483952 ) ) ;
#28528=CARTESIAN_POINT ( 'NONE',  ( -10.81189881249999729, 1.324075727343319199E-15, -114.7812500020483952 ) ) ;
#28530=CARTESIAN_POINT ( 'NONE',  ( 10.81189881249999729, 0.000000000000000000, -121.3437500020483952 ) ) ;
#28533=CARTESIAN_POINT ( 'NONE',  ( -9.999999999999998224, 1.224646799147353059E-15, -151.2500000000000000 ) ) ;
#28534=CARTESIAN_POINT ( 'NONE',  ( 5.000000000000000000, 8.660254037844385522, -15.24999999999995737 ) ) ;
#28537=CARTESIAN_POINT ( 'NONE',  ( 4.999999999999992006, -8.660254037844389075, -188.6250000040967905 ) ) ;
#28539=CARTESIAN_POINT ( 'NONE',  ( 10.81189881249999729, 0.000000000000000000, -37.34375000204836681 ) ) ;
#28541=CARTESIAN_POINT ( 'NONE',  ( 10.81189881249999551, -6.242252689847874514, -142.4687500020483810 ) ) ;
#28543=CARTESIAN_POINT ( 'NONE',  ( -9.999999999999998224, 1.224646799147353059E-15, -145.2500000000000000 ) ) ;
#28544=CARTESIAN_POINT ( 'NONE',  ( 9.999999999999998224, 0.000000000000000000, -78.49999999999998579 ) ) ;
#28545=CARTESIAN_POINT ( 'NONE',  ( -10.81189881249999907, -6.242252689847864744, -137.1562500020483810 ) ) ;
#28548=CARTESIAN_POINT ( 'NONE',  ( 7.070501591499376803E-16, 11.54700538379251284, -120.5000000040967905 ) ) ;
#28549=CARTESIAN_POINT ( 'NONE',  ( 5.000000000000000000, 8.660254037844385522, -117.6250000040967905 ) ) ;
#28551=CARTESIAN_POINT ( 'NONE',  ( -10.81189881249999729, 6.242252689847871849, -75.71875000204836681 ) ) ;
#28554=CARTESIAN_POINT ( 'NONE',  ( 9.999999999999998224, 0.000000000000000000, -131.3750000040967905 ) ) ;
#28555=CARTESIAN_POINT ( 'NONE',  ( 10.81189881249999907, 6.242252689847868297, -43.40625000204836681 ) ) ;
#28560=CARTESIAN_POINT ( 'NONE',  ( 4.999999999999992006, -8.660254037844389075, -173.6250000040968189 ) ) ;
#28562=( BOUNDED_CURVE ( )  B_SPLINE_CURVE ( 2, ( #30111, #31181, #41286, #41507, #21662, #18634, #8723 ),
 .UNSPECIFIED., .F., .F. ) 
 B_SPLINE_CURVE_WITH_KNOTS ( ( 3, 2, 2, 3 ),
 ( 0.3283582089552238847, 0.3296019900497513255, 0.3308457711442787108, 0.3320895522388061516 ),
 .UNSPECIFIED. ) 
 CURVE ( )  GEOMETRIC_REPRESENTATION_ITEM ( )  RATIONAL_B_SPLINE_CURVE ( ( 1.000000000000000000, 0.8660254037844387076, 1.000000000000000000, 0.8660254037844387076, 1.000000000000000000, 0.8660254037844207220, 1.000000000000017986 ) ) 
 REPRESENTATION_ITEM ( '' )  );
#28567=CARTESIAN_POINT ( 'NONE',  ( -9.999999999999998224, 1.224646799147353059E-15, -135.1250000040967620 ) ) ;
#28570=LINE ( 'NONE', #8282, #17746 ) ;
#28574=CARTESIAN_POINT ( 'NONE',  ( 10.81189881249999551, -6.242252689847874514, -133.4687500020483810 ) ) ;
#28575=CARTESIAN_POINT ( 'NONE',  ( -5.405949406250003975, -9.363379034771801557, -141.5312500020483810 ) ) ;
#28576=CARTESIAN_POINT ( 'NONE',  ( 5.405949406249992428, -9.363379034771808662, -148.5937500020483810 ) ) ;
#28579=CARTESIAN_POINT ( 'NONE',  ( -10.00000000000000000, -5.773502691896251982, -170.6250000000000284 ) ) ;
#28581=CARTESIAN_POINT ( 'NONE',  ( -5.000000000000003553, -8.660254037844383745, -114.9999999999999858 ) ) ;
#28584=CARTESIAN_POINT ( 'NONE',  ( -10.81189881249999729, 1.324075727343319199E-15, -168.5937500020484094 ) ) ;
#28588=CARTESIAN_POINT ( 'NONE',  ( 7.644554776091147741E-16, 12.48450537969573659, -35.65625000204835970 ) ) ;
#28590=CARTESIAN_POINT ( 'NONE',  ( -4.999999999999996447, 8.660254037844387298, -102.0000000000000000 ) ) ;
#28592=CARTESIAN_POINT ( 'NONE',  ( -5.405949406250003975, -9.363379034771801557, -120.5312500020483952 ) ) ;
#28593=CARTESIAN_POINT ( 'NONE',  ( 10.00000000000000000, 5.773502691896255534, -141.7500000040967905 ) ) ;
#28598=EDGE_CURVE ( 'NONE', #10904, #37078, #11391, .T. ) ;
#28600=CARTESIAN_POINT ( 'NONE',  ( 10.81189881249999729, 0.000000000000000000, -67.53125000204838102 ) ) ;
#28605=ORIENTED_EDGE ( 'NONE', *, *, #2901, .F. ) ;
#28607=CARTESIAN_POINT ( 'NONE',  ( -9.999999999999998224, 1.224646799147353059E-15, -172.6250000040968189 ) ) ;
#28613=CARTESIAN_POINT ( 'NONE',  ( 9.999999999999998224, 0.000000000000000000, -177.8750000040967905 ) ) ;
#28614=ORIENTED_EDGE ( 'NONE', *, *, #37969, .T. ) ;
#28618=DIRECTION ( 'NONE',  ( -0.000000000000000000, -0.000000000000000000, -1.000000000000000000 ) ) ;
#28621=ORIENTED_EDGE ( 'NONE', *, *, #18843, .F. ) ;
#28622=ADVANCED_FACE ( 'NONE', ( #17645 ), #37734, .F. ) ;
#28623=DIRECTION ( 'NONE',  ( -0.000000000000000000, -0.000000000000000000, -1.000000000000000000 ) ) ;
#28624=CARTESIAN_POINT ( 'NONE',  ( 10.00000000000000000, 5.773502691896255534, -34.87499999999996447 ) ) ;
#28627=CARTESIAN_POINT ( 'NONE',  ( 7.644554776091147741E-16, 12.48450537969573659, -159.9687500020483810 ) ) ;
#28628=CARTESIAN_POINT ( 'NONE',  ( -5.405949406249996869, 9.363379034771805109, -168.8437500020484094 ) ) ;
#28631=CARTESIAN_POINT ( 'NONE',  ( -9.999999999999227285, -5.773502691896698735, -127.1249999999999574 ) ) ;
#28632=CARTESIAN_POINT ( 'NONE',  ( -9.999999999999998224, 5.773502691896259087, -199.3750000000000000 ) ) ;
#28637=CARTESIAN_POINT ( 'NONE',  ( 10.81189881249999907, 6.242252689847868297, -68.90625000204839523 ) ) ;
#28639=CARTESIAN_POINT ( 'NONE',  ( 5.000000000000000000, 8.660254037844385522, -121.7500000000000000 ) ) ;
#28640=ADVANCED_FACE ( 'NONE', ( #18085 ), #24807, .F. ) ;
#28641=ORIENTED_EDGE ( 'NONE', *, *, #5437, .T. ) ;
#28642=CARTESIAN_POINT ( 'NONE',  ( -10.81189881249999729, 6.242252689847871849, -147.9062500020484094 ) ) ;
#28643=CARTESIAN_POINT ( 'NONE',  ( -5.405949406249996869, 9.363379034771805109, -164.5312500020484094 ) ) ;
#28646=CARTESIAN_POINT ( 'NONE',  ( -5.405949406249996869, 9.363379034771805109, -99.84375000204838102 ) ) ;
#28647=EDGE_LOOP ( 'NONE', ( #11515, #34345, #34986, #20617 ) ) ;
#28649=CARTESIAN_POINT ( 'NONE',  ( -10.81189881249999907, -6.242252689847864744, -195.4687500020484094 ) ) ;
#28651=CARTESIAN_POINT ( 'NONE',  ( -8.236488666302303585, -5.752346336555091533, -180.0000000000000284 ) ) ;
#28653=CARTESIAN_POINT ( 'NONE',  ( -10.81189881249999729, 6.242252689847871849, -92.40625000204838102 ) ) ;
#28656=CARTESIAN_POINT ( 'NONE',  ( 9.999999999999998224, 0.000000000000000000, -71.37500000409677625 ) ) ;
#28658=CARTESIAN_POINT ( 'NONE',  ( -2.293366432827344421E-15, -12.48450537969573659, -25.71875000204837391 ) ) ;
#28661=CARTESIAN_POINT ( 'NONE',  ( 10.81189881249999729, 0.000000000000000000, -19.53125000204835970 ) ) ;
#28664=VECTOR ( 'NONE', #12594, 1000.000000000000000 ) ;
#28665=CARTESIAN_POINT ( 'NONE',  ( -4.999999999999996447, 8.660254037844387298, 1.124999995903236405 ) ) ;
#28678=LINE ( 'NONE', #32341, #3189 ) ;
#28681=CARTESIAN_POINT ( 'NONE',  ( -9.999999999999998224, 1.224646799147353059E-15, -106.2499999999999858 ) ) ;
#28682=CARTESIAN_POINT ( 'NONE',  ( -10.81189881249999729, 6.242252689847871849, -153.9062500020483810 ) ) ;
#28684=CARTESIAN_POINT ( 'NONE',  ( -9.999999999999998224, 0.000000000000000000, -99.99999999999998579 ) ) ;
#28688=CIRCLE ( 'NONE', #20400, 35.00000000000000711 ) ;
#28689=CARTESIAN_POINT ( 'NONE',  ( 10.81189881249999729, 0.000000000000000000, -85.34375000204836681 ) ) ;
#28690=CARTESIAN_POINT ( 'NONE',  ( 5.405949406249999534, 9.363379034771803333, -91.28125000204838102 ) ) ;
#28694=CARTESIAN_POINT ( 'NONE',  ( -5.405949406250003975, -9.363379034771801557, -177.5312500020483810 ) ) ;
#28695=CARTESIAN_POINT ( 'NONE',  ( 10.81189881249999729, 0.000000000000000000, -186.0312500020484094 ) ) ;
#28697=CARTESIAN_POINT ( 'NONE',  ( -2.121150477449813534E-15, -11.54700538379251284, -163.2500000040967620 ) ) ;
#28699=CARTESIAN_POINT ( 'NONE',  ( -5.405949406249996869, 9.363379034771805109, -12.84375000204834905 ) ) ;
#28700=CARTESIAN_POINT ( 'NONE',  ( -9.999999999999742428, -5.773502691896402084, -157.1250000000000000 ) ) ;
#28701=CARTESIAN_POINT ( 'NONE',  ( -10.81189881249999729, 1.324075727343319199E-15, -120.5937500020483952 ) ) ;
#28703=CARTESIAN_POINT ( 'NONE',  ( -5.405949406250003975, -9.363379034771801557, -18.53125000204835970 ) ) ;
#28705=CARTESIAN_POINT ( 'NONE',  ( -9.999999999999998224, 1.224646799147353059E-15, -136.6250000040967620 ) ) ;
#28706=CARTESIAN_POINT ( 'NONE',  ( 10.81189881249999551, -6.242252689847874514, -115.6562500020483810 ) ) ;
#28709=( BOUNDED_CURVE ( )  B_SPLINE_CURVE ( 2, ( #36299, #7153, #12967, #26795, #6314, #25956, #36085 ),
 .UNSPECIFIED., .F., .F. ) 
 B_SPLINE_CURVE_WITH_KNOTS ( ( 3, 2, 2, 3 ),
 ( 0.4738805970149255198, 0.4751243781094529051, 0.4763681592039803459, 0.4776119402985076756 ),
 .UNSPECIFIED. ) 
 CURVE ( )  GEOMETRIC_REPRESENTATION_ITEM ( )  RATIONAL_B_SPLINE_CURVE ( ( 0.9999999999999820144, 0.8660254037844566932, 1.000000000000000000, 0.8660254037844387076, 1.000000000000000000, 0.8660254037844148378, 1.000000000000023981 ) ) 
 REPRESENTATION_ITEM ( '' )  );
#28710=CARTESIAN_POINT ( 'NONE',  ( 5.000000000000000000, 8.660254037844385522, -93.62500000409677625 ) ) ;
#28713=CARTESIAN_POINT ( 'NONE',  ( 10.81189881249999907, 6.242252689847868297, -49.21875000204835970 ) ) ;
#28718=CARTESIAN_POINT ( 'NONE',  ( -10.00000000000000000, -5.773502691896251982, -22.50000000409676915 ) ) ;
#28724=EDGE_LOOP ( 'NONE', ( #32580, #12237, #9621, #39781 ) ) ;
#28733=CARTESIAN_POINT ( 'NONE',  ( -5.405949406249996869, 9.363379034771805109, -191.5312500020484094 ) ) ;
#28737=CARTESIAN_POINT ( 'NONE',  ( -10.81189881249999729, 1.324075727343319199E-15, -110.0937500020483810 ) ) ;
#28739=CARTESIAN_POINT ( 'NONE',  ( 7.644554776091147741E-16, 12.48450537969573659, -115.1562500020483952 ) ) ;
#28741=CARTESIAN_POINT ( 'NONE',  ( 10.81189881249999551, -6.242252689847874514, -122.9687500020483952 ) ) ;
#28745=CARTESIAN_POINT ( 'NONE',  ( -4.999999999999996447, 8.660254037844387298, -139.5000000000000000 ) ) ;
#28746=CARTESIAN_POINT ( 'NONE',  ( -4.999999999999996447, 8.660254037844387298, -11.99999999999995559 ) ) ;
#28749=CARTESIAN_POINT ( 'NONE',  ( 9.999999999999996447, -5.773502691896262640, -185.5000000040967905 ) ) ;
#28751=CARTESIAN_POINT ( 'NONE',  ( -2.293366432827344421E-15, -12.48450537969573659, -40.71875000204835970 ) ) ;
#28753=CARTESIAN_POINT ( 'NONE',  ( 10.81189881249999551, -6.242252689847874514, -148.4687500020484094 ) ) ;
#28756=CARTESIAN_POINT ( 'NONE',  ( -9.999999999999998224, 1.224646799147353059E-15, -102.1250000040967905 ) ) ;
#28757=CARTESIAN_POINT ( 'NONE',  ( 9.999999999999996447, -5.773502691896262640, -75.62499999999998579 ) ) ;
#28758=CARTESIAN_POINT ( 'NONE',  ( -2.293366432827344421E-15, -12.48450537969573659, -141.4062500020483810 ) ) ;
#28760=ORIENTED_EDGE ( 'NONE', *, *, #18012, .F. ) ;
#28762=CARTESIAN_POINT ( 'NONE',  ( -4.999999999999996447, 8.660254037844387298, -115.8750000040967905 ) ) ;
#28764=CARTESIAN_POINT ( 'NONE',  ( 10.81189881249999551, -6.242252689847874514, -74.96875000204838102 ) ) ;
#28768=DIRECTION ( 'NONE',  ( -0.7071067811865463515, 0.000000000000000000, -0.7071067811865487940 ) ) ;
#28769=CARTESIAN_POINT ( 'NONE',  ( -5.405949406249996869, 9.363379034771805109, -34.03125000204837391 ) ) ;
#28770=CARTESIAN_POINT ( 'NONE',  ( 9.999999999999998224, 0.000000000000000000, -137.0000000000000000 ) ) ;
#28774=( BOUNDED_CURVE ( )  B_SPLINE_CURVE ( 2, ( #10018, #23196, #36356, #14082, #30321, #30957, #40850 ),
 .UNSPECIFIED., .F., .F. ) 
 B_SPLINE_CURVE_WITH_KNOTS ( ( 3, 2, 2, 3 ),
 ( 0.4776119402985076756, 0.4788557213930350054, 0.4800995024875623352, 0.4813432835820896649 ),
 .UNSPECIFIED. ) 
 CURVE ( )  GEOMETRIC_REPRESENTATION_ITEM ( )  RATIONAL_B_SPLINE_CURVE ( ( 0.9999999999999761302, 0.8660254037844625774, 1.000000000000000000, 0.8660254037844387076, 1.000000000000000000, 0.8660254037844267172, 1.000000000000011990 ) ) 
 REPRESENTATION_ITEM ( '' )  );
#28777=VERTEX_POINT ( 'NONE', #10963 ) ;
#28786=CARTESIAN_POINT ( 'NONE',  ( -10.81189881249999729, 6.242252689847871849, -131.2187500020483810 ) ) ;
#28787=CARTESIAN_POINT ( 'NONE',  ( 10.81189881249999907, 6.242252689847868297, -137.9062500020483810 ) ) ;
#28789=CARTESIAN_POINT ( 'NONE',  ( -5.405949406250003975, -9.363379034771801557, -150.3437500020483810 ) ) ;
#28792=CARTESIAN_POINT ( 'NONE',  ( -9.999999999999998224, 5.773502691896259087, -167.8749999999999716 ) ) ;
#28796=CARTESIAN_POINT ( 'NONE',  ( -2.293366432827344421E-15, -12.48450537969573659, -61.71875000204837391 ) ) ;
#28798=CARTESIAN_POINT ( 'NONE',  ( 10.81189881249999907, 6.242252689847868297, -169.2187500020483810 ) ) ;
#28802=CARTESIAN_POINT ( 'NONE',  ( 10.81189881249999551, -6.242252689847874514, -37.65625000204836681 ) ) ;
#28804=CARTESIAN_POINT ( 'NONE',  ( -9.999999999999998224, 5.773502691896259087, -103.3750000000000000 ) ) ;
#28805=VERTEX_POINT ( 'NONE', #17863 ) ;
#28806=CARTESIAN_POINT ( 'NONE',  ( 7.644554776091147741E-16, 12.48450537969573659, -118.1562500020483952 ) ) ;
#28807=CARTESIAN_POINT ( 'NONE',  ( -9.999999999999998224, 1.224646799147353059E-15, -138.1250000040967620 ) ) ;
#28814=CARTESIAN_POINT ( 'NONE',  ( 7.644554776091147741E-16, 12.48450537969573659, -61.15625000204838102 ) ) ;
#28818=CARTESIAN_POINT ( 'NONE',  ( 4.999999999999992006, -8.660254037844389075, -106.1250000040967763 ) ) ;
#28819=VECTOR ( 'NONE', #24810, 1000.000000000000000 ) ;
#28825=CARTESIAN_POINT ( 'NONE',  ( -5.000000000000003553, -8.660254037844383745, -178.3750000040967905 ) ) ;
#28834=CARTESIAN_POINT ( 'NONE',  ( 9.999999999999996447, -5.773502691896262640, -32.12499999999995737 ) ) ;
#28837=CARTESIAN_POINT ( 'NONE',  ( -10.81189881249999729, 6.242252689847871849, -158.2187500020483810 ) ) ;
#28838=CARTESIAN_POINT ( 'NONE',  ( 10.81189881249999551, -6.242252689847874514, -169.4687500020483810 ) ) ;
#28840=CARTESIAN_POINT ( 'NONE',  ( 9.999999999999998224, 0.000000000000000000, -198.5000000000000000 ) ) ;
#28846=CARTESIAN_POINT ( 'NONE',  ( -5.405949406250003975, -9.363379034771801557, -57.53125000204836681 ) ) ;
#28848=CARTESIAN_POINT ( 'NONE',  ( 4.999999999999992006, -8.660254037844389075, -126.7499999999999716 ) ) ;
#28850=CARTESIAN_POINT ( 'NONE',  ( 10.81189881249999551, -6.242252689847874514, -141.1562500020484094 ) ) ;
#28851=CARTESIAN_POINT ( 'NONE',  ( 10.81189881249999907, 6.242252689847868297, -154.4062500020484094 ) ) ;
#28854=CARTESIAN_POINT ( 'NONE',  ( 10.81189881249999551, -6.242252689847874514, -88.46875000204836681 ) ) ;
#28857=CARTESIAN_POINT ( 'NONE',  ( -5.405949406250003975, -9.363379034771801557, -184.8437500020483810 ) ) ;
#28859=EDGE_CURVE ( 'NONE', #17374, #5087, #27598, .T. ) ;
#28862=CARTESIAN_POINT ( 'NONE',  ( -5.405949406249996869, 9.363379034771805109, -80.53125000204838102 ) ) ;
#28865=CARTESIAN_POINT ( 'NONE',  ( -2.121150477449813534E-15, -11.54700538379251284, -70.25000000409679046 ) ) ;
#28867=CARTESIAN_POINT ( 'NONE',  ( -5.405949406249996869, 9.363379034771805109, -20.34375000204835615 ) ) ;
#28870=CARTESIAN_POINT ( 'NONE',  ( 10.81189881249999907, 6.242252689847868297, -19.40625000204837747 ) ) ;
#28880=CARTESIAN_POINT ( 'NONE',  ( 4.999999999999992006, -8.660254037844389075, -179.6250000040968189 ) ) ;
#28888=LINE ( 'NONE', #2349, #18072 ) ;
#28891=DIRECTION ( 'NONE',  ( 1.000000000000000000, 0.000000000000000000, -0.000000000000000000 ) ) ;
#28892=CARTESIAN_POINT ( 'NONE',  ( 10.81189881249999729, 0.000000000000000000, -160.5312500020484094 ) ) ;
#28897=CARTESIAN_POINT ( 'NONE',  ( -5.405949406250003975, -9.363379034771801557, -75.34375000204838102 ) ) ;
#28898=CARTESIAN_POINT ( 'NONE',  ( -10.81189881249999729, 6.242252689847871849, -86.40625000204836681 ) ) ;
#28901=CARTESIAN_POINT ( 'NONE',  ( 5.405949406249999534, 9.363379034771803333, -166.2812500020484094 ) ) ;
#28902=CARTESIAN_POINT ( 'NONE',  ( 5.405949406249999534, 9.363379034771803333, -179.7812500020484094 ) ) ;
#28904=CARTESIAN_POINT ( 'NONE',  ( -5.000000000000003553, -8.660254037844383745, -161.8750000040967905 ) ) ;
#28906=CARTESIAN_POINT ( 'NONE',  ( 5.405949406249992428, -9.363379034771808662, -16.59375000204835260 ) ) ;
#28907=CARTESIAN_POINT ( 'NONE',  ( 10.00000000000038369, -5.773502691896038819, -156.6250000000000284 ) ) ;
#28908=CARTESIAN_POINT ( 'NONE',  ( -5.405949406250003975, -9.363379034771801557, -112.8437500020483810 ) ) ;
#28910=CARTESIAN_POINT ( 'NONE',  ( -10.81189881249999729, 6.242252689847871849, -21.90625000204837391 ) ) ;
#28913=CARTESIAN_POINT ( 'NONE',  ( 7.644554776091147741E-16, 12.48450537969573659, -116.6562500020483952 ) ) ;
#28916=CARTESIAN_POINT ( 'NONE',  ( 7.070501591499377789E-16, 11.54700538379251284, -92.00000000409677625 ) ) ;
#28918=CARTESIAN_POINT ( 'NONE',  ( 10.81189881249999729, 0.000000000000000000, -49.34375000204838102 ) ) ;
#28921=AXIS2_PLACEMENT_3D ( 'NONE', #28433, #41127, #31453 ) ;
#28924=CARTESIAN_POINT ( 'NONE',  ( 9.999999999999998224, 0.000000000000000000, -23.37500000409675849 ) ) ;
#28926=EDGE_CURVE ( 'NONE', #21693, #17213, #29094, .T. ) ;
#28940=CARTESIAN_POINT ( 'NONE',  ( 10.81189881249999729, 0.000000000000000000, -184.5312500020484094 ) ) ;
#28942=CARTESIAN_POINT ( 'NONE',  ( -9.999999999999227285, -5.773502691896698735, -133.1249999999999716 ) ) ;
#28944=CARTESIAN_POINT ( 'NONE',  ( 5.405949406249992428, -9.363379034771808662, -105.0937500020483810 ) ) ;
#28946=CARTESIAN_POINT ( 'NONE',  ( 10.81189881249999907, 6.242252689847868297, -118.4062500020484094 ) ) ;
#28948=CARTESIAN_POINT ( 'NONE',  ( -2.293366432827344421E-15, -12.48450537969573659, -120.2187500020483952 ) ) ;
#28951=CARTESIAN_POINT ( 'NONE',  ( -2.121150477449813534E-15, -11.54700538379251284, -140.3750000000000000 ) ) ;
#28952=CARTESIAN_POINT ( 'NONE',  ( -9.999999999999998224, 5.773502691896259087, -10.37499999999996803 ) ) ;
#28955=CARTESIAN_POINT ( 'NONE',  ( -2.121150477449813534E-15, -11.54700538379251284, -190.2500000040967905 ) ) ;
#28957=CARTESIAN_POINT ( 'NONE',  ( 10.81189881249999729, 0.000000000000000000, -38.84375000204837391 ) ) ;
#28959=CARTESIAN_POINT ( 'NONE',  ( -10.81189881249999729, 1.324075727343319199E-15, -146.0937500020483810 ) ) ;
#28961=CARTESIAN_POINT ( 'NONE',  ( -9.999999999999998224, 5.773502691896259087, -65.87499999999998579 ) ) ;
#28962=CARTESIAN_POINT ( 'NONE',  ( -2.293366432827344421E-15, -12.48450537969573659, -138.4062500020483810 ) ) ;
#28966=CARTESIAN_POINT ( 'NONE',  ( 9.999999999999996447, -5.773502691896262640, -116.5000000040967763 ) ) ;
#28968=CARTESIAN_POINT ( 'NONE',  ( 5.405949406249992428, -9.363379034771808662, -70.59375000204836681 ) ) ;
#28972=CARTESIAN_POINT ( 'NONE',  ( 10.81189881249999551, -6.242252689847874514, -33.15625000204835970 ) ) ;
#28974=CARTESIAN_POINT ( 'NONE',  ( -9.999999999999227285, -5.773502691896698735, -139.1249999999999716 ) ) ;
#28991=CARTESIAN_POINT ( 'NONE',  ( -10.81189881249999907, -6.242252689847864744, -130.9687500020483810 ) ) ;
#28992=CARTESIAN_POINT ( 'NONE',  ( 5.405949406249992428, -9.363379034771808662, -142.7812500020483810 ) ) ;
#28994=CARTESIAN_POINT ( 'NONE',  ( 7.644554776091147741E-16, 12.48450537969573659, -149.4687500020484663 ) ) ;
#28996=CARTESIAN_POINT ( 'NONE',  ( -9.999999999999998224, 0.000000000000000000, -99.99999999999998579 ) ) ;
#28997=CARTESIAN_POINT ( 'NONE',  ( -2.121150477449813534E-15, -11.54700538379251284, -164.3750000000000000 ) ) ;
#29000=CARTESIAN_POINT ( 'NONE',  ( 5.405949406249992428, -9.363379034771808662, -64.59375000204836681 ) ) ;
#29002=CARTESIAN_POINT ( 'NONE',  ( -10.81189881249999907, -6.242252689847864744, -168.4687500020483526 ) ) ;
#29008=CARTESIAN_POINT ( 'NONE',  ( -9.999999999999998224, 1.224646799147353059E-15, -94.24999999999998579 ) ) ;
#29010=CARTESIAN_POINT ( 'NONE',  ( -10.81189881249999729, -6.242252689847864744, -117.6562500020483952 ) ) ;
#29011=CARTESIAN_POINT ( 'NONE',  ( -4.999999999999996447, 8.660254037844387298, -142.8750000040967905 ) ) ;
#29012=CARTESIAN_POINT ( 'NONE',  ( 9.999999999999998224, 0.000000000000000000, -158.0000000000000000 ) ) ;
#29018=CARTESIAN_POINT ( 'NONE',  ( -5.405949406249996869, 9.363379034771805109, -61.03125000204837391 ) ) ;
#29025=DIRECTION ( 'NONE',  ( 0.000000000000000000, 0.000000000000000000, 1.000000000000000000 ) ) ;
#29026=( GEOMETRIC_REPRESENTATION_CONTEXT ( 3 ) GLOBAL_UNCERTAINTY_ASSIGNED_CONTEXT ( ( #6998 ) ) GLOBAL_UNIT_ASSIGNED_CONTEXT ( ( #1003, #30782, #40672 ) ) REPRESENTATION_CONTEXT ( 'NONE', 'WORKASPACE' ) );
#29031=EDGE_LOOP ( 'NONE', ( #34559, #24898, #253, #18427 ) ) ;
#29032=ORIENTED_EDGE ( 'NONE', *, *, #38372, .F. ) ;
#29034=CARTESIAN_POINT ( 'NONE',  ( 5.000000000000000000, 8.660254037844385522, -126.6250000040967620 ) ) ;
#29040=CARTESIAN_POINT ( 'NONE',  ( 4.999999999999992006, -8.660254037844389075, -32.24999999999997158 ) ) ;
#29043=CARTESIAN_POINT ( 'NONE',  ( 10.81189881249999729, 0.000000000000000000, -160.3437500020484094 ) ) ;
#29044=CARTESIAN_POINT ( 'NONE',  ( -10.81189881249999729, -6.242252689847864744, -169.9687500020483526 ) ) ;
#29045=CARTESIAN_POINT ( 'NONE',  ( 9.999999999999998224, 0.000000000000000000, -153.5000000000000000 ) ) ;
#29046=CARTESIAN_POINT ( 'NONE',  ( -2.121150477449813534E-15, -11.54700538379251284, -126.8749999999999858 ) ) ;
#29047=CARTESIAN_POINT ( 'NONE',  ( 4.999999999999992006, -8.660254037844389075, -183.7500000000000000 ) ) ;
#29051=CARTESIAN_POINT ( 'NONE',  ( 9.999999999999998224, 1.224646799147353059E-15, -99.99999999999998579 ) ) ;
#29053=CARTESIAN_POINT ( 'NONE',  ( 7.644554776091147741E-16, 12.48450537969573659, -59.65625000204838102 ) ) ;
#29055=CARTESIAN_POINT ( 'NONE',  ( -5.000000000000003553, -8.660254037844383745, -124.0000000000000000 ) ) ;
#29056=( BOUNDED_CURVE ( )  B_SPLINE_CURVE ( 2, ( #38109, #15839, #9388, #18243, #12397, #15630, #21703 ),
 .UNSPECIFIED., .F., .F. ) 
 B_SPLINE_CURVE_WITH_KNOTS ( ( 3, 2, 2, 3 ),
 ( 0.4440298507462688282, 0.4452736318407962135, 0.4465174129353234878, 0.4477611940298508730 ),
 .UNSPECIFIED. ) 
 CURVE ( )  GEOMETRIC_REPRESENTATION_ITEM ( )  RATIONAL_B_SPLINE_CURVE ( ( 0.9999999999999820144, 0.8660254037844566932, 1.000000000000000000, 0.8660254037844387076, 1.000000000000000000, 0.8660254037844267172, 1.000000000000011990 ) ) 
 REPRESENTATION_ITEM ( '' )  );
#29058=CARTESIAN_POINT ( 'NONE',  ( 7.644554776091147741E-16, 12.48450537969573659, -139.1562500020484094 ) ) ;
#29059=CARTESIAN_POINT ( 'NONE',  ( 10.81189881249999551, -6.242252689847874514, -154.6562500020484379 ) ) ;
#29062=CARTESIAN_POINT ( 'NONE',  ( -9.999999999999998224, 1.224646799147353059E-15, -179.7500000000000284 ) ) ;
#29063=CARTESIAN_POINT ( 'NONE',  ( -2.293366432827344421E-15, -12.48450537969573659, -93.21875000204838102 ) ) ;
#29064=ORIENTED_EDGE ( 'NONE', *, *, #3276, .F. ) ;
#29066=CARTESIAN_POINT ( 'NONE',  ( 10.81189881249999907, 6.242252689847868297, -185.7187500020483810 ) ) ;
#29070=CARTESIAN_POINT ( 'NONE',  ( -10.81189881249999729, 6.242252689847871849, -86.40625000204836681 ) ) ;
#29072=CARTESIAN_POINT ( 'NONE',  ( -5.000000000000003553, -8.660254037844383745, -58.37500000409676204 ) ) ;
#29073=CARTESIAN_POINT ( 'NONE',  ( -10.81189881249999729, 6.242252689847871849, -14.21875000204836326 ) ) ;
#29074=ORIENTED_EDGE ( 'NONE', *, *, #26750, .F. ) ;
#29076=AXIS2_PLACEMENT_3D ( 'NONE', #30041, #9749, #39102 ) ;
#29077=CARTESIAN_POINT ( 'NONE',  ( 5.405949406249992428, -9.363379034771808662, -15.28125000204835793 ) ) ;
#29085=ORIENTED_EDGE ( 'NONE', *, *, #16511, .T. ) ;
#29086=CARTESIAN_POINT ( 'NONE',  ( -2.121150477449813534E-15, -11.54700538379251284, -179.7500000040967905 ) ) ;
#29089=CONICAL_SURFACE ( 'NONE', #841, 22.00000000000000711, 0.7853981633974466137 ) ;
#29094=LINE ( 'NONE', #11819, #2926 ) ;
#29095=EDGE_CURVE ( 'NONE', #30038, #26823, #28888, .T. ) ;
#29100=CARTESIAN_POINT ( 'NONE',  ( 5.405949406249992428, -9.363379034771808662, -157.7812500020484094 ) ) ;
#29107=CARTESIAN_POINT ( 'NONE',  ( 10.81189881249999729, 0.000000000000000000, -79.34375000204838102 ) ) ;
#29108=CARTESIAN_POINT ( 'NONE',  ( -10.81189881249999729, 1.324075727343319199E-15, -86.28125000204838102 ) ) ;
#29111=CARTESIAN_POINT ( 'NONE',  ( -5.405949406250003975, -9.363379034771801557, -167.0312500020484094 ) ) ;
#29112=CARTESIAN_POINT ( 'NONE',  ( 10.81189881249999729, 0.000000000000000000, -183.0312500020484094 ) ) ;
#29113=CARTESIAN_POINT ( 'NONE',  ( 4.999999999999992006, -8.660254037844389075, -160.1250000040967905 ) ) ;
#29115=CARTESIAN_POINT ( 'NONE',  ( -5.405949406249996869, 9.363379034771805109, -2.343750002048366810 ) ) ;
#29116=CARTESIAN_POINT ( 'NONE',  ( -4.999999999999996447, 8.660254037844387298, -162.3750000040967905 ) ) ;
#29117=CARTESIAN_POINT ( 'NONE',  ( -2.293366432827344421E-15, -12.48450537969573659, -115.7187500020483952 ) ) ;
#29119=CARTESIAN_POINT ( 'NONE',  ( 7.644554776091147741E-16, 12.48450537969573659, -16.15625000204837391 ) ) ;
#29121=EDGE_CURVE ( 'NONE', #223, #516, #20807, .T. ) ;
#29122=CARTESIAN_POINT ( 'NONE',  ( -5.000000000000003553, -8.660254037844383745, -170.8750000040968189 ) ) ;
#29123=CARTESIAN_POINT ( 'NONE',  ( -2.293366432827344421E-15, -12.48450537969573659, -109.9062500020483952 ) ) ;
#29126=CARTESIAN_POINT ( 'NONE',  ( 10.00000000000000000, 5.773502691896255534, -83.25000000409677625 ) ) ;
#29127=CARTESIAN_POINT ( 'NONE',  ( -2.121150477449813534E-15, -11.54700538379251284, -101.3750000000000000 ) ) ;
#29128=CARTESIAN_POINT ( 'NONE',  ( -5.405949406250003975, -9.363379034771801557, -43.84375000204837391 ) ) ;
#29129=ORIENTED_EDGE ( 'NONE', *, *, #31759, .F. ) ;
#29132=EDGE_CURVE ( 'NONE', #10904, #10629, #22375, .T. ) ;
#29133=CARTESIAN_POINT ( 'NONE',  ( -4.999999999999996447, 8.660254037844387298, -19.87500000409675494 ) ) ;
#29134=CYLINDRICAL_SURFACE ( 'NONE', #33235, 35.00000000000000711 ) ;
#29146=CARTESIAN_POINT ( 'NONE',  ( 10.81189881249999907, 6.242252689847868297, -181.4062500020484379 ) ) ;
#29149=EDGE_CURVE ( 'NONE', #36438, #40511, #2976, .T. ) ;
#29151=CARTESIAN_POINT ( 'NONE',  ( -5.405949406250003975, -9.363379034771801557, -97.84375000204838102 ) ) ;
#29152=CARTESIAN_POINT ( 'NONE',  ( -5.000000000000003553, -8.660254037844383745, -143.5000000000000000 ) ) ;
#29153=CARTESIAN_POINT ( 'NONE',  ( -2.293366432827344421E-15, -12.48450537969573659, -106.9062500020483952 ) ) ;
#29155=CARTESIAN_POINT ( 'NONE',  ( -10.81189881249999729, 1.324075727343319199E-15, -120.5937500020483952 ) ) ;
#29158=CARTESIAN_POINT ( 'NONE',  ( 4.999999999999992006, -8.660254037844389075, -143.2500000000000000 ) ) ;
#29159=CARTESIAN_POINT ( 'NONE',  ( -9.999999999999998224, 5.773502691896259087, -1.374999999999959588 ) ) ;
#29162=CARTESIAN_POINT ( 'NONE',  ( 10.00000000000000000, 5.773502691896255534, -177.7500000040967905 ) ) ;
#29164=CARTESIAN_POINT ( 'NONE',  ( -10.81189881249999729, 6.242252689847871849, -30.71875000204834905 ) ) ;
#29165=CARTESIAN_POINT ( 'NONE',  ( -9.999999999999479527, -5.773502691896549521, -142.5000000040967620 ) ) ;
#29166=CARTESIAN_POINT ( 'NONE',  ( -5.405949406249996869, 9.363379034771805109, -141.8437500020483810 ) ) ;
#29168=CARTESIAN_POINT ( 'NONE',  ( 9.999999999999998224, 0.000000000000000000, -147.5000000000000000 ) ) ;
#29169=CARTESIAN_POINT ( 'NONE',  ( -9.999999999999998224, 1.224646799147353059E-15, -65.74999999999997158 ) ) ;
#29170=CARTESIAN_POINT ( 'NONE',  ( -10.81189881249999729, 6.242252689847871849, -134.4062500020484094 ) ) ;
#29175=CARTESIAN_POINT ( 'NONE',  ( 4.999999999999992006, -8.660254037844389075, -119.6250000040967905 ) ) ;
#29177=CARTESIAN_POINT ( 'NONE',  ( 5.405949406249992428, -9.363379034771808662, -66.09375000204836681 ) ) ;
#29181=CARTESIAN_POINT ( 'NONE',  ( 4.999999999999992006, -8.660254037844389075, -157.1250000040967905 ) ) ;
#29182=CARTESIAN_POINT ( 'NONE',  ( -10.00000000000000000, -5.773502691896251982, -48.00000000409676204 ) ) ;
#29183=CARTESIAN_POINT ( 'NONE',  ( -5.405949406250003975, -9.363379034771801557, -33.53125000204837391 ) ) ;
#29184=( BOUNDED_CURVE ( )  B_SPLINE_CURVE ( 2, ( #37023, #6611, #13910, #10682, #13488, #7463, #30355 ),
 .UNSPECIFIED., .F., .F. ) 
 B_SPLINE_CURVE_WITH_KNOTS ( ( 3, 2, 2, 3 ),
 ( 0.1902985074626866169, 0.1915422885572139744, 0.1927860696517413319, 0.1940298507462686894 ),
 .UNSPECIFIED. ) 
 CURVE ( )  GEOMETRIC_REPRESENTATION_ITEM ( )  RATIONAL_B_SPLINE_CURVE ( ( 0.9999999999999940048, 0.8660254037844447028, 1.000000000000000000, 0.8660254037844387076, 1.000000000000000000, 0.8660254037844357100, 1.000000000000003109 ) ) 
 REPRESENTATION_ITEM ( '' )  );
#29185=DIRECTION ( 'NONE',  ( -1.000000000000000000, 0.000000000000000000, 0.000000000000000000 ) ) ;
#29188=CARTESIAN_POINT ( 'NONE',  ( 0.000000000000000000, 0.000000000000000000, -99.99999999999998579 ) ) ;
#29190=ORIENTED_EDGE ( 'NONE', *, *, #34818, .F. ) ;
#29191=ORIENTED_EDGE ( 'NONE', *, *, #10587, .T. ) ;
#29192=CARTESIAN_POINT ( 'NONE',  ( -10.00000000000076916, 5.773502691895813221, -135.2500000040967905 ) ) ;
#29195=CARTESIAN_POINT ( 'NONE',  ( 7.070501591499376803E-16, 11.54700538379251284, -144.5000000040967905 ) ) ;
#29198=CARTESIAN_POINT ( 'NONE',  ( 4.999999999999992006, -8.660254037844389075, -176.2500000000000284 ) ) ;
#29199=CARTESIAN_POINT ( 'NONE',  ( 5.405949406249992428, -9.363379034771808662, -126.0937500020483668 ) ) ;
#29200=CARTESIAN_POINT ( 'NONE',  ( 5.405949406249992428, -9.363379034771808662, -133.7812500020483810 ) ) ;
#29202=CARTESIAN_POINT ( 'NONE',  ( 10.81189881249999729, 6.242252689847867408, -146.7187500020484094 ) ) ;
#29203=CARTESIAN_POINT ( 'NONE',  ( 10.26323035265758499, -3.418996386904107787, -180.0000000000000000 ) ) ;
#29205=CARTESIAN_POINT ( 'NONE',  ( -9.999999999999998224, 5.773502691896259087, -164.8749999999999716 ) ) ;
#29210=CARTESIAN_POINT ( 'NONE',  ( 10.81189881249999729, 0.000000000000000000, -62.84375000204836681 ) ) ;
#29212=CARTESIAN_POINT ( 'NONE',  ( 10.81189881249999729, 0.000000000000000000, -163.3437500020484094 ) ) ;
#29217=CARTESIAN_POINT ( 'NONE',  ( 10.00000000000000000, 5.773502691896255534, -90.37499999999998579 ) ) ;
#29218=ORIENTED_EDGE ( 'NONE', *, *, #22114, .T. ) ;
#29219=CARTESIAN_POINT ( 'NONE',  ( -10.81189881249999729, 1.324075727343319199E-15, -122.2812500020483952 ) ) ;
#29220=CARTESIAN_POINT ( 'NONE',  ( -9.999999999999998224, 5.773502691896259087, -141.2500000040967905 ) ) ;
#29225=CARTESIAN_POINT ( 'NONE',  ( 7.644554776091147741E-16, 12.48450537969573659, -64.15625000204838102 ) ) ;
#29227=CARTESIAN_POINT ( 'NONE',  ( -9.999999999999998224, 0.000000000000000000, -99.99999999999998579 ) ) ;
#29242=DIRECTION ( 'NONE',  ( -0.000000000000000000, -0.000000000000000000, -1.000000000000000000 ) ) ;
#29243=CARTESIAN_POINT ( 'NONE',  ( -9.999999999999998224, 5.773502691896259087, -26.87499999999998579 ) ) ;
#29246=CARTESIAN_POINT ( 'NONE',  ( -5.405949406249996869, 9.363379034771805109, -147.8437500020483810 ) ) ;
#29247=CARTESIAN_POINT ( 'NONE',  ( 10.81189881249999551, -6.242252689847874514, -172.4687500020483810 ) ) ;
#29248=EDGE_CURVE ( 'NONE', #17582, #23938, #14667, .T. ) ;
#29251=CARTESIAN_POINT ( 'NONE',  ( -5.000000000000003553, -8.660254037844383745, -187.0000000000000000 ) ) ;
#29256=CARTESIAN_POINT ( 'NONE',  ( -5.405949406250003975, -9.363379034771801557, -195.3437500020484094 ) ) ;
#29259=CARTESIAN_POINT ( 'NONE',  ( 5.405949406249992428, -9.363379034771808662, -58.78125000204836681 ) ) ;
#29261=CARTESIAN_POINT ( 'NONE',  ( -2.121150477449813534E-15, -11.54700538379251284, -111.8749999999999858 ) ) ;
#29263=CARTESIAN_POINT ( 'NONE',  ( 5.405949406249992428, -9.363379034771808662, -141.2812500020483810 ) ) ;
#29264=CARTESIAN_POINT ( 'NONE',  ( -2.293366432827344421E-15, -12.48450537969573659, -153.4062500020483810 ) ) ;
#29266=CARTESIAN_POINT ( 'NONE',  ( 5.000000000000000000, 8.660254037844385522, -105.2499999999999858 ) ) ;
#29267=CARTESIAN_POINT ( 'NONE',  ( -5.405949406250003975, -9.363379034771801557, -91.84375000204838102 ) ) ;
#29270=CARTESIAN_POINT ( 'NONE',  ( -2.293366432827344421E-15, -12.48450537969573659, -189.2187500020484094 ) ) ;
#29273=CARTESIAN_POINT ( 'NONE',  ( 10.00000000000012257, -5.773502691896187144, -169.0000000040967620 ) ) ;
#29275=CARTESIAN_POINT ( 'NONE',  ( 5.405949406249999534, 9.363379034771803333, -82.28125000204838102 ) ) ;
#29277=CARTESIAN_POINT ( 'NONE',  ( 4.999999999999992006, -8.660254037844389075, -64.12500000409676204 ) ) ;
#29278=CARTESIAN_POINT ( 'NONE',  ( 7.644554776091147741E-16, 12.48450537969573659, -21.96875000204837391 ) ) ;
#29281=CARTESIAN_POINT ( 'NONE',  ( 10.81189881249999551, -6.242252689847874514, -10.65625000204836859 ) ) ;
#29302=CARTESIAN_POINT ( 'NONE',  ( 10.81189881249999907, 6.242252689847868297, -154.4062500020484094 ) ) ;
#29308=CARTESIAN_POINT ( 'NONE',  ( 5.405949406249992428, -9.363379034771808662, -78.09375000204838102 ) ) ;
#29310=CARTESIAN_POINT ( 'NONE',  ( -5.405949406249996869, 9.363379034771805109, -86.53125000204838102 ) ) ;
#29314=CARTESIAN_POINT ( 'NONE',  ( -5.405949406249996869, 9.363379034771805109, -167.5312500020484094 ) ) ;
#29315=CARTESIAN_POINT ( 'NONE',  ( -10.81189881249999907, -6.242252689847864744, -177.6562500020484094 ) ) ;
#29316=CARTESIAN_POINT ( 'NONE',  ( 9.999999999999998224, 0.000000000000000000, -155.3750000040967905 ) ) ;
#29317=FACE_OUTER_BOUND ( 'NONE', #3740, .T. ) ;
#29318=CARTESIAN_POINT ( 'NONE',  ( -5.405949406249996869, 9.363379034771805109, -6.843750002048371250 ) ) ;
#29320=CARTESIAN_POINT ( 'NONE',  ( -10.81189881249999729, 1.324075727343319199E-15, -117.5937500020483810 ) ) ;
#29322=CARTESIAN_POINT ( 'NONE',  ( 10.81189881249999907, 6.242252689847868297, -16.40625000204837036 ) ) ;
#29325=CARTESIAN_POINT ( 'NONE',  ( 7.644554776091147741E-16, 12.48450537969573659, -110.6562500020483952 ) ) ;
#29327=ORIENTED_EDGE ( 'NONE', *, *, #12535, .T. ) ;
#29329=CARTESIAN_POINT ( 'NONE',  ( 4.999999999999992006, -8.660254037844389075, -88.12500000409677625 ) ) ;
#29330=LINE ( 'NONE', #26096, #16711 ) ;
#29331=CARTESIAN_POINT ( 'NONE',  ( 10.81189881249999729, 0.000000000000000000, -38.84375000204837391 ) ) ;
#29336=CARTESIAN_POINT ( 'NONE',  ( 5.000000000000000000, 8.660254037844385522, -9.625000004096746054 ) ) ;
#29340=ORIENTED_EDGE ( 'NONE', *, *, #13676, .T. ) ;
#29343=AXIS2_PLACEMENT_3D ( 'NONE', #11586, #8384, #3705 ) ;
#29352=CARTESIAN_POINT ( 'NONE',  ( 5.405949406249992428, -9.363379034771808662, -177.2812500020484094 ) ) ;
#29354=CARTESIAN_POINT ( 'NONE',  ( 0.000000000000000000, 0.000000000000000000, -99.99999999999998579 ) ) ;
#29356=CARTESIAN_POINT ( 'NONE',  ( -10.81189881249999729, 1.324075727343319199E-15, -102.5937500020483810 ) ) ;
#29358=CARTESIAN_POINT ( 'NONE',  ( -10.81189881249999907, -6.242252689847864744, -108.6562500020483952 ) ) ;
#29360=CARTESIAN_POINT ( 'NONE',  ( -2.293366432827344421E-15, -12.48450537969573659, -112.7187500020483668 ) ) ;
#29363=CARTESIAN_POINT ( 'NONE',  ( 9.999999999999998224, 0.000000000000000000, -140.0000000000000000 ) ) ;
#29364=CARTESIAN_POINT ( 'NONE',  ( 7.070501591499377789E-16, 11.54700538379251284, -7.624999999999965361 ) ) ;
#29367=CARTESIAN_POINT ( 'NONE',  ( -9.999999999999998224, 1.224646799147353059E-15, -180.1250000040968189 ) ) ;
#29369=CARTESIAN_POINT ( 'NONE',  ( -10.81189881249999907, -6.242252689847864744, -27.46875000204837391 ) ) ;
#29371=CARTESIAN_POINT ( 'NONE',  ( 5.405949406249999534, 9.363379034771803333, -137.5937500020483810 ) ) ;
#29375=CARTESIAN_POINT ( 'NONE',  ( 9.999999999999996447, -5.773502691896262640, -65.12499999999998579 ) ) ;
#29376=CARTESIAN_POINT ( 'NONE',  ( 10.81189881249999907, 6.242252689847868297, -134.9062500020483810 ) ) ;
#29380=CARTESIAN_POINT ( 'NONE',  ( 9.999999999999996447, -5.773502691896262640, -110.5000000040967763 ) ) ;
#29382=CARTESIAN_POINT ( 'NONE',  ( 7.644554776091147741E-16, 12.48450537969573659, -68.46875000204838102 ) ) ;
#29383=ORIENTED_EDGE ( 'NONE', *, *, #12974, .T. ) ;
#29386=EDGE_CURVE ( 'NONE', #40028, #15924, #9862, .T. ) ;
#29389=CARTESIAN_POINT ( 'NONE',  ( 9.999999999999479527, 5.773502691896553074, -119.2500000040967620 ) ) ;
#29390=CARTESIAN_POINT ( 'NONE',  ( 9.999999999999996447, -5.773502691896262640, -35.50000000409675494 ) ) ;
#29391=CARTESIAN_POINT ( 'NONE',  ( 10.81189881249999907, 6.242252689847868297, -37.40625000204836681 ) ) ;
#29410=CARTESIAN_POINT ( 'NONE',  ( -2.121150477449813534E-15, -11.54700538379251284, -116.3749999999999858 ) ) ;
#29411=CARTESIAN_POINT ( 'NONE',  ( -10.81189881249999907, -6.242252689847864744, -126.4687500020483810 ) ) ;
#29412=CARTESIAN_POINT ( 'NONE',  ( 5.405949406249999534, 9.363379034771803333, -130.2812500020483810 ) ) ;
#29414=CARTESIAN_POINT ( 'NONE',  ( 5.405949406249999534, 9.363379034771803333, -139.0937500020483810 ) ) ;
#29415=CARTESIAN_POINT ( 'NONE',  ( 10.83509278446304691, 0.07525214450409632716, -180.0000000000000000 ) ) ;
#29417=CARTESIAN_POINT ( 'NONE',  ( 4.999999999999992006, -8.660254037844389075, -159.7500000000000000 ) ) ;
#29421=CARTESIAN_POINT ( 'NONE',  ( -5.405949406250003975, -9.363379034771801557, -49.84375000204838102 ) ) ;
#29423=CARTESIAN_POINT ( 'NONE',  ( -5.405949406249996869, 9.363379034771805109, -164.3437500020484094 ) ) ;
#29426=DIRECTION ( 'NONE',  ( -0.000000000000000000, -0.000000000000000000, -1.000000000000000000 ) ) ;
#29428=CARTESIAN_POINT ( 'NONE',  ( -10.00000000000000000, -5.773502691896251982, -89.62499999999997158 ) ) ;
#29431=CARTESIAN_POINT ( 'NONE',  ( 10.81189881249999729, 0.000000000000000000, -121.5312500020483952 ) ) ;
#29432=CARTESIAN_POINT ( 'NONE',  ( 7.070501591499377789E-16, 11.54700538379251284, -134.0000000040967905 ) ) ;
#29433=CARTESIAN_POINT ( 'NONE',  ( 9.999999999999742428, 5.773502691896404748, -159.3749999999999716 ) ) ;
#29438=CARTESIAN_POINT ( 'NONE',  ( -10.81189881249999729, 1.324075727343319199E-15, -62.28125000204837391 ) ) ;
#29442=CARTESIAN_POINT ( 'NONE',  ( -10.00000000000012434, 5.773502691896184480, -166.7500000040967905 ) ) ;
#29443=CARTESIAN_POINT ( 'NONE',  ( -4.999999999999996447, 8.660254037844387298, -171.3750000040968189 ) ) ;
#29444=ORIENTED_EDGE ( 'NONE', *, *, #25847, .F. ) ;
#29456=CARTESIAN_POINT ( 'NONE',  ( 9.999999999999998224, 0.000000000000000000, -111.8750000040967763 ) ) ;
#29457=CARTESIAN_POINT ( 'NONE',  ( -5.000000000000003553, -8.660254037844383745, -32.49999999999997158 ) ) ;
#29460=CARTESIAN_POINT ( 'NONE',  ( 5.405949406249992428, -9.363379034771808662, -147.0937500020483810 ) ) ;
#29461=CARTESIAN_POINT ( 'NONE',  ( -10.81189881249999729, -6.242252689847864744, -166.9687500020484094 ) ) ;
#29463=CYLINDRICAL_SURFACE ( 'NONE', #35038, 9.999999999999998224 ) ;
#29464=CARTESIAN_POINT ( 'NONE',  ( -2.121150477449813534E-15, -11.54700538379251284, -185.3750000000000284 ) ) ;
#29469=CARTESIAN_POINT ( 'NONE',  ( 10.81189881249999907, 6.242252689847868297, -182.7187500020484094 ) ) ;
#29471=CARTESIAN_POINT ( 'NONE',  ( 5.405949406249999534, 9.363379034771803333, -62.78125000204837391 ) ) ;
#29473=CARTESIAN_POINT ( 'NONE',  ( 9.999999999999996447, -5.773502691896262640, -111.6249999999999858 ) ) ;
#29475=CARTESIAN_POINT ( 'NONE',  ( 5.405949406249999534, 9.363379034771803333, -139.2812500020483810 ) ) ;
#29476=CARTESIAN_POINT ( 'NONE',  ( 5.405949406249999534, 9.363379034771803333, -155.7812500020484094 ) ) ;
#29479=CARTESIAN_POINT ( 'NONE',  ( -2.293366432827344421E-15, -12.48450537969573659, -87.21875000204838102 ) ) ;
#29480=VECTOR ( 'NONE', #26908, 1000.000000000000000 ) ;
#29483=CARTESIAN_POINT ( 'NONE',  ( -10.81189881249999729, 1.324075727343319199E-15, -188.0937500020483810 ) ) ;
#29485=VECTOR ( 'NONE', #6842, 1000.000000000000000 ) ;
#29486=CARTESIAN_POINT ( 'NONE',  ( -10.00000000000000000, -5.773502691896252870, -169.5000000040967905 ) ) ;
#29488=CARTESIAN_POINT ( 'NONE',  ( 10.81189881249999907, 6.242252689847868297, -80.90625000204839523 ) ) ;
#29490=CARTESIAN_POINT ( 'NONE',  ( 9.999999999999996447, -5.773502691896262640, -59.50000000409677625 ) ) ;
#29491=CARTESIAN_POINT ( 'NONE',  ( 5.405949406249992428, -9.363379034771808662, -21.09375000204835615 ) ) ;
#29494=CARTESIAN_POINT ( 'NONE',  ( 5.405949406249999534, 9.363379034771803333, -16.28125000204835970 ) ) ;
#29496=CARTESIAN_POINT ( 'NONE',  ( 5.000000000000000000, 8.660254037844385522, -114.6250000040967763 ) ) ;
#29497=DIRECTION ( 'NONE',  ( -1.000000000000000000, 0.000000000000000000, 0.000000000000000000 ) ) ;
#29503=CARTESIAN_POINT ( 'NONE',  ( 10.81189881249999551, -6.242252689847874514, -100.4687500020483952 ) ) ;
#29510=CARTESIAN_POINT ( 'NONE',  ( 9.999999999999998224, 0.000000000000000000, -114.8750000040967905 ) ) ;
#29511=AXIS2_PLACEMENT_3D ( 'NONE', #17976, #755, #41058 ) ;
#29517=CARTESIAN_POINT ( 'NONE',  ( -5.405949406250003975, -9.363379034771801557, -159.5312500020484094 ) ) ;
#29519=CARTESIAN_POINT ( 'NONE',  ( -10.00000000000025580, 5.773502691896109873, -121.3749999999999858 ) ) ;
#29523=CARTESIAN_POINT ( 'NONE',  ( 5.405949406249992428, -9.363379034771808662, -75.09375000204838102 ) ) ;
#29524=CARTESIAN_POINT ( 'NONE',  ( 10.81189881249999907, 6.242252689847868297, -85.40625000204839523 ) ) ;
#29527=CARTESIAN_POINT ( 'NONE',  ( 5.405949406249999534, 9.363379034771803333, -167.7812500020484094 ) ) ;
#29528=CARTESIAN_POINT ( 'NONE',  ( -10.81189881249999729, 6.242252689847871849, -176.4062500020484094 ) ) ;
#29529=CARTESIAN_POINT ( 'NONE',  ( -9.999999999999998224, 1.224646799147353059E-15, -153.1250000040967905 ) ) ;
#29531=CARTESIAN_POINT ( 'NONE',  ( -5.405949406249996869, 9.363379034771805109, -5.343750002048369474 ) ) ;
#29533=CARTESIAN_POINT ( 'NONE',  ( 7.644554776091147741E-16, 12.48450537969573659, -114.9687500020483668 ) ) ;
#29535=CARTESIAN_POINT ( 'NONE',  ( -5.405949406250003975, -9.363379034771801557, -11.03125000204835438 ) ) ;
#29538=CARTESIAN_POINT ( 'NONE',  ( -5.405949406249996869, 9.363379034771805109, -112.0312500020483810 ) ) ;
#29541=CARTESIAN_POINT ( 'NONE',  ( 9.999999999999998224, 0.000000000000000000, -81.87500000409676204 ) ) ;
#29543=CARTESIAN_POINT ( 'NONE',  ( -5.405949406249996869, 9.363379034771805109, -39.84375000204837391 ) ) ;
#29547=AXIS2_PLACEMENT_3D ( 'NONE', #23202, #16485, #22565 ) ;
#29548=CARTESIAN_POINT ( 'NONE',  ( 9.999999999999998224, 0.000000000000000000, -11.37500000409674783 ) ) ;
#29551=ORIENTED_EDGE ( 'NONE', *, *, #25109, .T. ) ;
#29563=CARTESIAN_POINT ( 'NONE',  ( 7.644554776091147741E-16, 12.48450537969573659, -181.1562500020484094 ) ) ;
#29565=EDGE_CURVE ( 'NONE', #20303, #9851, #27664, .T. ) ;
#29567=AXIS2_PLACEMENT_3D ( 'NONE', #39125, #35692, #35899 ) ;
#29568=CARTESIAN_POINT ( 'NONE',  ( 10.81189881249999551, -6.242252689847874514, -100.4687500020483952 ) ) ;
#29570=CARTESIAN_POINT ( 'NONE',  ( -10.81189881249999729, 6.242252689847871849, -108.9062500020483810 ) ) ;
#29572=CARTESIAN_POINT ( 'NONE',  ( -5.405949406250003975, -9.363379034771801557, -111.3437500020483810 ) ) ;
#29576=CARTESIAN_POINT ( 'NONE',  ( 5.000000000000000000, 8.660254037844385522, -139.7499999999999716 ) ) ;
#29577=CARTESIAN_POINT ( 'NONE',  ( -9.999999999999998224, 5.773502691896259087, -2.874999999999960920 ) ) ;
#29581=DESIGN_CONTEXT ( 'detailed design', #3865, 'design' ) ;
#29582=CARTESIAN_POINT ( 'NONE',  ( 5.000000000000000000, 8.660254037844385522, -179.1250000040968189 ) ) ;
#29584=CARTESIAN_POINT ( 'NONE',  ( -5.405949406250003975, -9.363379034771801557, -33.34375000204836681 ) ) ;
#29586=CARTESIAN_POINT ( 'NONE',  ( -2.293366432827344421E-15, -12.48450537969573659, -141.2187500020483810 ) ) ;
#29588=CARTESIAN_POINT ( 'NONE',  ( 10.81189881249999551, -6.242252689847874514, -34.65625000204835970 ) ) ;
#29589=CARTESIAN_POINT ( 'NONE',  ( 0.000000000000000000, 0.000000000000000000, -99.99999999999998579 ) ) ;
#29590=CARTESIAN_POINT ( 'NONE',  ( -9.999999999999998224, 5.773502691896259087, -68.87499999999998579 ) ) ;
#29591=CARTESIAN_POINT ( 'NONE',  ( 10.81189881249999729, 0.000000000000000000, -130.5312500020484094 ) ) ;
#29593=ORIENTED_EDGE ( 'NONE', *, *, #40713, .F. ) ;
#29595=CARTESIAN_POINT ( 'NONE',  ( 9.999999999999998224, 0.000000000000000000, -131.0000000000000000 ) ) ;
#29596=CARTESIAN_POINT ( 'NONE',  ( 9.999999999999998224, 0.000000000000000000, -110.3750000040967763 ) ) ;
#29597=CARTESIAN_POINT ( 'NONE',  ( -4.999999999999996447, 8.660254037844387298, -100.8750000040967905 ) ) ;
#29598=CARTESIAN_POINT ( 'NONE',  ( 10.81189881249999907, 6.242252689847868297, -68.71875000204838102 ) ) ;
#29603=CARTESIAN_POINT ( 'NONE',  ( 9.999999999999998224, 0.000000000000000000, -125.3750000040967905 ) ) ;
#29604=CARTESIAN_POINT ( 'NONE',  ( 5.000000000000000000, 8.660254037844385522, -38.12500000409676915 ) ) ;
#29607=FACE_OUTER_BOUND ( 'NONE', #19656, .T. ) ;
#29611=ORIENTED_EDGE ( 'NONE', *, *, #39233, .T. ) ;
#29621=CARTESIAN_POINT ( 'NONE',  ( -5.405949406250003975, -9.363379034771801557, -127.8437500020483952 ) ) ;
#29622=CARTESIAN_POINT ( 'NONE',  ( -10.81189881249999729, 6.242252689847871849, -135.9062500020484094 ) ) ;
#29624=CARTESIAN_POINT ( 'NONE',  ( 5.405949406249992428, -9.363379034771808662, -141.0937500020483810 ) ) ;
#29627=CARTESIAN_POINT ( 'NONE',  ( 4.999999999999992006, -8.660254037844389075, -102.7500000000000000 ) ) ;
#29628=CARTESIAN_POINT ( 'NONE',  ( 10.00000000000000000, 5.773502691896255534, -162.3750000000000000 ) ) ;
#29632=CARTESIAN_POINT ( 'NONE',  ( 10.81189881249999729, 0.000000000000000000, -55.34375000204835970 ) ) ;
#29634=CARTESIAN_POINT ( 'NONE',  ( 5.405949406249999534, 9.363379034771803333, -163.0937500020484094 ) ) ;
#29640=CARTESIAN_POINT ( 'NONE',  ( -5.000000000000003553, -8.660254037844383745, -92.49999999999998579 ) ) ;
#29641=ORIENTED_EDGE ( 'NONE', *, *, #37969, .F. ) ;
#29642=CARTESIAN_POINT ( 'NONE',  ( -2.293366432827344421E-15, -12.48450537969573659, -106.9062500020483810 ) ) ;
#29643=CARTESIAN_POINT ( 'NONE',  ( -2.121150477449813534E-15, -11.54700538379251284, -130.2500000040967905 ) ) ;
#29644=CARTESIAN_POINT ( 'NONE',  ( 0.000000000000000000, 0.000000000000000000, -99.99999999999998579 ) ) ;
#29650=CARTESIAN_POINT ( 'NONE',  ( 10.81189881249999907, 6.242252689847868297, -56.90625000204837391 ) ) ;
#29655=CARTESIAN_POINT ( 'NONE',  ( 7.070501591499376803E-16, 11.54700538379251284, -167.0000000040967905 ) ) ;
#29663=EDGE_LOOP ( 'NONE', ( #33389, #39835, #39720, #19486 ) ) ;
#29665=EDGE_CURVE ( 'NONE', #13539, #35190, #29056, .T. ) ;
#29672=CARTESIAN_POINT ( 'NONE',  ( 9.999999999999996447, -5.773502691896262640, -27.62499999999998224 ) ) ;
#29675=CARTESIAN_POINT ( 'NONE',  ( -10.81189881249999729, 6.242252689847871849, -153.7187500020483526 ) ) ;
#29677=CARTESIAN_POINT ( 'NONE',  ( 7.644554776091147741E-16, 12.48450537969573659, -165.9687500020483810 ) ) ;
#29680=CARTESIAN_POINT ( 'NONE',  ( -4.999999999999996447, 8.660254037844387298, -189.0000000000000000 ) ) ;
#29682=FACE_OUTER_BOUND ( 'NONE', #41430, .T. ) ;
#29685=CARTESIAN_POINT ( 'NONE',  ( -5.405949406249996869, 9.363379034771805109, -183.8437500020483810 ) ) ;
#29687=CARTESIAN_POINT ( 'NONE',  ( 10.81189881249999729, 0.000000000000000000, -61.53125000204837391 ) ) ;
#29689=CARTESIAN_POINT ( 'NONE',  ( 9.999999999999998224, 0.000000000000000000, -114.4999999999999858 ) ) ;
#29691=CARTESIAN_POINT ( 'NONE',  ( 10.81189881249999729, 6.242252689847867408, -142.4062500020484094 ) ) ;
#29692=CARTESIAN_POINT ( 'NONE',  ( -5.405949406249996869, 9.363379034771805109, -152.5312500020484094 ) ) ;
#29695=CARTESIAN_POINT ( 'NONE',  ( 10.81189881249999729, 0.000000000000000000, -91.34375000204838102 ) ) ;
#29698=CARTESIAN_POINT ( 'NONE',  ( -5.405949406249996869, 9.363379034771805109, -191.3437500020484094 ) ) ;
#29702=CARTESIAN_POINT ( 'NONE',  ( -10.81189881249999907, -6.242252689847864744, -83.15625000204836681 ) ) ;
#29705=CARTESIAN_POINT ( 'NONE',  ( -2.121150477449813534E-15, -11.54700538379251284, -59.75000000409678336 ) ) ;
#29706=CARTESIAN_POINT ( 'NONE',  ( -2.293366432827344421E-15, -12.48450537969573659, -18.21875000204836681 ) ) ;
#29710=CARTESIAN_POINT ( 'NONE',  ( -5.405949406250003975, -9.363379034771801557, -14.03125000204835615 ) ) ;
#29712=FACE_OUTER_BOUND ( 'NONE', #35622, .T. ) ;
#29713=AXIS2_PLACEMENT_3D ( 'NONE', #4007, #30772, #40661 ) ;
#29727=CARTESIAN_POINT ( 'NONE',  ( -9.999999999999479527, -5.773502691896549521, -115.5000000040967763 ) ) ;
#29731=CARTESIAN_POINT ( 'NONE',  ( 10.00000000000025402, -5.773502691896113426, -121.0000000040967763 ) ) ;
#29733=CARTESIAN_POINT ( 'NONE',  ( -10.81189881249999907, -6.242252689847864744, -146.1562500020484094 ) ) ;
#29740=CARTESIAN_POINT ( 'NONE',  ( -10.81189881249999729, 6.242252689847871849, -77.21875000204838102 ) ) ;
#29741=CARTESIAN_POINT ( 'NONE',  ( 5.405949406249992428, -9.363379034771808662, -84.28125000204838102 ) ) ;
#29744=CARTESIAN_POINT ( 'NONE',  ( -10.81189881249999729, 1.324075727343319199E-15, -162.7812500020484094 ) ) ;
#29745=CARTESIAN_POINT ( 'NONE',  ( 10.81189881249999907, 6.242252689847868297, -181.4062500020484379 ) ) ;
#29747=CARTESIAN_POINT ( 'NONE',  ( -5.000000000000003553, -8.660254037844383745, -152.8750000040967905 ) ) ;
#29749=CARTESIAN_POINT ( 'NONE',  ( 7.644554776091147741E-16, 12.48450537969573659, -8.468750002048359704 ) ) ;
#29750=CARTESIAN_POINT ( 'NONE',  ( 9.999999999999998224, 0.000000000000000000, -104.3750000040967763 ) ) ;
#29751=CARTESIAN_POINT ( 'NONE',  ( 10.81189881249999551, -6.242252689847874514, -113.9687500020483810 ) ) ;
#29753=CARTESIAN_POINT ( 'NONE',  ( -10.81189881249999729, 1.324075727343319199E-15, -9.781250002048352599 ) ) ;
#29755=DIRECTION ( 'NONE',  ( -0.000000000000000000, -0.000000000000000000, -1.000000000000000000 ) ) ;
#29756=CARTESIAN_POINT ( 'NONE',  ( -5.405949406250003975, -9.363379034771801557, -105.5312500020483810 ) ) ;
#29759=CARTESIAN_POINT ( 'NONE',  ( 9.999999999999996447, -5.773502691896262640, -86.50000000409676204 ) ) ;
#29761=CARTESIAN_POINT ( 'NONE',  ( 7.644554776091147741E-16, 12.48450537969573659, -44.46875000204836681 ) ) ;
#29766=CARTESIAN_POINT ( 'NONE',  ( 9.999999999999998224, 0.000000000000000000, -15.87500000409675138 ) ) ;
#29767=ADVANCED_FACE ( 'NONE', ( #19101 ), #22346, .F. ) ;
#29774=VERTEX_POINT ( 'NONE', #34674 ) ;
#29785=CARTESIAN_POINT ( 'NONE',  ( 5.405949406249999534, 9.363379034771803333, -178.2812500020484094 ) ) ;
#29788=CARTESIAN_POINT ( 'NONE',  ( 10.81189881249999729, 0.000000000000000000, -103.3437500020483668 ) ) ;
#29790=CARTESIAN_POINT ( 'NONE',  ( 7.644554776091147741E-16, 12.48450537969573659, -109.1562500020483810 ) ) ;
#29792=CARTESIAN_POINT ( 'NONE',  ( -10.81189881249999729, 6.242252689847871849, -111.7187500020483810 ) ) ;
#29797=CARTESIAN_POINT ( 'NONE',  ( 4.999999999999992006, -8.660254037844389075, -132.7499999999999716 ) ) ;
#29798=CARTESIAN_POINT ( 'NONE',  ( -2.121150477449813534E-15, -11.54700538379251284, -8.374999999999964473 ) ) ;
#29801=CARTESIAN_POINT ( 'NONE',  ( -9.999999999999998224, 5.773502691896259087, -181.7500000040967905 ) ) ;
#29803=CARTESIAN_POINT ( 'NONE',  ( 10.81189881249999551, -6.242252689847874514, -32.96875000204835260 ) ) ;
#29805=CARTESIAN_POINT ( 'NONE',  ( -10.81189881249999729, 1.324075727343319199E-15, -140.0937500020483810 ) ) ;
#29807=CARTESIAN_POINT ( 'NONE',  ( 7.644554776091147741E-16, 12.48450537969573659, -40.15625000204836681 ) ) ;
#29809=CARTESIAN_POINT ( 'NONE',  ( 4.999999999999992006, -8.660254037844389075, -63.74999999999997158 ) ) ;
#29810=CARTESIAN_POINT ( 'NONE',  ( 5.405949406249992428, -9.363379034771808662, -129.2812500020483810 ) ) ;
#29813=CARTESIAN_POINT ( 'NONE',  ( 9.999999999999479527, 5.773502691896553074, -142.8749999999999716 ) ) ;
#29814=CARTESIAN_POINT ( 'NONE',  ( -5.000000000000003553, -8.660254037844383745, -106.3750000040967763 ) ) ;
#29815=CARTESIAN_POINT ( 'NONE',  ( -5.000000000000003553, -8.660254037844383745, -146.5000000000000000 ) ) ;
#29816=CARTESIAN_POINT ( 'NONE',  ( -10.81189881249999729, 6.242252689847871849, -63.71875000204838102 ) ) ;
#29817=VERTEX_POINT ( 'NONE', #41550 ) ;
#29823=CARTESIAN_POINT ( 'NONE',  ( 9.999999999999998224, 0.000000000000000000, -35.37500000409676915 ) ) ;
#29830=( BOUNDED_CURVE ( )  B_SPLINE_CURVE ( 2, ( #9160, #15613, #21471, #35292, #28818, #41948, #41310 ),
 .UNSPECIFIED., .F., .F. ) 
 B_SPLINE_CURVE_WITH_KNOTS ( ( 3, 2, 2, 3 ),
 ( 0.4589552238805971740, 0.4601990049751245593, 0.4614427860696518890, 0.4626865671641792743 ),
 .UNSPECIFIED. ) 
 CURVE ( )  GEOMETRIC_REPRESENTATION_ITEM ( )  RATIONAL_B_SPLINE_CURVE ( ( 0.9999999999999820144, 0.8660254037844566932, 1.000000000000000000, 0.8660254037844387076, 1.000000000000000000, 0.8660254037844207220, 1.000000000000017986 ) ) 
 REPRESENTATION_ITEM ( '' )  );
#29831=ORIENTED_EDGE ( 'NONE', *, *, #11491, .T. ) ;
#29832=EDGE_LOOP ( 'NONE', ( #11799, #33053, #21205, #22019 ) ) ;
#29837=CARTESIAN_POINT ( 'NONE',  ( -9.999999999999998224, 1.224646799147353059E-15, -144.1250000040967905 ) ) ;
#29841=CARTESIAN_POINT ( 'NONE',  ( 5.405949406249992428, -9.363379034771808662, -124.5937500020483952 ) ) ;
#29842=CARTESIAN_POINT ( 'NONE',  ( 5.405949406249999534, 9.363379034771803333, -128.7812500020483810 ) ) ;
#29844=CARTESIAN_POINT ( 'NONE',  ( -10.81189881249999729, 6.242252689847871849, -137.2187500020483810 ) ) ;
#29847=CARTESIAN_POINT ( 'NONE',  ( -5.000000000000003553, -8.660254037844383745, -164.5000000000000000 ) ) ;
#29848=DIRECTION ( 'NONE',  ( -0.000000000000000000, -0.000000000000000000, -1.000000000000000000 ) ) ;
#29851=CARTESIAN_POINT ( 'NONE',  ( -10.81189881249999729, 6.242252689847871849, -53.21875000204836681 ) ) ;
#29853=CARTESIAN_POINT ( 'NONE',  ( 10.81189881249999551, -6.242252689847874514, -161.9687500020484094 ) ) ;
#29858=CARTESIAN_POINT ( 'NONE',  ( 7.070501591499377789E-16, 11.54700538379251284, -93.12500000000000000 ) ) ;
#29860=CARTESIAN_POINT ( 'NONE',  ( 7.644554776091147741E-16, 12.48450537969573659, -113.6562500020483952 ) ) ;
#29861=CARTESIAN_POINT ( 'NONE',  ( -9.999999999999998224, 5.773502691896259087, -132.2500000040967905 ) ) ;
#29862=DIRECTION ( 'NONE',  ( -1.000000000000000000, 0.000000000000000000, 0.000000000000000000 ) ) ;
#29865=CARTESIAN_POINT ( 'NONE',  ( 10.81189881249999907, 6.242252689847868297, -50.90625000204837391 ) ) ;
#29870=ADVANCED_FACE ( 'NONE', ( #2707 ), #5521, .F. ) ;
#29872=EDGE_CURVE ( 'NONE', #38366, #19560, #3963, .T. ) ;
#29883=CARTESIAN_POINT ( 'NONE',  ( -2.121150477449813534E-15, -11.54700538379251284, -134.3750000000000000 ) ) ;
#29888=CARTESIAN_POINT ( 'NONE',  ( 5.405949406249992428, -9.363379034771808662, -148.5937500020483810 ) ) ;
#29889=CARTESIAN_POINT ( 'NONE',  ( 10.81189881249999729, 6.242252689847867408, -166.2187500020483810 ) ) ;
#29890=CARTESIAN_POINT ( 'NONE',  ( -10.00000000000076916, 5.773502691895813221, -106.7500000040967620 ) ) ;
#29891=CARTESIAN_POINT ( 'NONE',  ( 10.00000000000012257, -5.773502691896188921, -161.5000000040968189 ) ) ;
#29892=CARTESIAN_POINT ( 'NONE',  ( -9.999999999999998224, 1.224646799147353059E-15, -190.2500000000000000 ) ) ;
#29896=FACE_OUTER_BOUND ( 'NONE', #6972, .T. ) ;
#29897=CARTESIAN_POINT ( 'NONE',  ( -2.293366432827344421E-15, -12.48450537969573659, -186.2187500020484094 ) ) ;
#29898=EDGE_CURVE ( 'NONE', #516, #223, #12335, .T. ) ;
#29901=CARTESIAN_POINT ( 'NONE',  ( 5.405949406249992428, -9.363379034771808662, -55.78125000204836681 ) ) ;
#29903=CARTESIAN_POINT ( 'NONE',  ( 9.999999999999998224, 0.000000000000000000, -112.9999999999999858 ) ) ;
#29905=CARTESIAN_POINT ( 'NONE',  ( -10.81189881249999729, 6.242252689847871849, -134.4062500020483810 ) ) ;
#29906=CARTESIAN_POINT ( 'NONE',  ( -2.293366432827344421E-15, -12.48450537969573659, -151.9062500020483810 ) ) ;
#29909=CARTESIAN_POINT ( 'NONE',  ( -2.293366432827344421E-15, -12.48450537969573659, -81.21875000204838102 ) ) ;
#29912=CARTESIAN_POINT ( 'NONE',  ( 7.644554776091147741E-16, 12.48450537969573659, -179.4687500020483810 ) ) ;
#29914=CARTESIAN_POINT ( 'NONE',  ( -2.121150477449813534E-15, -11.54700538379251284, -171.8750000000000284 ) ) ;
#29915=CARTESIAN_POINT ( 'NONE',  ( -9.999999999999998224, 1.224646799147353059E-15, -175.6250000040968189 ) ) ;
#29916=CARTESIAN_POINT ( 'NONE',  ( -10.81189881249999729, 6.242252689847871849, -77.40625000204838102 ) ) ;
#29918=CARTESIAN_POINT ( 'NONE',  ( -2.121150477449813534E-15, -11.54700538379251284, -56.75000000409676915 ) ) ;
#29919=CARTESIAN_POINT ( 'NONE',  ( -10.81189881249999907, -6.242252689847864744, -9.468750002048357928 ) ) ;
#29922=CARTESIAN_POINT ( 'NONE',  ( -5.405949406249996869, 9.363379034771805109, -16.03125000204835970 ) ) ;
#29925=EDGE_CURVE ( 'NONE', #27517, #34879, #1202, .T. ) ;
#29927=FACE_OUTER_BOUND ( 'NONE', #11115, .T. ) ;
#29935=CARTESIAN_POINT ( 'NONE',  ( -5.000000000000003553, -8.660254037844383745, -154.0000000000000000 ) ) ;
#29937=ORIENTED_EDGE ( 'NONE', *, *, #42299, .T. ) ;
#29942=CARTESIAN_POINT ( 'NONE',  ( 4.999999999999992006, -8.660254037844389075, -115.1250000040967905 ) ) ;
#29945=EDGE_CURVE ( 'NONE', #25155, #10539, #33479, .T. ) ;
#29949=CARTESIAN_POINT ( 'NONE',  ( -5.405949406250003975, -9.363379034771801557, -147.5312500020483810 ) ) ;
#29956=CARTESIAN_POINT ( 'NONE',  ( 7.644554776091147741E-16, 12.48450537969573659, -72.96875000204835260 ) ) ;
#29957=CARTESIAN_POINT ( 'NONE',  ( 7.644554776091147741E-16, 12.48450537969573659, -76.15625000204839523 ) ) ;
#29959=FACE_OUTER_BOUND ( 'NONE', #25746, .T. ) ;
#29960=CARTESIAN_POINT ( 'NONE',  ( 10.81189881249999729, 6.242252689847867408, -158.9062500020483810 ) ) ;
#29961=CARTESIAN_POINT ( 'NONE',  ( -5.405949406250003975, -9.363379034771801557, -176.0312500020483810 ) ) ;
#29963=CARTESIAN_POINT ( 'NONE',  ( -5.405949406249996869, 9.363379034771805109, -8.343750002048345493 ) ) ;
#29965=CARTESIAN_POINT ( 'NONE',  ( 5.405949406249999534, 9.363379034771803333, -109.0937500020483810 ) ) ;
#29967=CARTESIAN_POINT ( 'NONE',  ( 10.81189881249999729, 0.000000000000000000, -9.031250002048352599 ) ) ;
#29970=CARTESIAN_POINT ( 'NONE',  ( 10.81189881249999907, 6.242252689847868297, -104.9062500020483952 ) ) ;
#29973=CARTESIAN_POINT ( 'NONE',  ( 5.000000000000000000, 8.660254037844385522, -87.62500000409677625 ) ) ;
#29975=CARTESIAN_POINT ( 'NONE',  ( 10.81189881249999729, 0.000000000000000000, -41.84375000204837391 ) ) ;
#29980=CARTESIAN_POINT ( 'NONE',  ( -5.000000000000003553, -8.660254037844383745, -10.37500000409674605 ) ) ;
#29983=CARTESIAN_POINT ( 'NONE',  ( 0.000000000000000000, 0.000000000000000000, -99.99999999999998579 ) ) ;
#29995=CARTESIAN_POINT ( 'NONE',  ( -2.293366432827344421E-15, -12.48450537969573659, -174.4062500020483810 ) ) ;
#29996=CARTESIAN_POINT ( 'NONE',  ( -4.999999999999996447, 8.660254037844387298, -154.8750000040967905 ) ) ;
#29998=CARTESIAN_POINT ( 'NONE',  ( -10.81189881249999907, -6.242252689847864744, -93.46875000204836681 ) ) ;
#29999=CARTESIAN_POINT ( 'NONE',  ( -9.999999999999998224, 1.224646799147353059E-15, -112.6250000040967763 ) ) ;
#30000=CARTESIAN_POINT ( 'NONE',  ( -10.81189881249999729, 6.242252689847871849, -104.4062500020483810 ) ) ;
#30002=CARTESIAN_POINT ( 'NONE',  ( -5.405949406250003975, -9.363379034771801557, -114.3437500020483810 ) ) ;
#30005=CARTESIAN_POINT ( 'NONE',  ( 9.999999999999227285, 5.773502691896701400, -108.3749999999999289 ) ) ;
#30006=CARTESIAN_POINT ( 'NONE',  ( 10.00000000000051159, -5.773502691895965988, -113.5000000040967620 ) ) ;
#30007=CARTESIAN_POINT ( 'NONE',  ( -5.000000000000003553, -8.660254037844383745, -0.9999999999999731326 ) ) ;
#30010=CARTESIAN_POINT ( 'NONE',  ( -2.121150477449813534E-15, -11.54700538379251284, -181.2500000040967905 ) ) ;
#30012=CARTESIAN_POINT ( 'NONE',  ( -5.405949406250003975, -9.363379034771801557, -31.84375000204836681 ) ) ;
#30014=CARTESIAN_POINT ( 'NONE',  ( 5.405949406249992428, -9.363379034771808662, -138.0937500020483810 ) ) ;
#30016=CARTESIAN_POINT ( 'NONE',  ( -2.293366432827344421E-15, -12.48450537969573659, -34.90625000204835970 ) ) ;
#30017=CARTESIAN_POINT ( 'NONE',  ( 9.999999999999998224, 1.224646799147353059E-15, -99.99999999999998579 ) ) ;
#30018=CARTESIAN_POINT ( 'NONE',  ( 10.00000000000000000, 5.773502691896255534, -57.37499999999997868 ) ) ;
#30019=CARTESIAN_POINT ( 'NONE',  ( -2.293366432827344421E-15, -12.48450537969573659, -132.4062500020483810 ) ) ;
#30023=CARTESIAN_POINT ( 'NONE',  ( -9.999999999999998224, 1.224646799147353059E-15, -105.1250000040967763 ) ) ;
#30025=CARTESIAN_POINT ( 'NONE',  ( 9.999999999999998224, 0.000000000000000000, -106.9999999999999858 ) ) ;
#30026=CARTESIAN_POINT ( 'NONE',  ( -10.81189881249999729, 6.242252689847871849, -68.21875000204838102 ) ) ;
#30027=VERTEX_POINT ( 'NONE', #16051 ) ;
#30031=CARTESIAN_POINT ( 'NONE',  ( -10.00000000000051337, 5.773502691895962435, -124.7500000040967620 ) ) ;
#30033=CARTESIAN_POINT ( 'NONE',  ( 5.000000000000000000, 8.660254037844385522, -39.62500000409676915 ) ) ;
#30037=CARTESIAN_POINT ( 'NONE',  ( 5.000000000000000000, 8.660254037844385522, -122.1250000040967905 ) ) ;
#30038=VERTEX_POINT ( 'NONE', #16257 ) ;
#30040=CARTESIAN_POINT ( 'NONE',  ( -4.999999999999996447, 8.660254037844387298, -126.3750000040967905 ) ) ;
#30041=CARTESIAN_POINT ( 'NONE',  ( 0.000000000000000000, 0.000000000000000000, -99.99999999999998579 ) ) ;
#30043=CARTESIAN_POINT ( 'NONE',  ( -10.81189881249999729, 1.324075727343319199E-15, -192.7812500020484094 ) ) ;
#30049=ADVANCED_FACE ( 'NONE', ( #115 ), #6570, .F. ) ;
#30051=CARTESIAN_POINT ( 'NONE',  ( -2.293366432827344421E-15, -12.48450537969573659, -123.2187500020483952 ) ) ;
#30052=CARTESIAN_POINT ( 'NONE',  ( -9.999999999999998224, 5.773502691896259087, -193.7500000040967905 ) ) ;
#30054=CARTESIAN_POINT ( 'NONE',  ( -10.81189881249999729, 1.324075727343319199E-15, -134.2812500020483810 ) ) ;
#30057=CARTESIAN_POINT ( 'NONE',  ( -10.81189881249999729, 1.324075727343319199E-15, -140.0937500020483810 ) ) ;
#30061=CARTESIAN_POINT ( 'NONE',  ( -9.999999999999998224, 5.773502691896259087, -152.8749999999999716 ) ) ;
#30066=CARTESIAN_POINT ( 'NONE',  ( -5.405949406250003975, -9.363379034771801557, -57.34375000204835970 ) ) ;
#30068=CARTESIAN_POINT ( 'NONE',  ( -2.293366432827344421E-15, -12.48450537969573659, -165.2187500020484094 ) ) ;
#30071=FACE_OUTER_BOUND ( 'NONE', #2107, .T. ) ;
#30072=CARTESIAN_POINT ( 'NONE',  ( 9.999999999999996447, -5.773502691896262640, -81.62499999999998579 ) ) ;
#30076=CARTESIAN_POINT ( 'NONE',  ( 5.405949406249999534, 9.363379034771803333, -113.7812500020483952 ) ) ;
#30077=CARTESIAN_POINT ( 'NONE',  ( -9.999999999999998224, 1.224646799147353059E-15, -129.1250000040967620 ) ) ;
#30082=CARTESIAN_POINT ( 'NONE',  ( 10.81189881249999907, 6.242252689847868297, -52.40625000204838102 ) ) ;
#30100=DIRECTION ( 'NONE',  ( -0.000000000000000000, -0.000000000000000000, -1.000000000000000000 ) ) ;
#30103=CARTESIAN_POINT ( 'NONE',  ( -2.293366432827344421E-15, -12.48450537969573659, -153.2187500020483810 ) ) ;
#30104=CARTESIAN_POINT ( 'NONE',  ( -10.81189881249999729, 6.242252689847871849, -161.2187500020483810 ) ) ;
#30106=FACE_OUTER_BOUND ( 'NONE', #26419, .T. ) ;
#30107=CARTESIAN_POINT ( 'NONE',  ( -5.000000000000003553, -8.660254037844383745, -181.0000000000000000 ) ) ;
#30111=CARTESIAN_POINT ( 'NONE',  ( 9.999999999999998224, 0.000000000000000000, -134.0000000000000000 ) ) ;
#30113=CARTESIAN_POINT ( 'NONE',  ( -2.293366432827344421E-15, -12.48450537969573659, -183.2187500020484094 ) ) ;
#30116=CARTESIAN_POINT ( 'NONE',  ( -2.293366432827344421E-15, -12.48450537969573659, -55.90625000204838102 ) ) ;
#30118=CARTESIAN_POINT ( 'NONE',  ( -2.121150477449813534E-15, -11.54700538379251284, -119.3749999999999858 ) ) ;
#30120=CARTESIAN_POINT ( 'NONE',  ( 10.81189881249999729, 0.000000000000000000, -138.0312500020484094 ) ) ;
#30121=CARTESIAN_POINT ( 'NONE',  ( -10.81189881249999907, -6.242252689847864744, -144.6562500020484094 ) ) ;
#30123=CARTESIAN_POINT ( 'NONE',  ( -9.999999999999998224, 0.000000000000000000, -99.99999999999998579 ) ) ;
#30124=CARTESIAN_POINT ( 'NONE',  ( -10.81189881249999729, 6.242252689847871849, -80.21875000204838102 ) ) ;
#30127=CARTESIAN_POINT ( 'NONE',  ( -10.81189881249999729, 1.324075727343319199E-15, -182.0937500020483810 ) ) ;
#30130=CYLINDRICAL_SURFACE ( 'NONE', #11782, 9.999999999999998224 ) ;
#30131=CARTESIAN_POINT ( 'NONE',  ( 5.405949406249999534, 9.363379034771803333, -73.28125000204838102 ) ) ;
#30133=CARTESIAN_POINT ( 'NONE',  ( -4.999999999999996447, 8.660254037844387298, -51.37500000409675494 ) ) ;
#30134=CARTESIAN_POINT ( 'NONE',  ( 10.81189881249999551, -6.242252689847874514, -13.46875000204836503 ) ) ;
#30137=CARTESIAN_POINT ( 'NONE',  ( -10.81189881249999729, 6.242252689847871849, -6.906250002048365033 ) ) ;
#30141=DIRECTION ( 'NONE',  ( -0.000000000000000000, -0.000000000000000000, -1.000000000000000000 ) ) ;
#30146=CARTESIAN_POINT ( 'NONE',  ( 10.81189881249999551, -6.242252689847874514, -101.9687500020483810 ) ) ;
#30155=CARTESIAN_POINT ( 'NONE',  ( 5.000000000000000000, 8.660254037844385522, -48.24999999999998579 ) ) ;
#30159=LINE ( 'NONE', #23251, #42583 ) ;
#30160=CARTESIAN_POINT ( 'NONE',  ( -10.81189881249999729, 1.324075727343319199E-15, -144.7812500020483810 ) ) ;
#30164=CARTESIAN_POINT ( 'NONE',  ( -10.00000000000051337, 5.773502691895962435, -140.8750000000000000 ) ) ;
#30169=CARTESIAN_POINT ( 'NONE',  ( -10.81189881249999729, 6.242252689847871849, -69.71875000204838102 ) ) ;
#30170=CARTESIAN_POINT ( 'NONE',  ( -2.293366432827344421E-15, -12.48450537969573659, -75.40625000204838102 ) ) ;
#30173=CARTESIAN_POINT ( 'NONE',  ( -10.81189881249999729, -6.242252689847864744, -156.6562500020484094 ) ) ;
#30174=CARTESIAN_POINT ( 'NONE',  ( -2.293366432827344421E-15, -12.48450537969573659, -171.4062500020484379 ) ) ;
#30176=CARTESIAN_POINT ( 'NONE',  ( 0.000000000000000000, 0.000000000000000000, -99.99999999999998579 ) ) ;
#30177=LINE ( 'NONE', #40279, #31658 ) ;
#30178=CARTESIAN_POINT ( 'NONE',  ( 10.81189881249999729, 0.000000000000000000, -104.8437500020483810 ) ) ;
#30180=CARTESIAN_POINT ( 'NONE',  ( 10.81189881249999907, 6.242252689847868297, -7.406250002048365033 ) ) ;
#30182=CARTESIAN_POINT ( 'NONE',  ( -10.00000000000000000, -5.773502691896252870, -169.1249999999999716 ) ) ;
#30184=CARTESIAN_POINT ( 'NONE',  ( -5.405949406250003975, -9.363379034771801557, -102.5312500020483952 ) ) ;
#30187=CARTESIAN_POINT ( 'NONE',  ( -9.999999999999998224, 1.224646799147353059E-15, -76.62500000409677625 ) ) ;
#30188=DIRECTION ( 'NONE',  ( -0.000000000000000000, -0.000000000000000000, -1.000000000000000000 ) ) ;
#30189=CARTESIAN_POINT ( 'NONE',  ( -10.81189881249999729, 1.324075727343319199E-15, -30.59375000204836326 ) ) ;
#30192=CARTESIAN_POINT ( 'NONE',  ( -2.293366432827344421E-15, -12.48450537969573659, -30.40625000204835615 ) ) ;
#30194=CARTESIAN_POINT ( 'NONE',  ( -4.999999999999996447, 8.660254037844387298, -139.5000000000000000 ) ) ;
#30195=CARTESIAN_POINT ( 'NONE',  ( 10.00000000000000000, 5.773502691896255534, -14.25000000409676382 ) ) ;
#30199=CARTESIAN_POINT ( 'NONE',  ( 9.999999999999479527, 5.773502691896553074, -123.3749999999999858 ) ) ;
#30201=EDGE_LOOP ( 'NONE', ( #21265, #14396, #33007, #16351 ) ) ;
#30203=ORIENTED_EDGE ( 'NONE', *, *, #25160, .F. ) ;
#30213=CARTESIAN_POINT ( 'NONE',  ( 5.405949406249999534, 9.363379034771803333, -169.2812500020484094 ) ) ;
#30216=CARTESIAN_POINT ( 'NONE',  ( 10.81189881249999551, -6.242252689847874514, -97.46875000204838102 ) ) ;
#30217=CARTESIAN_POINT ( 'NONE',  ( 9.999999999999998224, 0.000000000000000000, -113.3750000040967763 ) ) ;
#30218=CARTESIAN_POINT ( 'NONE',  ( -5.405949406249996869, 9.363379034771805109, -98.53125000204839523 ) ) ;
#30220=CARTESIAN_POINT ( 'NONE',  ( -2.293366432827344421E-15, -12.48450537969573659, -117.2187500020483668 ) ) ;
#30223=CARTESIAN_POINT ( 'NONE',  ( 10.81189881249999551, -6.242252689847874514, -178.6562500020484094 ) ) ;
#30224=CARTESIAN_POINT ( 'NONE',  ( 10.81189881249999729, 0.000000000000000000, -193.5312500020484094 ) ) ;
#30227=CARTESIAN_POINT ( 'NONE',  ( -5.000000000000003553, -8.660254037844383745, -175.3750000040967905 ) ) ;
#30229=CARTESIAN_POINT ( 'NONE',  ( 7.644554776091147741E-16, 12.48450537969573659, -21.96875000204837391 ) ) ;
#30230=CYLINDRICAL_SURFACE ( 'NONE', #26117, 9.999999999999998224 ) ;
#30231=CARTESIAN_POINT ( 'NONE',  ( -5.405949406250003975, -9.363379034771801557, -126.3437500020483952 ) ) ;
#30233=CARTESIAN_POINT ( 'NONE',  ( -10.81189881249999729, 6.242252689847871849, -24.90625000204838102 ) ) ;
#30236=CARTESIAN_POINT ( 'NONE',  ( 9.999999999999998224, 0.000000000000000000, -55.99999999999996447 ) ) ;
#30237=CARTESIAN_POINT ( 'NONE',  ( 5.405949406249999534, 9.363379034771803333, -124.2812500020483952 ) ) ;
#30241=CARTESIAN_POINT ( 'NONE',  ( 10.00000000000000000, 5.773502691896255534, -107.2500000040967763 ) ) ;
#30242=CARTESIAN_POINT ( 'NONE',  ( -5.000000000000003553, -8.660254037844383745, -107.4999999999999858 ) ) ;
#30243=CARTESIAN_POINT ( 'NONE',  ( 10.81189881249999907, 6.242252689847868297, -59.71875000204838102 ) ) ;
#30244=VERTEX_POINT ( 'NONE', #35729 ) ;
#30246=EDGE_CURVE ( 'NONE', #7470, #6263, #2920, .T. ) ;
#30249=CARTESIAN_POINT ( 'NONE',  ( -2.121150477449813534E-15, -11.54700538379251284, -38.75000000409676204 ) ) ;
#30254=ORIENTED_EDGE ( 'NONE', *, *, #2100, .F. ) ;
#30259=CARTESIAN_POINT ( 'NONE',  ( -10.81189881249999907, -6.242252689847864744, -198.6562500020484094 ) ) ;
#30265=CARTESIAN_POINT ( 'NONE',  ( 10.81189881249999729, 0.000000000000000000, -119.8437500020483810 ) ) ;
#30266=CARTESIAN_POINT ( 'NONE',  ( 9.999999999999996447, -5.773502691896262640, -194.5000000040968189 ) ) ;
#30267=CARTESIAN_POINT ( 'NONE',  ( 7.644554776091147741E-16, 12.48450537969573659, -122.6562500020483952 ) ) ;
#30269=CARTESIAN_POINT ( 'NONE',  ( 10.81189881249999729, 0.000000000000000000, -136.3437500020484094 ) ) ;
#30273=CARTESIAN_POINT ( 'NONE',  ( 7.070501591499377789E-16, 11.54700538379251284, -151.6250000000000000 ) ) ;
#30274=CARTESIAN_POINT ( 'NONE',  ( 10.00000000000000000, 5.773502691896255534, -22.87499999999997868 ) ) ;
#30279=CARTESIAN_POINT ( 'NONE',  ( 10.81189881249999551, -6.242252689847874514, -44.96875000204835970 ) ) ;
#30280=CARTESIAN_POINT ( 'NONE',  ( 9.999999999999998224, 0.000000000000000000, -141.5000000000000000 ) ) ;
#30281=CARTESIAN_POINT ( 'NONE',  ( 5.405949406249992428, -9.363379034771808662, -157.5937500020483810 ) ) ;
#30285=CARTESIAN_POINT ( 'NONE',  ( 5.000000000000000000, 8.660254037844385522, -84.24999999999997158 ) ) ;
#30287=ORIENTED_EDGE ( 'NONE', *, *, #2632, .T. ) ;
#30288=CARTESIAN_POINT ( 'NONE',  ( -2.293366432827344421E-15, -12.48450537969573659, -108.4062500020483810 ) ) ;
#30289=CARTESIAN_POINT ( 'NONE',  ( -4.999999999999996447, 8.660254037844387298, -133.8750000040967905 ) ) ;
#30291=ADVANCED_FACE ( 'NONE', ( #956 ), #24266, .F. ) ;
#30293=FACE_OUTER_BOUND ( 'NONE', #33527, .T. ) ;
#30294=CARTESIAN_POINT ( 'NONE',  ( -10.81189881249999907, -6.242252689847864744, -50.15625000204837391 ) ) ;
#30302=EDGE_CURVE ( 'NONE', #23494, #21425, #21357, .T. ) ;
#30308=ORIENTED_EDGE ( 'NONE', *, *, #15854, .F. ) ;
#30317=CARTESIAN_POINT ( 'NONE',  ( -10.81189881249999729, 6.242252689847871849, -144.7187500020483810 ) ) ;
#30318=CARTESIAN_POINT ( 'NONE',  ( 5.405949406249992428, -9.363379034771808662, -159.0937500020484094 ) ) ;
#30320=( BOUNDED_CURVE ( )  B_SPLINE_CURVE ( 2, ( #27125, #18847, #32027, #13929, #40267, #10704, #23900 ),
 .UNSPECIFIED., .F., .F. ) 
 B_SPLINE_CURVE_WITH_KNOTS ( ( 3, 2, 2, 3 ),
 ( 0.2761194029850747578, 0.2773631840796020875, 0.2786069651741294728, 0.2798507462686568026 ),
 .UNSPECIFIED. ) 
 CURVE ( )  GEOMETRIC_REPRESENTATION_ITEM ( )  RATIONAL_B_SPLINE_CURVE ( ( 0.9999999999999880096, 0.8660254037844506980, 1.000000000000000000, 0.8660254037844387076, 1.000000000000000000, 0.8660254037844267172, 1.000000000000011990 ) ) 
 REPRESENTATION_ITEM ( '' )  );
#30321=CARTESIAN_POINT ( 'NONE',  ( -4.999999999999996447, 8.660254037844387298, -102.3750000040967905 ) ) ;
#30322=CARTESIAN_POINT ( 'NONE',  ( 5.000000000000000000, 8.660254037844385522, -183.2500000000000000 ) ) ;
#30323=VECTOR ( 'NONE', #16242, 1000.000000000000000 ) ;
#30328=CARTESIAN_POINT ( 'NONE',  ( -4.999999999999996447, 8.660254037844387298, -168.3750000040967905 ) ) ;
#30329=CARTESIAN_POINT ( 'NONE',  ( 5.405949406249992428, -9.363379034771808662, -184.5937500020483810 ) ) ;
#30332=CARTESIAN_POINT ( 'NONE',  ( 10.81189881249999551, -6.242252689847874514, -52.65625000204837391 ) ) ;
#30334=CARTESIAN_POINT ( 'NONE',  ( 5.000000000000000000, 8.660254037844385522, -109.7499999999999858 ) ) ;
#30337=CARTESIAN_POINT ( 'NONE',  ( 5.405949406249992428, -9.363379034771808662, -132.2812500020483810 ) ) ;
#30338=CARTESIAN_POINT ( 'NONE',  ( -10.81189881249999907, -6.242252689847864744, -147.6562500020483810 ) ) ;
#30340=CARTESIAN_POINT ( 'NONE',  ( -5.405949406250003975, -9.363379034771801557, -78.34375000204838102 ) ) ;
#30343=CARTESIAN_POINT ( 'NONE',  ( 5.405949406249999534, 9.363379034771803333, -178.0937500020484094 ) ) ;
#30345=CARTESIAN_POINT ( 'NONE',  ( 10.00000000000051159, -5.773502691895965988, -110.1249999999999858 ) ) ;
#30347=CARTESIAN_POINT ( 'NONE',  ( 10.81189881249999907, 6.242252689847868297, -79.40625000204839523 ) ) ;
#30349=CARTESIAN_POINT ( 'NONE',  ( 9.999999999999998224, 0.000000000000000000, -54.87500000409675494 ) ) ;
#30350=CARTESIAN_POINT ( 'NONE',  ( -2.293366432827344421E-15, -12.48450537969573659, -13.71875000204836326 ) ) ;
#30353=CARTESIAN_POINT ( 'NONE',  ( 5.405949406249992428, -9.363379034771808662, -4.781250002048375691 ) ) ;
#30355=CARTESIAN_POINT ( 'NONE',  ( 9.999999999999998224, 0.000000000000000000, -161.0000000000000000 ) ) ;
#30356=CARTESIAN_POINT ( 'NONE',  ( 7.070501591499376803E-16, 11.54700538379251284, -177.5000000040967905 ) ) ;
#30363=CARTESIAN_POINT ( 'NONE',  ( 10.81189881249999729, 6.242252689847867408, -100.2187500020483810 ) ) ;
#30371=CARTESIAN_POINT ( 'NONE',  ( 10.00000000000000000, 5.773502691896255534, -46.87499999999997158 ) ) ;
#30382=CARTESIAN_POINT ( 'NONE',  ( -10.81189881249999729, 1.324075727343319199E-15, -66.59375000204836681 ) ) ;
#30383=CARTESIAN_POINT ( 'NONE',  ( 5.405949406249992428, -9.363379034771808662, -78.28125000204838102 ) ) ;
#30385=CARTESIAN_POINT ( 'NONE',  ( -2.293366432827344421E-15, -12.48450537969573659, -154.9062500020483810 ) ) ;
#30386=CARTESIAN_POINT ( 'NONE',  ( -10.81189881249999729, 6.242252689847871849, -173.4062500020483810 ) ) ;
#30388=CYLINDRICAL_SURFACE ( 'NONE', #15085, 9.999999999999998224 ) ;
#30390=CARTESIAN_POINT ( 'NONE',  ( -2.293366432827344421E-15, -12.48450537969573659, -106.7187500020483668 ) ) ;
#30393=CARTESIAN_POINT ( 'NONE',  ( 7.644554776091147741E-16, 12.48450537969573659, -7.156250002048364145 ) ) ;
#30397=CARTESIAN_POINT ( 'NONE',  ( -10.81189881249999907, -6.242252689847864744, -101.1562500020483952 ) ) ;
#30399=CARTESIAN_POINT ( 'NONE',  ( 4.999999999999992006, -8.660254037844389075, -77.62500000409677625 ) ) ;
#30401=CARTESIAN_POINT ( 'NONE',  ( -5.405949406249996869, 9.363379034771805109, -33.84375000204836681 ) ) ;
#30404=CARTESIAN_POINT ( 'NONE',  ( -5.405949406250003975, -9.363379034771801557, -30.53125000204837036 ) ) ;
#30407=( BOUNDED_CURVE ( )  B_SPLINE_CURVE ( 2, ( #13928, #27337, #10703, #37045, #10919, #17387, #24113 ),
 .UNSPECIFIED., .F., .F. ) 
 B_SPLINE_CURVE_WITH_KNOTS ( ( 3, 2, 2, 3 ),
 ( 0.2611940298507463565, 0.2624378109452737418, 0.2636815920398011270, 0.2649253731343284568 ),
 .UNSPECIFIED. ) 
 CURVE ( )  GEOMETRIC_REPRESENTATION_ITEM ( )  RATIONAL_B_SPLINE_CURVE ( ( 0.9999999999999880096, 0.8660254037844506980, 1.000000000000000000, 0.8660254037844387076, 1.000000000000000000, 0.8660254037844267172, 1.000000000000011990 ) ) 
 REPRESENTATION_ITEM ( '' )  );
#30408=CARTESIAN_POINT ( 'NONE',  ( 9.999999999999996447, -5.773502691896262640, -2.500000004096753159 ) ) ;
#30413=ORIENTED_EDGE ( 'NONE', *, *, #31759, .T. ) ;
#30416=VERTEX_POINT ( 'NONE', #41913 ) ;
#30427=CARTESIAN_POINT ( 'NONE',  ( -10.81189881249999729, 6.242252689847871849, -170.4062500020484094 ) ) ;
#30429=EDGE_CURVE ( 'NONE', #37069, #12598, #28570, .T. ) ;
#30431=CARTESIAN_POINT ( 'NONE',  ( -5.405949406250003975, -9.363379034771801557, -96.34375000204838102 ) ) ;
#30433=CARTESIAN_POINT ( 'NONE',  ( -2.293366432827344421E-15, -12.48450537969573659, -100.9062500020483952 ) ) ;
#30435=CARTESIAN_POINT ( 'NONE',  ( -2.293366432827344421E-15, -12.48450537969573659, -103.7187500020483668 ) ) ;
#30438=CARTESIAN_POINT ( 'NONE',  ( -10.81189881249999907, -6.242252689847864744, -192.6562500020484094 ) ) ;
#30441=CARTESIAN_POINT ( 'NONE',  ( 9.999999999999996447, -5.773502691896262640, -170.5000000040967905 ) ) ;
#30443=CARTESIAN_POINT ( 'NONE',  ( 10.81189881249999907, 6.242252689847868297, -25.21875000204837747 ) ) ;
#30445=CARTESIAN_POINT ( 'NONE',  ( 5.405949406249992428, -9.363379034771808662, -129.0937500020483810 ) ) ;
#30447=CARTESIAN_POINT ( 'NONE',  ( 10.81189881249999907, 6.242252689847868297, -28.40625000204838457 ) ) ;
#30448=EDGE_CURVE ( 'NONE', #4764, #25488, #2597, .T. ) ;
#30450=CARTESIAN_POINT ( 'NONE',  ( 9.999999999999996447, -5.773502691896262640, -56.12499999999997868 ) ) ;
#30451=CARTESIAN_POINT ( 'NONE',  ( 5.405949406249992428, -9.363379034771808662, -124.7812500020483952 ) ) ;
#30457=CARTESIAN_POINT ( 'NONE',  ( 10.00000000000000000, 5.773502691896255534, -98.25000000409677625 ) ) ;
#30459=CARTESIAN_POINT ( 'NONE',  ( -10.81189881249999729, 6.242252689847871849, -57.71875000204837391 ) ) ;
#30465=CARTESIAN_POINT ( 'NONE',  ( -2.121150477449813534E-15, -11.54700538379251284, -26.75000000409677270 ) ) ;
#30473=ORIENTED_EDGE ( 'NONE', *, *, #28025, .T. ) ;
#30477=DIRECTION ( 'NONE',  ( -1.000000000000000000, 0.000000000000000000, 0.000000000000000000 ) ) ;
#30483=CARTESIAN_POINT ( 'NONE',  ( 7.644554776091147741E-16, 12.48450537969573659, -116.4687500020483952 ) ) ;
#30484=CARTESIAN_POINT ( 'NONE',  ( 4.999999999999992006, -8.660254037844389075, -197.6250000040967905 ) ) ;
#30485=CARTESIAN_POINT ( 'NONE',  ( -10.81189881249999729, 6.242252689847871849, -123.9062500020483952 ) ) ;
#30487=CARTESIAN_POINT ( 'NONE',  ( 10.81189881249999729, 0.000000000000000000, -130.3437500020484094 ) ) ;
#30491=CARTESIAN_POINT ( 'NONE',  ( 7.070501591499377789E-16, 11.54700538379251284, -153.1250000000000000 ) ) ;
#30492=CARTESIAN_POINT ( 'NONE',  ( 9.999999999999996447, -5.773502691896262640, -24.62499999999998224 ) ) ;
#30496=CARTESIAN_POINT ( 'NONE',  ( 9.999999999999998224, 1.224646799147353059E-15, -99.99999999999998579 ) ) ;
#30498=CARTESIAN_POINT ( 'NONE',  ( 10.81189881249999729, 0.000000000000000000, -46.34375000204838102 ) ) ;
#30499=CARTESIAN_POINT ( 'NONE',  ( 10.00000000000051159, -5.773502691895965988, -141.6250000000000000 ) ) ;
#30500=CARTESIAN_POINT ( 'NONE',  ( 10.81189881249999729, 0.000000000000000000, -152.8437500020483810 ) ) ;
#30503=CARTESIAN_POINT ( 'NONE',  ( 2.746439794587930194, 9.968836831075687854, -180.0000000000001421 ) ) ;
#30504=CARTESIAN_POINT ( 'NONE',  ( -4.999999999999996447, 8.660254037844387298, -86.99999999999998579 ) ) ;
#30507=CARTESIAN_POINT ( 'NONE',  ( -5.405949406249996869, 9.363379034771805109, -112.0312500020483810 ) ) ;
#30508=CARTESIAN_POINT ( 'NONE',  ( -2.121150477449813534E-15, -11.54700538379251284, -124.2500000040967763 ) ) ;
#30509=DIRECTION ( 'NONE',  ( 0.000000000000000000, 0.000000000000000000, -1.000000000000000000 ) ) ;
#30511=CYLINDRICAL_SURFACE ( 'NONE', #31812, 9.999999999999998224 ) ;
#30512=CARTESIAN_POINT ( 'NONE',  ( 7.644554776091147741E-16, 12.48450537969573659, -52.15625000204838102 ) ) ;
#30521=ORIENTED_EDGE ( 'NONE', *, *, #31252, .F. ) ;
#30525=CARTESIAN_POINT ( 'NONE',  ( 9.999999999999998224, 0.000000000000000000, -103.9999999999999858 ) ) ;
#30534=CARTESIAN_POINT ( 'NONE',  ( 10.81189881249999729, 0.000000000000000000, -143.8437500020483810 ) ) ;
#30535=CARTESIAN_POINT ( 'NONE',  ( -10.81189881249999729, 6.242252689847871849, -164.2187500020483810 ) ) ;
#30538=CARTESIAN_POINT ( 'NONE',  ( -2.121150477449813534E-15, -11.54700538379251284, -176.3750000000000000 ) ) ;
#30540=CARTESIAN_POINT ( 'NONE',  ( -4.999999999999996447, 8.660254037844387298, -151.5000000000000000 ) ) ;
#30542=CARTESIAN_POINT ( 'NONE',  ( -10.81189881249999729, 1.324075727343319199E-15, -174.5937500020484094 ) ) ;
#30545=CARTESIAN_POINT ( 'NONE',  ( 10.81189881249999551, -6.242252689847874514, -49.65625000204837391 ) ) ;
#30547=CARTESIAN_POINT ( 'NONE',  ( 4.999999999999992006, -8.660254037844389075, -110.2499999999999858 ) ) ;
#30550=CARTESIAN_POINT ( 'NONE',  ( 5.405949406249992428, -9.363379034771808662, -135.2812500020483810 ) ) ;
#30551=CARTESIAN_POINT ( 'NONE',  ( -4.999999999999996447, 8.660254037844387298, -157.8750000040967905 ) ) ;
#30552=CARTESIAN_POINT ( 'NONE',  ( 10.81189881249999551, -6.242252689847874514, -150.1562500020484094 ) ) ;
#30554=CARTESIAN_POINT ( 'NONE',  ( 10.81189881249999551, -6.242252689847874514, -82.46875000204836681 ) ) ;
#30557=CARTESIAN_POINT ( 'NONE',  ( 10.81189881249999729, 0.000000000000000000, -179.8437500020483810 ) ) ;
#30559=CARTESIAN_POINT ( 'NONE',  ( -10.81189881249999729, 1.324075727343319199E-15, -75.78125000204838102 ) ) ;
#30561=CARTESIAN_POINT ( 'NONE',  ( 7.070501591499377789E-16, 11.54700538379251284, -51.50000000409676915 ) ) ;
#30562=CARTESIAN_POINT ( 'NONE',  ( 5.405949406249992428, -9.363379034771808662, -10.59375000204834727 ) ) ;
#30565=CARTESIAN_POINT ( 'NONE',  ( 5.405949406249992428, -9.363379034771808662, -1.781250002048373471 ) ) ;
#30569=( BOUNDED_CURVE ( )  B_SPLINE_CURVE ( 2, ( #36391, #16298, #39614, #20613, #20195, #23663, #366 ),
 .UNSPECIFIED., .F., .F. ) 
 B_SPLINE_CURVE_WITH_KNOTS ( ( 3, 2, 2, 3 ),
 ( 0.2500000000000001110, 0.2512437810945274963, 0.2524875621890548261, 0.2537313432835822113 ),
 .UNSPECIFIED. ) 
 CURVE ( )  GEOMETRIC_REPRESENTATION_ITEM ( )  RATIONAL_B_SPLINE_CURVE ( ( 0.9999999999999880096, 0.8660254037844506980, 1.000000000000000000, 0.8660254037844387076, 1.000000000000000000, 0.8660254037844267172, 1.000000000000011990 ) ) 
 REPRESENTATION_ITEM ( '' )  );
#30580=CARTESIAN_POINT ( 'NONE',  ( 10.00000000000025402, -5.773502691896113426, -122.1250000000000000 ) ) ;
#30581=CARTESIAN_POINT ( 'NONE',  ( 4.999999999999992006, -8.660254037844389075, -47.24999999999998579 ) ) ;
#30583=CARTESIAN_POINT ( 'NONE',  ( 5.405949406249992428, -9.363379034771808662, -163.5937500020484094 ) ) ;
#30587=CARTESIAN_POINT ( 'NONE',  ( 35.00000000000000711, 4.286263797015737285E-15, -176.9999999999999432 ) ) ;
#30593=CARTESIAN_POINT ( 'NONE',  ( -10.81189881249999729, 1.324075727343319199E-15, -69.59375000204836681 ) ) ;
#30594=CARTESIAN_POINT ( 'NONE',  ( -2.293366432827344421E-15, -12.48450537969573659, -76.90625000204839523 ) ) ;
#30596=CARTESIAN_POINT ( 'NONE',  ( 10.00000000000000000, 5.773502691896255534, -129.3750000000000000 ) ) ;
#30597=CARTESIAN_POINT ( 'NONE',  ( 5.405949406249999534, 9.363379034771803333, -157.2812500020484094 ) ) ;
#30598=CARTESIAN_POINT ( 'NONE',  ( 10.81189881249999729, 0.000000000000000000, -175.5312500020483810 ) ) ;
#30599=CARTESIAN_POINT ( 'NONE',  ( 10.81189881249999729, 0.000000000000000000, 0.1562499979516351889 ) ) ;
#30601=CARTESIAN_POINT ( 'NONE',  ( 10.81189881249999729, 0.000000000000000000, -106.3437500020483810 ) ) ;
#30604=CARTESIAN_POINT ( 'NONE',  ( -5.405949406250003975, -9.363379034771801557, -8.031250002048350822 ) ) ;
#30606=CARTESIAN_POINT ( 'NONE',  ( 4.999999999999992006, -8.660254037844389075, -168.7500000000000000 ) ) ;
#30607=CARTESIAN_POINT ( 'NONE',  ( -5.405949406249996869, 9.363379034771805109, -101.5312500020483952 ) ) ;
#30609=CARTESIAN_POINT ( 'NONE',  ( 10.00000000000000000, 5.773502691896255534, -72.75000000409674783 ) ) ;
#30611=CARTESIAN_POINT ( 'NONE',  ( 7.644554776091147741E-16, 12.48450537969573659, -33.96875000204835260 ) ) ;
#30612=ORIENTED_EDGE ( 'NONE', *, *, #34237, .F. ) ;
#30614=CARTESIAN_POINT ( 'NONE',  ( -10.81189881249999729, 1.324075727343319199E-15, -32.28125000204837391 ) ) ;
#30617=CARTESIAN_POINT ( 'NONE',  ( 4.999999999999992006, -8.660254037844389075, -1.125000004096765593 ) ) ;
#30622=ORIENTED_EDGE ( 'NONE', *, *, #33066, .F. ) ;
#30624=ORIENTED_EDGE ( 'NONE', *, *, #21185, .T. ) ;
#30630=CARTESIAN_POINT ( 'NONE',  ( 10.00000000000025402, -5.773502691896113426, -128.5000000040967905 ) ) ;
#30632=CARTESIAN_POINT ( 'NONE',  ( -10.81189881249999907, -6.242252689847864744, -174.6562500020483810 ) ) ;
#30635=CARTESIAN_POINT ( 'NONE',  ( 10.81189881249999907, 6.242252689847868297, -95.71875000204838102 ) ) ;
#30636=CARTESIAN_POINT ( 'NONE',  ( 7.070501591499376803E-16, 11.54700538379251284, -113.0000000040967763 ) ) ;
#30637=CARTESIAN_POINT ( 'NONE',  ( 5.405949406249992428, -9.363379034771808662, -99.28125000204839523 ) ) ;
#30639=CARTESIAN_POINT ( 'NONE',  ( 10.81189881249999729, 0.000000000000000000, -107.8437500020483810 ) ) ;
#30642=CARTESIAN_POINT ( 'NONE',  ( 4.999999999999992006, -8.660254037844389075, -152.6250000040967905 ) ) ;
#30643=CARTESIAN_POINT ( 'NONE',  ( 7.070501591499377789E-16, 11.54700538379251284, -0.1249999999999584777 ) ) ;
#30646=CARTESIAN_POINT ( 'NONE',  ( -9.999999999999998224, 5.773502691896259087, -168.2500000040967905 ) ) ;
#30648=CARTESIAN_POINT ( 'NONE',  ( 10.81189881249999729, 0.000000000000000000, -23.84375000204835970 ) ) ;
#30650=CARTESIAN_POINT ( 'NONE',  ( 7.644554776091147741E-16, 12.48450537969573659, -128.4687500020483810 ) ) ;
#30651=EDGE_CURVE ( 'NONE', #34879, #42377, #40875, .T. ) ;
#30653=CARTESIAN_POINT ( 'NONE',  ( 7.644554776091147741E-16, 12.48450537969573659, -26.65625000204838102 ) ) ;
#30655=( BOUNDED_CURVE ( )  B_SPLINE_CURVE ( 2, ( #13871, #23832, #7635 ),
 .UNSPECIFIED., .F., .F. ) 
 B_SPLINE_CURVE_WITH_KNOTS ( ( 3, 3 ),
 ( 0.09950248756218914303, 0.1007462686567163757 ),
 .UNSPECIFIED. ) 
 CURVE ( )  GEOMETRIC_REPRESENTATION_ITEM ( )  RATIONAL_B_SPLINE_CURVE ( ( 0.9999999999999910072, 0.8660254037844521413, 0.9999999999999955591 ) ) 
 REPRESENTATION_ITEM ( '' )  );
#30656=CARTESIAN_POINT ( 'NONE',  ( 5.000000000000000000, 8.660254037844385522, -158.1250000040967905 ) ) ;
#30657=EDGE_CURVE ( 'NONE', #29774, #23180, #2870, .T. ) ;
#30658=CARTESIAN_POINT ( 'NONE',  ( 9.999999999999998224, 0.000000000000000000, -61.99999999999997158 ) ) ;
#30659=CARTESIAN_POINT ( 'NONE',  ( -2.293366432827344421E-15, -12.48450537969573659, -123.4062500020484094 ) ) ;
#30663=CARTESIAN_POINT ( 'NONE',  ( 4.999999999999992006, -8.660254037844389075, -98.62500000409677625 ) ) ;
#30664=CARTESIAN_POINT ( 'NONE',  ( -2.121150477449813534E-15, -11.54700538379251284, -151.2500000040968189 ) ) ;
#30665=CARTESIAN_POINT ( 'NONE',  ( -10.81189881249999729, 6.242252689847871849, -60.71875000204838102 ) ) ;
#30671=CARTESIAN_POINT ( 'NONE',  ( -9.999999999999998224, 1.224646799147353059E-15, -31.62500000409676559 ) ) ;
#30677=LINE ( 'NONE', #31110, #38305 ) ;
#30681=CARTESIAN_POINT ( 'NONE',  ( 10.81189881249999551, -6.242252689847874514, -193.6562500020484379 ) ) ;
#30683=CARTESIAN_POINT ( 'NONE',  ( 7.070501591499376803E-16, 11.54700538379251284, -150.1250000000000000 ) ) ;
#30687=CARTESIAN_POINT ( 'NONE',  ( 10.81189881249999551, -6.242252689847874514, -119.9687500020483952 ) ) ;
#30688=CARTESIAN_POINT ( 'NONE',  ( -4.999999999999996447, 8.660254037844387298, -196.8750000040967905 ) ) ;
#30689=CARTESIAN_POINT ( 'NONE',  ( 10.81189881249999729, 0.000000000000000000, -124.5312500020483952 ) ) ;
#30691=CARTESIAN_POINT ( 'NONE',  ( -10.81189881249999729, 6.242252689847871849, -129.7187500020483810 ) ) ;
#30694=CARTESIAN_POINT ( 'NONE',  ( 9.999999999999612754, 5.773502691896477579, -179.2500000040967905 ) ) ;
#30695=CARTESIAN_POINT ( 'NONE',  ( -5.000000000000003553, -8.660254037844383745, -158.5000000000000000 ) ) ;
#30696=CARTESIAN_POINT ( 'NONE',  ( -4.999999999999996447, 8.660254037844387298, -22.49999999999996447 ) ) ;
#30701=CARTESIAN_POINT ( 'NONE',  ( -5.405949406249996869, 9.363379034771805109, -44.34375000204837391 ) ) ;
#30703=CARTESIAN_POINT ( 'NONE',  ( 7.644554776091147741E-16, 12.48450537969573659, -150.9687500020483810 ) ) ;
#30707=CARTESIAN_POINT ( 'NONE',  ( -4.999999999999996447, 8.660254037844387298, -180.0000000000000000 ) ) ;
#30708=AXIS2_PLACEMENT_3D ( 'NONE', #31606, #11292, #40635 ) ;
#30709=CARTESIAN_POINT ( 'NONE',  ( -9.999999999999998224, 1.224646799147353059E-15, -85.24999999999997158 ) ) ;
#30714=CARTESIAN_POINT ( 'NONE',  ( -9.999999999999872102, -5.773502691896326589, -164.6249999999999716 ) ) ;
#30715=CARTESIAN_POINT ( 'NONE',  ( 4.999999999999992006, -8.660254037844389075, -121.1250000040967905 ) ) ;
#30721=CARTESIAN_POINT ( 'NONE',  ( -10.81189881249999907, -6.242252689847864744, -53.15625000204837391 ) ) ;
#30725=CARTESIAN_POINT ( 'NONE',  ( -9.999999999999998224, 1.224646799147353059E-15, -165.1250000040967905 ) ) ;
#30727=DIRECTION ( 'NONE',  ( -0.000000000000000000, -0.000000000000000000, -1.000000000000000000 ) ) ;
#30728=VERTEX_POINT ( 'NONE', #42547 ) ;
#30741=CARTESIAN_POINT ( 'NONE',  ( -5.405949406250003975, -9.363379034771801557, -138.3437500020484094 ) ) ;
#30742=CARTESIAN_POINT ( 'NONE',  ( -5.405949406250003975, -9.363379034771801557, -156.3437500020483810 ) ) ;
#30745=CARTESIAN_POINT ( 'NONE',  ( -2.121150477449813534E-15, -11.54700538379251284, -180.8750000000000000 ) ) ;
#30747=CARTESIAN_POINT ( 'NONE',  ( -2.170677449821584837, 10.59771640374526314, -100.0000000000000000 ) ) ;
#30749=CARTESIAN_POINT ( 'NONE',  ( -10.81189881249999907, -6.242252689847864744, -174.4687500020484094 ) ) ;
#30753=CARTESIAN_POINT ( 'NONE',  ( -5.405949406250003975, -9.363379034771801557, -42.53125000204838102 ) ) ;
#30755=CARTESIAN_POINT ( 'NONE',  ( 5.000000000000000000, 8.660254037844385522, -103.7500000000000000 ) ) ;
#30757=CARTESIAN_POINT ( 'NONE',  ( 7.644554776091147741E-16, 12.48450537969573659, -134.6562500020483810 ) ) ;
#30758=CARTESIAN_POINT ( 'NONE',  ( 4.999999999999992006, -8.660254037844389075, -149.6250000040967905 ) ) ;
#30759=CARTESIAN_POINT ( 'NONE',  ( -10.81189881249999729, 1.324075727343319199E-15, -146.2812500020483810 ) ) ;
#30761=VERTEX_POINT ( 'NONE', #33070 ) ;
#30763=CARTESIAN_POINT ( 'NONE',  ( -5.405949406249996869, 9.363379034771805109, -179.3437500020483810 ) ) ;
#30766=DIRECTION ( 'NONE',  ( -0.000000000000000000, -0.000000000000000000, -1.000000000000000000 ) ) ;
#30767=CARTESIAN_POINT ( 'NONE',  ( -5.405949406250003975, -9.363379034771801557, -74.03125000204838102 ) ) ;
#30770=CARTESIAN_POINT ( 'NONE',  ( 9.999999999999998224, 0.000000000000000000, -48.87500000409678336 ) ) ;
#30771=CARTESIAN_POINT ( 'NONE',  ( -10.81189881249999907, -6.242252689847864744, -12.46875000204836326 ) ) ;
#30772=DIRECTION ( 'NONE',  ( -0.000000000000000000, -0.000000000000000000, -1.000000000000000000 ) ) ;
#30774=EDGE_CURVE ( 'NONE', #40153, #32646, #22718, .T. ) ;
#30775=CARTESIAN_POINT ( 'NONE',  ( 10.81189881249999907, 6.242252689847868297, -2.906250002048360592 ) ) ;
#30778=DIRECTION ( 'NONE',  ( -1.000000000000000000, 0.000000000000000000, 0.000000000000000000 ) ) ;
#30782=( NAMED_UNIT ( * ) PLANE_ANGLE_UNIT ( ) SI_UNIT ( $, .RADIAN. ) );
#30783=DIRECTION ( 'NONE',  ( -1.000000000000000000, 0.000000000000000000, 0.000000000000000000 ) ) ;
#30785=ORIENTED_EDGE ( 'NONE', *, *, #34658, .F. ) ;
#30791=CARTESIAN_POINT ( 'NONE',  ( -4.999999999999996447, 8.660254037844387298, -41.99999999999997868 ) ) ;
#30793=CARTESIAN_POINT ( 'NONE',  ( -10.81189881249999729, 6.242252689847871849, -162.7187500020483810 ) ) ;
#30801=CARTESIAN_POINT ( 'NONE',  ( 5.405949406249992428, -9.363379034771808662, -69.09375000204836681 ) ) ;
#30802=CARTESIAN_POINT ( 'NONE',  ( 10.81189881249999551, -6.242252689847874514, -76.65625000204838102 ) ) ;
#30804=CARTESIAN_POINT ( 'NONE',  ( -2.121150477449813534E-15, -11.54700538379251284, -129.8750000000000000 ) ) ;
#30805=CARTESIAN_POINT ( 'NONE',  ( 10.81189881249999729, 6.242252689847867408, -161.9062500020483810 ) ) ;
#30806=CARTESIAN_POINT ( 'NONE',  ( 10.81189881249999729, 0.000000000000000000, -174.0312500020484094 ) ) ;
#30809=CARTESIAN_POINT ( 'NONE',  ( 10.81189881249999907, 6.242252689847868297, -109.2187500020483810 ) ) ;
#30810=CARTESIAN_POINT ( 'NONE',  ( -10.00000000000038547, 5.773502691896036154, -155.8749999999999432 ) ) ;
#30812=CARTESIAN_POINT ( 'NONE',  ( -10.81189881249999729, 6.242252689847871849, -0.9062500020483588159 ) ) ;
#30815=CARTESIAN_POINT ( 'NONE',  ( -5.405949406249996869, 9.363379034771805109, -97.03125000204839523 ) ) ;
#30817=( BOUNDED_SURFACE ( )  B_SPLINE_SURFACE ( 1, 2, ( 
 ( #14237, #7155, #10379, #36714, #4557, #14460, #40157, #30259, #20307, #24431, #906, #1111, #698, #4131, #10586, #34138, #27010, #13817, #23775, #33923, #10802, #37362, #20953, #21163, #37135, #7372, #20518, #490, #3716, #7805, #33706, #17272, #14021, #17697, #27214, #40361, #33500, #1328, #3924, #17488, #30891, #23993, #7583, #20736, #26797, #4347, #27650, #30681, #27438, #40575, #40791, #37574, #8019, #16845, #30043, #13603, #17917, #18358, #41654, #8871, #12091, #22033, #15325, #31333, #28733, #2192, #41860, #38217, #27867, #38644, #25072, #41001, #11657, #9078, #14893, #21603, #35205, #5635, #14680, #38007, #25284, #24856, #15530, #15104, #8452, #1764, #12297, #18784, #24645, #31972, #34782, #8662, #4768, #38429, #4996, #37788, #28091, #5203, #5424, #31763, #31547, #1547, #41218, #1980, #34996, #2400, #25494, #34350, #11445, #28301, #41438, #11876, #31114, #8232, #21815, #21382, #34565, #18137, #18576, #28523, #28940, #2817, #42285, #19414, #33017, #25702, #26539, #12707, #15949, #6054, #25905, #19621, #42077, #226, #3028, #39267, #8, #32182, #19205, #26328, #9702, #32393, #22881, #3446, #36040, #29146, #39056, #29563, #36250, #13132, #19833, #6680, #39479, #35834, #15740, #12508, #38852, #22450, #9495, #2610, #9279, #39688, #5841, #3238, #9912, #23088, #16364, #32806, #16583, #26113, #29785, #22662, #6476, #13348, #22245, #18998, #32604, #6268, #29352, #16155, #35416, #35628, #42491, #12918, #17647, #6893, #14187, #20264, #858, #33661, #33241, #33452, #27386, #27170, #13975, #4086, #13768, #30842, #33872, #30632, #23945, #29995, #36458, #36879, #17436, #20686, #3667, #34082, #20046, #20898, #39900, #37307, #40313, #3880, #1279, #4504, #16796, #26748, #13558, #26955, #10331, #17224, #20474, #7323, #441, #10754, #17015, #14407, #27601, #37090, #10124, #23302, #7533, #30427, #4297, #40110, #23520, #1063, #36668, #7110, #40522, #10966, #30213, #650, #24162, #10542, #23728, #7753, #14839, #31494, #14630, #4939, #41604, #31282, #4717, #34517, #8181, #28036, #1712, #37954, #28473, #2139, #5154, #27818, #8610, #34732, #41164, #38164, #12037, #18088, #15479, #11603, #31924, #24590, #21764, #1495, #17866, #31060, #25232, #8817, #24811, #11395, #34300, #5578, #8401, #34942, #37738, #21551, #18305, #38378, #21329, #1926, #15053, #28250, #41386, #5367, #15274, #40742, #11822, #25023, #18520, #37522, #11184, #31709, #21974, #35153, #18731, #2352, #24381, #7965, #40951, #21113, #28892, #42448, #42659, #42237, #2770, #19366, #2563, #35578, #29517, #19155, #35367, #22401, #38805, #15895, #32346, #25857, #16318, #32755, #35789, #15693, #39221, #22615, #29100, #26070, #13083, #6007, #3400, #12662, #19784, #12455, #9658, #32133, #5794, #18947, #26281, #39433, #39012, #42025, #22193, #36197, #9449, #22831, #25648, #6221, #32552, #9866, #9232, #2982, #16106, #29302, #12875, #35994, #3192, #28682, #6428, #19572, #23039, #25441, #41811, #6634, #32971, #12249, #38587, #9027, #16965, #7064, #10076, #14732, #16747, #30953, #31173, #26698, #7860, #40062, #39634, #39849, #34407, #34198, #21009, #10494, #20215, #37847, #40847, #37633, #1385, #36411, #178, #601, #24481, #27709, #23252, #41055, #13300, #27924, #3620, #1602, #4615, #10283, #8289, #11498, #6845, #33189, #19998, #33403, #29949, #23682, #26906, #13716, #26489, #17758, #23470, #24701, #34620, #14515, #16535, #29733, #11286, #37418, #8072, #3829, #390, #21222, #13508, #36617, #4827, #17973, #30160, #21436, #35474, #31599, #25757, #19054, #35048, #34835, #15796, #32236, #24913, #22509, #11716, #28360, #25123, #2256, #28992, #8500, #9341, #38269, #41497, #2032, #8715, #2454, #38059, #38910, #28575, #22087, #25548, #14945, #15161, #9132, #35262, #11931, #5696, #42131, #18846, #21869, #5475, #12350, #2662, #38698, #12563, #5047, #22302, #18625, #41278, #21653, #5258, #18410, #31821, #28145, #15375, #18192, #31384, #28787, #5900, #1819, #41918, #15586, #41705, #8925, #12143, #25336, #32026, #38481, #26593, #19258, #32865, #6528, #65, #29622, #35683, #19892, #19470, #33298, #499, #32449, #39743, #10178, #13401, #23363, #16640, #32655, #30054, #3502, #13614, #39535, #29200, #39957, #26383, #42340, #12976, #10388, #16211, #22940, #36515, #6952, #16005, #39319, #20108, #26173, #16853, #16424, #9759, #3083, #26806, #3723, #25964, #6111, #36093, #9965, #2875, #12771, #6325, #39113, #29412, #19679, #6738, #33075, #3297, #9549, #42552, #13190, #36307, #22723, #35888, #23144, #29842, #280, #20526, #20744, #1555, #40799, #40584, #27448, #4355, #27225, #14687, #4565, #1337, #37370, #706, #7163, #7591, #30902, #34147, #17070, #4777, #20315, #34361, #10597, #8027, #11025, #17280, #27876, #17925, #3932, #40165, #27018, #40369, #23783, #30689, #33932, #17496, #33509, #14245, #30485, #31122, #41008, #7813, #23577, #36724, #24219, #1122, #20961, #10810, #30267, #17707, #13825, #36938, #14468, #27658, #7380, #33714, #11240, #4139, #914, #37143, #24003, #24439, #14029, #37582, #21171, #1986, #18144, #5209, #21609, #28307, #15112, #8667, #41865, #15537, #18581, #28099, #22040, #5430, #41446, #8877, #12303, #18365, #28946, #31553, #2616, #38013, #35212, #14900, #31340, #1770, #25500, #22252, #11882, #24865, #5003, #19004, #38223, #5642, #8458, #25078, #21821, #38649, #34788, #35001, #31769, #41660, #2197, #18791, #28739, #11453, #15331, #28528, #12096, #8241, #24653, #2406, #25289, #38434, #31980, #9084, #35422, #5849, #41227, #32189, #11664, #15747, #37796, #21389, #34572, #22887, #22457, #22670, #16588, #16801, #32813, #12714, #39063, #38858, #42083, #33023, #32610, #3035, #42497, #6687, #12925, #16162, #35634, #39693, #42292, #13138, #13353, #9501, #3244, #36046, #6061, #35841, #29790, #16370, #29570, #6482, #29358, #20052, #23094, #19838, #26333, #19211, #25708, #26120, #3452, #9918, #32400, #23308, #9285, #10129, #29153, #26544, #15, #6273, #33246, #36463, #2823, #15956, #25911, #39274, #19419, #19629, #9708, #39485, #36257, #231, #6899, #3673, #12515, #1069, #30000, #4723, #33880, #13979, #27176, #33666, #39906, #17441, #446, #13563, #37095, #7538, #7115, #10337, #17653, #13775, #7970, #863, #4090, #20692, #3884, #36884, #30848, #20479, #36674, #23733, #40115, #17232, #30433, #40319, #1285, #34087, #4302, #17019, #40529, #23951, #10760, #27392, #14414, #7330, #26754, #30637, #21119, #26959, #10972, #33457, #20269, #30218, #27608, #40748, #14193, #657, #23525, #37529, #24168, #37315, #10548, #7761, #20905, #11190, #4510, #24388, #34308, #5375, #25029, #25240, #38172, #8616, #37744, #40958, #5586, #1718, #38594, #31502, #34738, #21772, #34524, #24817, #18739, #8407, #24595, #11609, #28043, #5160, #21558, #15059, #31931, #21982, #34950, #4947, #28479, #11829, #18312, #15281, #2358, #37962, #35373, #1932, #9034, #14847, #41610, #21335, #8188, #18094, #15485, #28690, #28257, #31289, #11401, #25448, #41394, #12044, #41170, #18526, #31715, #41817, #2146, #38384, #8825, #35160, #12255, #22199, #17872, #31068, #1502, #14636, #27824, #2570, #5800, #39440, #39020, #9456, #6228, #13090, #19374, #22622, #42032, #3407, #6014, #19579, #19791, #15904, #39228, #29310, #28898, #29108, #23047, #22839, #9666, #42455, #35797, #26498, #29524, #26290, #32763, #25655, #32140, #32561, #9874, #16325, #12462, #29741, #15699, #16542, #35586, #32978, #36002, #42244, #39643, #188, #38811, #22408, #9239, #2989, #19164, #12882, #16114, #26077, #32353, #6436, #12669, #13308, #23259, #3199, #18952, #2778, #42666, #36205, #6641, #10083, #25865, #23908, #36419, #11139, #1024, #24121, #17396, #33830, #14145, #40274, #37260, #16973, #10713, #4254, #27345, #20006, #33619, #7281, #815, #30383, #6853, #20643, #20222, #34043, #1240, #33198, #40480, #10927, #7710, #20859, #30594, #33412, #30802, #4464, #14364, #37053, #29957, #40696, #27131, #397, #13725, #3629, #30170, #23690, #17606, #27562, #16757, #40072, #13517, #26914, #26705, #17185, #10502, #3838, #39857, #10291, #23478, #36626, #36837, #7490, #7073, #609, #20434, #4040, #13938, #37913, #38122, #21717, #8357, #34262, #34474, #21508, #24981, #8775, #41562, #38332, #17826, #34690, #21288, #5110, #2312, #21931, #11561, #11353, #35110, #5535, #1451, #41770, #31021, #4896, #1667, #18259, #18684, #27775, #28637, #14796, #18044, #8140, #27992, #34900, #14586, #15439, #31448, #41343, #2097, #4678, #31240, #28426, #11779, #41121, #8567, #31882, #5322, #24769, #1882, #31663, #24339, #15227, #37480, #7924, #11995, #15011, #40911, #24547, #37698, #28208, #18476, #25191, #21073, #16488, #38541, #35944, #9404, #25812, #19314, #6174, #12202, #39177, #38762, #9817, #19742, #8982, #16272, #29471, #32712, #42613, #6387, #9188, #6586, #22784, #32922, #16066, #5752, #29687, #2937, #18905, #32301, #25395, #35535, #42192, #13040, #26235, #35324, #15855, #3145, #2722, #36153, #35746, #29053, #22359, #3356, #39384, #2520, #22998, #12619, #29259, #22149, #32086, #25604, #15646, #5964, #38968, #26024, #9610, #22567, #28846, #19115, #32508, #12834, #41981, #12411, #42402, #19528, #40019, #39804, #10449, #20804, #14091, #30116, #29901, #10871, #27292, #19954, #17552, #6800, #23423, #20171, #23641, #24064, #3570, #4413, #33360, #36572, #26654, #3780, #40224, #33142, #33992, #36787, #17131, #20588, #10026, #10236, #4198, #30332, #7018, #762, #37206, #13885, #16914, #553, #7435, #40428, #33776, #7653, #130, #17342, #13673, #36365, #16704, #339, #13461, #26865, #23207, #7224, #13253, #26440, #23851, #30545, #973, #37000, #10658, #39592, #3988, #20375, #33564, #27081, #41291, #21666, #14308, #14529, #8086, #28157, #7873, #8729, #11512, #5060, #8513, #40642, #27723, #34848, #18207, #40859, #31397, #11945, #1831, #11299, #24493, #38073, #2046, #5271, #28373, #15176, #18423, #1616, #24285, #37430, #21020, #30969, #34422, #11084, #4627, #35061, #27508, #11730, #31613, #41513, #24929, #25136, #38282, #34633, #21883, #37646, #14959, #5489, #30753, #34211, #27938, #14745, #37860, #24714, #1186, #17773, #21236, #1399, #4841, #17986, #31186, #41067, #8305, #21450, #247, #15600, #13578, #29807, #26769, #23111, #12156, #23541, #9932, #25349, #38715, #36690, #41934, #6496, #20068, #6915, #41719, #22316, #39708, #9148, #462, #31, #35489, #28802, #39922, #33263, #8939, #3689, #19645, #36273, #31833, #10145, #32042, #22103, #12365, #32829, #33041, #16604, #3260, #28588, #25563, #16388, #19856, #16817, #36480, #30016, #38495, #29588, #13154, #26348, #10352, #18639, #39501, #5710, #2269, #15391, #35277, #18861, #2471, #6704, #3469, #13369, #26561, #23325, #11414, #40335, #878, #37543, #11204, #14209, #23748, #17668, #1083, #10777, #4525, #7983, #13995, #24608, #27191, #40971, #33679, #30862, #10562, #13791, #26974, #21134, #17885, #23966, #20494, #673, #14650, #33895, #1298, #4106, #7554, #37110, #34322, #30447, #17247, #20707, #37330, #27408, #14429, #24402, #7130, #40544, #4317, #17456, #3899, #20284, #40762, #30653, #10988, #24183, #27622, #7777, #20920, #40133, #4739, #7345, #34102, #31083, #1516, #27839, #33473, #30233, #17034, #36901, #12057, #41623, #18539, #41408, #15711, #18753, #15497, #8840, #14860, #21350, #21785, #2371, #5599, #31302, #18965, #34536, #5812, #24830, #22212, #25253, #31515, #28910, #32152, #18107, #11623, #41183, #11842, #37976, #2160, #5388, #34965, #4960, #28491, #1945, #2582, #12473, #21996, #37757, #8201, #38398, #31730, #15294, #25043, #1734, #35174, #28057, #8420, #31943, #28703, #21571, #34752, #25463, #5172, #42047, #8629, #38185, #41830, #18326, #15070, #38608, #28272, #12267, #9047, #35388, #42466, #29322, #22850, #29119, #32365, #2789, #26508, #36429, #19384, #39031, #19176, #33209, #9677, #23060, #22635, #26088, #32574, #13319, #6240, #35808, #3000, #13103, #32774, #32990, #198, #407, #16337, #9466, #16125, #22420, #25668, #16555, #12894, #39239, #36012, #3418, #6449, #19591, #15918, #23270, #25877, #39451, #39655, #3210, #29535, #42677, #6026, #26302, #10092, #9886, #36216, #6652, #19802, #3640, #29753, #6865, #20016, #42255, #9251, #16767, #29967, #38822, #12680, #35598, #10301, #24349, #618, #40707, #30604, #7291, #4687, #37490, #36636, #30180, #16982, #30393, #13734, #20652, #23917, #40283, #39867, #4265, #20443, #7934, #31031, #27356, #13528, #26715, #17406, #10724, #37061, #17194, #23488, #1033, #7082, #20232, #33839, #14156, #33421, #3847, #1251, #40081, #34272, #27140, #826, #40491, #26923, #33628, #14375, #4050, #10512, #13947, #23699, #7500, #10937, #24130, #27572, #17617, #37272, #36848, #7721, #20869, #34053, #4475, #11150, #30812, #21084, #17836, #35336, #28002, #12007, #22161, #25202, #21942, #15240, #21298, #27786 ),
 ( #15021, #18269, #34910, #18055, #8369, #2322, #34700, #8150, #37923, #11572, #31458, #5120, #41353, #31894, #5546, #8577, #31250, #38343, #38134, #1892, #41574, #15451, #21519, #18916, #28220, #5763, #41132, #8785, #4908, #34486, #1678, #28649, #12213, #11790, #14806, #37708, #8993, #24992, #35122, #24778, #21727, #5332, #41779, #18487, #31675, #2109, #28438, #18698, #25406, #38552, #1463, #14596, #40920, #11363, #24558, #32099, #23010, #22580, #35758, #32520, #39396, #2949, #6186, #25616, #29698, #32312, #3156, #3367, #42204, #22795, #12845, #12422, #12630, #6597, #6398, #35957, #26037, #19325, #25824, #38979, #16077, #29270, #42414, #19753, #36164, #39189, #5976, #42623, #9623, #19539, #29483, #32935, #9415, #6812, #32723, #23219, #15865, #13053, #35546, #38774, #9200, #16500, #144, #16285, #2735, #22369, #39603, #26247, #9828, #29066, #13265, #26451, #10037, #36377, #2532, #15657, #28857, #41993, #19127, #37216, #37440, #10669, #33372, #16926, #16717, #19967, #10883, #10460, #23651, #20385, #27303, #33576, #36797, #13473, #17563, #20182, #33787, #34002, #30127, #23863, #772, #351, #564, #7663, #37011, #7447, #13898, #7235, #40651, #984, #40439, #4210, #39815, #3583, #3999, #24075, #30557, #26665, #1196, #29912, #30763, #7030, #4423, #20600, #13684, #17142, #20816, #40030, #14320, #27091, #30343, #26875, #27519, #11093, #10247, #24296, #40234, #17353, #33153, #23435, #3792, #36583, #14101, #11521, #28166, #41301, #24723, #17783, #21246, #41076, #1842, #2056, #5280, #15186, #30980, #37869, #8095, #8314, #38292, #31622, #27949, #11310, #28383, #41524, #1409, #14539, #18433, #37655, #8738, #21459, #14754, #18217, #40869, #17995, #11954, #31195, #27733, #4852, #34432, #34643, #5069, #31407, #25145, #34858, #14968, #24503, #11739, #24938, #1625, #38081, #21892, #8522, #7883, #21675, #21031, #34221, #4637, #17594, #41108, #37469, #21497, #40900, #7695, #37247, #4885, #11548, #18032, #37903, #24756, #31229, #11123, #33819, #4241, #17384, #40468, #1227, #7480, #14133, #1874, #23895, #21278, #1654, #27980, #34463, #37685, #14784, #1439, #8347, #20848, #14573, #8125, #34679, #37042, #7913, #24328, #4664, #34251, #40263, #24536, #24109, #5101, #18247, #20629, #31438, #15000, #10700, #30583, #1013, #34032, #27334, #10916, #4452, #27762, #30793, #14354, #31010, #27551, #40685, #21060, #17815, #11342, #5525, #18675, #38323, #31872, #5955, #2304, #9392, #8973, #15429, #25181, #22557, #29043, #18465, #15843, #28627, #32076, #41332, #19105, #41554, #31653, #8764, #41758, #41969, #25595, #12193, #38113, #21920, #25384, #28837, #12608, #2711, #42181, #34889, #38531, #2925, #35100, #2087, #22139, #35313, #5743, #18896, #32287, #2511, #35734, #15635, #12402, #38750, #6163, #25802, #15217, #38959, #9179, #22350, #11770, #19303, #11986, #28416, #35526, #32497, #28199, #24971, #8557, #21707, #5314, #29675, #16692, #542, #33348, #30103, #9598, #13241, #13029, #26428, #36773, #13660, #3344, #3132, #26852, #40006, #35933, #33552, #22772, #39371, #36143, #39579, #10437, #19517, #20363, #6574, #9807, #42603, #19730, #13447, #6373, #7211, #10015, #33130, #36560, #26013, #26223, #23192, #32912, #16902, #36353, #23628, #29888, #22986, #16476, #23411, #16055, #7006, #29246, #42390, #20157, #120, #32701, #16261, #29460, #6786, #19941, #39165, #3557, #12822, #327, #39791, #3768, #26642, #10224, #1384, #11285, #7859, #4826, #27277, #21008, #14514, #37632, #30317, #1171, #17539, #11070, #40628, #3977, #30952, #30534, #1601, #11497, #752, #8071, #21221, #24480, #34406, #27708, #961, #41054, #40846, #24700, #34197, #40212, #8288, #37417, #20791, #7640, #14295, #17972, #31172, #24271, #20573, #14731, #4614, #37191, #27922, #37846, #40415, #21435, #10859, #17117, #14079, #13874, #17757, #33978, #27069, #10644, #23838, #24050, #17331, #36987, #7423, #30741, #33763, #4400, #27494, #4186, #22301, #15160, #31598, #2031, #22086, #41703, #41917, #9131, #9339, #25335, #5257, #28359, #31383, #34619, #25547, #25122, #38267, #35047, #12349, #5474, #8714, #28144, #32235, #34833, #5695, #5898, #41496, #38480, #15374, #14944, #11930, #35473, #8924, #35261, #28574, #21868, #12562, #15585, #38697, #18845, #11715, #18191, #18624, #19053, #2452, #41277, #15795, #1818, #2661, #21652, #2255, #32025, #28786, #31820, #28991, #24912, #8499, #38058, #12142, #18409, #42130, #25756, #38909, #5046, #13189, #16209, #16852, #39955, #36306, #22508, #35682, #26382, #6527, #19677, #26172, #32448, #9964, #6110, #19257, #29621, #64, #42339, #2874, #10177, #6324, #497, #36092, #39318, #39534, #39112, #29411, #23362, #12975, #29199, #42551, #32654, #3296, #9758, #13612, #3501, #279, #6737, #12769, #16004, #32864, #29841, #33074, #25963, #3722, #9548, #33297, #22722, #16423, #19891, #16639, #22939, #30051, #35887, #19469, #3082, #23142, #13400, #26591, #39742, #36514, #6951, #20107, #26804, #4775, #27874, #24217, #10386, #23575, #14243, #37141, #7589, #14027, #20313, #40582, #36722, #7161, #17494, #30687, #30265, #33506, #40797, #36935, #31120, #24001, #27223, #1119, #27016, #17278, #11238, #912, #17068, #4137, #20524, #40367, #10808, #20742, #24437, #14466, #27446, #40163, #20959, #4353, #33930, #7811, #37580, #30483, #3930, #11023, #1553, #7378, #34145, #37368, #4563, #704, #27656, #21169, #17705, #23781, #13823, #17923, #30900, #1335, #33712, #8025, #34359, #14686, #10595, #38011, #8456, #28526, #5428, #5640, #15535, #15745, #31767, #11662, #21607, #37794, #41007, #31978, #31551, #1984, #41444, #18789, #11880, #15110, #34570, #38647, #41225, #12094, #12302, #34786, #2195, #21819, #21387, #5207, #28737, #15329, #41658, #18142, #24651, #25076, #2404, #8876, #5001, #22250, #8239, #9082, #28097, #8665, #38432, #35210, #28305, #35420, #31338, #14898, #1769, #38221, #24863, #18579, #34999, #25287, #18362, #22038, #41863, #5847, #11451, #25498, #19002, #32187, #2614, #12923, #26118, #32608, #38857, #16368, #28944, #3671, #36044, #6480, #6059, #9283, #16586, #12712, #6897, #42495, #3033, #19627, #2821, #35839, #29788, #19417, #35632, #22668, #39061, #16160, #29356, #39272, #229, #33021, #32811, #15954, #39483, #22885, #9707, #26332, #13351, #6271, #42081, #3242, #20050, #25909, #9916, #29568, #13, #12513, #3450, #39691, #13136, #42290, #22455, #36461, #23092, #36255, #9499, #6685, #19836, #26542, #10128, #23306, #33244, #25706, #19209, #32398, #29151, #34305, #7536, #30216, #13773, #13561, #16799, #7758, #7328, #20477, #17230, #24165, #30431, #33664, #10335, #14411, #17018, #30635, #30845, #26958, #20690, #40317, #39904, #40113, #34085, #33878, #4300, #10758, #4089, #37526, #40526, #37312, #1067, #17650, #10546, #29998, #23731, #7967, #655, #27389, #17439, #861, #444, #4507, #27605, #36882, #13977, #23523, #24385, #27174, #14190, #23949, #37093, #10969, #1282, #20902, #40745, #11187, #21116, #26752, #36672, #7113, #20267, #33455, #3883, #1715, #1499, #4720, #38382, #37959, #8404, #5157, #12042, #18309, #21555, #40955, #2357, #4944, #18524, #18737, #14844, #38169, #28254, #27821, #28040, #21980, #21769, #8613, #41391, #34735, #25447, #28477, #25238, #31713, #24592, #31065, #31499, #8823, #15279, #11398, #28689, #14633, #15484, #34521, #15056, #2144, #41608, #1929, #41816, #37741, #21332, #8185, #11826, #18091, #25026, #34947, #5372, #31286, #35158, #41167, #12254, #22198, #5584, #17869, #11606, #31929, #38593, #9033, #24814, #2569, #22838, #35372, #10082, #42454, #12881, #12461, #15698, #23046, #19163, #13307, #6227, #9455, #26076, #9238, #42243, #36203, #25863, #42031, #29107, #2777, #22621, #39019, #32560, #6640, #39439, #39227, #22407, #3198, #29308, #35796, #32761, #16541, #16113, #19373, #32352, #29740, #19790, #25654, #32977, #2988, #9665, #5799, #13089, #6013, #38810, #15903, #36001, #6435, #16324, #19578, #28897, #12668, #29523, #42665, #3406, #9873, #187, #35585, #26289, #26497, #39642, #18951, #32139, #10501, #10290, #34042, #37258, #396, #40695, #29956, #3836, #608, #20433, #4463, #26704, #27561, #13724, #16972, #7072, #26913, #20641, #13516, #1239, #4038, #40273, #1023, #33197, #20221, #17184, #40071, #24120, #33618, #17605, #23907, #33411, #30169, #30593, #7709, #14143, #20858, #30801, #27344, #36836, #16756, #39856, #23477, #36625, #23689, #3628, #7279, #23258, #6852, #4253, #40479, #10926, #17395, #33829, #14363, #27130, #36418, #30382, #10711, #20005, #814, #13937, #37052, #7489, #18257, #5109, #11137, #38708, #37697, #9349, #19265, #7923, #15804, #29000, #32244, #42141, #35483, #8139, #6120, #22310, #32458, #15594, #4677, #16014, #2464, #17825, #31239, #29210, #34473, #14585, #1665, #14795, #21287, #27990, #2671, #41120, #28796, #4895, #2884, #24338, #25557, #37479, #21071, #41927, #37912, #8356, #11560, #34261, #12359, #31020, #1450, #31447, #9142, #27773, #40910, #12572, #18043, #11352, #24768, #21507, #5910, #24545, #34689, #25765, #19063, #38918, #22518, #35691, #16433, #3305, #39543, #30066, #3733, #6748, #16221, #10188, #36316, #32874, #39753, #508, #36103, #17080, #6537, #33519, #26182, #23373, #3513, #29632, #42349, #16863, #10398, #19690, #12985, #35898, #7173, #26392, #36523, #39329, #75, #13199, #13624, #22949, #9769, #9974, #29851, #19901, #6963, #26816, #12781, #33085, #23154, #16650, #39124, #25973, #33308, #289, #13410, #26603, #20120, #39968, #23588, #6335, #36735, #42561, #20325, #3942, #9558, #22732, #19478, #32664, #3094, #29421, #4576, #34158, #11037, #33945, #8253, #11251, #8038, #1349, #7391, #13837, #14256, #37594, #40811, #23794, #11464, #27031, #41020, #17294, #40595, #27673, #24449, #4367, #24665, #10607, #4150, #33727, #17506, #30498, #37382, #24231, #27459, #40175, #36949, #20972, #24014, #37807, #5015, #14478, #30279, #718, #17718, #7825, #30913, #30701, #20538, #21182, #924, #14040, #34372, #4788, #27236, #40379, #17936, #10821, #21400, #1133, #31135, #1568, #37155, #7602, #14698, #20756, #27887, #34585, #28318, #35013, #21833, #15342, #5861, #22264, #25301, #34800, #28751, #12106, #8679, #15549, #19015, #11894, #35645, #25089, #9298, #1998, #41878, #22051, #5442, #18156, #35433, #28957, #38234, #31565, #11676, #25720, #2210, #12314, #15123, #18594, #31780, #32200, #41459, #28539, #41671, #5655, #38445, #25512, #2627, #31351, #8888, #35224, #18803, #14911, #1781, #9097, #31991, #2417, #38660, #15759, #42094, #12527, #24876, #38869, #18376, #22468, #28111, #41238, #38026, #8470, #21621, #5220, #23321, #23107, #9928, #29584, #9719, #26765, #29803, #26557, #19852, #25923, #32412, #32825, #13365, #16600, #42304, #30012, #2834, #16813, #35852, #16383, #3465, #243, #22902, #458, #29164, #22684, #9514, #36058, #6286, #13150, #27, #3256, #19222, #39705, #19431, #32621, #3046, #19641, #33036, #10141, #26345, #15968, #16174, #39497, #6700, #33259, #36476, #20064, #12726, #36269, #29369, #6910, #39918, #3685, #6493, #42510, #13574, #10348, #39075, #23536, #12937, #26133, #39286, #6075, #4735, #40128, #40967, #27187, #30443, #20490, #13990, #34099, #13787, #14646, #17452, #10984, #14425, #3895, #33676, #30648, #40331, #37539, #33891, #17882, #37326, #4102, #17243, #1295, #7979, #27618, #34318, #21129, #40758, #7550, #30229, #669, #26970, #36897, #10773, #17030, #10558, #11410, #20281, #17664, #11200, #24398, #30858, #4520, #31079, #40540, #1512, #874, #24179, #27835, #36686, #33469, #4313, #20703, #1079, #14205, #7126, #20916, #23962, #23744, #7341, #37106, #27404, #7773, #2367, #41826, #5595, #21567, #18961, #35170, #32148, #28487, #18103, #28906, #15290, #31298, #1941, #42043, #5168, #28053, #15067, #28267, #34748, #41404, #15494, #11838, #5808, #5384, #25039, #18322, #2578, #25459, #14856, #12263, #38181, #41619, #1730, #31511, #8625, #21781, #34961, #18535, #38604, #28699, #31726, #41179, #18748, #2155, #12053, #21992, #9043, #25249, #24604, #38394, #15707, #8416, #31940, #8836, #22208, #37753, #35383, #8197, #21346, #37972, #11618, #34532, #4956, #24826, #9463, #12890, #19380, #194, #35804, #22631, #6236, #42673, #19587, #19798, #29749, #29963, #3206, #25872, #32570, #9246, #12470, #3414, #2996, #16121, #26084, #32985, #39235, #29318, #6022, #10089, #12676, #26298, #26504, #42462, #16332, #36008, #35594, #9673, #13315, #29531, #13099, #6445, #22846, #33205, #36212, #16551, #39447, #32361, #38819, #32770, #39651, #23056, #19172, #36425, #22416, #23266, #42251, #9882, #6648, #6860, #20012, #3636, #2785, #29115, #15914, #16763, #39027, #25664, #10719, #27135, #26711, #33835, #36843, #37486, #17832, #14151, #403, #13525, #4260, #40278, #23912, #4045, #10297, #30599, #39863, #23484, #7495, #20648 ) ),
 .UNSPECIFIED., .F., .F., .F. ) 
 B_SPLINE_SURFACE_WITH_KNOTS ( ( 2, 2 ),
 ( 3, 2, 2, 2, 2, 2, 2, 2, 2, 2, 2, 2, 2, 2, 2, 2, 2, 2, 2, 2, 2, 2, 2, 2, 2, 2, 2, 2, 2, 2, 2, 2, 2, 2, 2, 2, 2, 2, 2, 2, 2, 2, 2, 2, 2, 2, 2, 2, 2, 2, 2, 2, 2, 2, 2, 2, 2, 2, 2, 2, 2, 2, 2, 2, 2, 2, 2, 2, 2, 2, 2, 2, 2, 2, 2, 2, 2, 2, 2, 2, 2, 2, 2, 2, 2, 2, 2, 2, 2, 2, 2, 2, 2, 2, 2, 2, 2, 2, 2, 2, 2, 2, 2, 2, 2, 2, 2, 2, 2, 2, 2, 2, 2, 2, 2, 2, 2, 2, 2, 2, 2, 2, 2, 2, 2, 2, 2, 2, 2, 2, 2, 2, 2, 2, 2, 2, 2, 2, 2, 2, 2, 2, 2, 2, 2, 2, 2, 2, 2, 2, 2, 2, 2, 2, 2, 2, 2, 2, 2, 2, 2, 2, 2, 2, 2, 2, 2, 2, 2, 2, 2, 2, 2, 2, 2, 2, 2, 2, 2, 2, 2, 2, 2, 2, 2, 2, 2, 2, 2, 2, 2, 2, 2, 2, 2, 2, 2, 2, 2, 2, 2, 2, 2, 2, 2, 2, 2, 2, 2, 2, 2, 2, 2, 2, 2, 2, 2, 2, 2, 2, 2, 2, 2, 2, 2, 2, 2, 2, 2, 2, 2, 2, 2, 2, 2, 2, 2, 2, 2, 2, 2, 2, 2, 2, 2, 2, 2, 2, 2, 2, 2, 2, 2, 2, 2, 2, 2, 2, 2, 2, 2, 2, 2, 2, 2, 2, 2, 2, 2, 2, 2, 2, 2, 2, 2, 2, 2, 2, 2, 2, 2, 2, 2, 2, 2, 2, 2, 2, 2, 2, 2, 2, 2, 2, 2, 2, 2, 2, 2, 2, 2, 2, 2, 2, 2, 2, 2, 2, 2, 2, 2, 2, 2, 2, 2, 2, 2, 2, 2, 2, 2, 2, 2, 2, 2, 2, 2, 2, 2, 2, 2, 2, 2, 2, 2, 2, 2, 2, 2, 2, 2, 2, 2, 2, 2, 2, 2, 2, 2, 2, 2, 2, 2, 2, 2, 2, 2, 2, 2, 2, 2, 2, 2, 2, 2, 2, 2, 2, 2, 2, 2, 2, 2, 2, 2, 2, 2, 2, 2, 2, 2, 2, 2, 2, 2, 2, 2, 2, 2, 2, 2, 2, 2, 2, 2, 2, 2, 2, 2, 2, 2, 2, 2, 2, 2, 2, 2, 2, 2, 2, 2, 2, 2, 2, 2, 2, 2, 2, 2, 2, 2, 2, 2, 2, 2, 2, 2, 2, 2, 2, 2, 2, 2, 2, 2, 2, 2, 2, 2, 2, 2, 2, 2, 2, 2, 2, 2, 2, 2, 2, 2, 2, 2, 2, 2, 2, 2, 2, 2, 2, 2, 2, 2, 2, 2, 2, 2, 2, 2, 2, 2, 2, 2, 2, 2, 2, 2, 2, 2, 2, 2, 2, 2, 2, 2, 2, 2, 2, 2, 2, 2, 2, 2, 2, 2, 2, 2, 2, 2, 2, 2, 2, 2, 2, 2, 2, 2, 2, 2, 2, 2, 2, 2, 2, 2, 2, 2, 2, 2, 2, 2, 2, 2, 2, 2, 2, 2, 2, 2, 2, 2, 2, 2, 2, 2, 2, 2, 2, 2, 2, 2, 2, 2, 2, 2, 2, 2, 2, 2, 2, 2, 2, 2, 2, 2, 2, 2, 2, 2, 2, 2, 2, 2, 2, 2, 2, 2, 2, 2, 2, 2, 2, 2, 2, 2, 2, 2, 2, 2, 2, 2, 2, 2, 2, 2, 2, 2, 2, 2, 2, 2, 2, 2, 2, 2, 2, 2, 2, 2, 2, 2, 2, 2, 2, 2, 2, 2, 2, 2, 2, 2, 2, 2, 2, 2, 2, 2, 2, 2, 2, 2, 2, 2, 2, 2, 2, 2, 2, 2, 2, 2, 2, 2, 2, 2, 2, 2, 2, 2, 2, 2, 2, 2, 2, 2, 2, 2, 2, 2, 2, 2, 2, 2, 2, 2, 2, 2, 2, 2, 2, 2, 2, 2, 2, 2, 2, 2, 2, 2, 2, 2, 2, 2, 2, 2, 2, 2, 2, 2, 2, 2, 2, 2, 2, 2, 2, 2, 2, 2, 2, 2, 2, 2, 2, 2, 2, 2, 2, 2, 2, 2, 2, 2, 2, 2, 2, 2, 2, 2, 2, 2, 2, 2, 2, 2, 2, 2, 2, 2, 2, 2, 2, 2, 2, 2, 2, 2, 2, 2, 2, 2, 2, 2, 2, 2, 2, 2, 2, 2, 2, 2, 2, 2, 2, 2, 2, 2, 2, 2, 2, 2, 2, 2, 2, 2, 2, 2, 2, 2, 2, 2, 2, 2, 2, 2, 2, 2, 2, 2, 2, 2, 2, 2, 2, 2, 2, 2, 2, 2, 2, 2, 2, 2, 2, 2, 2, 2, 2, 2, 2, 2, 2, 2, 2, 2, 2, 2, 2, 2, 2, 3 ),
 ( 0.000000000000000000, 1.000000000000000000 ),
 ( 0.000000000000000000, 0.001243781094527363160, 0.002487562189054726321, 0.003731343283582089481, 0.004975124378109452641, 0.006218905472636816235, 0.007462686567164178962, 0.008706467661691542556, 0.009950248756218905283, 0.01119402985074626801, 0.01243781094527363247, 0.01368159203980099520, 0.01492537313432835792, 0.01616915422885572065, 0.01741293532338308511, 0.01865671641791044610, 0.01990049751243781057, 0.02114427860696517503, 0.02238805970149253602, 0.02363184079601990048, 0.02487562189054726494, 0.02611940298507462593, 0.02736318407960199039, 0.02860696517412935486, 0.02985074626865671585, 0.03109452736318408031, 0.03233830845771144130, 0.03358208955223880576, 0.03482587064676617022, 0.03606965174129353469, 0.03731343283582089221, 0.03855721393034825667, 0.03980099502487562113, 0.04104477611940298559, 0.04228855721393035005, 0.04353233830845771452, 0.04477611940298507204, 0.04601990049751243650, 0.04726368159203980096, 0.04850746268656716542, 0.04975124378109452988, 0.05099502487562188741, 0.05223880597014925187, 0.05348258706467661633, 0.05472636815920398079, 0.05597014925373134525, 0.05721393034825870971, 0.05845771144278606724, 0.05970149253731343170, 0.06094527363184079616, 0.06218905472636816062, 0.06343283582089552508, 0.06467661691542288260, 0.06592039800995025400, 0.06716417910447761153, 0.06840796019900496905, 0.06965174129353234045, 0.07089552238805969797, 0.07213930348258706937, 0.07338308457711442689, 0.07462686567164178442, 0.07587064676616915582, 0.07711442786069651334, 0.07835820895522388474, 0.07960199004975124226, 0.08084577114427861366, 0.08208955223880597118, 0.08333333333333332871, 0.08457711442786070011, 0.08582089552238805763, 0.08706467661691542903, 0.08830845771144278655, 0.08955223880597014408, 0.09079601990049751548, 0.09203980099502487300, 0.09328358208955224440, 0.09452736318407960192, 0.09577114427860695944, 0.09701492537313433084, 0.09825870646766168837, 0.09950248756218905977, 0.1007462686567164173, 0.1019900497512437748, 0.1032338308457711462, 0.1044776119402985037, 0.1057213930348258751, 0.1069651741293532327, 0.1082089552238805902, 0.1094527363184079616, 0.1106965174129353191, 0.1119402985074626905, 0.1131840796019900480, 0.1144278606965174194, 0.1156716417910447769, 0.1169154228855721345, 0.1181592039800995059, 0.1194029850746268634, 0.1206467661691542348, 0.1218905472636815923, 0.1231343283582089498, 0.1243781094527363212, 0.1256218905472636926, 0.1268656716417910502, 0.1281094527363184077, 0.1293532338308457652, 0.1305970149253731227, 0.1318407960199005080, 0.1330845771144278655, 0.1343283582089552231, 0.1355721393034825806, 0.1368159203980099381, 0.1380597014925373234, 0.1393034825870646809, 0.1405472636815920384, 0.1417910447761193959, 0.1430348258706467535, 0.1442786069651741387, 0.1455223880597014963, 0.1467661691542288538, 0.1480099502487562113, 0.1492537313432835688, 0.1504975124378109541, 0.1517412935323383116, 0.1529850746268656692, 0.1542288557213930267, 0.1554726368159203842, 0.1567164179104477695, 0.1579601990049751270, 0.1592039800995024845, 0.1604477611940298420, 0.1616915422885572273, 0.1629353233830845848, 0.1641791044776119424, 0.1654228855721392999, 0.1666666666666666574, 0.1679104477611940427, 0.1691542288557214002, 0.1703980099502487577, 0.1716417910447761153, 0.1728855721393034728, 0.1741293532338308581, 0.1753731343283582156, 0.1766169154228855731, 0.1778606965174129306, 0.1791044776119402882, 0.1803482587064676734, 0.1815920398009950310, 0.1828358208955223885, 0.1840796019900497460, 0.1853233830845771035, 0.1865671641791044888, 0.1878109452736318463, 0.1890547263681592038, 0.1902985074626865614, 0.1915422885572139189, 0.1927860696517413042, 0.1940298507462686617, 0.1952736318407960192, 0.1965174129353233767, 0.1977611940298507343, 0.1990049751243781195, 0.2002487562189054771, 0.2014925373134328346, 0.2027363184079601921, 0.2039800995024875496, 0.2052238805970149349, 0.2064676616915422924, 0.2077114427860696499, 0.2089552238805970075, 0.2101990049751243650, 0.2114427860696517503, 0.2126865671641791078, 0.2139303482587064653, 0.2151741293532338228, 0.2164179104477611804, 0.2176616915422885656, 0.2189054726368159232, 0.2201492537313432807, 0.2213930348258706382, 0.2226368159203980235, 0.2238805970149253810, 0.2251243781094527385, 0.2263681592039800961, 0.2276119402985074536, 0.2288557213930348389, 0.2300995024875621964, 0.2313432835820895539, 0.2325870646766169114, 0.2338308457711442689, 0.2350746268656716542, 0.2363184079601990117, 0.2375621890547263693, 0.2388059701492537268, 0.2400497512437810843, 0.2412935323383084696, 0.2425373134328358271, 0.2437810945273631846, 0.2450248756218905422, 0.2462686567164178997, 0.2475124378109452850, 0.2487562189054726425, 0.2500000000000000000, 0.2512437810945273853, 0.2524875621890547150, 0.2537313432835821003, 0.2549751243781094301, 0.2562189054726368154, 0.2574626865671642006, 0.2587064676616915304, 0.2599502487562189157, 0.2611940298507462455, 0.2624378109452736307, 0.2636815920398010160, 0.2649253731343283458, 0.2661691542288557311, 0.2674129353233830608, 0.2686567164179104461, 0.2699004975124378314, 0.2711442786069651611, 0.2723880597014925464, 0.2736318407960198762, 0.2748756218905472615, 0.2761194029850746468, 0.2773631840796019765, 0.2786069651741293618, 0.2798507462686566916, 0.2810945273631840768, 0.2823383084577114621, 0.2835820895522387919, 0.2848258706467661772, 0.2860696517412935069, 0.2873134328358208922, 0.2885572139303482775, 0.2898009950248756073, 0.2910447761194029925, 0.2922885572139303223, 0.2935323383084577076, 0.2947761194029850929, 0.2960199004975124226, 0.2972636815920398079, 0.2985074626865671377, 0.2997512437810945229, 0.3009950248756219082, 0.3022388059701492380, 0.3034825870646766233, 0.3047263681592039530, 0.3059701492537313383, 0.3072139303482587236, 0.3084577114427860534, 0.3097014925373134386, 0.3109452736318407684, 0.3121890547263681537, 0.3134328358208955390, 0.3146766169154228687, 0.3159203980099502540, 0.3171641791044776393, 0.3184079601990049690, 0.3196517412935323543, 0.3208955223880596841, 0.3221393034825870694, 0.3233830845771144546, 0.3246268656716417844, 0.3258706467661691697, 0.3271144278606964995, 0.3283582089552238847, 0.3296019900497512700, 0.3308457711442785998, 0.3320895522388059851, 0.3333333333333333148, 0.3345771144278607001, 0.3358208955223880854, 0.3370646766169154152, 0.3383084577114428004, 0.3395522388059701302, 0.3407960199004975155, 0.3420398009950249008, 0.3432835820895522305, 0.3445273631840796158, 0.3457711442786069456, 0.3470149253731343308, 0.3482587064676617161, 0.3495024875621890459, 0.3507462686567164312, 0.3519900497512437609, 0.3532338308457711462, 0.3544776119402985315, 0.3557213930348258613, 0.3569651741293532465, 0.3582089552238805763, 0.3594527363184079616, 0.3606965174129353469, 0.3619402985074626766, 0.3631840796019900619, 0.3644278606965173917, 0.3656716417910447769, 0.3669154228855721622, 0.3681592039800994920, 0.3694029850746268773, 0.3706467661691542070, 0.3718905472636815923, 0.3731343283582089776, 0.3743781094527363074, 0.3756218905472636926, 0.3768656716417910224, 0.3781094527363184077, 0.3793532338308457930, 0.3805970149253731227, 0.3818407960199005080, 0.3830845771144278378, 0.3843283582089552231, 0.3855721393034826083, 0.3868159203980099381, 0.3880597014925373234, 0.3893034825870646531, 0.3905472636815920384, 0.3917910447761194237, 0.3930348258706467535, 0.3942786069651741387, 0.3955223880597014685, 0.3967661691542288538, 0.3980099502487562391, 0.3992537313432835688, 0.4004975124378109541, 0.4017412935323382839, 0.4029850746268656692, 0.4042288557213930544, 0.4054726368159203842, 0.4067164179104477695, 0.4079601990049750992, 0.4092039800995024845, 0.4104477611940298698, 0.4116915422885571996, 0.4129353233830845848, 0.4141791044776119146, 0.4154228855721392999, 0.4166666666666666852, 0.4179104477611940149, 0.4191542288557214002, 0.4203980099502487300, 0.4216417910447761153, 0.4228855721393035005, 0.4241293532338308303, 0.4253731343283582156, 0.4266169154228855454, 0.4278606965174129306, 0.4291044776119403159, 0.4303482587064676457, 0.4315920398009950310, 0.4328358208955223607, 0.4340796019900497460, 0.4353233830845771313, 0.4365671641791044610, 0.4378109452736318463, 0.4390547263681592316, 0.4402985074626865614, 0.4415422885572139466, 0.4427860696517412764, 0.4440298507462686617, 0.4452736318407960470, 0.4465174129353233767, 0.4477611940298507620, 0.4490049751243780918, 0.4502487562189054771, 0.4514925373134328623, 0.4527363184079601921, 0.4539800995024875774, 0.4552238805970149071, 0.4564676616915422924, 0.4577114427860696777, 0.4589552238805970075, 0.4601990049751243927, 0.4614427860696517225, 0.4626865671641791078, 0.4639303482587064931, 0.4651741293532338228, 0.4664179104477612081, 0.4676616915422885379, 0.4689054726368159232, 0.4701492537313433084, 0.4713930348258706382, 0.4726368159203980235, 0.4738805970149253532, 0.4751243781094527385, 0.4763681592039801238, 0.4776119402985074536, 0.4788557213930348389, 0.4800995024875621686, 0.4813432835820895539, 0.4825870646766169392, 0.4838308457711442689, 0.4850746268656716542, 0.4863184079601989840, 0.4875621890547263693, 0.4888059701492537545, 0.4900497512437810843, 0.4912935323383084696, 0.4925373134328357994, 0.4937810945273631846, 0.4950248756218905699, 0.4962686567164178997, 0.4975124378109452850, 0.4987562189054726147, 0.5000000000000000000, 0.5012437810945273853, 0.5024875621890547706, 0.5037313432835820448, 0.5049751243781094301, 0.5062189054726368154, 0.5074626865671642006, 0.5087064676616915859, 0.5099502487562188602, 0.5111940298507462455, 0.5124378109452736307, 0.5136815920398010160, 0.5149253731343284013, 0.5161691542288556755, 0.5174129353233830608, 0.5186567164179104461, 0.5199004975124378314, 0.5211442786069652167, 0.5223880597014924909, 0.5236318407960198762, 0.5248756218905472615, 0.5261194029850746468, 0.5273631840796020320, 0.5286069651741293063, 0.5298507462686566916, 0.5310945273631840768, 0.5323383084577114621, 0.5335820895522388474, 0.5348258706467661217, 0.5360696517412935069, 0.5373134328358208922, 0.5385572139303482775, 0.5398009950248756628, 0.5410447761194029370, 0.5422885572139303223, 0.5435323383084577076, 0.5447761194029850929, 0.5460199004975124781, 0.5472636815920397524, 0.5485074626865671377, 0.5497512437810945229, 0.5509950248756219082, 0.5522388059701492935, 0.5534825870646765678, 0.5547263681592039530, 0.5559701492537313383, 0.5572139303482587236, 0.5584577114427861089, 0.5597014925373133831, 0.5609452736318407684, 0.5621890547263681537, 0.5634328358208955390, 0.5646766169154229242, 0.5659203980099501985, 0.5671641791044775838, 0.5684079601990049690, 0.5696517412935323543, 0.5708955223880597396, 0.5721393034825870139, 0.5733830845771143991, 0.5746268656716417844, 0.5758706467661691697, 0.5771144278606965550, 0.5783582089552238292, 0.5796019900497512145, 0.5808457711442785998, 0.5820895522388059851, 0.5833333333333333703, 0.5845771144278606446, 0.5858208955223880299, 0.5870646766169154152, 0.5883084577114428004, 0.5895522388059701857, 0.5907960199004974600, 0.5920398009950248452, 0.5932835820895522305, 0.5945273631840796158, 0.5957711442786070011, 0.5970149253731342753, 0.5982587064676616606, 0.5995024875621890459, 0.6007462686567164312, 0.6019900497512438164, 0.6032338308457710907, 0.6044776119402984760, 0.6057213930348258613, 0.6069651741293532465, 0.6082089552238806318, 0.6094527363184079061, 0.6106965174129352913, 0.6119402985074626766, 0.6131840796019900619, 0.6144278606965174472, 0.6156716417910447214, 0.6169154228855721067, 0.6181592039800994920, 0.6194029850746268773, 0.6206467661691542625, 0.6218905472636815368, 0.6231343283582089221, 0.6243781094527363074, 0.6256218905472636926, 0.6268656716417910779, 0.6281094527363184632, 0.6293532338308457375, 0.6305970149253731227, 0.6318407960199005080, 0.6330845771144278933, 0.6343283582089552786, 0.6355721393034825528, 0.6368159203980099381, 0.6380597014925373234, 0.6393034825870647087, 0.6405472636815920939, 0.6417910447761193682, 0.6430348258706467535, 0.6442786069651741387, 0.6455223880597015240, 0.6467661691542289093, 0.6480099502487561836, 0.6492537313432835688, 0.6504975124378109541, 0.6517412935323383394, 0.6529850746268657247, 0.6542288557213929989, 0.6554726368159203842, 0.6567164179104477695, 0.6579601990049751548, 0.6592039800995025400, 0.6604477611940298143, 0.6616915422885571996, 0.6629353233830845848, 0.6641791044776119701, 0.6654228855721393554, 0.6666666666666666297, 0.6679104477611940149, 0.6691542288557214002, 0.6703980099502487855, 0.6716417910447761708, 0.6728855721393034450, 0.6741293532338308303, 0.6753731343283582156, 0.6766169154228856009, 0.6778606965174129861, 0.6791044776119402604, 0.6803482587064676457, 0.6815920398009950310, 0.6828358208955224162, 0.6840796019900498015, 0.6853233830845770758, 0.6865671641791044610, 0.6878109452736318463, 0.6890547263681592316, 0.6902985074626866169, 0.6915422885572138911, 0.6927860696517412764, 0.6940298507462686617, 0.6952736318407960470, 0.6965174129353234322, 0.6977611940298507065, 0.6990049751243780918, 0.7002487562189054771, 0.7014925373134328623, 0.7027363184079602476, 0.7039800995024875219, 0.7052238805970149071, 0.7064676616915422924, 0.7077114427860696777, 0.7089552238805970630, 0.7101990049751243372, 0.7114427860696517225, 0.7126865671641791078, 0.7139303482587064931, 0.7151741293532338783, 0.7164179104477611526, 0.7176616915422885379, 0.7189054726368159232, 0.7201492537313433084, 0.7213930348258706937, 0.7226368159203979680, 0.7238805970149253532, 0.7251243781094527385, 0.7263681592039801238, 0.7276119402985075091, 0.7288557213930347833, 0.7300995024875621686, 0.7313432835820895539, 0.7325870646766169392, 0.7338308457711443245, 0.7350746268656715987, 0.7363184079601989840, 0.7375621890547263693, 0.7388059701492537545, 0.7400497512437811398, 0.7412935323383084141, 0.7425373134328357994, 0.7437810945273631846, 0.7450248756218905699, 0.7462686567164179552, 0.7475124378109452294, 0.7487562189054726147, 0.7500000000000000000, 0.7512437810945273853, 0.7524875621890547706, 0.7537313432835820448, 0.7549751243781094301, 0.7562189054726368154, 0.7574626865671642006, 0.7587064676616915859, 0.7599502487562188602, 0.7611940298507462455, 0.7624378109452736307, 0.7636815920398010160, 0.7649253731343284013, 0.7661691542288556755, 0.7674129353233830608, 0.7686567164179104461, 0.7699004975124378314, 0.7711442786069652167, 0.7723880597014924909, 0.7736318407960198762, 0.7748756218905472615, 0.7761194029850746468, 0.7773631840796020320, 0.7786069651741293063, 0.7798507462686566916, 0.7810945273631840768, 0.7823383084577114621, 0.7835820895522388474, 0.7848258706467661217, 0.7860696517412935069, 0.7873134328358208922, 0.7885572139303482775, 0.7898009950248756628, 0.7910447761194029370, 0.7922885572139303223, 0.7935323383084577076, 0.7947761194029850929, 0.7960199004975124781, 0.7972636815920397524, 0.7985074626865671377, 0.7997512437810945229, 0.8009950248756219082, 0.8022388059701492935, 0.8034825870646765678, 0.8047263681592039530, 0.8059701492537313383, 0.8072139303482587236, 0.8084577114427861089, 0.8097014925373133831, 0.8109452736318407684, 0.8121890547263681537, 0.8134328358208955390, 0.8146766169154229242, 0.8159203980099501985, 0.8171641791044775838, 0.8184079601990049690, 0.8196517412935323543, 0.8208955223880597396, 0.8221393034825870139, 0.8233830845771143991, 0.8246268656716417844, 0.8258706467661691697, 0.8271144278606965550, 0.8283582089552238292, 0.8296019900497512145, 0.8308457711442785998, 0.8320895522388059851, 0.8333333333333333703, 0.8345771144278606446, 0.8358208955223880299, 0.8370646766169154152, 0.8383084577114428004, 0.8395522388059701857, 0.8407960199004974600, 0.8420398009950248452, 0.8432835820895522305, 0.8445273631840796158, 0.8457711442786070011, 0.8470149253731342753, 0.8482587064676616606, 0.8495024875621890459, 0.8507462686567164312, 0.8519900497512438164, 0.8532338308457710907, 0.8544776119402984760, 0.8557213930348258613, 0.8569651741293532465, 0.8582089552238806318, 0.8594527363184079061, 0.8606965174129352913, 0.8619402985074626766, 0.8631840796019900619, 0.8644278606965174472, 0.8656716417910447214, 0.8669154228855721067, 0.8681592039800994920, 0.8694029850746268773, 0.8706467661691542625, 0.8718905472636815368, 0.8731343283582089221, 0.8743781094527363074, 0.8756218905472636926, 0.8768656716417910779, 0.8781094527363184632, 0.8793532338308457375, 0.8805970149253731227, 0.8818407960199005080, 0.8830845771144278933, 0.8843283582089552786, 0.8855721393034825528, 0.8868159203980099381, 0.8880597014925373234, 0.8893034825870647087, 0.8905472636815920939, 0.8917910447761193682, 0.8930348258706467535, 0.8942786069651741387, 0.8955223880597015240, 0.8967661691542289093, 0.8980099502487561836, 0.8992537313432835688, 0.9004975124378109541, 0.9017412935323383394, 0.9029850746268657247, 0.9042288557213929989, 0.9054726368159203842, 0.9067164179104477695, 0.9079601990049751548, 0.9092039800995025400, 0.9104477611940298143, 0.9116915422885571996, 0.9129353233830845848, 0.9141791044776119701, 0.9154228855721393554, 0.9166666666666666297, 0.9179104477611940149, 0.9191542288557214002, 0.9203980099502487855, 0.9216417910447761708, 0.9228855721393034450, 0.9241293532338308303, 0.9253731343283582156, 0.9266169154228856009, 0.9278606965174129861, 0.9291044776119402604, 0.9303482587064676457, 0.9315920398009950310, 0.9328358208955224162, 0.9340796019900498015, 0.9353233830845770758, 0.9365671641791044610, 0.9378109452736318463, 0.9390547263681592316, 0.9402985074626866169, 0.9415422885572138911, 0.9427860696517412764, 0.9440298507462686617, 0.9452736318407960470, 0.9465174129353234322, 0.9477611940298507065, 0.9490049751243780918, 0.9502487562189054771, 0.9514925373134328623, 0.9527363184079602476, 0.9539800995024875219, 0.9552238805970149071, 0.9564676616915422924, 0.9577114427860696777, 0.9589552238805970630, 0.9601990049751243372, 0.9614427860696517225, 0.9626865671641791078, 0.9639303482587064931, 0.9651741293532338783, 0.9664179104477611526, 0.9676616915422885379, 0.9689054726368159232, 0.9701492537313433084, 0.9713930348258706937, 0.9726368159203979680, 0.9738805970149253532, 0.9751243781094527385, 0.9763681592039801238, 0.9776119402985075091, 0.9788557213930347833, 0.9800995024875621686, 0.9813432835820895539, 0.9825870646766169392, 0.9838308457711443245, 0.9850746268656715987, 0.9863184079601989840, 0.9875621890547263693, 0.9888059701492537545, 0.9900497512437811398, 0.9912935323383084141, 0.9925373134328357994, 0.9937810945273631846, 0.9950248756218905699 ),
 .UNSPECIFIED. ) 
 GEOMETRIC_REPRESENTATION_ITEM ( )  RATIONAL_B_SPLINE_SURFACE ( (
 ( 1.000000000000000000, 0.8660254037844387076, 1.000000000000000000, 0.8660254037844387076, 1.000000000000000000, 0.8660254037844387076, 1.000000000000000000, 0.8660254037844387076, 1.000000000000000000, 0.8660254037844387076, 1.000000000000000000, 0.8660254037844387076, 1.000000000000000000, 0.8660254037844387076, 1.000000000000000000, 0.8660254037844387076, 1.000000000000000000, 0.8660254037844387076, 1.000000000000000000, 0.8660254037844387076, 1.000000000000000000, 0.8660254037844387076, 1.000000000000000000, 0.8660254037844387076, 1.000000000000000000, 0.8660254037844387076, 1.000000000000000000, 0.8660254037844387076, 1.000000000000000000, 0.8660254037844387076, 1.000000000000000000, 0.8660254037844387076, 1.000000000000000000, 0.8660254037844387076, 1.000000000000000000, 0.8660254037844387076, 1.000000000000000000, 0.8660254037844387076, 1.000000000000000000, 0.8660254037844387076, 1.000000000000000000, 0.8660254037844387076, 1.000000000000000000, 0.8660254037844387076, 1.000000000000000000, 0.8660254037844387076, 1.000000000000000000, 0.8660254037844387076, 1.000000000000000000, 0.8660254037844387076, 1.000000000000000000, 0.8660254037844387076, 1.000000000000000000, 0.8660254037844387076, 1.000000000000000000, 0.8660254037844387076, 1.000000000000000000, 0.8660254037844387076, 1.000000000000000000, 0.8660254037844387076, 1.000000000000000000, 0.8660254037844387076, 1.000000000000000000, 0.8660254037844387076, 1.000000000000000000, 0.8660254037844387076, 1.000000000000000000, 0.8660254037844387076, 1.000000000000000000, 0.8660254037844387076, 1.000000000000000000, 0.8660254037844387076, 1.000000000000000000, 0.8660254037844387076, 1.000000000000000000, 0.8660254037844387076, 1.000000000000000000, 0.8660254037844387076, 1.000000000000000000, 0.8660254037844387076, 1.000000000000000000, 0.8660254037844387076, 1.000000000000000000, 0.8660254037844387076, 1.000000000000000000, 0.8660254037844387076, 1.000000000000000000, 0.8660254037844387076, 1.000000000000000000, 0.8660254037844387076, 1.000000000000000000, 0.8660254037844387076, 1.000000000000000000, 0.8660254037844387076, 1.000000000000000000, 0.8660254037844387076, 1.000000000000000000, 0.8660254037844387076, 1.000000000000000000, 0.8660254037844387076, 1.000000000000000000, 0.8660254037844387076, 1.000000000000000000, 0.8660254037844387076, 1.000000000000000000, 0.8660254037844387076, 1.000000000000000000, 0.8660254037844387076, 1.000000000000000000, 0.8660254037844387076, 1.000000000000000000, 0.8660254037844387076, 1.000000000000000000, 0.8660254037844387076, 1.000000000000000000, 0.8660254037844387076, 1.000000000000000000, 0.8660254037844387076, 1.000000000000000000, 0.8660254037844387076, 1.000000000000000000, 0.8660254037844387076, 1.000000000000000000, 0.8660254037844387076, 1.000000000000000000, 0.8660254037844387076, 1.000000000000000000, 0.8660254037844387076, 1.000000000000000000, 0.8660254037844387076, 1.000000000000000000, 0.8660254037844387076, 1.000000000000000000, 0.8660254037844387076, 1.000000000000000000, 0.8660254037844387076, 1.000000000000000000, 0.8660254037844387076, 1.000000000000000000, 0.8660254037844387076, 1.000000000000000000, 0.8660254037844387076, 1.000000000000000000, 0.8660254037844387076, 1.000000000000000000, 0.8660254037844387076, 1.000000000000000000, 0.8660254037844387076, 1.000000000000000000, 0.8660254037844387076, 1.000000000000000000, 0.8660254037844387076, 1.000000000000000000, 0.8660254037844387076, 1.000000000000000000, 0.8660254037844387076, 1.000000000000000000, 0.8660254037844387076, 1.000000000000000000, 0.8660254037844387076, 1.000000000000000000, 0.8660254037844387076, 1.000000000000000000, 0.8660254037844387076, 1.000000000000000000, 0.8660254037844387076, 1.000000000000000000, 0.8660254037844387076, 1.000000000000000000, 0.8660254037844387076, 1.000000000000000000, 0.8660254037844387076, 1.000000000000000000, 0.8660254037844387076, 1.000000000000000000, 0.8660254037844387076, 1.000000000000000000, 0.8660254037844387076, 1.000000000000000000, 0.8660254037844387076, 1.000000000000000000, 0.8660254037844387076, 1.000000000000000000, 0.8660254037844387076, 1.000000000000000000, 0.8660254037844387076, 1.000000000000000000, 0.8660254037844387076, 1.000000000000000000, 0.8660254037844387076, 1.000000000000000000, 0.8660254037844387076, 1.000000000000000000, 0.8660254037844387076, 1.000000000000000000, 0.8660254037844387076, 1.000000000000000000, 0.8660254037844387076, 1.000000000000000000, 0.8660254037844387076, 1.000000000000000000, 0.8660254037844387076, 1.000000000000000000, 0.8660254037844387076, 1.000000000000000000, 0.8660254037844387076, 1.000000000000000000, 0.8660254037844387076, 1.000000000000000000, 0.8660254037844387076, 1.000000000000000000, 0.8660254037844387076, 1.000000000000000000, 0.8660254037844387076, 1.000000000000000000, 0.8660254037844387076, 1.000000000000000000, 0.8660254037844387076, 1.000000000000000000, 0.8660254037844387076, 1.000000000000000000, 0.8660254037844387076, 1.000000000000000000, 0.8660254037844387076, 1.000000000000000000, 0.8660254037844387076, 1.000000000000000000, 0.8660254037844387076, 1.000000000000000000, 0.8660254037844387076, 1.000000000000000000, 0.8660254037844387076, 1.000000000000000000, 0.8660254037844387076, 1.000000000000000000, 0.8660254037844387076, 1.000000000000000000, 0.8660254037844387076, 1.000000000000000000, 0.8660254037844387076, 1.000000000000000000, 0.8660254037844387076, 1.000000000000000000, 0.8660254037844387076, 1.000000000000000000, 0.8660254037844387076, 1.000000000000000000, 0.8660254037844387076, 1.000000000000000000, 0.8660254037844387076, 1.000000000000000000, 0.8660254037844387076, 1.000000000000000000, 0.8660254037844387076, 1.000000000000000000, 0.8660254037844387076, 1.000000000000000000, 0.8660254037844387076, 1.000000000000000000, 0.8660254037844387076, 1.000000000000000000, 0.8660254037844387076, 1.000000000000000000, 0.8660254037844387076, 1.000000000000000000, 0.8660254037844387076, 1.000000000000000000, 0.8660254037844387076, 1.000000000000000000, 0.8660254037844387076, 1.000000000000000000, 0.8660254037844387076, 1.000000000000000000, 0.8660254037844387076, 1.000000000000000000, 0.8660254037844387076, 1.000000000000000000, 0.8660254037844387076, 1.000000000000000000, 0.8660254037844387076, 1.000000000000000000, 0.8660254037844387076, 1.000000000000000000, 0.8660254037844387076, 1.000000000000000000, 0.8660254037844387076, 1.000000000000000000, 0.8660254037844387076, 1.000000000000000000, 0.8660254037844387076, 1.000000000000000000, 0.8660254037844387076, 1.000000000000000000, 0.8660254037844387076, 1.000000000000000000, 0.8660254037844387076, 1.000000000000000000, 0.8660254037844387076, 1.000000000000000000, 0.8660254037844387076, 1.000000000000000000, 0.8660254037844387076, 1.000000000000000000, 0.8660254037844387076, 1.000000000000000000, 0.8660254037844387076, 1.000000000000000000, 0.8660254037844387076, 1.000000000000000000, 0.8660254037844387076, 1.000000000000000000, 0.8660254037844387076, 1.000000000000000000, 0.8660254037844387076, 1.000000000000000000, 0.8660254037844387076, 1.000000000000000000, 0.8660254037844387076, 1.000000000000000000, 0.8660254037844387076, 1.000000000000000000, 0.8660254037844387076, 1.000000000000000000, 0.8660254037844387076, 1.000000000000000000, 0.8660254037844387076, 1.000000000000000000, 0.8660254037844387076, 1.000000000000000000, 0.8660254037844387076, 1.000000000000000000, 0.8660254037844387076, 1.000000000000000000, 0.8660254037844387076, 1.000000000000000000, 0.8660254037844387076, 1.000000000000000000, 0.8660254037844387076, 1.000000000000000000, 0.8660254037844387076, 1.000000000000000000, 0.8660254037844387076, 1.000000000000000000, 0.8660254037844387076, 1.000000000000000000, 0.8660254037844387076, 1.000000000000000000, 0.8660254037844387076, 1.000000000000000000, 0.8660254037844387076, 1.000000000000000000, 0.8660254037844387076, 1.000000000000000000, 0.8660254037844387076, 1.000000000000000000, 0.8660254037844387076, 1.000000000000000000, 0.8660254037844387076, 1.000000000000000000, 0.8660254037844387076, 1.000000000000000000, 0.8660254037844387076, 1.000000000000000000, 0.8660254037844387076, 1.000000000000000000, 0.8660254037844387076, 1.000000000000000000, 0.8660254037844387076, 1.000000000000000000, 0.8660254037844387076, 1.000000000000000000, 0.8660254037844387076, 1.000000000000000000, 0.8660254037844387076, 1.000000000000000000, 0.8660254037844387076, 1.000000000000000000, 0.8660254037844387076, 1.000000000000000000, 0.8660254037844387076, 1.000000000000000000, 0.8660254037844387076, 1.000000000000000000, 0.8660254037844387076, 1.000000000000000000, 0.8660254037844387076, 1.000000000000000000, 0.8660254037844387076, 1.000000000000000000, 0.8660254037844387076, 1.000000000000000000, 0.8660254037844387076, 1.000000000000000000, 0.8660254037844387076, 1.000000000000000000, 0.8660254037844387076, 1.000000000000000000, 0.8660254037844387076, 1.000000000000000000, 0.8660254037844387076, 1.000000000000000000, 0.8660254037844387076, 1.000000000000000000, 0.8660254037844387076, 1.000000000000000000, 0.8660254037844387076, 1.000000000000000000, 0.8660254037844387076, 1.000000000000000000, 0.8660254037844387076, 1.000000000000000000, 0.8660254037844387076, 1.000000000000000000, 0.8660254037844387076, 1.000000000000000000, 0.8660254037844387076, 1.000000000000000000, 0.8660254037844387076, 1.000000000000000000, 0.8660254037844387076, 1.000000000000000000, 0.8660254037844387076, 1.000000000000000000, 0.8660254037844387076, 1.000000000000000000, 0.8660254037844387076, 1.000000000000000000, 0.8660254037844387076, 1.000000000000000000, 0.8660254037844387076, 1.000000000000000000, 0.8660254037844387076, 1.000000000000000000, 0.8660254037844387076, 1.000000000000000000, 0.8660254037844387076, 1.000000000000000000, 0.8660254037844387076, 1.000000000000000000, 0.8660254037844387076, 1.000000000000000000, 0.8660254037844387076, 1.000000000000000000, 0.8660254037844387076, 1.000000000000000000, 0.8660254037844387076, 1.000000000000000000, 0.8660254037844387076, 1.000000000000000000, 0.8660254037844387076, 1.000000000000000000, 0.8660254037844387076, 1.000000000000000000, 0.8660254037844387076, 1.000000000000000000, 0.8660254037844387076, 1.000000000000000000, 0.8660254037844387076, 1.000000000000000000, 0.8660254037844387076, 1.000000000000000000, 0.8660254037844387076, 1.000000000000000000, 0.8660254037844387076, 1.000000000000000000, 0.8660254037844387076, 1.000000000000000000, 0.8660254037844387076, 1.000000000000000000, 0.8660254037844387076, 1.000000000000000000, 0.8660254037844387076, 1.000000000000000000, 0.8660254037844387076, 1.000000000000000000, 0.8660254037844387076, 1.000000000000000000, 0.8660254037844387076, 1.000000000000000000, 0.8660254037844387076, 1.000000000000000000, 0.8660254037844387076, 1.000000000000000000, 0.8660254037844387076, 1.000000000000000000, 0.8660254037844387076, 1.000000000000000000, 0.8660254037844387076, 1.000000000000000000, 0.8660254037844387076, 1.000000000000000000, 0.8660254037844387076, 1.000000000000000000, 0.8660254037844387076, 1.000000000000000000, 0.8660254037844387076, 1.000000000000000000, 0.8660254037844387076, 1.000000000000000000, 0.8660254037844387076, 1.000000000000000000, 0.8660254037844387076, 1.000000000000000000, 0.8660254037844387076, 1.000000000000000000, 0.8660254037844387076, 1.000000000000000000, 0.8660254037844387076, 1.000000000000000000, 0.8660254037844387076, 1.000000000000000000, 0.8660254037844387076, 1.000000000000000000, 0.8660254037844387076, 1.000000000000000000, 0.8660254037844387076, 1.000000000000000000, 0.8660254037844387076, 1.000000000000000000, 0.8660254037844387076, 1.000000000000000000, 0.8660254037844387076, 1.000000000000000000, 0.8660254037844387076, 1.000000000000000000, 0.8660254037844387076, 1.000000000000000000, 0.8660254037844387076, 1.000000000000000000, 0.8660254037844387076, 1.000000000000000000, 0.8660254037844387076, 1.000000000000000000, 0.8660254037844387076, 1.000000000000000000, 0.8660254037844387076, 1.000000000000000000, 0.8660254037844387076, 1.000000000000000000, 0.8660254037844387076, 1.000000000000000000, 0.8660254037844387076, 1.000000000000000000, 0.8660254037844387076, 1.000000000000000000, 0.8660254037844387076, 1.000000000000000000, 0.8660254037844387076, 1.000000000000000000, 0.8660254037844387076, 1.000000000000000000, 0.8660254037844387076, 1.000000000000000000, 0.8660254037844387076, 1.000000000000000000, 0.8660254037844387076, 1.000000000000000000, 0.8660254037844387076, 1.000000000000000000, 0.8660254037844387076, 1.000000000000000000, 0.8660254037844387076, 1.000000000000000000, 0.8660254037844387076, 1.000000000000000000, 0.8660254037844387076, 1.000000000000000000, 0.8660254037844387076, 1.000000000000000000, 0.8660254037844387076, 1.000000000000000000, 0.8660254037844387076, 1.000000000000000000, 0.8660254037844387076, 1.000000000000000000, 0.8660254037844387076, 1.000000000000000000, 0.8660254037844387076, 1.000000000000000000, 0.8660254037844387076, 1.000000000000000000, 0.8660254037844387076, 1.000000000000000000, 0.8660254037844387076, 1.000000000000000000, 0.8660254037844387076, 1.000000000000000000, 0.8660254037844387076, 1.000000000000000000, 0.8660254037844387076, 1.000000000000000000, 0.8660254037844387076, 1.000000000000000000, 0.8660254037844387076, 1.000000000000000000, 0.8660254037844387076, 1.000000000000000000, 0.8660254037844387076, 1.000000000000000000, 0.8660254037844387076, 1.000000000000000000, 0.8660254037844387076, 1.000000000000000000, 0.8660254037844387076, 1.000000000000000000, 0.8660254037844387076, 1.000000000000000000, 0.8660254037844387076, 1.000000000000000000, 0.8660254037844387076, 1.000000000000000000, 0.8660254037844387076, 1.000000000000000000, 0.8660254037844387076, 1.000000000000000000, 0.8660254037844387076, 1.000000000000000000, 0.8660254037844387076, 1.000000000000000000, 0.8660254037844387076, 1.000000000000000000, 0.8660254037844387076, 1.000000000000000000, 0.8660254037844387076, 1.000000000000000000, 0.8660254037844387076, 1.000000000000000000, 0.8660254037844387076, 1.000000000000000000, 0.8660254037844387076, 1.000000000000000000, 0.8660254037844387076, 1.000000000000000000, 0.8660254037844387076, 1.000000000000000000, 0.8660254037844387076, 1.000000000000000000, 0.8660254037844387076, 1.000000000000000000, 0.8660254037844387076, 1.000000000000000000, 0.8660254037844387076, 1.000000000000000000, 0.8660254037844387076, 1.000000000000000000, 0.8660254037844387076, 1.000000000000000000, 0.8660254037844387076, 1.000000000000000000, 0.8660254037844387076, 1.000000000000000000, 0.8660254037844387076, 1.000000000000000000, 0.8660254037844387076, 1.000000000000000000, 0.8660254037844387076, 1.000000000000000000, 0.8660254037844387076, 1.000000000000000000, 0.8660254037844387076, 1.000000000000000000, 0.8660254037844387076, 1.000000000000000000, 0.8660254037844387076, 1.000000000000000000, 0.8660254037844387076, 1.000000000000000000, 0.8660254037844387076, 1.000000000000000000, 0.8660254037844387076, 1.000000000000000000, 0.8660254037844387076, 1.000000000000000000, 0.8660254037844387076, 1.000000000000000000, 0.8660254037844387076, 1.000000000000000000, 0.8660254037844387076, 1.000000000000000000, 0.8660254037844387076, 1.000000000000000000, 0.8660254037844387076, 1.000000000000000000, 0.8660254037844387076, 1.000000000000000000, 0.8660254037844387076, 1.000000000000000000, 0.8660254037844387076, 1.000000000000000000, 0.8660254037844387076, 1.000000000000000000, 0.8660254037844387076, 1.000000000000000000, 0.8660254037844387076, 1.000000000000000000, 0.8660254037844387076, 1.000000000000000000, 0.8660254037844387076, 1.000000000000000000, 0.8660254037844387076, 1.000000000000000000, 0.8660254037844387076, 1.000000000000000000, 0.8660254037844387076, 1.000000000000000000, 0.8660254037844387076, 1.000000000000000000, 0.8660254037844387076, 1.000000000000000000, 0.8660254037844387076, 1.000000000000000000, 0.8660254037844387076, 1.000000000000000000, 0.8660254037844387076, 1.000000000000000000, 0.8660254037844387076, 1.000000000000000000, 0.8660254037844387076, 1.000000000000000000, 0.8660254037844387076, 1.000000000000000000, 0.8660254037844387076, 1.000000000000000000, 0.8660254037844387076, 1.000000000000000000, 0.8660254037844387076, 1.000000000000000000, 0.8660254037844387076, 1.000000000000000000, 0.8660254037844387076, 1.000000000000000000, 0.8660254037844387076, 1.000000000000000000, 0.8660254037844387076, 1.000000000000000000, 0.8660254037844387076, 1.000000000000000000, 0.8660254037844387076, 1.000000000000000000, 0.8660254037844387076, 1.000000000000000000, 0.8660254037844387076, 1.000000000000000000, 0.8660254037844387076, 1.000000000000000000, 0.8660254037844387076, 1.000000000000000000, 0.8660254037844387076, 1.000000000000000000, 0.8660254037844387076, 1.000000000000000000, 0.8660254037844387076, 1.000000000000000000, 0.8660254037844387076, 1.000000000000000000, 0.8660254037844387076, 1.000000000000000000, 0.8660254037844387076, 1.000000000000000000, 0.8660254037844387076, 1.000000000000000000, 0.8660254037844387076, 1.000000000000000000, 0.8660254037844387076, 1.000000000000000000, 0.8660254037844387076, 1.000000000000000000, 0.8660254037844387076, 1.000000000000000000, 0.8660254037844387076, 1.000000000000000000, 0.8660254037844387076, 1.000000000000000000, 0.8660254037844387076, 1.000000000000000000, 0.8660254037844387076, 1.000000000000000000, 0.8660254037844387076, 1.000000000000000000, 0.8660254037844387076, 1.000000000000000000, 0.8660254037844387076, 1.000000000000000000, 0.8660254037844387076, 1.000000000000000000, 0.8660254037844387076, 1.000000000000000000, 0.8660254037844387076, 1.000000000000000000, 0.8660254037844387076, 1.000000000000000000, 0.8660254037844387076, 1.000000000000000000, 0.8660254037844387076, 1.000000000000000000, 0.8660254037844387076, 1.000000000000000000, 0.8660254037844387076, 1.000000000000000000, 0.8660254037844387076, 1.000000000000000000, 0.8660254037844387076, 1.000000000000000000, 0.8660254037844387076, 1.000000000000000000, 0.8660254037844387076, 1.000000000000000000, 0.8660254037844387076, 1.000000000000000000, 0.8660254037844387076, 1.000000000000000000, 0.8660254037844387076, 1.000000000000000000, 0.8660254037844387076, 1.000000000000000000, 0.8660254037844387076, 1.000000000000000000, 0.8660254037844387076, 1.000000000000000000, 0.8660254037844387076, 1.000000000000000000, 0.8660254037844387076, 1.000000000000000000, 0.8660254037844387076, 1.000000000000000000, 0.8660254037844387076, 1.000000000000000000, 0.8660254037844387076, 1.000000000000000000, 0.8660254037844387076, 1.000000000000000000, 0.8660254037844387076, 1.000000000000000000, 0.8660254037844387076, 1.000000000000000000, 0.8660254037844387076, 1.000000000000000000, 0.8660254037844387076, 1.000000000000000000, 0.8660254037844387076, 1.000000000000000000, 0.8660254037844387076, 1.000000000000000000, 0.8660254037844387076, 1.000000000000000000, 0.8660254037844387076, 1.000000000000000000, 0.8660254037844387076, 1.000000000000000000, 0.8660254037844387076, 1.000000000000000000, 0.8660254037844387076, 1.000000000000000000, 0.8660254037844387076, 1.000000000000000000, 0.8660254037844387076, 1.000000000000000000, 0.8660254037844387076, 1.000000000000000000, 0.8660254037844387076, 1.000000000000000000, 0.8660254037844387076, 1.000000000000000000, 0.8660254037844387076, 1.000000000000000000, 0.8660254037844387076, 1.000000000000000000, 0.8660254037844387076, 1.000000000000000000, 0.8660254037844387076, 1.000000000000000000, 0.8660254037844387076, 1.000000000000000000, 0.8660254037844387076, 1.000000000000000000, 0.8660254037844387076, 1.000000000000000000, 0.8660254037844387076, 1.000000000000000000, 0.8660254037844387076, 1.000000000000000000, 0.8660254037844387076, 1.000000000000000000, 0.8660254037844387076, 1.000000000000000000, 0.8660254037844387076, 1.000000000000000000, 0.8660254037844387076, 1.000000000000000000, 0.8660254037844387076, 1.000000000000000000, 0.8660254037844387076, 1.000000000000000000, 0.8660254037844387076, 1.000000000000000000, 0.8660254037844387076, 1.000000000000000000, 0.8660254037844387076, 1.000000000000000000, 0.8660254037844387076, 1.000000000000000000, 0.8660254037844387076, 1.000000000000000000, 0.8660254037844387076, 1.000000000000000000, 0.8660254037844387076, 1.000000000000000000, 0.8660254037844387076, 1.000000000000000000, 0.8660254037844387076, 1.000000000000000000, 0.8660254037844387076, 1.000000000000000000, 0.8660254037844387076, 1.000000000000000000, 0.8660254037844387076, 1.000000000000000000, 0.8660254037844387076, 1.000000000000000000, 0.8660254037844387076, 1.000000000000000000, 0.8660254037844387076, 1.000000000000000000, 0.8660254037844387076, 1.000000000000000000, 0.8660254037844387076, 1.000000000000000000, 0.8660254037844387076, 1.000000000000000000, 0.8660254037844387076, 1.000000000000000000, 0.8660254037844387076, 1.000000000000000000, 0.8660254037844387076, 1.000000000000000000, 0.8660254037844387076, 1.000000000000000000, 0.8660254037844387076, 1.000000000000000000, 0.8660254037844387076, 1.000000000000000000, 0.8660254037844387076, 1.000000000000000000, 0.8660254037844387076, 1.000000000000000000, 0.8660254037844387076, 1.000000000000000000, 0.8660254037844387076, 1.000000000000000000, 0.8660254037844387076, 1.000000000000000000, 0.8660254037844387076, 1.000000000000000000, 0.8660254037844387076, 1.000000000000000000, 0.8660254037844387076, 1.000000000000000000, 0.8660254037844387076, 1.000000000000000000, 0.8660254037844387076, 1.000000000000000000, 0.8660254037844387076, 1.000000000000000000, 0.8660254037844387076, 1.000000000000000000, 0.8660254037844387076, 1.000000000000000000, 0.8660254037844387076, 1.000000000000000000, 0.8660254037844387076, 1.000000000000000000, 0.8660254037844387076, 1.000000000000000000, 0.8660254037844387076, 1.000000000000000000, 0.8660254037844387076, 1.000000000000000000, 0.8660254037844387076, 1.000000000000000000, 0.8660254037844387076, 1.000000000000000000, 0.8660254037844387076, 1.000000000000000000, 0.8660254037844387076, 1.000000000000000000, 0.8660254037844387076, 1.000000000000000000, 0.8660254037844387076, 1.000000000000000000, 0.8660254037844387076, 1.000000000000000000, 0.8660254037844387076, 1.000000000000000000, 0.8660254037844387076, 1.000000000000000000, 0.8660254037844387076, 1.000000000000000000, 0.8660254037844387076, 1.000000000000000000, 0.8660254037844387076, 1.000000000000000000, 0.8660254037844387076, 1.000000000000000000, 0.8660254037844387076, 1.000000000000000000, 0.8660254037844387076, 1.000000000000000000, 0.8660254037844387076, 1.000000000000000000, 0.8660254037844387076, 1.000000000000000000, 0.8660254037844387076, 1.000000000000000000, 0.8660254037844387076, 1.000000000000000000, 0.8660254037844387076, 1.000000000000000000, 0.8660254037844387076, 1.000000000000000000, 0.8660254037844387076, 1.000000000000000000, 0.8660254037844387076, 1.000000000000000000, 0.8660254037844387076, 1.000000000000000000, 0.8660254037844387076, 1.000000000000000000, 0.8660254037844387076, 1.000000000000000000, 0.8660254037844387076, 1.000000000000000000, 0.8660254037844387076, 1.000000000000000000, 0.8660254037844387076, 1.000000000000000000, 0.8660254037844387076, 1.000000000000000000, 0.8660254037844387076, 1.000000000000000000, 0.8660254037844387076, 1.000000000000000000, 0.8660254037844387076, 1.000000000000000000, 0.8660254037844387076, 1.000000000000000000, 0.8660254037844387076, 1.000000000000000000, 0.8660254037844387076, 1.000000000000000000, 0.8660254037844387076, 1.000000000000000000, 0.8660254037844387076, 1.000000000000000000, 0.8660254037844387076, 1.000000000000000000, 0.8660254037844387076, 1.000000000000000000, 0.8660254037844387076, 1.000000000000000000, 0.8660254037844387076, 1.000000000000000000, 0.8660254037844387076, 1.000000000000000000, 0.8660254037844387076, 1.000000000000000000, 0.8660254037844387076, 1.000000000000000000, 0.8660254037844387076, 1.000000000000000000, 0.8660254037844387076, 1.000000000000000000, 0.8660254037844387076, 1.000000000000000000, 0.8660254037844387076, 1.000000000000000000, 0.8660254037844387076, 1.000000000000000000, 0.8660254037844387076, 1.000000000000000000, 0.8660254037844387076, 1.000000000000000000, 0.8660254037844387076, 1.000000000000000000, 0.8660254037844387076, 1.000000000000000000, 0.8660254037844387076, 1.000000000000000000, 0.8660254037844387076, 1.000000000000000000, 0.8660254037844387076, 1.000000000000000000, 0.8660254037844387076, 1.000000000000000000, 0.8660254037844387076, 1.000000000000000000, 0.8660254037844387076, 1.000000000000000000, 0.8660254037844387076, 1.000000000000000000, 0.8660254037844387076, 1.000000000000000000, 0.8660254037844387076, 1.000000000000000000, 0.8660254037844387076, 1.000000000000000000, 0.8660254037844387076, 1.000000000000000000, 0.8660254037844387076, 1.000000000000000000, 0.8660254037844387076, 1.000000000000000000, 0.8660254037844387076, 1.000000000000000000, 0.8660254037844387076, 1.000000000000000000, 0.8660254037844387076, 1.000000000000000000, 0.8660254037844387076, 1.000000000000000000, 0.8660254037844387076, 1.000000000000000000, 0.8660254037844387076, 1.000000000000000000, 0.8660254037844387076, 1.000000000000000000, 0.8660254037844387076, 1.000000000000000000, 0.8660254037844387076, 1.000000000000000000, 0.8660254037844387076, 1.000000000000000000, 0.8660254037844387076, 1.000000000000000000, 0.8660254037844387076, 1.000000000000000000, 0.8660254037844387076, 1.000000000000000000, 0.8660254037844387076, 1.000000000000000000, 0.8660254037844387076, 1.000000000000000000, 0.8660254037844387076, 1.000000000000000000, 0.8660254037844387076, 1.000000000000000000, 0.8660254037844387076, 1.000000000000000000, 0.8660254037844387076, 1.000000000000000000, 0.8660254037844387076, 1.000000000000000000, 0.8660254037844387076, 1.000000000000000000, 0.8660254037844387076, 1.000000000000000000, 0.8660254037844387076, 1.000000000000000000, 0.8660254037844387076, 1.000000000000000000, 0.8660254037844387076, 1.000000000000000000, 0.8660254037844387076, 1.000000000000000000, 0.8660254037844387076, 1.000000000000000000, 0.8660254037844387076, 1.000000000000000000, 0.8660254037844387076, 1.000000000000000000, 0.8660254037844387076, 1.000000000000000000, 0.8660254037844387076, 1.000000000000000000, 0.8660254037844387076, 1.000000000000000000, 0.8660254037844387076, 1.000000000000000000, 0.8660254037844387076, 1.000000000000000000, 0.8660254037844387076, 1.000000000000000000, 0.8660254037844387076, 1.000000000000000000, 0.8660254037844387076, 1.000000000000000000, 0.8660254037844387076, 1.000000000000000000, 0.8660254037844387076, 1.000000000000000000, 0.8660254037844387076, 1.000000000000000000, 0.8660254037844387076, 1.000000000000000000, 0.8660254037844387076, 1.000000000000000000, 0.8660254037844387076, 1.000000000000000000, 0.8660254037844387076, 1.000000000000000000, 0.8660254037844387076, 1.000000000000000000, 0.8660254037844387076, 1.000000000000000000, 0.8660254037844387076, 1.000000000000000000, 0.8660254037844387076, 1.000000000000000000, 0.8660254037844387076, 1.000000000000000000, 0.8660254037844387076, 1.000000000000000000, 0.8660254037844387076, 1.000000000000000000, 0.8660254037844387076, 1.000000000000000000, 0.8660254037844387076, 1.000000000000000000, 0.8660254037844387076, 1.000000000000000000, 0.8660254037844387076, 1.000000000000000000, 0.8660254037844387076, 1.000000000000000000, 0.8660254037844387076, 1.000000000000000000, 0.8660254037844387076, 1.000000000000000000, 0.8660254037844387076, 1.000000000000000000, 0.8660254037844387076, 1.000000000000000000, 0.8660254037844387076, 1.000000000000000000, 0.8660254037844387076, 1.000000000000000000, 0.8660254037844387076, 1.000000000000000000, 0.8660254037844387076, 1.000000000000000000, 0.8660254037844387076, 1.000000000000000000, 0.8660254037844387076, 1.000000000000000000, 0.8660254037844387076, 1.000000000000000000, 0.8660254037844387076, 1.000000000000000000, 0.8660254037844387076, 1.000000000000000000, 0.8660254037844387076, 1.000000000000000000, 0.8660254037844387076, 1.000000000000000000, 0.8660254037844387076, 1.000000000000000000, 0.8660254037844387076, 1.000000000000000000, 0.8660254037844387076, 1.000000000000000000, 0.8660254037844387076, 1.000000000000000000, 0.8660254037844387076, 1.000000000000000000, 0.8660254037844387076, 1.000000000000000000, 0.8660254037844387076, 1.000000000000000000, 0.8660254037844387076, 1.000000000000000000, 0.8660254037844387076, 1.000000000000000000, 0.8660254037844387076, 1.000000000000000000, 0.8660254037844387076, 1.000000000000000000, 0.8660254037844387076, 1.000000000000000000, 0.8660254037844387076, 1.000000000000000000, 0.8660254037844387076, 1.000000000000000000, 0.8660254037844387076, 1.000000000000000000, 0.8660254037844387076, 1.000000000000000000, 0.8660254037844387076, 1.000000000000000000, 0.8660254037844387076, 1.000000000000000000, 0.8660254037844387076, 1.000000000000000000, 0.8660254037844387076, 1.000000000000000000, 0.8660254037844387076, 1.000000000000000000, 0.8660254037844387076, 1.000000000000000000, 0.8660254037844387076, 1.000000000000000000, 0.8660254037844387076, 1.000000000000000000, 0.8660254037844387076, 1.000000000000000000, 0.8660254037844387076, 1.000000000000000000, 0.8660254037844387076, 1.000000000000000000, 0.8660254037844387076, 1.000000000000000000, 0.8660254037844387076, 1.000000000000000000, 0.8660254037844387076, 1.000000000000000000, 0.8660254037844387076, 1.000000000000000000, 0.8660254037844387076, 1.000000000000000000, 0.8660254037844387076, 1.000000000000000000, 0.8660254037844387076, 1.000000000000000000, 0.8660254037844387076, 1.000000000000000000, 0.8660254037844387076, 1.000000000000000000, 0.8660254037844387076, 1.000000000000000000, 0.8660254037844387076, 1.000000000000000000, 0.8660254037844387076, 1.000000000000000000, 0.8660254037844387076, 1.000000000000000000, 0.8660254037844387076, 1.000000000000000000, 0.8660254037844387076, 1.000000000000000000, 0.8660254037844387076, 1.000000000000000000, 0.8660254037844387076, 1.000000000000000000, 0.8660254037844387076, 1.000000000000000000, 0.8660254037844387076, 1.000000000000000000, 0.8660254037844387076, 1.000000000000000000, 0.8660254037844387076, 1.000000000000000000, 0.8660254037844387076, 1.000000000000000000, 0.8660254037844387076, 1.000000000000000000, 0.8660254037844387076, 1.000000000000000000, 0.8660254037844387076, 1.000000000000000000, 0.8660254037844387076, 1.000000000000000000, 0.8660254037844387076, 1.000000000000000000, 0.8660254037844387076, 1.000000000000000000, 0.8660254037844387076, 1.000000000000000000, 0.8660254037844387076, 1.000000000000000000, 0.8660254037844387076, 1.000000000000000000, 0.8660254037844387076, 1.000000000000000000, 0.8660254037844387076, 1.000000000000000000, 0.8660254037844387076, 1.000000000000000000, 0.8660254037844387076, 1.000000000000000000, 0.8660254037844387076, 1.000000000000000000, 0.8660254037844387076, 1.000000000000000000, 0.8660254037844387076, 1.000000000000000000, 0.8660254037844387076, 1.000000000000000000, 0.8660254037844387076, 1.000000000000000000, 0.8660254037844387076, 1.000000000000000000, 0.8660254037844387076, 1.000000000000000000, 0.8660254037844387076, 1.000000000000000000, 0.8660254037844387076, 1.000000000000000000, 0.8660254037844387076, 1.000000000000000000, 0.8660254037844387076, 1.000000000000000000, 0.8660254037844387076, 1.000000000000000000, 0.8660254037844387076, 1.000000000000000000, 0.8660254037844387076, 1.000000000000000000, 0.8660254037844387076, 1.000000000000000000, 0.8660254037844387076, 1.000000000000000000, 0.8660254037844387076, 1.000000000000000000, 0.8660254037844387076, 1.000000000000000000, 0.8660254037844387076, 1.000000000000000000, 0.8660254037844387076, 1.000000000000000000, 0.8660254037844387076, 1.000000000000000000, 0.8660254037844387076, 1.000000000000000000, 0.8660254037844387076, 1.000000000000000000, 0.8660254037844387076, 1.000000000000000000, 0.8660254037844387076, 1.000000000000000000, 0.8660254037844387076, 1.000000000000000000, 0.8660254037844387076, 1.000000000000000000, 0.8660254037844387076, 1.000000000000000000, 0.8660254037844387076, 1.000000000000000000, 0.8660254037844387076, 1.000000000000000000, 0.8660254037844387076, 1.000000000000000000, 0.8660254037844387076, 1.000000000000000000, 0.8660254037844387076, 1.000000000000000000, 0.8660254037844387076, 1.000000000000000000, 0.8660254037844387076, 1.000000000000000000, 0.8660254037844387076, 1.000000000000000000, 0.8660254037844387076, 1.000000000000000000, 0.8660254037844387076, 1.000000000000000000, 0.8660254037844387076, 1.000000000000000000, 0.8660254037844387076, 1.000000000000000000, 0.8660254037844387076, 1.000000000000000000, 0.8660254037844387076, 1.000000000000000000, 0.8660254037844387076, 1.000000000000000000, 0.8660254037844387076, 1.000000000000000000, 0.8660254037844387076, 1.000000000000000000, 0.8660254037844387076, 1.000000000000000000, 0.8660254037844387076, 1.000000000000000000, 0.8660254037844387076, 1.000000000000000000, 0.8660254037844387076, 1.000000000000000000, 0.8660254037844387076, 1.000000000000000000, 0.8660254037844387076, 1.000000000000000000, 0.8660254037844387076, 1.000000000000000000, 0.8660254037844387076, 1.000000000000000000, 0.8660254037844387076, 1.000000000000000000, 0.8660254037844387076, 1.000000000000000000, 0.8660254037844387076, 1.000000000000000000, 0.8660254037844387076, 1.000000000000000000, 0.8660254037844387076, 1.000000000000000000, 0.8660254037844387076, 1.000000000000000000, 0.8660254037844387076, 1.000000000000000000, 0.8660254037844387076, 1.000000000000000000, 0.8660254037844387076, 1.000000000000000000, 0.8660254037844387076, 1.000000000000000000, 0.8660254037844387076, 1.000000000000000000, 0.8660254037844387076, 1.000000000000000000, 0.8660254037844387076, 1.000000000000000000, 0.8660254037844387076, 1.000000000000000000, 0.8660254037844387076, 1.000000000000000000, 0.8660254037844387076, 1.000000000000000000, 0.8660254037844387076, 1.000000000000000000, 0.8660254037844387076, 1.000000000000000000, 0.8660254037844387076, 1.000000000000000000, 0.8660254037844387076, 1.000000000000000000, 0.8660254037844387076, 1.000000000000000000, 0.8660254037844387076, 1.000000000000000000, 0.8660254037844387076, 1.000000000000000000, 0.8660254037844387076, 1.000000000000000000, 0.8660254037844387076, 1.000000000000000000, 0.8660254037844387076, 1.000000000000000000, 0.8660254037844387076, 1.000000000000000000, 0.8660254037844387076, 1.000000000000000000, 0.8660254037844387076, 1.000000000000000000, 0.8660254037844387076, 1.000000000000000000, 0.8660254037844387076, 1.000000000000000000, 0.8660254037844387076, 1.000000000000000000, 0.8660254037844387076, 1.000000000000000000, 0.8660254037844387076, 1.000000000000000000, 0.8660254037844387076, 1.000000000000000000, 0.8660254037844387076, 1.000000000000000000, 0.8660254037844387076, 1.000000000000000000, 0.8660254037844387076, 1.000000000000000000, 0.8660254037844387076, 1.000000000000000000, 0.8660254037844387076, 1.000000000000000000, 0.8660254037844387076, 1.000000000000000000, 0.8660254037844387076, 1.000000000000000000, 0.8660254037844387076, 1.000000000000000000, 0.8660254037844387076, 1.000000000000000000, 0.8660254037844387076, 1.000000000000000000, 0.8660254037844387076, 1.000000000000000000, 0.8660254037844387076, 1.000000000000000000, 0.8660254037844387076, 1.000000000000000000, 0.8660254037844387076, 1.000000000000000000, 0.8660254037844387076, 1.000000000000000000, 0.8660254037844387076, 1.000000000000000000, 0.8660254037844387076, 1.000000000000000000, 0.8660254037844387076, 1.000000000000000000, 0.8660254037844387076, 1.000000000000000000, 0.8660254037844387076, 1.000000000000000000, 0.8660254037844387076, 1.000000000000000000, 0.8660254037844387076, 1.000000000000000000, 0.8660254037844387076, 1.000000000000000000, 0.8660254037844387076, 1.000000000000000000),
 ( 1.000000000000000000, 0.8660254037844387076, 1.000000000000000000, 0.8660254037844387076, 1.000000000000000000, 0.8660254037844387076, 1.000000000000000000, 0.8660254037844387076, 1.000000000000000000, 0.8660254037844387076, 1.000000000000000000, 0.8660254037844387076, 1.000000000000000000, 0.8660254037844387076, 1.000000000000000000, 0.8660254037844387076, 1.000000000000000000, 0.8660254037844387076, 1.000000000000000000, 0.8660254037844387076, 1.000000000000000000, 0.8660254037844387076, 1.000000000000000000, 0.8660254037844387076, 1.000000000000000000, 0.8660254037844387076, 1.000000000000000000, 0.8660254037844387076, 1.000000000000000000, 0.8660254037844387076, 1.000000000000000000, 0.8660254037844387076, 1.000000000000000000, 0.8660254037844387076, 1.000000000000000000, 0.8660254037844387076, 1.000000000000000000, 0.8660254037844387076, 1.000000000000000000, 0.8660254037844387076, 1.000000000000000000, 0.8660254037844387076, 1.000000000000000000, 0.8660254037844387076, 1.000000000000000000, 0.8660254037844387076, 1.000000000000000000, 0.8660254037844387076, 1.000000000000000000, 0.8660254037844387076, 1.000000000000000000, 0.8660254037844387076, 1.000000000000000000, 0.8660254037844387076, 1.000000000000000000, 0.8660254037844387076, 1.000000000000000000, 0.8660254037844387076, 1.000000000000000000, 0.8660254037844387076, 1.000000000000000000, 0.8660254037844387076, 1.000000000000000000, 0.8660254037844387076, 1.000000000000000000, 0.8660254037844387076, 1.000000000000000000, 0.8660254037844387076, 1.000000000000000000, 0.8660254037844387076, 1.000000000000000000, 0.8660254037844387076, 1.000000000000000000, 0.8660254037844387076, 1.000000000000000000, 0.8660254037844387076, 1.000000000000000000, 0.8660254037844387076, 1.000000000000000000, 0.8660254037844387076, 1.000000000000000000, 0.8660254037844387076, 1.000000000000000000, 0.8660254037844387076, 1.000000000000000000, 0.8660254037844387076, 1.000000000000000000, 0.8660254037844387076, 1.000000000000000000, 0.8660254037844387076, 1.000000000000000000, 0.8660254037844387076, 1.000000000000000000, 0.8660254037844387076, 1.000000000000000000, 0.8660254037844387076, 1.000000000000000000, 0.8660254037844387076, 1.000000000000000000, 0.8660254037844387076, 1.000000000000000000, 0.8660254037844387076, 1.000000000000000000, 0.8660254037844387076, 1.000000000000000000, 0.8660254037844387076, 1.000000000000000000, 0.8660254037844387076, 1.000000000000000000, 0.8660254037844387076, 1.000000000000000000, 0.8660254037844387076, 1.000000000000000000, 0.8660254037844387076, 1.000000000000000000, 0.8660254037844387076, 1.000000000000000000, 0.8660254037844387076, 1.000000000000000000, 0.8660254037844387076, 1.000000000000000000, 0.8660254037844387076, 1.000000000000000000, 0.8660254037844387076, 1.000000000000000000, 0.8660254037844387076, 1.000000000000000000, 0.8660254037844387076, 1.000000000000000000, 0.8660254037844387076, 1.000000000000000000, 0.8660254037844387076, 1.000000000000000000, 0.8660254037844387076, 1.000000000000000000, 0.8660254037844387076, 1.000000000000000000, 0.8660254037844387076, 1.000000000000000000, 0.8660254037844387076, 1.000000000000000000, 0.8660254037844387076, 1.000000000000000000, 0.8660254037844387076, 1.000000000000000000, 0.8660254037844387076, 1.000000000000000000, 0.8660254037844387076, 1.000000000000000000, 0.8660254037844387076, 1.000000000000000000, 0.8660254037844387076, 1.000000000000000000, 0.8660254037844387076, 1.000000000000000000, 0.8660254037844387076, 1.000000000000000000, 0.8660254037844387076, 1.000000000000000000, 0.8660254037844387076, 1.000000000000000000, 0.8660254037844387076, 1.000000000000000000, 0.8660254037844387076, 1.000000000000000000, 0.8660254037844387076, 1.000000000000000000, 0.8660254037844387076, 1.000000000000000000, 0.8660254037844387076, 1.000000000000000000, 0.8660254037844387076, 1.000000000000000000, 0.8660254037844387076, 1.000000000000000000, 0.8660254037844387076, 1.000000000000000000, 0.8660254037844387076, 1.000000000000000000, 0.8660254037844387076, 1.000000000000000000, 0.8660254037844387076, 1.000000000000000000, 0.8660254037844387076, 1.000000000000000000, 0.8660254037844387076, 1.000000000000000000, 0.8660254037844387076, 1.000000000000000000, 0.8660254037844387076, 1.000000000000000000, 0.8660254037844387076, 1.000000000000000000, 0.8660254037844387076, 1.000000000000000000, 0.8660254037844387076, 1.000000000000000000, 0.8660254037844387076, 1.000000000000000000, 0.8660254037844387076, 1.000000000000000000, 0.8660254037844387076, 1.000000000000000000, 0.8660254037844387076, 1.000000000000000000, 0.8660254037844387076, 1.000000000000000000, 0.8660254037844387076, 1.000000000000000000, 0.8660254037844387076, 1.000000000000000000, 0.8660254037844387076, 1.000000000000000000, 0.8660254037844387076, 1.000000000000000000, 0.8660254037844387076, 1.000000000000000000, 0.8660254037844387076, 1.000000000000000000, 0.8660254037844387076, 1.000000000000000000, 0.8660254037844387076, 1.000000000000000000, 0.8660254037844387076, 1.000000000000000000, 0.8660254037844387076, 1.000000000000000000, 0.8660254037844387076, 1.000000000000000000, 0.8660254037844387076, 1.000000000000000000, 0.8660254037844387076, 1.000000000000000000, 0.8660254037844387076, 1.000000000000000000, 0.8660254037844387076, 1.000000000000000000, 0.8660254037844387076, 1.000000000000000000, 0.8660254037844387076, 1.000000000000000000, 0.8660254037844387076, 1.000000000000000000, 0.8660254037844387076, 1.000000000000000000, 0.8660254037844387076, 1.000000000000000000, 0.8660254037844387076, 1.000000000000000000, 0.8660254037844387076, 1.000000000000000000, 0.8660254037844387076, 1.000000000000000000, 0.8660254037844387076, 1.000000000000000000, 0.8660254037844387076, 1.000000000000000000, 0.8660254037844387076, 1.000000000000000000, 0.8660254037844387076, 1.000000000000000000, 0.8660254037844387076, 1.000000000000000000, 0.8660254037844387076, 1.000000000000000000, 0.8660254037844387076, 1.000000000000000000, 0.8660254037844387076, 1.000000000000000000, 0.8660254037844387076, 1.000000000000000000, 0.8660254037844387076, 1.000000000000000000, 0.8660254037844387076, 1.000000000000000000, 0.8660254037844387076, 1.000000000000000000, 0.8660254037844387076, 1.000000000000000000, 0.8660254037844387076, 1.000000000000000000, 0.8660254037844387076, 1.000000000000000000, 0.8660254037844387076, 1.000000000000000000, 0.8660254037844387076, 1.000000000000000000, 0.8660254037844387076, 1.000000000000000000, 0.8660254037844387076, 1.000000000000000000, 0.8660254037844387076, 1.000000000000000000, 0.8660254037844387076, 1.000000000000000000, 0.8660254037844387076, 1.000000000000000000, 0.8660254037844387076, 1.000000000000000000, 0.8660254037844387076, 1.000000000000000000, 0.8660254037844387076, 1.000000000000000000, 0.8660254037844387076, 1.000000000000000000, 0.8660254037844387076, 1.000000000000000000, 0.8660254037844387076, 1.000000000000000000, 0.8660254037844387076, 1.000000000000000000, 0.8660254037844387076, 1.000000000000000000, 0.8660254037844387076, 1.000000000000000000, 0.8660254037844387076, 1.000000000000000000, 0.8660254037844387076, 1.000000000000000000, 0.8660254037844387076, 1.000000000000000000, 0.8660254037844387076, 1.000000000000000000, 0.8660254037844387076, 1.000000000000000000, 0.8660254037844387076, 1.000000000000000000, 0.8660254037844387076, 1.000000000000000000, 0.8660254037844387076, 1.000000000000000000, 0.8660254037844387076, 1.000000000000000000, 0.8660254037844387076, 1.000000000000000000, 0.8660254037844387076, 1.000000000000000000, 0.8660254037844387076, 1.000000000000000000, 0.8660254037844387076, 1.000000000000000000, 0.8660254037844387076, 1.000000000000000000, 0.8660254037844387076, 1.000000000000000000, 0.8660254037844387076, 1.000000000000000000, 0.8660254037844387076, 1.000000000000000000, 0.8660254037844387076, 1.000000000000000000, 0.8660254037844387076, 1.000000000000000000, 0.8660254037844387076, 1.000000000000000000, 0.8660254037844387076, 1.000000000000000000, 0.8660254037844387076, 1.000000000000000000, 0.8660254037844387076, 1.000000000000000000, 0.8660254037844387076, 1.000000000000000000, 0.8660254037844387076, 1.000000000000000000, 0.8660254037844387076, 1.000000000000000000, 0.8660254037844387076, 1.000000000000000000, 0.8660254037844387076, 1.000000000000000000, 0.8660254037844387076, 1.000000000000000000, 0.8660254037844387076, 1.000000000000000000, 0.8660254037844387076, 1.000000000000000000, 0.8660254037844387076, 1.000000000000000000, 0.8660254037844387076, 1.000000000000000000, 0.8660254037844387076, 1.000000000000000000, 0.8660254037844387076, 1.000000000000000000, 0.8660254037844387076, 1.000000000000000000, 0.8660254037844387076, 1.000000000000000000, 0.8660254037844387076, 1.000000000000000000, 0.8660254037844387076, 1.000000000000000000, 0.8660254037844387076, 1.000000000000000000, 0.8660254037844387076, 1.000000000000000000, 0.8660254037844387076, 1.000000000000000000, 0.8660254037844387076, 1.000000000000000000, 0.8660254037844387076, 1.000000000000000000, 0.8660254037844387076, 1.000000000000000000, 0.8660254037844387076, 1.000000000000000000, 0.8660254037844387076, 1.000000000000000000, 0.8660254037844387076, 1.000000000000000000, 0.8660254037844387076, 1.000000000000000000, 0.8660254037844387076, 1.000000000000000000, 0.8660254037844387076, 1.000000000000000000, 0.8660254037844387076, 1.000000000000000000, 0.8660254037844387076, 1.000000000000000000, 0.8660254037844387076, 1.000000000000000000, 0.8660254037844387076, 1.000000000000000000, 0.8660254037844387076, 1.000000000000000000, 0.8660254037844387076, 1.000000000000000000, 0.8660254037844387076, 1.000000000000000000, 0.8660254037844387076, 1.000000000000000000, 0.8660254037844387076, 1.000000000000000000, 0.8660254037844387076, 1.000000000000000000, 0.8660254037844387076, 1.000000000000000000, 0.8660254037844387076, 1.000000000000000000, 0.8660254037844387076, 1.000000000000000000, 0.8660254037844387076, 1.000000000000000000, 0.8660254037844387076, 1.000000000000000000, 0.8660254037844387076, 1.000000000000000000, 0.8660254037844387076, 1.000000000000000000, 0.8660254037844387076, 1.000000000000000000, 0.8660254037844387076, 1.000000000000000000, 0.8660254037844387076, 1.000000000000000000, 0.8660254037844387076, 1.000000000000000000, 0.8660254037844387076, 1.000000000000000000, 0.8660254037844387076, 1.000000000000000000, 0.8660254037844387076, 1.000000000000000000, 0.8660254037844387076, 1.000000000000000000, 0.8660254037844387076, 1.000000000000000000, 0.8660254037844387076, 1.000000000000000000, 0.8660254037844387076, 1.000000000000000000, 0.8660254037844387076, 1.000000000000000000, 0.8660254037844387076, 1.000000000000000000, 0.8660254037844387076, 1.000000000000000000, 0.8660254037844387076, 1.000000000000000000, 0.8660254037844387076, 1.000000000000000000, 0.8660254037844387076, 1.000000000000000000, 0.8660254037844387076, 1.000000000000000000, 0.8660254037844387076, 1.000000000000000000, 0.8660254037844387076, 1.000000000000000000, 0.8660254037844387076, 1.000000000000000000, 0.8660254037844387076, 1.000000000000000000, 0.8660254037844387076, 1.000000000000000000, 0.8660254037844387076, 1.000000000000000000, 0.8660254037844387076, 1.000000000000000000, 0.8660254037844387076, 1.000000000000000000, 0.8660254037844387076, 1.000000000000000000, 0.8660254037844387076, 1.000000000000000000, 0.8660254037844387076, 1.000000000000000000, 0.8660254037844387076, 1.000000000000000000, 0.8660254037844387076, 1.000000000000000000, 0.8660254037844387076, 1.000000000000000000, 0.8660254037844387076, 1.000000000000000000, 0.8660254037844387076, 1.000000000000000000, 0.8660254037844387076, 1.000000000000000000, 0.8660254037844387076, 1.000000000000000000, 0.8660254037844387076, 1.000000000000000000, 0.8660254037844387076, 1.000000000000000000, 0.8660254037844387076, 1.000000000000000000, 0.8660254037844387076, 1.000000000000000000, 0.8660254037844387076, 1.000000000000000000, 0.8660254037844387076, 1.000000000000000000, 0.8660254037844387076, 1.000000000000000000, 0.8660254037844387076, 1.000000000000000000, 0.8660254037844387076, 1.000000000000000000, 0.8660254037844387076, 1.000000000000000000, 0.8660254037844387076, 1.000000000000000000, 0.8660254037844387076, 1.000000000000000000, 0.8660254037844387076, 1.000000000000000000, 0.8660254037844387076, 1.000000000000000000, 0.8660254037844387076, 1.000000000000000000, 0.8660254037844387076, 1.000000000000000000, 0.8660254037844387076, 1.000000000000000000, 0.8660254037844387076, 1.000000000000000000, 0.8660254037844387076, 1.000000000000000000, 0.8660254037844387076, 1.000000000000000000, 0.8660254037844387076, 1.000000000000000000, 0.8660254037844387076, 1.000000000000000000, 0.8660254037844387076, 1.000000000000000000, 0.8660254037844387076, 1.000000000000000000, 0.8660254037844387076, 1.000000000000000000, 0.8660254037844387076, 1.000000000000000000, 0.8660254037844387076, 1.000000000000000000, 0.8660254037844387076, 1.000000000000000000, 0.8660254037844387076, 1.000000000000000000, 0.8660254037844387076, 1.000000000000000000, 0.8660254037844387076, 1.000000000000000000, 0.8660254037844387076, 1.000000000000000000, 0.8660254037844387076, 1.000000000000000000, 0.8660254037844387076, 1.000000000000000000, 0.8660254037844387076, 1.000000000000000000, 0.8660254037844387076, 1.000000000000000000, 0.8660254037844387076, 1.000000000000000000, 0.8660254037844387076, 1.000000000000000000, 0.8660254037844387076, 1.000000000000000000, 0.8660254037844387076, 1.000000000000000000, 0.8660254037844387076, 1.000000000000000000, 0.8660254037844387076, 1.000000000000000000, 0.8660254037844387076, 1.000000000000000000, 0.8660254037844387076, 1.000000000000000000, 0.8660254037844387076, 1.000000000000000000, 0.8660254037844387076, 1.000000000000000000, 0.8660254037844387076, 1.000000000000000000, 0.8660254037844387076, 1.000000000000000000, 0.8660254037844387076, 1.000000000000000000, 0.8660254037844387076, 1.000000000000000000, 0.8660254037844387076, 1.000000000000000000, 0.8660254037844387076, 1.000000000000000000, 0.8660254037844387076, 1.000000000000000000, 0.8660254037844387076, 1.000000000000000000, 0.8660254037844387076, 1.000000000000000000, 0.8660254037844387076, 1.000000000000000000, 0.8660254037844387076, 1.000000000000000000, 0.8660254037844387076, 1.000000000000000000, 0.8660254037844387076, 1.000000000000000000, 0.8660254037844387076, 1.000000000000000000, 0.8660254037844387076, 1.000000000000000000, 0.8660254037844387076, 1.000000000000000000, 0.8660254037844387076, 1.000000000000000000, 0.8660254037844387076, 1.000000000000000000, 0.8660254037844387076, 1.000000000000000000, 0.8660254037844387076, 1.000000000000000000, 0.8660254037844387076, 1.000000000000000000, 0.8660254037844387076, 1.000000000000000000, 0.8660254037844387076, 1.000000000000000000, 0.8660254037844387076, 1.000000000000000000, 0.8660254037844387076, 1.000000000000000000, 0.8660254037844387076, 1.000000000000000000, 0.8660254037844387076, 1.000000000000000000, 0.8660254037844387076, 1.000000000000000000, 0.8660254037844387076, 1.000000000000000000, 0.8660254037844387076, 1.000000000000000000, 0.8660254037844387076, 1.000000000000000000, 0.8660254037844387076, 1.000000000000000000, 0.8660254037844387076, 1.000000000000000000, 0.8660254037844387076, 1.000000000000000000, 0.8660254037844387076, 1.000000000000000000, 0.8660254037844387076, 1.000000000000000000, 0.8660254037844387076, 1.000000000000000000, 0.8660254037844387076, 1.000000000000000000, 0.8660254037844387076, 1.000000000000000000, 0.8660254037844387076, 1.000000000000000000, 0.8660254037844387076, 1.000000000000000000, 0.8660254037844387076, 1.000000000000000000, 0.8660254037844387076, 1.000000000000000000, 0.8660254037844387076, 1.000000000000000000, 0.8660254037844387076, 1.000000000000000000, 0.8660254037844387076, 1.000000000000000000, 0.8660254037844387076, 1.000000000000000000, 0.8660254037844387076, 1.000000000000000000, 0.8660254037844387076, 1.000000000000000000, 0.8660254037844387076, 1.000000000000000000, 0.8660254037844387076, 1.000000000000000000, 0.8660254037844387076, 1.000000000000000000, 0.8660254037844387076, 1.000000000000000000, 0.8660254037844387076, 1.000000000000000000, 0.8660254037844387076, 1.000000000000000000, 0.8660254037844387076, 1.000000000000000000, 0.8660254037844387076, 1.000000000000000000, 0.8660254037844387076, 1.000000000000000000, 0.8660254037844387076, 1.000000000000000000, 0.8660254037844387076, 1.000000000000000000, 0.8660254037844387076, 1.000000000000000000, 0.8660254037844387076, 1.000000000000000000, 0.8660254037844387076, 1.000000000000000000, 0.8660254037844387076, 1.000000000000000000, 0.8660254037844387076, 1.000000000000000000, 0.8660254037844387076, 1.000000000000000000, 0.8660254037844387076, 1.000000000000000000, 0.8660254037844387076, 1.000000000000000000, 0.8660254037844387076, 1.000000000000000000, 0.8660254037844387076, 1.000000000000000000, 0.8660254037844387076, 1.000000000000000000, 0.8660254037844387076, 1.000000000000000000, 0.8660254037844387076, 1.000000000000000000, 0.8660254037844387076, 1.000000000000000000, 0.8660254037844387076, 1.000000000000000000, 0.8660254037844387076, 1.000000000000000000, 0.8660254037844387076, 1.000000000000000000, 0.8660254037844387076, 1.000000000000000000, 0.8660254037844387076, 1.000000000000000000, 0.8660254037844387076, 1.000000000000000000, 0.8660254037844387076, 1.000000000000000000, 0.8660254037844387076, 1.000000000000000000, 0.8660254037844387076, 1.000000000000000000, 0.8660254037844387076, 1.000000000000000000, 0.8660254037844387076, 1.000000000000000000, 0.8660254037844387076, 1.000000000000000000, 0.8660254037844387076, 1.000000000000000000, 0.8660254037844387076, 1.000000000000000000, 0.8660254037844387076, 1.000000000000000000, 0.8660254037844387076, 1.000000000000000000, 0.8660254037844387076, 1.000000000000000000, 0.8660254037844387076, 1.000000000000000000, 0.8660254037844387076, 1.000000000000000000, 0.8660254037844387076, 1.000000000000000000, 0.8660254037844387076, 1.000000000000000000, 0.8660254037844387076, 1.000000000000000000, 0.8660254037844387076, 1.000000000000000000, 0.8660254037844387076, 1.000000000000000000, 0.8660254037844387076, 1.000000000000000000, 0.8660254037844387076, 1.000000000000000000, 0.8660254037844387076, 1.000000000000000000, 0.8660254037844387076, 1.000000000000000000, 0.8660254037844387076, 1.000000000000000000, 0.8660254037844387076, 1.000000000000000000, 0.8660254037844387076, 1.000000000000000000, 0.8660254037844387076, 1.000000000000000000, 0.8660254037844387076, 1.000000000000000000, 0.8660254037844387076, 1.000000000000000000, 0.8660254037844387076, 1.000000000000000000, 0.8660254037844387076, 1.000000000000000000, 0.8660254037844387076, 1.000000000000000000, 0.8660254037844387076, 1.000000000000000000, 0.8660254037844387076, 1.000000000000000000, 0.8660254037844387076, 1.000000000000000000, 0.8660254037844387076, 1.000000000000000000, 0.8660254037844387076, 1.000000000000000000, 0.8660254037844387076, 1.000000000000000000, 0.8660254037844387076, 1.000000000000000000, 0.8660254037844387076, 1.000000000000000000, 0.8660254037844387076, 1.000000000000000000, 0.8660254037844387076, 1.000000000000000000, 0.8660254037844387076, 1.000000000000000000, 0.8660254037844387076, 1.000000000000000000, 0.8660254037844387076, 1.000000000000000000, 0.8660254037844387076, 1.000000000000000000, 0.8660254037844387076, 1.000000000000000000, 0.8660254037844387076, 1.000000000000000000, 0.8660254037844387076, 1.000000000000000000, 0.8660254037844387076, 1.000000000000000000, 0.8660254037844387076, 1.000000000000000000, 0.8660254037844387076, 1.000000000000000000, 0.8660254037844387076, 1.000000000000000000, 0.8660254037844387076, 1.000000000000000000, 0.8660254037844387076, 1.000000000000000000, 0.8660254037844387076, 1.000000000000000000, 0.8660254037844387076, 1.000000000000000000, 0.8660254037844387076, 1.000000000000000000, 0.8660254037844387076, 1.000000000000000000, 0.8660254037844387076, 1.000000000000000000, 0.8660254037844387076, 1.000000000000000000, 0.8660254037844387076, 1.000000000000000000, 0.8660254037844387076, 1.000000000000000000, 0.8660254037844387076, 1.000000000000000000, 0.8660254037844387076, 1.000000000000000000, 0.8660254037844387076, 1.000000000000000000, 0.8660254037844387076, 1.000000000000000000, 0.8660254037844387076, 1.000000000000000000, 0.8660254037844387076, 1.000000000000000000, 0.8660254037844387076, 1.000000000000000000, 0.8660254037844387076, 1.000000000000000000, 0.8660254037844387076, 1.000000000000000000, 0.8660254037844387076, 1.000000000000000000, 0.8660254037844387076, 1.000000000000000000, 0.8660254037844387076, 1.000000000000000000, 0.8660254037844387076, 1.000000000000000000, 0.8660254037844387076, 1.000000000000000000, 0.8660254037844387076, 1.000000000000000000, 0.8660254037844387076, 1.000000000000000000, 0.8660254037844387076, 1.000000000000000000, 0.8660254037844387076, 1.000000000000000000, 0.8660254037844387076, 1.000000000000000000, 0.8660254037844387076, 1.000000000000000000, 0.8660254037844387076, 1.000000000000000000, 0.8660254037844387076, 1.000000000000000000, 0.8660254037844387076, 1.000000000000000000, 0.8660254037844387076, 1.000000000000000000, 0.8660254037844387076, 1.000000000000000000, 0.8660254037844387076, 1.000000000000000000, 0.8660254037844387076, 1.000000000000000000, 0.8660254037844387076, 1.000000000000000000, 0.8660254037844387076, 1.000000000000000000, 0.8660254037844387076, 1.000000000000000000, 0.8660254037844387076, 1.000000000000000000, 0.8660254037844387076, 1.000000000000000000, 0.8660254037844387076, 1.000000000000000000, 0.8660254037844387076, 1.000000000000000000, 0.8660254037844387076, 1.000000000000000000, 0.8660254037844387076, 1.000000000000000000, 0.8660254037844387076, 1.000000000000000000, 0.8660254037844387076, 1.000000000000000000, 0.8660254037844387076, 1.000000000000000000, 0.8660254037844387076, 1.000000000000000000, 0.8660254037844387076, 1.000000000000000000, 0.8660254037844387076, 1.000000000000000000, 0.8660254037844387076, 1.000000000000000000, 0.8660254037844387076, 1.000000000000000000, 0.8660254037844387076, 1.000000000000000000, 0.8660254037844387076, 1.000000000000000000, 0.8660254037844387076, 1.000000000000000000, 0.8660254037844387076, 1.000000000000000000, 0.8660254037844387076, 1.000000000000000000, 0.8660254037844387076, 1.000000000000000000, 0.8660254037844387076, 1.000000000000000000, 0.8660254037844387076, 1.000000000000000000, 0.8660254037844387076, 1.000000000000000000, 0.8660254037844387076, 1.000000000000000000, 0.8660254037844387076, 1.000000000000000000, 0.8660254037844387076, 1.000000000000000000, 0.8660254037844387076, 1.000000000000000000, 0.8660254037844387076, 1.000000000000000000, 0.8660254037844387076, 1.000000000000000000, 0.8660254037844387076, 1.000000000000000000, 0.8660254037844387076, 1.000000000000000000, 0.8660254037844387076, 1.000000000000000000, 0.8660254037844387076, 1.000000000000000000, 0.8660254037844387076, 1.000000000000000000, 0.8660254037844387076, 1.000000000000000000, 0.8660254037844387076, 1.000000000000000000, 0.8660254037844387076, 1.000000000000000000, 0.8660254037844387076, 1.000000000000000000, 0.8660254037844387076, 1.000000000000000000, 0.8660254037844387076, 1.000000000000000000, 0.8660254037844387076, 1.000000000000000000, 0.8660254037844387076, 1.000000000000000000, 0.8660254037844387076, 1.000000000000000000, 0.8660254037844387076, 1.000000000000000000, 0.8660254037844387076, 1.000000000000000000, 0.8660254037844387076, 1.000000000000000000, 0.8660254037844387076, 1.000000000000000000, 0.8660254037844387076, 1.000000000000000000, 0.8660254037844387076, 1.000000000000000000, 0.8660254037844387076, 1.000000000000000000, 0.8660254037844387076, 1.000000000000000000, 0.8660254037844387076, 1.000000000000000000, 0.8660254037844387076, 1.000000000000000000, 0.8660254037844387076, 1.000000000000000000, 0.8660254037844387076, 1.000000000000000000, 0.8660254037844387076, 1.000000000000000000, 0.8660254037844387076, 1.000000000000000000, 0.8660254037844387076, 1.000000000000000000, 0.8660254037844387076, 1.000000000000000000, 0.8660254037844387076, 1.000000000000000000, 0.8660254037844387076, 1.000000000000000000, 0.8660254037844387076, 1.000000000000000000, 0.8660254037844387076, 1.000000000000000000, 0.8660254037844387076, 1.000000000000000000, 0.8660254037844387076, 1.000000000000000000, 0.8660254037844387076, 1.000000000000000000, 0.8660254037844387076, 1.000000000000000000, 0.8660254037844387076, 1.000000000000000000, 0.8660254037844387076, 1.000000000000000000, 0.8660254037844387076, 1.000000000000000000, 0.8660254037844387076, 1.000000000000000000, 0.8660254037844387076, 1.000000000000000000, 0.8660254037844387076, 1.000000000000000000, 0.8660254037844387076, 1.000000000000000000, 0.8660254037844387076, 1.000000000000000000, 0.8660254037844387076, 1.000000000000000000, 0.8660254037844387076, 1.000000000000000000, 0.8660254037844387076, 1.000000000000000000, 0.8660254037844387076, 1.000000000000000000, 0.8660254037844387076, 1.000000000000000000, 0.8660254037844387076, 1.000000000000000000, 0.8660254037844387076, 1.000000000000000000, 0.8660254037844387076, 1.000000000000000000, 0.8660254037844387076, 1.000000000000000000, 0.8660254037844387076, 1.000000000000000000, 0.8660254037844387076, 1.000000000000000000, 0.8660254037844387076, 1.000000000000000000, 0.8660254037844387076, 1.000000000000000000, 0.8660254037844387076, 1.000000000000000000, 0.8660254037844387076, 1.000000000000000000, 0.8660254037844387076, 1.000000000000000000, 0.8660254037844387076, 1.000000000000000000, 0.8660254037844387076, 1.000000000000000000, 0.8660254037844387076, 1.000000000000000000, 0.8660254037844387076, 1.000000000000000000, 0.8660254037844387076, 1.000000000000000000, 0.8660254037844387076, 1.000000000000000000, 0.8660254037844387076, 1.000000000000000000, 0.8660254037844387076, 1.000000000000000000, 0.8660254037844387076, 1.000000000000000000, 0.8660254037844387076, 1.000000000000000000, 0.8660254037844387076, 1.000000000000000000, 0.8660254037844387076, 1.000000000000000000, 0.8660254037844387076, 1.000000000000000000, 0.8660254037844387076, 1.000000000000000000, 0.8660254037844387076, 1.000000000000000000, 0.8660254037844387076, 1.000000000000000000, 0.8660254037844387076, 1.000000000000000000, 0.8660254037844387076, 1.000000000000000000, 0.8660254037844387076, 1.000000000000000000, 0.8660254037844387076, 1.000000000000000000, 0.8660254037844387076, 1.000000000000000000, 0.8660254037844387076, 1.000000000000000000, 0.8660254037844387076, 1.000000000000000000, 0.8660254037844387076, 1.000000000000000000, 0.8660254037844387076, 1.000000000000000000, 0.8660254037844387076, 1.000000000000000000, 0.8660254037844387076, 1.000000000000000000, 0.8660254037844387076, 1.000000000000000000, 0.8660254037844387076, 1.000000000000000000, 0.8660254037844387076, 1.000000000000000000, 0.8660254037844387076, 1.000000000000000000, 0.8660254037844387076, 1.000000000000000000, 0.8660254037844387076, 1.000000000000000000, 0.8660254037844387076, 1.000000000000000000, 0.8660254037844387076, 1.000000000000000000, 0.8660254037844387076, 1.000000000000000000, 0.8660254037844387076, 1.000000000000000000, 0.8660254037844387076, 1.000000000000000000, 0.8660254037844387076, 1.000000000000000000, 0.8660254037844387076, 1.000000000000000000, 0.8660254037844387076, 1.000000000000000000, 0.8660254037844387076, 1.000000000000000000, 0.8660254037844387076, 1.000000000000000000, 0.8660254037844387076, 1.000000000000000000, 0.8660254037844387076, 1.000000000000000000, 0.8660254037844387076, 1.000000000000000000, 0.8660254037844387076, 1.000000000000000000, 0.8660254037844387076, 1.000000000000000000, 0.8660254037844387076, 1.000000000000000000, 0.8660254037844387076, 1.000000000000000000, 0.8660254037844387076, 1.000000000000000000, 0.8660254037844387076, 1.000000000000000000, 0.8660254037844387076, 1.000000000000000000, 0.8660254037844387076, 1.000000000000000000, 0.8660254037844387076, 1.000000000000000000, 0.8660254037844387076, 1.000000000000000000, 0.8660254037844387076, 1.000000000000000000, 0.8660254037844387076, 1.000000000000000000, 0.8660254037844387076, 1.000000000000000000, 0.8660254037844387076, 1.000000000000000000, 0.8660254037844387076, 1.000000000000000000, 0.8660254037844387076, 1.000000000000000000, 0.8660254037844387076, 1.000000000000000000, 0.8660254037844387076, 1.000000000000000000, 0.8660254037844387076, 1.000000000000000000, 0.8660254037844387076, 1.000000000000000000, 0.8660254037844387076, 1.000000000000000000, 0.8660254037844387076, 1.000000000000000000, 0.8660254037844387076, 1.000000000000000000, 0.8660254037844387076, 1.000000000000000000, 0.8660254037844387076, 1.000000000000000000, 0.8660254037844387076, 1.000000000000000000, 0.8660254037844387076, 1.000000000000000000, 0.8660254037844387076, 1.000000000000000000, 0.8660254037844387076, 1.000000000000000000, 0.8660254037844387076, 1.000000000000000000, 0.8660254037844387076, 1.000000000000000000, 0.8660254037844387076, 1.000000000000000000, 0.8660254037844387076, 1.000000000000000000, 0.8660254037844387076, 1.000000000000000000, 0.8660254037844387076, 1.000000000000000000, 0.8660254037844387076, 1.000000000000000000, 0.8660254037844387076, 1.000000000000000000, 0.8660254037844387076, 1.000000000000000000, 0.8660254037844387076, 1.000000000000000000, 0.8660254037844387076, 1.000000000000000000, 0.8660254037844387076, 1.000000000000000000, 0.8660254037844387076, 1.000000000000000000, 0.8660254037844387076, 1.000000000000000000, 0.8660254037844387076, 1.000000000000000000, 0.8660254037844387076, 1.000000000000000000, 0.8660254037844387076, 1.000000000000000000, 0.8660254037844387076, 1.000000000000000000, 0.8660254037844387076, 1.000000000000000000, 0.8660254037844387076, 1.000000000000000000, 0.8660254037844387076, 1.000000000000000000, 0.8660254037844387076, 1.000000000000000000, 0.8660254037844387076, 1.000000000000000000, 0.8660254037844387076, 1.000000000000000000, 0.8660254037844387076, 1.000000000000000000, 0.8660254037844387076, 1.000000000000000000, 0.8660254037844387076, 1.000000000000000000, 0.8660254037844387076, 1.000000000000000000, 0.8660254037844387076, 1.000000000000000000, 0.8660254037844387076, 1.000000000000000000, 0.8660254037844387076, 1.000000000000000000, 0.8660254037844387076, 1.000000000000000000, 0.8660254037844387076, 1.000000000000000000, 0.8660254037844387076, 1.000000000000000000, 0.8660254037844387076, 1.000000000000000000, 0.8660254037844387076, 1.000000000000000000, 0.8660254037844387076, 1.000000000000000000, 0.8660254037844387076, 1.000000000000000000, 0.8660254037844387076, 1.000000000000000000, 0.8660254037844387076, 1.000000000000000000, 0.8660254037844387076, 1.000000000000000000, 0.8660254037844387076, 1.000000000000000000, 0.8660254037844387076, 1.000000000000000000, 0.8660254037844387076, 1.000000000000000000, 0.8660254037844387076, 1.000000000000000000, 0.8660254037844387076, 1.000000000000000000, 0.8660254037844387076, 1.000000000000000000, 0.8660254037844387076, 1.000000000000000000, 0.8660254037844387076, 1.000000000000000000, 0.8660254037844387076, 1.000000000000000000, 0.8660254037844387076, 1.000000000000000000, 0.8660254037844387076, 1.000000000000000000, 0.8660254037844387076, 1.000000000000000000, 0.8660254037844387076, 1.000000000000000000, 0.8660254037844387076, 1.000000000000000000, 0.8660254037844387076, 1.000000000000000000, 0.8660254037844387076, 1.000000000000000000, 0.8660254037844387076, 1.000000000000000000, 0.8660254037844387076, 1.000000000000000000, 0.8660254037844387076, 1.000000000000000000, 0.8660254037844387076, 1.000000000000000000, 0.8660254037844387076, 1.000000000000000000, 0.8660254037844387076, 1.000000000000000000, 0.8660254037844387076, 1.000000000000000000, 0.8660254037844387076, 1.000000000000000000, 0.8660254037844387076, 1.000000000000000000, 0.8660254037844387076, 1.000000000000000000, 0.8660254037844387076, 1.000000000000000000, 0.8660254037844387076, 1.000000000000000000, 0.8660254037844387076, 1.000000000000000000, 0.8660254037844387076, 1.000000000000000000, 0.8660254037844387076, 1.000000000000000000, 0.8660254037844387076, 1.000000000000000000, 0.8660254037844387076, 1.000000000000000000, 0.8660254037844387076, 1.000000000000000000, 0.8660254037844387076, 1.000000000000000000, 0.8660254037844387076, 1.000000000000000000, 0.8660254037844387076, 1.000000000000000000, 0.8660254037844387076, 1.000000000000000000, 0.8660254037844387076, 1.000000000000000000, 0.8660254037844387076, 1.000000000000000000, 0.8660254037844387076, 1.000000000000000000, 0.8660254037844387076, 1.000000000000000000, 0.8660254037844387076, 1.000000000000000000, 0.8660254037844387076, 1.000000000000000000, 0.8660254037844387076, 1.000000000000000000, 0.8660254037844387076, 1.000000000000000000, 0.8660254037844387076, 1.000000000000000000, 0.8660254037844387076, 1.000000000000000000, 0.8660254037844387076, 1.000000000000000000, 0.8660254037844387076, 1.000000000000000000, 0.8660254037844387076, 1.000000000000000000, 0.8660254037844387076, 1.000000000000000000, 0.8660254037844387076, 1.000000000000000000, 0.8660254037844387076, 1.000000000000000000, 0.8660254037844387076, 1.000000000000000000, 0.8660254037844387076, 1.000000000000000000, 0.8660254037844387076, 1.000000000000000000, 0.8660254037844387076, 1.000000000000000000, 0.8660254037844387076, 1.000000000000000000, 0.8660254037844387076, 1.000000000000000000, 0.8660254037844387076, 1.000000000000000000, 0.8660254037844387076, 1.000000000000000000, 0.8660254037844387076, 1.000000000000000000, 0.8660254037844387076, 1.000000000000000000, 0.8660254037844387076, 1.000000000000000000, 0.8660254037844387076, 1.000000000000000000, 0.8660254037844387076, 1.000000000000000000, 0.8660254037844387076, 1.000000000000000000, 0.8660254037844387076, 1.000000000000000000, 0.8660254037844387076, 1.000000000000000000, 0.8660254037844387076, 1.000000000000000000, 0.8660254037844387076, 1.000000000000000000, 0.8660254037844387076, 1.000000000000000000, 0.8660254037844387076, 1.000000000000000000, 0.8660254037844387076, 1.000000000000000000, 0.8660254037844387076, 1.000000000000000000, 0.8660254037844387076, 1.000000000000000000, 0.8660254037844387076, 1.000000000000000000, 0.8660254037844387076, 1.000000000000000000, 0.8660254037844387076, 1.000000000000000000, 0.8660254037844387076, 1.000000000000000000, 0.8660254037844387076, 1.000000000000000000, 0.8660254037844387076, 1.000000000000000000, 0.8660254037844387076, 1.000000000000000000, 0.8660254037844387076, 1.000000000000000000, 0.8660254037844387076, 1.000000000000000000, 0.8660254037844387076, 1.000000000000000000, 0.8660254037844387076, 1.000000000000000000, 0.8660254037844387076, 1.000000000000000000, 0.8660254037844387076, 1.000000000000000000, 0.8660254037844387076, 1.000000000000000000, 0.8660254037844387076, 1.000000000000000000, 0.8660254037844387076, 1.000000000000000000, 0.8660254037844387076, 1.000000000000000000, 0.8660254037844387076, 1.000000000000000000, 0.8660254037844387076, 1.000000000000000000, 0.8660254037844387076, 1.000000000000000000, 0.8660254037844387076, 1.000000000000000000, 0.8660254037844387076, 1.000000000000000000, 0.8660254037844387076, 1.000000000000000000, 0.8660254037844387076, 1.000000000000000000, 0.8660254037844387076, 1.000000000000000000, 0.8660254037844387076, 1.000000000000000000, 0.8660254037844387076, 1.000000000000000000, 0.8660254037844387076, 1.000000000000000000, 0.8660254037844387076, 1.000000000000000000, 0.8660254037844387076, 1.000000000000000000, 0.8660254037844387076, 1.000000000000000000, 0.8660254037844387076, 1.000000000000000000, 0.8660254037844387076, 1.000000000000000000, 0.8660254037844387076, 1.000000000000000000, 0.8660254037844387076, 1.000000000000000000, 0.8660254037844387076, 1.000000000000000000, 0.8660254037844387076, 1.000000000000000000) ) ) 
 REPRESENTATION_ITEM ( '' )  SURFACE ( )  );
#30818=CARTESIAN_POINT ( 'NONE',  ( -4.999999999999996447, 8.660254037844387298, -79.87500000409677625 ) ) ;
#30819=CARTESIAN_POINT ( 'NONE',  ( 9.999999999999998224, 0.000000000000000000, -119.0000000000000000 ) ) ;
#30820=CARTESIAN_POINT ( 'NONE',  ( 5.405949406249999534, 9.363379034771803333, -37.09375000204836681 ) ) ;
#30821=EDGE_LOOP ( 'NONE', ( #27201, #6775, #8335, #30874 ) ) ;
#30823=CARTESIAN_POINT ( 'NONE',  ( -10.81189881249999729, 1.324075727343319199E-15, -30.78125000204837036 ) ) ;
#30826=CARTESIAN_POINT ( 'NONE',  ( -9.999999999999998224, 5.773502691896259087, -0.2500000040967509385 ) ) ;
#30829=CARTESIAN_POINT ( 'NONE',  ( -4.999999999999996447, 8.660254037844387298, -120.0000000000000000 ) ) ;
#30831=VERTEX_POINT ( 'NONE', #32650 ) ;
#30839=DIRECTION ( 'NONE',  ( -0.000000000000000000, -0.000000000000000000, -1.000000000000000000 ) ) ;
#30841=CARTESIAN_POINT ( 'NONE',  ( 9.999999999999998224, 0.000000000000000000, -105.8750000040967763 ) ) ;
#30842=CARTESIAN_POINT ( 'NONE',  ( -10.81189881249999729, 6.242252689847871849, -174.9062500020483810 ) ) ;
#30845=CARTESIAN_POINT ( 'NONE',  ( 5.405949406249999534, 9.363379034771803333, -95.59375000204838102 ) ) ;
#30848=CARTESIAN_POINT ( 'NONE',  ( 7.644554776091147741E-16, 12.48450537969573659, -101.6562500020483952 ) ) ;
#30850=CARTESIAN_POINT ( 'NONE',  ( 10.81189881249999729, 6.242252689847867408, -104.7187500020483810 ) ) ;
#30852=EDGE_CURVE ( 'NONE', #11384, #26823, #12762, .T. ) ;
#30853=CARTESIAN_POINT ( 'NONE',  ( 10.81189881249999907, 6.242252689847868297, -199.4062500020484094 ) ) ;
#30856=CARTESIAN_POINT ( 'NONE',  ( -10.00000000000000000, -5.773502691896251982, -169.5000000040967620 ) ) ;
#30858=CARTESIAN_POINT ( 'NONE',  ( 7.644554776091147741E-16, 12.48450537969573659, -20.46875000204837036 ) ) ;
#30860=CARTESIAN_POINT ( 'NONE',  ( 10.81189881249999907, 6.242252689847868297, -127.2187500020483668 ) ) ;
#30862=CARTESIAN_POINT ( 'NONE',  ( -2.293366432827344421E-15, -12.48450537969573659, -30.40625000204835615 ) ) ;
#30865=CARTESIAN_POINT ( 'NONE',  ( -10.00000000000000000, -5.773502691896251982, -62.62499999999997868 ) ) ;
#30866=CARTESIAN_POINT ( 'NONE',  ( 10.81189881249999729, 0.000000000000000000, -123.0312500020483952 ) ) ;
#30869=CARTESIAN_POINT ( 'NONE',  ( -9.999999999999998224, 1.224646799147353059E-15, -118.2500000000000000 ) ) ;
#30870=CARTESIAN_POINT ( 'NONE',  ( 9.999999999999996447, -5.773502691896262640, -98.50000000409677625 ) ) ;
#30873=CARTESIAN_POINT ( 'NONE',  ( -5.405949406249996869, 9.363379034771805109, -60.84375000204836681 ) ) ;
#30874=ORIENTED_EDGE ( 'NONE', *, *, #18202, .F. ) ;
#30881=CARTESIAN_POINT ( 'NONE',  ( -5.000000000000003553, -8.660254037844383745, -25.37500000409675849 ) ) ;
#30887=ORIENTED_EDGE ( 'NONE', *, *, #11956, .T. ) ;
#30891=CARTESIAN_POINT ( 'NONE',  ( -5.405949406249996869, 9.363379034771805109, -194.5312500020484094 ) ) ;
#30894=AXIS2_PLACEMENT_3D ( 'NONE', #18678, #2714, #32290 ) ;
#30900=CARTESIAN_POINT ( 'NONE',  ( -10.81189881249999729, 1.324075727343319199E-15, -114.5937500020483810 ) ) ;
#30901=CARTESIAN_POINT ( 'NONE',  ( -10.00000000000000000, -5.773502691896251982, -195.0000000040967905 ) ) ;
#30902=CARTESIAN_POINT ( 'NONE',  ( -10.81189881249999907, -6.242252689847864744, -126.6562500020483810 ) ) ;
#30904=CARTESIAN_POINT ( 'NONE',  ( -10.81189881249999729, 1.324075727343319199E-15, -129.5937500020483810 ) ) ;
#30907=CARTESIAN_POINT ( 'NONE',  ( 10.00000000000000000, 5.773502691896255534, -145.8750000000000284 ) ) ;
#30908=CARTESIAN_POINT ( 'NONE',  ( 9.999999999999998224, 0.000000000000000000, -24.49999999999996447 ) ) ;
#30913=CARTESIAN_POINT ( 'NONE',  ( 7.644554776091147741E-16, 12.48450537969573659, -44.46875000204836681 ) ) ;
#30914=CARTESIAN_POINT ( 'NONE',  ( -9.999999999999998224, 1.224646799147353059E-15, -151.2500000000000000 ) ) ;
#30915=CARTESIAN_POINT ( 'NONE',  ( -10.81189881249999907, -6.242252689847864744, -157.9687500020484379 ) ) ;
#30918=CARTESIAN_POINT ( 'NONE',  ( 4.366535267995796055, 9.446561771012207842, -179.9999999999999147 ) ) ;
#30919=CARTESIAN_POINT ( 'NONE',  ( -2.121150477449813534E-15, -11.54700538379251284, -80.37499999999997158 ) ) ;
#30922=CARTESIAN_POINT ( 'NONE',  ( 5.405949406249992428, -9.363379034771808662, -102.2812500020483952 ) ) ;
#30923=CARTESIAN_POINT ( 'NONE',  ( -5.000000000000003553, -8.660254037844383745, -121.3750000040967905 ) ) ;
#30927=CARTESIAN_POINT ( 'NONE',  ( -2.293366432827344421E-15, -12.48450537969573659, -45.40625000204837391 ) ) ;
#30932=AXIS2_PLACEMENT_3D ( 'NONE', #31352, #4789, #1782 ) ;
#30936=ORIENTED_EDGE ( 'NONE', *, *, #18251, .T. ) ;
#30939=ORIENTED_EDGE ( 'NONE', *, *, #11435, .T. ) ;
#30941=EDGE_CURVE ( 'NONE', #33014, #30027, #4938, .T. ) ;
#30952=CARTESIAN_POINT ( 'NONE',  ( 10.81189881249999551, -6.242252689847874514, -143.9687500020483810 ) ) ;
#30953=CARTESIAN_POINT ( 'NONE',  ( -2.293366432827344421E-15, -12.48450537969573659, -151.9062500020483810 ) ) ;
#30954=CARTESIAN_POINT ( 'NONE',  ( -10.81189881249999729, 6.242252689847871849, -155.2187500020483810 ) ) ;
#30957=CARTESIAN_POINT ( 'NONE',  ( -10.00000000000051337, 5.773502691895962435, -102.2500000040967905 ) ) ;
#30958=CARTESIAN_POINT ( 'NONE',  ( -5.000000000000003553, -8.660254037844383745, -179.5000000000000000 ) ) ;
#30963=CARTESIAN_POINT ( 'NONE',  ( -2.293366432827344421E-15, -12.48450537969573659, -178.7187500020484094 ) ) ;
#30968=CYLINDRICAL_SURFACE ( 'NONE', #13044, 9.999999999999998224 ) ;
#30969=CARTESIAN_POINT ( 'NONE',  ( 7.644554776091147741E-16, 12.48450537969573659, -44.65625000204836681 ) ) ;
#30971=CARTESIAN_POINT ( 'NONE',  ( -9.999999999999998224, 1.224646799147353059E-15, -107.7499999999999858 ) ) ;
#30972=VERTEX_POINT ( 'NONE', #16847 ) ;
#30973=CARTESIAN_POINT ( 'NONE',  ( 10.81189881249999729, 6.242252689847867408, -127.4062500020483810 ) ) ;
#30974=CARTESIAN_POINT ( 'NONE',  ( -10.00000000000000000, -5.773502691896251982, -147.0000000040967905 ) ) ;
#30980=CARTESIAN_POINT ( 'NONE',  ( 5.405949406249999534, 9.363379034771803333, -175.0937500020484094 ) ) ;
#30982=EDGE_CURVE ( 'NONE', #17741, #28218, #26027, .T. ) ;
#30983=CARTESIAN_POINT ( 'NONE',  ( -31.99999999999997158, 3.918869757271527108E-15, -180.0000000000000000 ) ) ;
#30985=CARTESIAN_POINT ( 'NONE',  ( 10.81189881249999729, 0.000000000000000000, -64.53125000204836681 ) ) ;
#30987=CARTESIAN_POINT ( 'NONE',  ( 10.00000000000000000, 5.773502691896255534, -53.25000000409676915 ) ) ;
#30989=CARTESIAN_POINT ( 'NONE',  ( 10.81189881249999729, 0.000000000000000000, -4.343750002048368586 ) ) ;
#30996=DIRECTION ( 'NONE',  ( -0.000000000000000000, -0.000000000000000000, -1.000000000000000000 ) ) ;
#30998=ORIENTED_EDGE ( 'NONE', *, *, #25847, .T. ) ;
#31008=CARTESIAN_POINT ( 'NONE',  ( 7.070501591499377789E-16, 11.54700538379251284, -45.12499999999997158 ) ) ;
#31010=CARTESIAN_POINT ( 'NONE',  ( -10.81189881249999907, -6.242252689847864744, -162.4687500020483526 ) ) ;
#31011=CARTESIAN_POINT ( 'NONE',  ( -5.405949406250003975, -9.363379034771801557, -177.3437500020483810 ) ) ;
#31012=CARTESIAN_POINT ( 'NONE',  ( 9.999999999999998224, 1.224646799147353059E-15, -99.99999999999998579 ) ) ;
#31020=CARTESIAN_POINT ( 'NONE',  ( 5.405949406249992428, -9.363379034771808662, -60.09375000204835970 ) ) ;
#31021=CARTESIAN_POINT ( 'NONE',  ( -10.81189881249999907, -6.242252689847864744, -69.65625000204839523 ) ) ;
#31023=CARTESIAN_POINT ( 'NONE',  ( 9.999999999999998224, 0.000000000000000000, -134.0000000000000000 ) ) ;
#31025=CARTESIAN_POINT ( 'NONE',  ( -10.81189881249999729, -6.242252689847864744, -149.1562500020484094 ) ) ;
#31026=CARTESIAN_POINT ( 'NONE',  ( 10.81189881249999907, 6.242252689847868297, -167.9062500020484094 ) ) ;
#31028=CARTESIAN_POINT ( 'NONE',  ( -9.999999999999998224, 1.224646799147353059E-15, -159.1250000040967905 ) ) ;
#31029=CARTESIAN_POINT ( 'NONE',  ( -10.81189881249999729, 6.242252689847871849, -101.2187500020483810 ) ) ;
#31031=CARTESIAN_POINT ( 'NONE',  ( 10.81189881249999729, 0.000000000000000000, -6.031250002048377468 ) ) ;
#31035=CARTESIAN_POINT ( 'NONE',  ( -5.405949406249996869, 9.363379034771805109, -100.0312500020483952 ) ) ;
#31037=CARTESIAN_POINT ( 'NONE',  ( -9.999999999999998224, 5.773502691896259087, -79.75000000409677625 ) ) ;
#31039=CARTESIAN_POINT ( 'NONE',  ( -10.81189881249999907, -6.242252689847864744, -33.46875000204835260 ) ) ;
#31043=CARTESIAN_POINT ( 'NONE',  ( -10.81189881249999907, -6.242252689847864744, -27.65625000204838457 ) ) ;
#31046=CARTESIAN_POINT ( 'NONE',  ( 7.070501591499377789E-16, 11.54700538379251284, -6.500000004096756712 ) ) ;
#31052=CYLINDRICAL_SURFACE ( 'NONE', #26215, 9.999999999999998224 ) ;
#31058=CARTESIAN_POINT ( 'NONE',  ( -9.999999999999998224, 0.000000000000000000, -99.99999999999998579 ) ) ;
#31059=CARTESIAN_POINT ( 'NONE',  ( 10.00000000000076916, -5.773502691895816774, -108.6249999999999858 ) ) ;
#31060=CARTESIAN_POINT ( 'NONE',  ( 10.81189881249999907, 6.242252689847868297, -164.9062500020484094 ) ) ;
#31063=EDGE_CURVE ( 'NONE', #15993, #4202, #11125, .T. ) ;
#31065=CARTESIAN_POINT ( 'NONE',  ( -10.81189881249999907, -6.242252689847864744, -85.96875000204836681 ) ) ;
#31067=CARTESIAN_POINT ( 'NONE',  ( 10.81189881249999551, -6.242252689847874514, -194.9687500020484094 ) ) ;
#31068=CARTESIAN_POINT ( 'NONE',  ( -5.405949406250003975, -9.363379034771801557, -89.03125000204838102 ) ) ;
#31070=CARTESIAN_POINT ( 'NONE',  ( 5.405949406249992428, -9.363379034771808662, -106.5937500020483810 ) ) ;
#31072=( BOUNDED_CURVE ( )  B_SPLINE_CURVE ( 2, ( #22288, #15780, #42116, #28343, #21640, #35459, #5884 ),
 .UNSPECIFIED., .F., .F. ) 
 B_SPLINE_CURVE_WITH_KNOTS ( ( 3, 2, 2, 3 ),
 ( 0.1679104477611940427, 0.1691542288557214002, 0.1703980099502487855, 0.1716417910447761430 ),
 .UNSPECIFIED. ) 
 CURVE ( )  GEOMETRIC_REPRESENTATION_ITEM ( )  RATIONAL_B_SPLINE_CURVE ( ( 1.000000000000000000, 0.8660254037844387076, 1.000000000000000000, 0.8660254037844387076, 1.000000000000000000, 0.8660254037844357100, 1.000000000000003109 ) ) 
 REPRESENTATION_ITEM ( '' )  );
#31074=CARTESIAN_POINT ( 'NONE',  ( 10.00000000000038369, -5.773502691896038819, -152.5000000040967620 ) ) ;
#31075=CARTESIAN_POINT ( 'NONE',  ( -10.81189881249999729, 6.242252689847871849, -198.9062500020484094 ) ) ;
#31077=CARTESIAN_POINT ( 'NONE',  ( 9.999999999999996447, -5.773502691896262640, -169.0000000040967905 ) ) ;
#31079=CARTESIAN_POINT ( 'NONE',  ( -10.81189881249999729, 6.242252689847871849, -20.21875000204836681 ) ) ;
#31081=CARTESIAN_POINT ( 'NONE',  ( 10.81189881249999551, -6.242252689847874514, -130.4687500020483810 ) ) ;
#31083=CARTESIAN_POINT ( 'NONE',  ( 10.81189881249999907, 6.242252689847868297, -25.40625000204838102 ) ) ;
#31086=CARTESIAN_POINT ( 'NONE',  ( -2.121150477449813534E-15, -11.54700538379251284, -48.87499999999997868 ) ) ;
#31087=CARTESIAN_POINT ( 'NONE',  ( 5.405949406249999534, 9.363379034771803333, -121.2812500020483952 ) ) ;
#31089=EDGE_CURVE ( 'NONE', #17480, #9895, #34516, .T. ) ;
#31091=CARTESIAN_POINT ( 'NONE',  ( 9.999999999999998224, 0.000000000000000000, -102.8750000040967763 ) ) ;
#31094=CARTESIAN_POINT ( 'NONE',  ( -10.81189881249999907, -6.242252689847864744, -54.46875000204836681 ) ) ;
#31095=ORIENTED_EDGE ( 'NONE', *, *, #32284, .F. ) ;
#31100=CARTESIAN_POINT ( 'NONE',  ( -10.00000000000000000, -5.773502691896251982, -30.00000000409674783 ) ) ;
#31105=CARTESIAN_POINT ( 'NONE',  ( 0.000000000000000000, 0.000000000000000000, -99.99999999999998579 ) ) ;
#31109=ORIENTED_EDGE ( 'NONE', *, *, #18814, .F. ) ;
#31110=CARTESIAN_POINT ( 'NONE',  ( 9.999999999999998224, 1.224646799147353059E-15, -99.99999999999998579 ) ) ;
#31114=CARTESIAN_POINT ( 'NONE',  ( -5.405949406249996869, 9.363379034771805109, -185.5312500020484094 ) ) ;
#31116=FACE_OUTER_BOUND ( 'NONE', #2286, .T. ) ;
#31120=CARTESIAN_POINT ( 'NONE',  ( -5.405949406249996869, 9.363379034771805109, -119.3437500020483810 ) ) ;
#31122=CARTESIAN_POINT ( 'NONE',  ( -10.81189881249999729, 1.324075727343319199E-15, -123.7812500020483952 ) ) ;
#31124=CARTESIAN_POINT ( 'NONE',  ( -10.81189881249999729, 1.324075727343319199E-15, -132.5937500020483810 ) ) ;
#31126=CARTESIAN_POINT ( 'NONE',  ( -9.999999999999998224, 1.224646799147353059E-15, -163.2500000000000000 ) ) ;
#31128=CARTESIAN_POINT ( 'NONE',  ( 5.000000000000000000, 8.660254037844385522, -145.7500000000000000 ) ) ;
#31129=CARTESIAN_POINT ( 'NONE',  ( 9.999999999999996447, -5.773502691896262640, -23.12499999999997868 ) ) ;
#31135=CARTESIAN_POINT ( 'NONE',  ( -10.81189881249999729, 6.242252689847871849, -42.71875000204835970 ) ) ;
#31137=CARTESIAN_POINT ( 'NONE',  ( 5.405949406249999534, 9.363379034771803333, -152.5937500020483810 ) ) ;
#31141=CARTESIAN_POINT ( 'NONE',  ( -10.00000000000000000, -5.773502691896251982, -74.62499999999997158 ) ) ;
#31144=CARTESIAN_POINT ( 'NONE',  ( -2.293366432827344421E-15, -12.48450537969573659, -100.9062500020483952 ) ) ;
#31145=CARTESIAN_POINT ( 'NONE',  ( -9.999999999999998224, 1.224646799147353059E-15, -124.6250000040967763 ) ) ;
#31149=EDGE_CURVE ( 'NONE', #40511, #9826, #20212, .T. ) ;
#31150=CARTESIAN_POINT ( 'NONE',  ( 5.000000000000000000, 8.660254037844385522, -130.7499999999999716 ) ) ;
#31151=CARTESIAN_POINT ( 'NONE',  ( 10.81189881249999907, 6.242252689847868297, -44.90625000204836681 ) ) ;
#31157=CARTESIAN_POINT ( 'NONE',  ( -9.999999999999998224, 1.224646799147353059E-15, -102.1250000040967905 ) ) ;
#31158=EDGE_LOOP ( 'NONE', ( #13967, #5130, #13700, #10360 ) ) ;
#31159=AXIS2_PLACEMENT_3D ( 'NONE', #33591, #11106, #17155 ) ;
#31172=CARTESIAN_POINT ( 'NONE',  ( -2.293366432827344421E-15, -12.48450537969573659, -141.2187500020483810 ) ) ;
#31173=CARTESIAN_POINT ( 'NONE',  ( 5.405949406249992428, -9.363379034771808662, -151.7812500020484094 ) ) ;
#31174=CARTESIAN_POINT ( 'NONE',  ( -5.405949406249996869, 9.363379034771805109, -150.8437500020483810 ) ) ;
#31177=CARTESIAN_POINT ( 'NONE',  ( 10.00000000000000000, 5.773502691896255534, -172.8750000000000000 ) ) ;
#31179=CARTESIAN_POINT ( 'NONE',  ( -6.652853726956784897, 8.522716305231336165, -100.0000000000000142 ) ) ;
#31181=CARTESIAN_POINT ( 'NONE',  ( 10.00000000000000000, 5.773502691896255534, -133.8750000000000000 ) ) ;
#31182=CARTESIAN_POINT ( 'NONE',  ( -5.405949406249996869, 9.363379034771805109, -180.8437500020483810 ) ) ;
#31185=CARTESIAN_POINT ( 'NONE',  ( 0.000000000000000000, 0.000000000000000000, -99.99999999999998579 ) ) ;
#31186=CARTESIAN_POINT ( 'NONE',  ( -5.405949406250003975, -9.363379034771801557, -41.03125000204838102 ) ) ;
#31188=CARTESIAN_POINT ( 'NONE',  ( 10.00000000000000000, 5.773502691896255534, -109.8750000000000000 ) ) ;
#31190=CARTESIAN_POINT ( 'NONE',  ( -2.293366432827344421E-15, -12.48450537969573659, -126.4062500020483810 ) ) ;
#31191=CARTESIAN_POINT ( 'NONE',  ( -9.999999999999998224, 5.773502691896259087, -151.7500000040967620 ) ) ;
#31195=CARTESIAN_POINT ( 'NONE',  ( 10.81189881249999551, -6.242252689847874514, -172.4687500020484094 ) ) ;
#31201=CARTESIAN_POINT ( 'NONE',  ( 7.644554776091147741E-16, 12.48450537969573659, -70.15625000204839523 ) ) ;
#31203=CARTESIAN_POINT ( 'NONE',  ( -5.000000000000003553, -8.660254037844383745, -44.87500000409677625 ) ) ;
#31204=CARTESIAN_POINT ( 'NONE',  ( 5.405949406249992428, -9.363379034771808662, -1.593750002048366365 ) ) ;
#31205=FACE_OUTER_BOUND ( 'NONE', #20949, .T. ) ;
#31212=CARTESIAN_POINT ( 'NONE',  ( -9.999999999999998224, 0.000000000000000000, -99.99999999999998579 ) ) ;
#31213=( BOUNDED_CURVE ( )  B_SPLINE_CURVE ( 2, ( #15775, #41896, #3274, #36074, #38678, #19033, #28554 ),
 .UNSPECIFIED., .F., .F. ) 
 B_SPLINE_CURVE_WITH_KNOTS ( ( 3, 2, 2, 3 ),
 ( 0.3320895522388061516, 0.3333333333333334259, 0.3345771144278607556, 0.3358208955223880854 ),
 .UNSPECIFIED. ) 
 CURVE ( )  GEOMETRIC_REPRESENTATION_ITEM ( )  RATIONAL_B_SPLINE_CURVE ( ( 0.9999999999999820144, 0.8660254037844566932, 1.000000000000000000, 0.8660254037844387076, 1.000000000000000000, 0.8660254037844387076, 1.000000000000000000 ) ) 
 REPRESENTATION_ITEM ( '' )  );
#31217=ORIENTED_EDGE ( 'NONE', *, *, #2500, .T. ) ;
#31218=ORIENTED_EDGE ( 'NONE', *, *, #21729, .F. ) ;
#31226=CARTESIAN_POINT ( 'NONE',  ( 9.999999999999996447, -5.773502691896262640, -36.62499999999996447 ) ) ;
#31229=CARTESIAN_POINT ( 'NONE',  ( -2.293366432827344421E-15, -12.48450537969573659, -168.2187500020483810 ) ) ;
#31234=CARTESIAN_POINT ( 'NONE',  ( -5.000000000000003553, -8.660254037844383745, -196.0000000000000000 ) ) ;
#31239=CARTESIAN_POINT ( 'NONE',  ( 10.81189881249999551, -6.242252689847874514, -62.96875000204838102 ) ) ;
#31240=CARTESIAN_POINT ( 'NONE',  ( 10.81189881249999907, 6.242252689847868297, -67.40625000204839523 ) ) ;
#31242=CARTESIAN_POINT ( 'NONE',  ( -5.000000000000003553, -8.660254037844383745, -131.5000000000000000 ) ) ;
#31243=CARTESIAN_POINT ( 'NONE',  ( -5.405949406249996869, 9.363379034771805109, -152.5312500020484094 ) ) ;
#31244=CARTESIAN_POINT ( 'NONE',  ( -10.81189881249999729, 6.242252689847871849, -164.4062500020484094 ) ) ;
#31247=CARTESIAN_POINT ( 'NONE',  ( -2.293366432827344421E-15, -12.48450537969573659, -97.71875000204838102 ) ) ;
#31250=CARTESIAN_POINT ( 'NONE',  ( -5.405949406249996869, 9.363379034771805109, -197.3437500020484094 ) ) ;
#31252=EDGE_CURVE ( 'NONE', #17462, #17801, #21861, .T. ) ;
#31253=CARTESIAN_POINT ( 'NONE',  ( -3.767292561726145905, -9.597395893938625022, -179.9999999999999716 ) ) ;
#31254=CARTESIAN_POINT ( 'NONE',  ( -2.293366432827344421E-15, -12.48450537969573659, -90.40625000204838102 ) ) ;
#31257=CARTESIAN_POINT ( 'NONE',  ( -2.121150477449813534E-15, -11.54700538379251284, -68.75000000409679046 ) ) ;
#31258=CARTESIAN_POINT ( 'NONE',  ( 9.999999999999742428, 5.773502691896404748, -135.3750000000000000 ) ) ;
#31259=CARTESIAN_POINT ( 'NONE',  ( -10.81189881249999907, -6.242252689847864744, -24.46875000204837036 ) ) ;
#31263=CARTESIAN_POINT ( 'NONE',  ( -10.81189881249999907, -6.242252689847864744, -18.65625000204837747 ) ) ;
#31266=CARTESIAN_POINT ( 'NONE',  ( -5.000000000000003553, -8.660254037844383745, -2.875000004096767370 ) ) ;
#31272=FACE_OUTER_BOUND ( 'NONE', #14967, .T. ) ;
#31280=CARTESIAN_POINT ( 'NONE',  ( -2.121150477449813534E-15, -11.54700538379251284, -128.7500000040967905 ) ) ;
#31281=CARTESIAN_POINT ( 'NONE',  ( 9.999999999999998224, 1.224646799147353059E-15, -99.99999999999998579 ) ) ;
#31282=CARTESIAN_POINT ( 'NONE',  ( 10.81189881249999907, 6.242252689847868297, -167.9062500020484094 ) ) ;
#31286=CARTESIAN_POINT ( 'NONE',  ( -10.81189881249999729, 6.242252689847871849, -83.21875000204838102 ) ) ;
#31288=CARTESIAN_POINT ( 'NONE',  ( 5.405949406249992428, -9.363379034771808662, -196.5937500020484094 ) ) ;
#31289=CARTESIAN_POINT ( 'NONE',  ( -5.405949406249996869, 9.363379034771805109, -91.03125000204838102 ) ) ;
#31293=CARTESIAN_POINT ( 'NONE',  ( 5.405949406249999534, 9.363379034771803333, -178.2812500020484094 ) ) ;
#31294=CARTESIAN_POINT ( 'NONE',  ( -10.81189881249999729, 6.242252689847871849, -188.4062500020484094 ) ) ;
#31296=CARTESIAN_POINT ( 'NONE',  ( 7.070501591499377789E-16, 11.54700538379251284, -161.0000000040967905 ) ) ;
#31298=CARTESIAN_POINT ( 'NONE',  ( 10.81189881249999729, 0.000000000000000000, -16.34375000204835260 ) ) ;
#31300=CARTESIAN_POINT ( 'NONE',  ( 10.81189881249999907, 6.242252689847868297, -124.2187500020483952 ) ) ;
#31302=CARTESIAN_POINT ( 'NONE',  ( -2.293366432827344421E-15, -12.48450537969573659, -22.90625000204837747 ) ) ;
#31305=CARTESIAN_POINT ( 'NONE',  ( -5.000000000000003553, -8.660254037844383745, -51.99999999999996447 ) ) ;
#31306=CARTESIAN_POINT ( 'NONE',  ( 7.644554776091147741E-16, 12.48450537969573659, -119.6562500020484094 ) ) ;
#31308=VERTEX_POINT ( 'NONE', #32550 ) ;
#31309=CARTESIAN_POINT ( 'NONE',  ( -4.999999999999996447, 8.660254037844387298, -96.37500000409677625 ) ) ;
#31310=CARTESIAN_POINT ( 'NONE',  ( 4.999999999999992006, -8.660254037844389075, -113.2499999999999858 ) ) ;
#31312=CARTESIAN_POINT ( 'NONE',  ( 7.644554776091147741E-16, 12.48450537969573659, -47.46875000204836681 ) ) ;
#31313=ORIENTED_EDGE ( 'NONE', *, *, #1914, .F. ) ;
#31318=CARTESIAN_POINT ( 'NONE',  ( 4.999999999999992006, -8.660254037844389075, -31.12500000409676559 ) ) ;
#31319=CYLINDRICAL_SURFACE ( 'NONE', #37350, 9.999999999999998224 ) ;
#31327=ORIENTED_EDGE ( 'NONE', *, *, #39233, .F. ) ;
#31328=VERTEX_POINT ( 'NONE', #12453 ) ;
#31333=CARTESIAN_POINT ( 'NONE',  ( 7.644554776091147741E-16, 12.48450537969573659, -191.6562500020484094 ) ) ;
#31338=CARTESIAN_POINT ( 'NONE',  ( 10.81189881249999729, 0.000000000000000000, -107.8437500020483810 ) ) ;
#31340=CARTESIAN_POINT ( 'NONE',  ( -10.81189881249999907, -6.242252689847864744, -117.6562500020483952 ) ) ;
#31342=CARTESIAN_POINT ( 'NONE',  ( 7.644554776091147741E-16, 12.48450537969573659, -131.4687500020483810 ) ) ;
#31345=CARTESIAN_POINT ( 'NONE',  ( 10.00000000000000000, 5.773502691896255534, -148.8750000000000000 ) ) ;
#31346=CARTESIAN_POINT ( 'NONE',  ( -10.00000000000000000, -5.773502691896251982, -16.12499999999997158 ) ) ;
#31349=CARTESIAN_POINT ( 'NONE',  ( -9.999999999999998224, 5.773502691896259087, -190.7500000040968189 ) ) ;
#31351=CARTESIAN_POINT ( 'NONE',  ( -10.81189881249999729, 1.324075727343319199E-15, -36.59375000204836681 ) ) ;
#31352=CARTESIAN_POINT ( 'NONE',  ( 0.000000000000000000, 0.000000000000000000, -99.99999999999998579 ) ) ;
#31353=CARTESIAN_POINT ( 'NONE',  ( 10.81189881249999907, 6.242252689847868297, -146.7187500020484094 ) ) ;
#31355=CARTESIAN_POINT ( 'NONE',  ( -10.00000000000076916, 5.773502691895813221, -136.3749999999999716 ) ) ;
#31356=CARTESIAN_POINT ( 'NONE',  ( 9.999999999999998224, 0.000000000000000000, -75.49999999999998579 ) ) ;
#31358=ORIENTED_EDGE ( 'NONE', *, *, #1117, .F. ) ;
#31360=CARTESIAN_POINT ( 'NONE',  ( -9.999999999999998224, 5.773502691896259087, -127.7500000040967905 ) ) ;
#31361=CARTESIAN_POINT ( 'NONE',  ( 9.999999999999998224, 0.000000000000000000, -143.3750000040967905 ) ) ;
#31362=CARTESIAN_POINT ( 'NONE',  ( -10.81189881249999729, 6.242252689847871849, -78.71875000204838102 ) ) ;
#31365=CARTESIAN_POINT ( 'NONE',  ( 10.81189881249999729, 0.000000000000000000, -42.03125000204838102 ) ) ;
#31374=VERTEX_POINT ( 'NONE', #28681 ) ;
#31383=CARTESIAN_POINT ( 'NONE',  ( 10.81189881249999907, 6.242252689847868297, -136.2187500020483810 ) ) ;
#31384=CARTESIAN_POINT ( 'NONE',  ( 10.81189881249999729, 0.000000000000000000, -138.0312500020484094 ) ) ;
#31385=CARTESIAN_POINT ( 'NONE',  ( -10.81189881249999729, -6.242252689847864744, -157.9687500020484379 ) ) ;
#31388=CARTESIAN_POINT ( 'NONE',  ( 7.070501591499377789E-16, 11.54700538379251284, -169.6250000000000000 ) ) ;
#31392=CARTESIAN_POINT ( 'NONE',  ( -9.955545358920547372, 3.667973230269648610, -99.99999999999998579 ) ) ;
#31393=CARTESIAN_POINT ( 'NONE',  ( 10.81189881249999551, -6.242252689847874514, -169.4687500020483810 ) ) ;
#31397=CARTESIAN_POINT ( 'NONE',  ( 10.81189881249999729, 0.000000000000000000, -46.53125000204838813 ) ) ;
#31399=CARTESIAN_POINT ( 'NONE',  ( -4.999999999999996447, 8.660254037844387298, -98.99999999999998579 ) ) ;
#31402=CARTESIAN_POINT ( 'NONE',  ( 5.405949406249992428, -9.363379034771808662, -129.2812500020483810 ) ) ;
#31403=CARTESIAN_POINT ( 'NONE',  ( -9.999999999999998224, 1.224646799147353059E-15, -147.1250000040967905 ) ) ;
#31407=CARTESIAN_POINT ( 'NONE',  ( -10.81189881249999729, 6.242252689847871849, -171.7187500020483810 ) ) ;
#31411=CARTESIAN_POINT ( 'NONE',  ( -2.293366432827344421E-15, -12.48450537969573659, -67.90625000204838102 ) ) ;
#31412=CARTESIAN_POINT ( 'NONE',  ( -4.999999999999996447, 8.660254037844387298, -43.87500000409677625 ) ) ;
#31413=CARTESIAN_POINT ( 'NONE',  ( -5.405949406249996869, 9.363379034771805109, -3.843750002048368586 ) ) ;
#31416=CARTESIAN_POINT ( 'NONE',  ( 9.999999999999998224, 0.000000000000000000, -112.9999999999999858 ) ) ;
#31423=ORIENTED_EDGE ( 'NONE', *, *, #28393, .T. ) ;
#31433=DIRECTION ( 'NONE',  ( -1.000000000000000000, 0.000000000000000000, 0.000000000000000000 ) ) ;
#31435=CARTESIAN_POINT ( 'NONE',  ( 5.000000000000000000, 8.660254037844385522, -37.74999999999997868 ) ) ;
#31438=CARTESIAN_POINT ( 'NONE',  ( -10.81189881249999907, -6.242252689847864744, -163.9687500020484094 ) ) ;
#31439=CARTESIAN_POINT ( 'NONE',  ( 7.644554776091147741E-16, 12.48450537969573659, -176.4687500020484094 ) ) ;
#31441=CARTESIAN_POINT ( 'NONE',  ( 10.00000000000025402, -5.773502691896113426, -126.6249999999999858 ) ) ;
#31442=CARTESIAN_POINT ( 'NONE',  ( -9.999999999999998224, 1.224646799147353059E-15, -191.7500000000000000 ) ) ;
#31447=CARTESIAN_POINT ( 'NONE',  ( 10.81189881249999729, 0.000000000000000000, -59.84375000204835970 ) ) ;
#31448=CARTESIAN_POINT ( 'NONE',  ( -2.293366432827344421E-15, -12.48450537969573659, -67.90625000204838102 ) ) ;
#31450=CARTESIAN_POINT ( 'NONE',  ( -5.000000000000003553, -8.660254037844383745, -122.5000000000000000 ) ) ;
#31451=CARTESIAN_POINT ( 'NONE',  ( -5.405949406250003975, -9.363379034771801557, -147.5312500020483810 ) ) ;
#31452=CARTESIAN_POINT ( 'NONE',  ( -5.405949406249996869, 9.363379034771805109, -166.0312500020484094 ) ) ;
#31453=DIRECTION ( 'NONE',  ( -1.000000000000000000, 0.000000000000000000, 0.000000000000000000 ) ) ;
#31455=CARTESIAN_POINT ( 'NONE',  ( 5.405949406249999534, 9.363379034771803333, -95.59375000204838102 ) ) ;
#31456=ORIENTED_EDGE ( 'NONE', *, *, #27172, .F. ) ;
#31458=CARTESIAN_POINT ( 'NONE',  ( 5.405949406249992428, -9.363379034771808662, -198.0937500020484094 ) ) ;
#31461=CARTESIAN_POINT ( 'NONE',  ( 7.644554776091147741E-16, 12.48450537969573659, -92.65625000204839523 ) ) ;
#31463=( BOUNDED_CURVE ( )  B_SPLINE_CURVE ( 2, ( #40325, #20484, #23738, #27398, #36680, #1290, #40122 ),
 .UNSPECIFIED., .F., .F. ) 
 B_SPLINE_CURVE_WITH_KNOTS ( ( 3, 2, 2, 3 ),
 ( 0.3283582089552238847, 0.3296019900497513255, 0.3308457711442787108, 0.3320895522388061516 ),
 .UNSPECIFIED. ) 
 CURVE ( )  GEOMETRIC_REPRESENTATION_ITEM ( )  RATIONAL_B_SPLINE_CURVE ( ( 1.000000000000000000, 0.8660254037844387076, 1.000000000000000000, 0.8660254037844387076, 1.000000000000000000, 0.8660254037844207220, 1.000000000000017986 ) ) 
 REPRESENTATION_ITEM ( '' )  );
#31464=CARTESIAN_POINT ( 'NONE',  ( 7.070501591499377789E-16, 11.54700538379251284, -65.00000000409677625 ) ) ;
#31466=CARTESIAN_POINT ( 'NONE',  ( -5.405949406250003975, -9.363379034771801557, -24.34375000204835970 ) ) ;
#31469=CARTESIAN_POINT ( 'NONE',  ( -10.81189881249999729, 1.324075727343319199E-15, -21.78125000204836326 ) ) ;
#31483=ORIENTED_EDGE ( 'NONE', *, *, #33653, .F. ) ;
#31489=CARTESIAN_POINT ( 'NONE',  ( 9.999999999999998224, 1.224646799147353059E-15, -99.99999999999998579 ) ) ;
#31492=EDGE_CURVE ( 'NONE', #9851, #35407, #7062, .T. ) ;
#31494=CARTESIAN_POINT ( 'NONE',  ( -2.293366432827344421E-15, -12.48450537969573659, -168.4062500020483810 ) ) ;
#31499=CARTESIAN_POINT ( 'NONE',  ( -5.405949406250003975, -9.363379034771801557, -85.84375000204836681 ) ) ;
#31501=CARTESIAN_POINT ( 'NONE',  ( -10.81189881249999729, 1.324075727343319199E-15, -197.0937500020484094 ) ) ;
#31502=CARTESIAN_POINT ( 'NONE',  ( -10.81189881249999729, 1.324075727343319199E-15, -95.28125000204838102 ) ) ;
#31506=CARTESIAN_POINT ( 'NONE',  ( -10.81189881249999729, -6.242252689847864744, -177.6562500020484094 ) ) ;
#31507=CARTESIAN_POINT ( 'NONE',  ( 10.81189881249999907, 6.242252689847868297, -188.9062500020484379 ) ) ;
#31509=CARTESIAN_POINT ( 'NONE',  ( -2.121150477449813534E-15, -11.54700538379251284, -167.7500000040968189 ) ) ;
#31511=CARTESIAN_POINT ( 'NONE',  ( 5.405949406249992428, -9.363379034771808662, -13.59375000204834905 ) ) ;
#31513=CARTESIAN_POINT ( 'NONE',  ( 5.405949406249992428, -9.363379034771808662, -120.0937500020483952 ) ) ;
#31515=CARTESIAN_POINT ( 'NONE',  ( -5.405949406249996869, 9.363379034771805109, -22.03125000204836326 ) ) ;
#31519=CARTESIAN_POINT ( 'NONE',  ( -2.121150477449813534E-15, -11.54700538379251284, -54.87499999999997868 ) ) ;
#31520=CARTESIAN_POINT ( 'NONE',  ( 10.81189881249999729, 0.000000000000000000, -115.5312500020483952 ) ) ;
#31523=CARTESIAN_POINT ( 'NONE',  ( -4.999999999999996447, 8.660254037844387298, -93.37500000409677625 ) ) ;
#31526=CARTESIAN_POINT ( 'NONE',  ( -5.405949406249996869, 9.363379034771805109, -51.84375000204835260 ) ) ;
#31528=EDGE_CURVE ( 'NONE', #13549, #39100, #14398, .T. ) ;
#31532=CARTESIAN_POINT ( 'NONE',  ( -9.999999999999998224, 5.773502691896259087, -18.25000000409676559 ) ) ;
#31538=ORIENTED_EDGE ( 'NONE', *, *, #4281, .F. ) ;
#31547=CARTESIAN_POINT ( 'NONE',  ( -5.405949406249996869, 9.363379034771805109, -187.0312500020484094 ) ) ;
#31551=CARTESIAN_POINT ( 'NONE',  ( 5.405949406249999534, 9.363379034771803333, -112.0937500020483810 ) ) ;
#31553=CARTESIAN_POINT ( 'NONE',  ( 5.405949406249999534, 9.363379034771803333, -118.2812500020483952 ) ) ;
#31555=CARTESIAN_POINT ( 'NONE',  ( 5.405949406249992428, -9.363379034771808662, -120.0937500020483952 ) ) ;
#31558=CARTESIAN_POINT ( 'NONE',  ( 10.00000000000000000, 5.773502691896255534, -144.3750000000000284 ) ) ;
#31559=CARTESIAN_POINT ( 'NONE',  ( 7.070501591499377789E-16, 11.54700538379251284, -10.62499999999996803 ) ) ;
#31563=CARTESIAN_POINT ( 'NONE',  ( 7.070501591499377789E-16, 11.54700538379251284, -191.0000000040968189 ) ) ;
#31565=CARTESIAN_POINT ( 'NONE',  ( 5.405949406249999534, 9.363379034771803333, -38.59375000204837391 ) ) ;
#31567=CARTESIAN_POINT ( 'NONE',  ( -10.81189881249999729, 1.324075727343319199E-15, -147.5937500020483810 ) ) ;
#31569=LINE ( 'NONE', #41242, #16880 ) ;
#31570=CARTESIAN_POINT ( 'NONE',  ( -4.999999999999996447, 8.660254037844387298, -74.99999999999998579 ) ) ;
#31571=CARTESIAN_POINT ( 'NONE',  ( 10.81189881249999907, 6.242252689847868297, -137.9062500020483810 ) ) ;
#31574=CARTESIAN_POINT ( 'NONE',  ( 10.00000000000025402, -5.773502691896113426, -164.1250000000000284 ) ) ;
#31575=CARTESIAN_POINT ( 'NONE',  ( -5.000000000000003553, -8.660254037844383745, -118.3750000040967905 ) ) ;
#31576=CARTESIAN_POINT ( 'NONE',  ( -9.999999999999998224, 1.224646799147353059E-15, -140.7500000000000000 ) ) ;
#31577=CARTESIAN_POINT ( 'NONE',  ( -10.81189881249999729, 6.242252689847871849, -71.21875000204839523 ) ) ;
#31580=CARTESIAN_POINT ( 'NONE',  ( 10.81189881249999729, 0.000000000000000000, -48.03125000204838813 ) ) ;
#31598=CARTESIAN_POINT ( 'NONE',  ( 7.644554776091147741E-16, 12.48450537969573659, -137.4687500020483810 ) ) ;
#31599=CARTESIAN_POINT ( 'NONE',  ( -2.293366432827344421E-15, -12.48450537969573659, -144.4062500020484094 ) ) ;
#31600=CARTESIAN_POINT ( 'NONE',  ( -10.81189881249999729, 1.324075727343319199E-15, -144.5937500020483810 ) ) ;
#31603=CARTESIAN_POINT ( 'NONE',  ( 5.000000000000000000, 8.660254037844385522, -169.7500000000000000 ) ) ;
#31606=CARTESIAN_POINT ( 'NONE',  ( 0.000000000000000000, 0.000000000000000000, -99.99999999999998579 ) ) ;
#31608=CARTESIAN_POINT ( 'NONE',  ( -10.18354000214830002, 2.855663046881824485, -99.99999999999992895 ) ) ;
#31609=CARTESIAN_POINT ( 'NONE',  ( -5.405949406250003975, -9.363379034771801557, -166.8437500020484094 ) ) ;
#31613=CARTESIAN_POINT ( 'NONE',  ( 5.405949406249992428, -9.363379034771808662, -43.78125000204838102 ) ) ;
#31615=CARTESIAN_POINT ( 'NONE',  ( -10.00000000000000000, -5.773502691896251982, -95.62499999999998579 ) ) ;
#31616=VERTEX_POINT ( 'NONE', #23250 ) ;
#31617=CARTESIAN_POINT ( 'NONE',  ( -5.405949406250003975, -9.363379034771801557, -129.5312500020484094 ) ) ;
#31618=CARTESIAN_POINT ( 'NONE',  ( -5.000000000000003553, -8.660254037844383745, -136.3750000040967905 ) ) ;
#31621=ORIENTED_EDGE ( 'NONE', *, *, #651, .T. ) ;
#31622=CARTESIAN_POINT ( 'NONE',  ( -10.81189881249999907, -6.242252689847864744, -174.4687500020484094 ) ) ;
#31626=CARTESIAN_POINT ( 'NONE',  ( 0.000000000000000000, 0.000000000000000000, -180.0000000000000000 ) ) ;
#31627=CARTESIAN_POINT ( 'NONE',  ( -5.405949406249996869, 9.363379034771805109, -71.53125000204838102 ) ) ;
#31629=CARTESIAN_POINT ( 'NONE',  ( 9.999999999999996447, -5.773502691896262640, -43.00000000409676915 ) ) ;
#31630=CARTESIAN_POINT ( 'NONE',  ( 7.644554776091147741E-16, 12.48450537969573659, -3.968750002048354819 ) ) ;
#31635=EDGE_LOOP ( 'NONE', ( #41908, #40459, #28376, #1686 ) ) ;
#31639=ORIENTED_EDGE ( 'NONE', *, *, #34818, .T. ) ;
#31649=CARTESIAN_POINT ( 'NONE',  ( 7.070501591499377789E-16, 11.54700538379251284, -34.62499999999995737 ) ) ;
#31653=CARTESIAN_POINT ( 'NONE',  ( -5.405949406250003975, -9.363379034771801557, -159.3437500020484094 ) ) ;
#31654=CARTESIAN_POINT ( 'NONE',  ( 7.644554776091147741E-16, 12.48450537969573659, -174.9687500020484094 ) ) ;
#31657=CARTESIAN_POINT ( 'NONE',  ( -4.999999999999996447, 8.660254037844387298, -198.0000000000000000 ) ) ;
#31658=VECTOR ( 'NONE', #3415, 1000.000000000000000 ) ;
#31663=CARTESIAN_POINT ( 'NONE',  ( 5.405949406249992428, -9.363379034771808662, -66.28125000204838102 ) ) ;
#31665=CARTESIAN_POINT ( 'NONE',  ( 9.999999999999998224, 0.000000000000000000, -126.5000000000000000 ) ) ;
#31666=ORIENTED_EDGE ( 'NONE', *, *, #1721, .T. ) ;
#31668=CARTESIAN_POINT ( 'NONE',  ( 7.644554776091147741E-16, 12.48450537969573659, -149.6562500020484094 ) ) ;
#31669=CARTESIAN_POINT ( 'NONE',  ( 10.81189881249999907, 6.242252689847868297, -160.4062500020484094 ) ) ;
#31672=CARTESIAN_POINT ( 'NONE',  ( 5.405949406249999534, 9.363379034771803333, -101.5937500020483810 ) ) ;
#31675=CARTESIAN_POINT ( 'NONE',  ( -5.405949406250003975, -9.363379034771801557, -193.8437500020484094 ) ) ;
#31677=FACE_OUTER_BOUND ( 'NONE', #29832, .T. ) ;
#31679=CARTESIAN_POINT ( 'NONE',  ( -10.81189881249999729, 6.242252689847871849, -93.90625000204839523 ) ) ;
#31681=CARTESIAN_POINT ( 'NONE',  ( -5.000000000000003553, -8.660254037844383745, -65.87500000409676204 ) ) ;
#31683=CARTESIAN_POINT ( 'NONE',  ( 7.644554776091147741E-16, 12.48450537969573659, -23.46875000204837391 ) ) ;
#31686=CARTESIAN_POINT ( 'NONE',  ( 7.644554776091147741E-16, 12.48450537969573659, -22.15625000204837747 ) ) ;
#31687=EDGE_CURVE ( 'NONE', #39101, #28777, #20850, .T. ) ;
#31697=VERTEX_POINT ( 'NONE', #34034 ) ;
#31698=CARTESIAN_POINT ( 'NONE',  ( -9.999999999999998224, 1.224646799147353059E-15, -111.1250000040967763 ) ) ;
#31706=DIRECTION ( 'NONE',  ( -0.000000000000000000, -0.000000000000000000, -1.000000000000000000 ) ) ;
#31708=CARTESIAN_POINT ( 'NONE',  ( 4.999999999999992006, -8.660254037844389075, -127.1250000040967620 ) ) ;
#31709=CARTESIAN_POINT ( 'NONE',  ( 7.644554776091147741E-16, 12.48450537969573659, -161.6562500020484379 ) ) ;
#31711=DIRECTION ( 'NONE',  ( -1.000000000000000000, 0.000000000000000000, 0.000000000000000000 ) ) ;
#31713=CARTESIAN_POINT ( 'NONE',  ( -10.81189881249999729, 6.242252689847871849, -86.21875000204838102 ) ) ;
#31714=CARTESIAN_POINT ( 'NONE',  ( 10.81189881249999551, -6.242252689847874514, -197.9687500020484094 ) ) ;
#31715=CARTESIAN_POINT ( 'NONE',  ( 10.81189881249999551, -6.242252689847874514, -90.15625000204836681 ) ) ;
#31719=CARTESIAN_POINT ( 'NONE',  ( 9.999999999999998224, 0.000000000000000000, -150.5000000000000000 ) ) ;
#31720=CARTESIAN_POINT ( 'NONE',  ( 10.81189881249999551, -6.242252689847874514, -172.6562500020484094 ) ) ;
#31721=CARTESIAN_POINT ( 'NONE',  ( 10.81189881249999907, 6.242252689847868297, -184.4062500020484094 ) ) ;
#31724=CARTESIAN_POINT ( 'NONE',  ( 7.070501591499377789E-16, 11.54700538379251284, -167.0000000040967905 ) ) ;
#31726=CARTESIAN_POINT ( 'NONE',  ( -10.81189881249999729, 6.242252689847871849, -12.71875000204836326 ) ) ;
#31728=CARTESIAN_POINT ( 'NONE',  ( -5.405949406249996869, 9.363379034771805109, -119.3437500020483810 ) ) ;
#31730=CARTESIAN_POINT ( 'NONE',  ( 10.81189881249999729, 0.000000000000000000, -19.53125000204835970 ) ) ;
#31733=CARTESIAN_POINT ( 'NONE',  ( -9.999999999999998224, 1.224646799147353059E-15, -55.24999999999996447 ) ) ;
#31734=CARTESIAN_POINT ( 'NONE',  ( 10.81189881249999729, 0.000000000000000000, -117.0312500020483952 ) ) ;
#31737=( BOUNDED_CURVE ( )  B_SPLINE_CURVE ( 2, ( #9578, #19499, #3114, #29655, #16241, #29442, #13008 ),
 .UNSPECIFIED., .F., .F. ) 
 B_SPLINE_CURVE_WITH_KNOTS ( ( 3, 2, 2, 3 ),
 ( 0.1567164179104477695, 0.1579601990049751270, 0.1592039800995025123, 0.1604477611940298698 ),
 .UNSPECIFIED. ) 
 CURVE ( )  GEOMETRIC_REPRESENTATION_ITEM ( )  RATIONAL_B_SPLINE_CURVE ( ( 1.000000000000000000, 0.8660254037844387076, 1.000000000000000000, 0.8660254037844387076, 1.000000000000000000, 0.8660254037844357100, 1.000000000000003109 ) ) 
 REPRESENTATION_ITEM ( '' )  );
#31738=CARTESIAN_POINT ( 'NONE',  ( 7.070501591499377789E-16, 11.54700538379251284, -89.00000000409677625 ) ) ;
#31739=CYLINDRICAL_SURFACE ( 'NONE', #34652, 9.999999999999998224 ) ;
#31741=CARTESIAN_POINT ( 'NONE',  ( 5.405949406249999534, 9.363379034771803333, -49.09375000204838102 ) ) ;
#31747=CARTESIAN_POINT ( 'NONE',  ( 9.999999999999998224, 0.000000000000000000, -21.87500000409675494 ) ) ;
#31757=ORIENTED_EDGE ( 'NONE', *, *, #21759, .F. ) ;
#31758=ORIENTED_EDGE ( 'NONE', *, *, #23406, .F. ) ;
#31759=EDGE_CURVE ( 'NONE', #19819, #18647, #35113, .T. ) ;
#31761=LINE ( 'NONE', #15323, #22873 ) ;
#31763=CARTESIAN_POINT ( 'NONE',  ( 7.644554776091147741E-16, 12.48450537969573659, -187.1562500020484094 ) ) ;
#31767=CARTESIAN_POINT ( 'NONE',  ( -5.405949406250003975, -9.363379034771801557, -112.8437500020483810 ) ) ;
#31768=CARTESIAN_POINT ( 'NONE',  ( 9.999999999999998224, 0.000000000000000000, -147.8750000040967905 ) ) ;
#31769=CARTESIAN_POINT ( 'NONE',  ( 10.81189881249999551, -6.242252689847874514, -115.6562500020483810 ) ) ;
#31771=CARTESIAN_POINT ( 'NONE',  ( 10.81189881249999729, 6.242252689847867408, -121.2187500020483952 ) ) ;
#31774=CARTESIAN_POINT ( 'NONE',  ( 5.000000000000000000, 8.660254037844385522, -150.2500000000000000 ) ) ;
#31775=CARTESIAN_POINT ( 'NONE',  ( -5.000000000000003553, -8.660254037844383745, -11.49999999999995381 ) ) ;
#31778=CARTESIAN_POINT ( 'NONE',  ( -5.000000000000003553, -8.660254037844383745, -184.3750000040967905 ) ) ;
#31780=CARTESIAN_POINT ( 'NONE',  ( -2.293366432827344421E-15, -12.48450537969573659, -37.71875000204835970 ) ) ;
#31782=CARTESIAN_POINT ( 'NONE',  ( 10.81189881249999729, 0.000000000000000000, -143.8437500020483810 ) ) ;
#31785=CARTESIAN_POINT ( 'NONE',  ( -10.00000000000000000, -5.773502691896251982, -76.12499999999997158 ) ) ;
#31786=CARTESIAN_POINT ( 'NONE',  ( -2.293366432827344421E-15, -12.48450537969573659, -139.9062500020484094 ) ) ;
#31790=CARTESIAN_POINT ( 'NONE',  ( -10.00000000000000000, -5.773502691896251982, -120.0000000040967905 ) ) ;
#31792=CARTESIAN_POINT ( 'NONE',  ( 5.405949406249999534, 9.363379034771803333, -71.59375000204836681 ) ) ;
#31798=CARTESIAN_POINT ( 'NONE',  ( 9.999999999999998224, 0.000000000000000000, -131.0000000000000000 ) ) ;
#31799=CARTESIAN_POINT ( 'NONE',  ( -10.81189881249999729, 6.242252689847871849, -44.40625000204836681 ) ) ;
#31806=( BOUNDED_CURVE ( )  B_SPLINE_CURVE ( 2, ( #27397, #30005, #24392, #10976, #27180, #24172, #34092 ),
 .UNSPECIFIED., .F., .F. ) 
 B_SPLINE_CURVE_WITH_KNOTS ( ( 3, 2, 2, 3 ),
 ( 0.4552238805970150737, 0.4564676616915424590, 0.4577114427860698442, 0.4589552238805971740 ),
 .UNSPECIFIED. ) 
 CURVE ( )  GEOMETRIC_REPRESENTATION_ITEM ( )  RATIONAL_B_SPLINE_CURVE ( ( 0.9999999999999820144, 0.8660254037844566932, 1.000000000000000000, 0.8660254037844387076, 1.000000000000000000, 0.8660254037844207220, 1.000000000000017986 ) ) 
 REPRESENTATION_ITEM ( '' )  );
#31809=ORIENTED_EDGE ( 'NONE', *, *, #31252, .T. ) ;
#31812=AXIS2_PLACEMENT_3D ( 'NONE', #39982, #36962, #36330 ) ;
#31820=CARTESIAN_POINT ( 'NONE',  ( -10.81189881249999729, 1.324075727343319199E-15, -131.0937500020483810 ) ) ;
#31821=CARTESIAN_POINT ( 'NONE',  ( -5.405949406250003975, -9.363379034771801557, -138.5312500020484094 ) ) ;
#31822=CARTESIAN_POINT ( 'NONE',  ( 5.405949406249992428, -9.363379034771808662, -142.5937500020483810 ) ) ;
#31824=CARTESIAN_POINT ( 'NONE',  ( 5.000000000000000000, 8.660254037844385522, -171.2500000000000000 ) ) ;
#31829=CARTESIAN_POINT ( 'NONE',  ( 10.81189881249999551, -6.242252689847874514, -167.9687500020483810 ) ) ;
#31832=FACE_OUTER_BOUND ( 'NONE', #22077, .T. ) ;
#31833=CARTESIAN_POINT ( 'NONE',  ( -10.81189881249999729, 1.324075727343319199E-15, -36.78125000204837391 ) ) ;
#31835=CARTESIAN_POINT ( 'NONE',  ( 4.999999999999992006, -8.660254037844389075, -98.24999999999998579 ) ) ;
#31837=CARTESIAN_POINT ( 'NONE',  ( 10.81189881249999551, -6.242252689847874514, -127.6562500020483810 ) ) ;
#31838=CARTESIAN_POINT ( 'NONE',  ( 7.070501591499377789E-16, 11.54700538379251284, -141.5000000040967905 ) ) ;
#31844=CARTESIAN_POINT ( 'NONE',  ( -10.81189881249999729, 1.324075727343319199E-15, -68.28125000204838102 ) ) ;
#31847=CYLINDRICAL_SURFACE ( 'NONE', #36557, 9.999999999999998224 ) ;
#31850=CARTESIAN_POINT ( 'NONE',  ( -5.000000000000003553, -8.660254037844383745, -163.0000000000000000 ) ) ;
#31854=CARTESIAN_POINT ( 'NONE',  ( 5.000000000000000000, 8.660254037844385522, -173.1250000040968189 ) ) ;
#31859=ORIENTED_EDGE ( 'NONE', *, *, #37405, .F. ) ;
#31861=VERTEX_POINT ( 'NONE', #4244 ) ;
#31868=DIRECTION ( 'NONE',  ( -0.000000000000000000, -0.000000000000000000, -1.000000000000000000 ) ) ;
#31869=CARTESIAN_POINT ( 'NONE',  ( -4.999999999999996447, 8.660254037844387298, -40.49999999999997868 ) ) ;
#31872=CARTESIAN_POINT ( 'NONE',  ( -5.405949406249996869, 9.363379034771805109, -161.3437500020484094 ) ) ;
#31874=CARTESIAN_POINT ( 'NONE',  ( -2.293366432827344421E-15, -12.48450537969573659, -168.2187500020483810 ) ) ;
#31877=CARTESIAN_POINT ( 'NONE',  ( 5.000000000000000000, 8.660254037844385522, -196.7500000000000000 ) ) ;
#31882=CARTESIAN_POINT ( 'NONE',  ( -10.81189881249999729, 1.324075727343319199E-15, -66.78125000204838102 ) ) ;
#31884=CARTESIAN_POINT ( 'NONE',  ( -9.999999999999998224, 5.773502691896259087, -122.8750000000000142 ) ) ;
#31885=VERTEX_POINT ( 'NONE', #35102 ) ;
#31886=CARTESIAN_POINT ( 'NONE',  ( -10.81189881249999729, 6.242252689847871849, -152.4062500020483810 ) ) ;
#31887=CARTESIAN_POINT ( 'NONE',  ( 10.81189881249999551, -6.242252689847874514, -166.6562500020484094 ) ) ;
#31890=CARTESIAN_POINT ( 'NONE',  ( -9.999999999999998224, 1.224646799147353059E-15, -169.2500000000000000 ) ) ;
#31891=CARTESIAN_POINT ( 'NONE',  ( 10.81189881249999551, -6.242252689847874514, -94.46875000204838102 ) ) ;
#31894=CARTESIAN_POINT ( 'NONE',  ( 10.81189881249999907, 6.242252689847868297, -197.7187500020484094 ) ) ;
#31896=CARTESIAN_POINT ( 'NONE',  ( -6.910789922881853897, -7.414454835661850041, -179.9999999999999716 ) ) ;
#31898=CARTESIAN_POINT ( 'NONE',  ( -10.81189881249999729, 1.324075727343319199E-15, -93.78125000204838102 ) ) ;
#31900=CARTESIAN_POINT ( 'NONE',  ( -9.999999999999998224, 1.224646799147353059E-15, -69.12500000409677625 ) ) ;
#31901=CARTESIAN_POINT ( 'NONE',  ( 10.81189881249999907, 6.242252689847868297, -26.71875000204837391 ) ) ;
#31904=CARTESIAN_POINT ( 'NONE',  ( 10.81189881249999907, 6.242252689847868297, -16.40625000204837036 ) ) ;
#31922=CARTESIAN_POINT ( 'NONE',  ( 9.980591063997303891, -1.864246421445880042, -99.99999999999995737 ) ) ;
#31924=CARTESIAN_POINT ( 'NONE',  ( -5.405949406250003975, -9.363379034771801557, -165.5312500020484094 ) ) ;
#31929=CARTESIAN_POINT ( 'NONE',  ( 10.81189881249999907, 6.242252689847868297, -82.21875000204836681 ) ) ;
#31930=CARTESIAN_POINT ( 'NONE',  ( -5.405949406250003975, -9.363379034771801557, -190.8437500020484094 ) ) ;
#31931=CARTESIAN_POINT ( 'NONE',  ( -10.81189881249999907, -6.242252689847864744, -93.65625000204840944 ) ) ;
#31935=CARTESIAN_POINT ( 'NONE',  ( 10.81189881249999729, 6.242252689847867408, -173.9062500020483810 ) ) ;
#31936=CARTESIAN_POINT ( 'NONE',  ( -2.293366432827344421E-15, -12.48450537969573659, -186.4062500020484094 ) ) ;
#31938=CARTESIAN_POINT ( 'NONE',  ( -9.999999999999998224, 1.224646799147353059E-15, -166.6250000040967905 ) ) ;
#31940=CARTESIAN_POINT ( 'NONE',  ( -10.81189881249999729, 6.242252689847871849, -11.21875000204835970 ) ) ;
#31941=CARTESIAN_POINT ( 'NONE',  ( 7.644554776091147741E-16, 12.48450537969573659, -123.9687500020483952 ) ) ;
#31943=CARTESIAN_POINT ( 'NONE',  ( -10.81189881249999907, -6.242252689847864744, -18.65625000204837747 ) ) ;
#31946=CARTESIAN_POINT ( 'NONE',  ( 5.405949406249999534, 9.363379034771803333, -115.2812500020483952 ) ) ;
#31948=ORIENTED_EDGE ( 'NONE', *, *, #13997, .T. ) ;
#31949=CARTESIAN_POINT ( 'NONE',  ( -2.121150477449813534E-15, -11.54700538379251284, -88.25000000409677625 ) ) ;
#31952=CARTESIAN_POINT ( 'NONE',  ( 10.81189881249999907, 6.242252689847868297, -50.71875000204837391 ) ) ;
#31957=CARTESIAN_POINT ( 'NONE',  ( -10.00000000000000000, -5.773502691896251982, -16.50000000409676559 ) ) ;
#31958=DIRECTION ( 'NONE',  ( 0.000000000000000000, 0.000000000000000000, -1.000000000000000000 ) ) ;
#31972=CARTESIAN_POINT ( 'NONE',  ( -10.81189881249999729, 6.242252689847871849, -188.4062500020484094 ) ) ;
#31978=CARTESIAN_POINT ( 'NONE',  ( 10.81189881249999907, 6.242252689847868297, -112.2187500020483810 ) ) ;
#31980=CARTESIAN_POINT ( 'NONE',  ( 10.81189881249999907, 6.242252689847868297, -113.9062500020483952 ) ) ;
#31982=CARTESIAN_POINT ( 'NONE',  ( -10.81189881249999729, 6.242252689847871849, -120.7187500020483952 ) ) ;
#31985=CARTESIAN_POINT ( 'NONE',  ( 4.999999999999992006, -8.660254037844389075, -140.2500000000000000 ) ) ;
#31986=CARTESIAN_POINT ( 'NONE',  ( -9.999999999999998224, 5.773502691896259087, -14.87499999999997335 ) ) ;
#31989=CARTESIAN_POINT ( 'NONE',  ( 9.999999999999998224, 0.000000000000000000, -191.3750000040967905 ) ) ;
#31991=CARTESIAN_POINT ( 'NONE',  ( 10.81189881249999907, 6.242252689847868297, -35.71875000204835970 ) ) ;
#31993=CARTESIAN_POINT ( 'NONE',  ( 5.405949406249992428, -9.363379034771808662, -148.5937500020483810 ) ) ;
#31995=CARTESIAN_POINT ( 'NONE',  ( -10.00000000000051337, 5.773502691895962435, -145.3750000000000000 ) ) ;
#31996=CARTESIAN_POINT ( 'NONE',  ( -9.999999999999998224, 1.224646799147353059E-15, -79.24999999999998579 ) ) ;
#31997=CARTESIAN_POINT ( 'NONE',  ( 10.81189881249999729, 0.000000000000000000, -136.5312500020484094 ) ) ;
#32001=CARTESIAN_POINT ( 'NONE',  ( -10.00000000000000000, -5.773502691896251982, -112.5000000040967905 ) ) ;
#32003=CARTESIAN_POINT ( 'NONE',  ( -10.81189881249999907, -6.242252689847864744, -73.96875000204836681 ) ) ;
#32007=CARTESIAN_POINT ( 'NONE',  ( -35.00000000000000711, 0.000000000000000000, -169.9999999999999716 ) ) ;
#32008=CARTESIAN_POINT ( 'NONE',  ( -2.293366432827344421E-15, -12.48450537969573659, -34.90625000204835970 ) ) ;
#32014=VERTEX_POINT ( 'NONE', #29045 ) ;
#32016=ORIENTED_EDGE ( 'NONE', *, *, #32342, .F. ) ;
#32025=CARTESIAN_POINT ( 'NONE',  ( -5.405949406249996869, 9.363379034771805109, -131.3437500020484094 ) ) ;
#32026=CARTESIAN_POINT ( 'NONE',  ( 5.405949406249992428, -9.363379034771808662, -136.7812500020483810 ) ) ;
#32027=CARTESIAN_POINT ( 'NONE',  ( 5.000000000000000000, 8.660254037844385522, -144.2500000000000000 ) ) ;
#32028=CARTESIAN_POINT ( 'NONE',  ( 10.81189881249999551, -6.242252689847874514, -146.9687500020484094 ) ) ;
#32032=CARTESIAN_POINT ( 'NONE',  ( -4.999999999999996447, 8.660254037844387298, -171.0000000000000000 ) ) ;
#32036=CARTESIAN_POINT ( 'NONE',  ( -8.408428485261246976, 6.678869664728471101, -100.0000000000000000 ) ) ;
#32037=CARTESIAN_POINT ( 'NONE',  ( -2.293366432827344421E-15, -12.48450537969573659, -171.2187500020484094 ) ) ;
#32042=CARTESIAN_POINT ( 'NONE',  ( -5.405949406250003975, -9.363379034771801557, -36.53125000204837391 ) ) ;
#32044=CARTESIAN_POINT ( 'NONE',  ( -9.999999999999998224, 5.773502691896259087, -100.3750000000000000 ) ) ;
#32045=ORIENTED_EDGE ( 'NONE', *, *, #35749, .F. ) ;
#32046=CARTESIAN_POINT ( 'NONE',  ( -5.405949406249996869, 9.363379034771805109, -121.0312500020483952 ) ) ;
#32047=CARTESIAN_POINT ( 'NONE',  ( 5.000000000000000000, 8.660254037844385522, -140.1250000040967905 ) ) ;
#32053=CARTESIAN_POINT ( 'NONE',  ( -10.81189881249999907, -6.242252689847864744, -59.15625000204838102 ) ) ;
#32059=CARTESIAN_POINT ( 'NONE',  ( 9.999999999999998224, 0.000000000000000000, -173.3750000040968189 ) ) ;
#32064=CARTESIAN_POINT ( 'NONE',  ( 9.999999999999998224, 1.224646799147353059E-15, -99.99999999999998579 ) ) ;
#32065=ORIENTED_EDGE ( 'NONE', *, *, #3533, .F. ) ;
#32071=ORIENTED_EDGE ( 'NONE', *, *, #12806, .T. ) ;
#32073=CARTESIAN_POINT ( 'NONE',  ( -9.999999999999998224, 1.224646799147353059E-15, -35.74999999999997868 ) ) ;
#32076=CARTESIAN_POINT ( 'NONE',  ( -5.405949406249996869, 9.363379034771805109, -159.8437500020484094 ) ) ;
#32077=CARTESIAN_POINT ( 'NONE',  ( 10.81189881249999729, 0.000000000000000000, -173.8437500020484094 ) ) ;
#32079=VECTOR ( 'NONE', #12847, 1000.000000000000000 ) ;
#32080=CARTESIAN_POINT ( 'NONE',  ( -9.999999999999998224, 0.000000000000000000, -99.99999999999998579 ) ) ;
#32081=CARTESIAN_POINT ( 'NONE',  ( 9.999999999999996447, -5.773502691896262640, -192.6250000000000284 ) ) ;
#32086=CARTESIAN_POINT ( 'NONE',  ( 10.81189881249999729, 0.000000000000000000, -58.53125000204836681 ) ) ;
#32088=CARTESIAN_POINT ( 'NONE',  ( -4.999999999999996447, 8.660254037844387298, -124.5000000000000000 ) ) ;
#32090=EDGE_LOOP ( 'NONE', ( #3183, #10581, #26160, #23925 ) ) ;
#32091=CARTESIAN_POINT ( 'NONE',  ( 10.81189881249999551, -6.242252689847874514, -142.6562500020484094 ) ) ;
#32092=CARTESIAN_POINT ( 'NONE',  ( 10.81189881249999729, 0.000000000000000000, -159.0312500020484094 ) ) ;
#32096=CARTESIAN_POINT ( 'NONE',  ( 5.405949406249999534, 9.363379034771803333, -88.09375000204836681 ) ) ;
#32099=CARTESIAN_POINT ( 'NONE',  ( -10.81189881249999907, -6.242252689847864744, -192.4687500020484094 ) ) ;
#32101=CARTESIAN_POINT ( 'NONE',  ( 5.000000000000000000, 8.660254037844385522, -165.2500000000000000 ) ) ;
#32102=CARTESIAN_POINT ( 'NONE',  ( 9.999999999999998224, 0.000000000000000000, -117.5000000000000000 ) ) ;
#32103=CARTESIAN_POINT ( 'NONE',  ( 10.81189881249999907, 6.242252689847868297, -88.40625000204839523 ) ) ;
#32106=CARTESIAN_POINT ( 'NONE',  ( 4.999999999999992006, -8.660254037844389075, -65.62500000409676204 ) ) ;
#32108=CARTESIAN_POINT ( 'NONE',  ( 7.644554776091147741E-16, 12.48450537969573659, -29.46875000204835260 ) ) ;
#32111=CARTESIAN_POINT ( 'NONE',  ( -5.405949406250003975, -9.363379034771801557, -20.03125000204836326 ) ) ;
#32127=DIRECTION ( 'NONE',  ( -0.000000000000000000, -0.000000000000000000, -1.000000000000000000 ) ) ;
#32133=CARTESIAN_POINT ( 'NONE',  ( -10.81189881249999907, -6.242252689847864744, -156.6562500020483810 ) ) ;
#32139=CARTESIAN_POINT ( 'NONE',  ( -5.405949406250003975, -9.363379034771801557, -73.84375000204838102 ) ) ;
#32140=CARTESIAN_POINT ( 'NONE',  ( -10.81189881249999729, 6.242252689847871849, -84.90625000204838102 ) ) ;
#32143=CARTESIAN_POINT ( 'NONE',  ( -2.293366432827344421E-15, -12.48450537969573659, -168.4062500020484379 ) ) ;
#32144=CARTESIAN_POINT ( 'NONE',  ( -5.405949406249996869, 9.363379034771805109, -188.5312500020484094 ) ) ;
#32146=CARTESIAN_POINT ( 'NONE',  ( 5.000000000000000000, 8.660254037844385522, -164.1250000040967905 ) ) ;
#32148=CARTESIAN_POINT ( 'NONE',  ( -10.81189881249999907, -6.242252689847864744, -16.96875000204836681 ) ) ;
#32150=CARTESIAN_POINT ( 'NONE',  ( 7.644554776091147741E-16, 12.48450537969573659, -117.9687500020483668 ) ) ;
#32152=CARTESIAN_POINT ( 'NONE',  ( -10.81189881249999729, 1.324075727343319199E-15, -21.78125000204836326 ) ) ;
#32155=CARTESIAN_POINT ( 'NONE',  ( -5.405949406250003975, -9.363379034771801557, -113.0312500020483952 ) ) ;
#32158=CARTESIAN_POINT ( 'NONE',  ( 9.999999999999996447, -5.773502691896262640, -94.00000000409677625 ) ) ;
#32161=CARTESIAN_POINT ( 'NONE',  ( 10.81189881249999729, 0.000000000000000000, -53.84375000204835970 ) ) ;
#32166=CARTESIAN_POINT ( 'NONE',  ( 5.000000000000000000, 8.660254037844385522, -18.62500000409675494 ) ) ;
#32168=ADVANCED_FACE ( 'NONE', ( #8766 ), #19107, .F. ) ;
#32173=EDGE_LOOP ( 'NONE', ( #32045, #41549, #7728, #15784 ) ) ;
#32182=CARTESIAN_POINT ( 'NONE',  ( -10.81189881249999729, 6.242252689847871849, -182.4062500020483810 ) ) ;
#32184=DIRECTION ( 'NONE',  ( -0.000000000000000000, -0.000000000000000000, -1.000000000000000000 ) ) ;
#32187=CARTESIAN_POINT ( 'NONE',  ( 7.644554776091147741E-16, 12.48450537969573659, -105.9687500020483668 ) ) ;
#32188=CARTESIAN_POINT ( 'NONE',  ( -2.121150477449813534E-15, -11.54700538379251284, -143.3750000000000000 ) ) ;
#32189=CARTESIAN_POINT ( 'NONE',  ( -10.81189881249999729, 1.324075727343319199E-15, -113.2812500020483952 ) ) ;
#32191=CARTESIAN_POINT ( 'NONE',  ( -10.81189881249999729, 6.242252689847871849, -119.2187500020483810 ) ) ;
#32194=CARTESIAN_POINT ( 'NONE',  ( -9.999999999999998224, 1.224646799147353059E-15, -136.2499999999999716 ) ) ;
#32195=CARTESIAN_POINT ( 'NONE',  ( -10.00000000000000000, -5.773502691896251982, -13.12499999999997158 ) ) ;
#32198=CARTESIAN_POINT ( 'NONE',  ( -10.00000000000000000, -5.773502691896251982, -192.0000000040968189 ) ) ;
#32200=CARTESIAN_POINT ( 'NONE',  ( 5.405949406249992428, -9.363379034771808662, -37.59375000204837391 ) ) ;
#32201=CARTESIAN_POINT ( 'NONE',  ( 4.999999999999992006, -8.660254037844389075, -142.1250000040967905 ) ) ;
#32202=CARTESIAN_POINT ( 'NONE',  ( -5.405949406250003975, -9.363379034771801557, -147.3437500020483810 ) ) ;
#32204=DIRECTION ( 'NONE',  ( -0.000000000000000000, -0.000000000000000000, -1.000000000000000000 ) ) ;
#32205=CARTESIAN_POINT ( 'NONE',  ( -10.00000000000000000, -5.773502691896251982, -70.12500000000000000 ) ) ;
#32206=CARTESIAN_POINT ( 'NONE',  ( 10.81189881249999729, 0.000000000000000000, -142.5312500020483810 ) ) ;
#32210=CARTESIAN_POINT ( 'NONE',  ( -9.999999999999998224, 5.773502691896259087, -118.7500000040967905 ) ) ;
#32212=CARTESIAN_POINT ( 'NONE',  ( -10.81189881249999907, -6.242252689847864744, -70.96875000204838102 ) ) ;
#32216=CARTESIAN_POINT ( 'NONE',  ( 10.00000000000025402, -5.773502691896113426, -157.0000000040968189 ) ) ;
#32217=CARTESIAN_POINT ( 'NONE',  ( 10.81189881249999729, 0.000000000000000000, -36.03125000204837391 ) ) ;
#32222=CARTESIAN_POINT ( 'NONE',  ( 5.000000000000000000, 8.660254037844385522, -153.2500000000000000 ) ) ;
#32235=CARTESIAN_POINT ( 'NONE',  ( 10.81189881249999551, -6.242252689847874514, -134.9687500020483810 ) ) ;
#32236=CARTESIAN_POINT ( 'NONE',  ( 7.644554776091147741E-16, 12.48450537969573659, -143.6562500020484094 ) ) ;
#32238=CARTESIAN_POINT ( 'NONE',  ( 10.81189881249999551, -6.242252689847874514, -143.9687500020484094 ) ) ;
#32240=CARTESIAN_POINT ( 'NONE',  ( -4.999999999999996447, 8.660254037844387298, -166.5000000000000000 ) ) ;
#32242=CARTESIAN_POINT ( 'NONE',  ( -2.121150477449813534E-15, -11.54700538379251284, -114.8749999999999716 ) ) ;
#32244=CARTESIAN_POINT ( 'NONE',  ( 10.81189881249999551, -6.242252689847874514, -64.46875000204838102 ) ) ;
#32245=CARTESIAN_POINT ( 'NONE',  ( -5.000000000000003553, -8.660254037844383745, -175.0000000000000284 ) ) ;
#32246=CARTESIAN_POINT ( 'NONE',  ( 10.81189881249999729, 0.000000000000000000, -169.3437500020484094 ) ) ;
#32251=CARTESIAN_POINT ( 'NONE',  ( -5.000000000000003553, -8.660254037844383745, -89.49999999999998579 ) ) ;
#32253=CARTESIAN_POINT ( 'NONE',  ( -10.81189881249999729, 1.324075727343319199E-15, -119.2812500020483952 ) ) ;
#32254=CARTESIAN_POINT ( 'NONE',  ( -5.000000000000003553, -8.660254037844383745, -137.8750000040967905 ) ) ;
#32259=CARTESIAN_POINT ( 'NONE',  ( -2.293366432827344421E-15, -12.48450537969573659, -61.90625000204838813 ) ) ;
#32282=DIRECTION ( 'NONE',  ( -1.000000000000000000, 0.000000000000000000, 0.000000000000000000 ) ) ;
#32283=CARTESIAN_POINT ( 'NONE',  ( -2.121150477449813534E-15, -11.54700538379251284, -27.87499999999998224 ) ) ;
#32284=EDGE_CURVE ( 'NONE', #11758, #21425, #16904, .T. ) ;
#32287=CARTESIAN_POINT ( 'NONE',  ( -10.81189881249999729, 1.324075727343319199E-15, -156.5937500020483810 ) ) ;
#32288=CARTESIAN_POINT ( 'NONE',  ( -10.81189881249999729, 1.324075727343319199E-15, -173.0937500020484094 ) ) ;
#32290=DIRECTION ( 'NONE',  ( -1.000000000000000000, 0.000000000000000000, 0.000000000000000000 ) ) ;
#32292=CARTESIAN_POINT ( 'NONE',  ( -2.121150477449813534E-15, -11.54700538379251284, -183.8750000000000284 ) ) ;
#32301=CARTESIAN_POINT ( 'NONE',  ( 7.644554776091147741E-16, 12.48450537969573659, -61.15625000204838102 ) ) ;
#32303=CARTESIAN_POINT ( 'NONE',  ( -5.000000000000003553, -8.660254037844383745, -125.5000000000000000 ) ) ;
#32304=VERTEX_POINT ( 'NONE', #19519 ) ;
#32305=CARTESIAN_POINT ( 'NONE',  ( 7.644554776091147741E-16, 12.48450537969573659, -140.6562500020484094 ) ) ;
#32306=CARTESIAN_POINT ( 'NONE',  ( 10.81189881249999729, 0.000000000000000000, -156.0312500020484094 ) ) ;
#32309=CARTESIAN_POINT ( 'NONE',  ( -10.81189881249999907, -6.242252689847864744, -88.96875000204836681 ) ) ;
#32312=CARTESIAN_POINT ( 'NONE',  ( -10.81189881249999729, 6.242252689847871849, -191.2187500020484663 ) ) ;
#32314=LINE ( 'NONE', #42416, #32079 ) ;
#32315=CARTESIAN_POINT ( 'NONE',  ( 9.999999999999998224, 0.000000000000000000, -123.5000000000000000 ) ) ;
#32316=CARTESIAN_POINT ( 'NONE',  ( 5.405949406249992428, -9.363379034771808662, -87.28125000204838102 ) ) ;
#32318=CARTESIAN_POINT ( 'NONE',  ( 4.999999999999992006, -8.660254037844389075, -61.12500000409676204 ) ) ;
#32319=CARTESIAN_POINT ( 'NONE',  ( 10.81189881249999907, 6.242252689847868297, -14.71875000204836326 ) ) ;
#32322=CARTESIAN_POINT ( 'NONE',  ( 10.81189881249999551, -6.242252689847874514, -9.156250002048365033 ) ) ;
#32324=CARTESIAN_POINT ( 'NONE',  ( -9.999999999999998224, 1.224646799147353059E-15, -136.6250000040967620 ) ) ;
#32325=CARTESIAN_POINT ( 'NONE',  ( -10.00000000000000000, -5.773502691896251982, -4.096750716442443263E-09 ) ) ;
#32330=EDGE_CURVE ( 'NONE', #15832, #5830, #18837, .T. ) ;
#32333=CARTESIAN_POINT ( 'NONE',  ( -5.000000000000003553, -8.660254037844383745, -179.8750000040967905 ) ) ;
#32341=CARTESIAN_POINT ( 'NONE',  ( 22.00000000000000711, 2.694222958124177598E-15, -99.99999999999998579 ) ) ;
#32342=EDGE_CURVE ( 'NONE', #22977, #29817, #14134, .T. ) ;
#32346=CARTESIAN_POINT ( 'NONE',  ( 5.405949406249999534, 9.363379034771803333, -158.7812500020484094 ) ) ;
#32352=CARTESIAN_POINT ( 'NONE',  ( -5.405949406249996869, 9.363379034771805109, -77.34375000204838102 ) ) ;
#32353=CARTESIAN_POINT ( 'NONE',  ( 7.644554776091147741E-16, 12.48450537969573659, -82.15625000204838102 ) ) ;
#32355=( BOUNDED_CURVE ( )  B_SPLINE_CURVE ( 2, ( #30819, #4693, #1257, #4914, #27146, #40715, #18062 ),
 .UNSPECIFIED., .F., .F. ) 
 B_SPLINE_CURVE_WITH_KNOTS ( ( 3, 2, 2, 3 ),
 ( 0.4029850746268657802, 0.4042288557213931655, 0.4054726368159204397, 0.4067164179104478250 ),
 .UNSPECIFIED. ) 
 CURVE ( )  GEOMETRIC_REPRESENTATION_ITEM ( )  RATIONAL_B_SPLINE_CURVE ( ( 0.9999999999999880096, 0.8660254037844506980, 1.000000000000000000, 0.8660254037844387076, 1.000000000000000000, 0.8660254037844327124, 1.000000000000005995 ) ) 
 REPRESENTATION_ITEM ( '' )  );
#32357=CARTESIAN_POINT ( 'NONE',  ( -10.81189881249999729, 6.242252689847871849, -167.4062500020484094 ) ) ;
#32358=CARTESIAN_POINT ( 'NONE',  ( 10.81189881249999907, 6.242252689847868297, -178.4062500020484094 ) ) ;
#32359=CARTESIAN_POINT ( 'NONE',  ( -2.121150477449813534E-15, -11.54700538379251284, -152.7500000040967620 ) ) ;
#32361=CARTESIAN_POINT ( 'NONE',  ( 10.81189881249999729, 0.000000000000000000, -4.343750002048368586 ) ) ;
#32363=CARTESIAN_POINT ( 'NONE',  ( 7.644554776091147741E-16, 12.48450537969573659, -110.4687500020483668 ) ) ;
#32365=CARTESIAN_POINT ( 'NONE',  ( -5.405949406249996869, 9.363379034771805109, -16.03125000204835970 ) ) ;
#32367=CARTESIAN_POINT ( 'NONE',  ( -9.999999999999998224, 1.224646799147353059E-15, -171.1250000040968189 ) ) ;
#32368=CARTESIAN_POINT ( 'NONE',  ( -10.81189881249999729, 6.242252689847871849, -110.4062500020483810 ) ) ;
#32371=CARTESIAN_POINT ( 'NONE',  ( -4.999999999999996447, 8.660254037844387298, -81.37500000409677625 ) ) ;
#32373=CARTESIAN_POINT ( 'NONE',  ( -10.81189881249999729, 1.324075727343319199E-15, -39.59375000204837391 ) ) ;
#32378=CARTESIAN_POINT ( 'NONE',  ( 7.070501591499377789E-16, 11.54700538379251284, -18.50000000409676559 ) ) ;
#32384=ORIENTED_EDGE ( 'NONE', *, *, #24919, .F. ) ;
#32387=EDGE_CURVE ( 'NONE', #3006, #6776, #22774, .T. ) ;
#32393=CARTESIAN_POINT ( 'NONE',  ( -2.293366432827344421E-15, -12.48450537969573659, -181.9062500020483810 ) ) ;
#32394=CARTESIAN_POINT ( 'NONE',  ( 9.999999999999998224, 1.224646799147353059E-15, -99.99999999999998579 ) ) ;
#32398=CARTESIAN_POINT ( 'NONE',  ( -10.81189881249999907, -6.242252689847864744, -97.96875000204838102 ) ) ;
#32400=CARTESIAN_POINT ( 'NONE',  ( -10.81189881249999729, 6.242252689847871849, -107.4062500020483810 ) ) ;
#32402=CARTESIAN_POINT ( 'NONE',  ( -5.405949406250003975, -9.363379034771801557, -126.3437500020483952 ) ) ;
#32406=CARTESIAN_POINT ( 'NONE',  ( 9.999999999999996447, -5.773502691896262640, -137.1250000000000000 ) ) ;
#32407=CARTESIAN_POINT ( 'NONE',  ( 4.999999999999992006, -8.660254037844389075, -0.7499999999999729106 ) ) ;
#32410=CARTESIAN_POINT ( 'NONE',  ( -9.999999999999998224, 5.773502691896259087, -177.2500000040967905 ) ) ;
#32412=CARTESIAN_POINT ( 'NONE',  ( 7.644554776091147741E-16, 12.48450537969573659, -32.46875000204835260 ) ) ;
#32413=CARTESIAN_POINT ( 'NONE',  ( 9.999999999999998224, 0.000000000000000000, -109.9999999999999858 ) ) ;
#32414=CARTESIAN_POINT ( 'NONE',  ( 7.644554776091147741E-16, 12.48450537969573659, -138.9687500020484094 ) ) ;
#32417=CARTESIAN_POINT ( 'NONE',  ( -10.00000000000000000, -5.773502691896251982, -67.12499999999998579 ) ) ;
#32418=CARTESIAN_POINT ( 'NONE',  ( -5.405949406249996869, 9.363379034771805109, -142.0312500020483810 ) ) ;
#32421=CARTESIAN_POINT ( 'NONE',  ( 9.999999999999998224, 0.000000000000000000, -120.8750000040967905 ) ) ;
#32422=CARTESIAN_POINT ( 'NONE',  ( 10.00000000000000000, 5.773502691896255534, -116.2500000040967905 ) ) ;
#32423=CARTESIAN_POINT ( 'NONE',  ( -5.405949406250003975, -9.363379034771801557, -72.34375000204836681 ) ) ;
#32427=( BOUNDED_CURVE ( )  B_SPLINE_CURVE ( 2, ( #14431, #40764, #40336, #11206, #20285, #20923, #23967 ),
 .UNSPECIFIED., .F., .F. ) 
 B_SPLINE_CURVE_WITH_KNOTS ( ( 3, 2, 2, 3 ),
 ( 0.4850746268656717652, 0.4863184079601990950, 0.4875621890547264248, 0.4888059701492538101 ),
 .UNSPECIFIED. ) 
 CURVE ( )  GEOMETRIC_REPRESENTATION_ITEM ( )  RATIONAL_B_SPLINE_CURVE ( ( 0.9999999999999880096, 0.8660254037844506980, 1.000000000000000000, 0.8660254037844387076, 1.000000000000000000, 0.8660254037844327124, 1.000000000000005995 ) ) 
 REPRESENTATION_ITEM ( '' )  );
#32429=CARTESIAN_POINT ( 'NONE',  ( 9.999999999999996447, -5.773502691896262640, -44.50000000409676915 ) ) ;
#32430=CARTESIAN_POINT ( 'NONE',  ( 10.81189881249999907, 6.242252689847868297, -32.90625000204835970 ) ) ;
#32431=CARTESIAN_POINT ( 'NONE',  ( 9.999999999999998224, 0.000000000000000000, -167.0000000000000000 ) ) ;
#32443=CARTESIAN_POINT ( 'NONE',  ( 7.070501591499376803E-16, 11.54700538379251284, -111.5000000040967763 ) ) ;
#32448=CARTESIAN_POINT ( 'NONE',  ( -5.405949406249996869, 9.363379034771805109, -128.3437500020484094 ) ) ;
#32449=CARTESIAN_POINT ( 'NONE',  ( 10.81189881249999551, -6.242252689847874514, -135.1562500020484094 ) ) ;
#32451=CARTESIAN_POINT ( 'NONE',  ( 5.405949406249992428, -9.363379034771808662, -147.0937500020483810 ) ) ;
#32453=CARTESIAN_POINT ( 'NONE',  ( -4.999999999999996447, 8.660254037844387298, -141.3750000040967905 ) ) ;
#32454=CARTESIAN_POINT ( 'NONE',  ( -10.00000000000000000, -5.773502691896251982, -164.6249999999999716 ) ) ;
#32455=FACE_OUTER_BOUND ( 'NONE', #18670, .T. ) ;
#32458=CARTESIAN_POINT ( 'NONE',  ( -10.81189881249999729, 6.242252689847871849, -63.71875000204838102 ) ) ;
#32459=LINE ( 'NONE', #38919, #18541 ) ;
#32460=CARTESIAN_POINT ( 'NONE',  ( -5.405949406249996869, 9.363379034771805109, -161.3437500020484094 ) ) ;
#32461=VECTOR ( 'NONE', #33108, 1000.000000000000000 ) ;
#32464=LINE ( 'NONE', #26610, #4112 ) ;
#32466=CARTESIAN_POINT ( 'NONE',  ( -5.000000000000003553, -8.660254037844383745, -93.99999999999998579 ) ) ;
#32467=( BOUNDED_CURVE ( )  B_SPLINE_CURVE ( 2, ( #347, #13469, #26661, #20178, #3788, #36579, #32930 ),
 .UNSPECIFIED., .F., .F. ) 
 B_SPLINE_CURVE_WITH_KNOTS ( ( 3, 2, 2, 3 ),
 ( 0.3694029850746270438, 0.3706467661691543181, 0.3718905472636817033, 0.3731343283582090331 ),
 .UNSPECIFIED. ) 
 CURVE ( )  GEOMETRIC_REPRESENTATION_ITEM ( )  RATIONAL_B_SPLINE_CURVE ( ( 0.9999999999999820144, 0.8660254037844566932, 1.000000000000000000, 0.8660254037844387076, 1.000000000000000000, 0.8660254037844327124, 1.000000000000005995 ) ) 
 REPRESENTATION_ITEM ( '' )  );
#32469=CARTESIAN_POINT ( 'NONE',  ( -5.405949406250003975, -9.363379034771801557, -119.0312500020483952 ) ) ;
#32470=CARTESIAN_POINT ( 'NONE',  ( -10.00000000000000000, -5.773502691896251982, -141.0000000040967905 ) ) ;
#32475=CARTESIAN_POINT ( 'NONE',  ( 10.81189881249999729, 0.000000000000000000, -58.53125000204836681 ) ) ;
#32494=CARTESIAN_POINT ( 'NONE',  ( 4.999999999999992006, -8.660254037844389075, -27.74999999999996803 ) ) ;
#32497=CARTESIAN_POINT ( 'NONE',  ( 10.81189881249999551, -6.242252689847874514, -154.4687500020484094 ) ) ;
#32498=CARTESIAN_POINT ( 'NONE',  ( -5.405949406250003975, -9.363379034771801557, -174.3437500020484094 ) ) ;
#32500=CARTESIAN_POINT ( 'NONE',  ( 9.999999999999996447, -5.773502691896262640, -189.6250000000000000 ) ) ;
#32504=LINE ( 'NONE', #29051, #24036 ) ;
#32508=CARTESIAN_POINT ( 'NONE',  ( 5.405949406249992428, -9.363379034771808662, -57.28125000204836681 ) ) ;
#32510=CARTESIAN_POINT ( 'NONE',  ( 10.00000000000000000, 5.773502691896255534, -114.3750000000000000 ) ) ;
#32511=ORIENTED_EDGE ( 'NONE', *, *, #6065, .F. ) ;
#32512=CARTESIAN_POINT ( 'NONE',  ( 10.81189881249999551, -6.242252689847874514, -144.1562500020484094 ) ) ;
#32513=CARTESIAN_POINT ( 'NONE',  ( 7.644554776091147741E-16, 12.48450537969573659, -155.6562500020484094 ) ) ;
#32516=CARTESIAN_POINT ( 'NONE',  ( -5.000000000000003553, -8.660254037844383745, -179.5000000000000000 ) ) ;
#32517=CARTESIAN_POINT ( 'NONE',  ( 5.405949406249999534, 9.363379034771803333, -89.59375000204838102 ) ) ;
#32518=ORIENTED_EDGE ( 'NONE', *, *, #13460, .F. ) ;
#32520=CARTESIAN_POINT ( 'NONE',  ( 10.81189881249999551, -6.242252689847874514, -191.9687500020484379 ) ) ;
#32524=CARTESIAN_POINT ( 'NONE',  ( 5.405949406249992428, -9.363379034771808662, -82.78125000204838102 ) ) ;
#32526=CARTESIAN_POINT ( 'NONE',  ( 7.070501591499377789E-16, 11.54700538379251284, -60.50000000409677625 ) ) ;
#32527=CARTESIAN_POINT ( 'NONE',  ( 10.81189881249999907, 6.242252689847868297, -16.21875000204836326 ) ) ;
#32528=LINE ( 'NONE', #2957, #21413 ) ;
#32531=CARTESIAN_POINT ( 'NONE',  ( 5.405949406249999534, 9.363379034771803333, -11.78125000204835438 ) ) ;
#32547=CARTESIAN_POINT ( 'NONE',  ( 0.000000000000000000, 0.000000000000000000, -180.0000000000000000 ) ) ;
#32550=CARTESIAN_POINT ( 'NONE',  ( 9.999999999999998224, 0.000000000000000000, -159.8750000040967905 ) ) ;
#32552=CARTESIAN_POINT ( 'NONE',  ( -5.405949406250003975, -9.363379034771801557, -155.0312500020484094 ) ) ;
#32554=AXIS2_PLACEMENT_3D ( 'NONE', #14114, #18007, #7676 ) ;
#32560=CARTESIAN_POINT ( 'NONE',  ( -5.405949406249996869, 9.363379034771805109, -78.84375000204838102 ) ) ;
#32561=CARTESIAN_POINT ( 'NONE',  ( -10.81189881249999729, 1.324075727343319199E-15, -84.78125000204838102 ) ) ;
#32565=CARTESIAN_POINT ( 'NONE',  ( 10.81189881249999729, 0.000000000000000000, -165.0312500020484094 ) ) ;
#32566=CARTESIAN_POINT ( 'NONE',  ( -10.81189881249999729, 6.242252689847871849, -177.9062500020484094 ) ) ;
#32568=CARTESIAN_POINT ( 'NONE',  ( -9.999999999999998224, 5.773502691896259087, -156.2500000040967905 ) ) ;
#32570=CARTESIAN_POINT ( 'NONE',  ( -10.81189881249999907, -6.242252689847864744, -7.968750002048358816 ) ) ;
#32572=CARTESIAN_POINT ( 'NONE',  ( 10.81189881249999729, 0.000000000000000000, -116.8437500020483810 ) ) ;
#32574=CARTESIAN_POINT ( 'NONE',  ( -5.405949406249996869, 9.363379034771805109, -14.53125000204835615 ) ) ;
#32578=CARTESIAN_POINT ( 'NONE',  ( -5.405949406249996869, 9.363379034771805109, -106.0312500020483810 ) ) ;
#32580=ORIENTED_EDGE ( 'NONE', *, *, #21185, .F. ) ;
#32582=CARTESIAN_POINT ( 'NONE',  ( -10.00000000000000000, -5.773502691896251982, -85.50000000409677625 ) ) ;
#32584=CARTESIAN_POINT ( 'NONE',  ( -10.81189881249999729, 1.324075727343319199E-15, -45.59375000204838102 ) ) ;
#32588=CARTESIAN_POINT ( 'NONE',  ( 5.000000000000000000, 8.660254037844385522, -15.62500000409675138 ) ) ;
#32589=VECTOR ( 'NONE', #18761, 1000.000000000000000 ) ;
#32595=( BOUNDED_CURVE ( )  B_SPLINE_CURVE ( 2, ( #30217, #4301, #14192, #30636, #10759, #17652, #29999 ),
 .UNSPECIFIED., .F., .F. ) 
 B_SPLINE_CURVE_WITH_KNOTS ( ( 3, 2, 2, 3 ),
 ( 0.4253731343283583266, 0.4266169154228856564, 0.4278606965174130417, 0.4291044776119404269 ),
 .UNSPECIFIED. ) 
 CURVE ( )  GEOMETRIC_REPRESENTATION_ITEM ( )  RATIONAL_B_SPLINE_CURVE ( ( 0.9999999999999880096, 0.8660254037844506980, 1.000000000000000000, 0.8660254037844387076, 1.000000000000000000, 0.8660254037844267172, 1.000000000000011990 ) ) 
 REPRESENTATION_ITEM ( '' )  );
#32604=CARTESIAN_POINT ( 'NONE',  ( -5.405949406250003975, -9.363379034771801557, -177.5312500020483810 ) ) ;
#32606=CARTESIAN_POINT ( 'NONE',  ( 9.999999999999998224, 0.000000000000000000, -155.3750000040967905 ) ) ;
#32608=CARTESIAN_POINT ( 'NONE',  ( -10.81189881249999907, -6.242252689847864744, -105.4687500020483668 ) ) ;
#32610=CARTESIAN_POINT ( 'NONE',  ( 10.81189881249999551, -6.242252689847874514, -111.1562500020483952 ) ) ;
#32612=CARTESIAN_POINT ( 'NONE',  ( -2.293366432827344421E-15, -12.48450537969573659, -114.2187500020483668 ) ) ;
#32615=CARTESIAN_POINT ( 'NONE',  ( -4.999999999999996447, 8.660254037844387298, -136.5000000000000000 ) ) ;
#32616=CARTESIAN_POINT ( 'NONE',  ( 9.999999999999996447, -5.773502691896262640, -8.124999999999966249 ) ) ;
#32619=CARTESIAN_POINT ( 'NONE',  ( -9.999999999999998224, 5.773502691896259087, -183.2500000040968189 ) ) ;
#32621=CARTESIAN_POINT ( 'NONE',  ( -5.405949406249996869, 9.363379034771805109, -29.34375000204836326 ) ) ;
#32622=CARTESIAN_POINT ( 'NONE',  ( -2.121150477449813534E-15, -11.54700538379251284, -142.2500000040967905 ) ) ;
#32623=CARTESIAN_POINT ( 'NONE',  ( 10.81189881249999729, 0.000000000000000000, -139.3437500020484094 ) ) ;
#32625=CARTESIAN_POINT ( 'NONE',  ( -9.999999999999998224, 1.224646799147353059E-15, -110.7499999999999858 ) ) ;
#32626=CARTESIAN_POINT ( 'NONE',  ( -5.000000000000003553, -8.660254037844383745, -66.99999999999997158 ) ) ;
#32627=CARTESIAN_POINT ( 'NONE',  ( 7.644554776091147741E-16, 12.48450537969573659, -133.1562500020483810 ) ) ;
#32631=CARTESIAN_POINT ( 'NONE',  ( -9.999999999999998224, 5.773502691896259087, -106.7500000040967620 ) ) ;
#32632=CARTESIAN_POINT ( 'NONE',  ( -9.999999999999996447, 5.773502691896259975, -169.3750000000000000 ) ) ;
#32633=CARTESIAN_POINT ( 'NONE',  ( -2.293366432827344421E-15, -12.48450537969573659, -66.21875000204838102 ) ) ;
#32639=CARTESIAN_POINT ( 'NONE',  ( 9.999999999999996447, -5.773502691896262640, -47.50000000409676915 ) ) ;
#32640=CARTESIAN_POINT ( 'NONE',  ( 10.81189881249999551, -6.242252689847874514, -39.15625000204835970 ) ) ;
#32644=CARTESIAN_POINT ( 'NONE',  ( -4.999999999999996447, 8.660254037844387298, -150.3750000040967905 ) ) ;
#32646=VERTEX_POINT ( 'NONE', #37849 ) ;
#32650=CARTESIAN_POINT ( 'NONE',  ( -9.999999999999998224, 1.224646799147353059E-15, -113.7499999999999858 ) ) ;
#32653=CARTESIAN_POINT ( 'NONE',  ( 10.00000000000051159, -5.773502691895965988, -119.1249999999999858 ) ) ;
#32654=CARTESIAN_POINT ( 'NONE',  ( 10.81189881249999729, 0.000000000000000000, -125.8437500020483952 ) ) ;
#32655=CARTESIAN_POINT ( 'NONE',  ( -10.81189881249999729, 6.242252689847871849, -134.4062500020484094 ) ) ;
#32657=CARTESIAN_POINT ( 'NONE',  ( 10.81189881249999551, -6.242252689847874514, -134.9687500020483810 ) ) ;
#32658=CARTESIAN_POINT ( 'NONE',  ( 10.00000000000025402, -5.773502691896113426, -125.5000000040967763 ) ) ;
#32659=CARTESIAN_POINT ( 'NONE',  ( -9.999999999999998224, 1.224646799147353059E-15, -103.2500000000000000 ) ) ;
#32660=CARTESIAN_POINT ( 'NONE',  ( -4.999999999999996447, 8.660254037844387298, -160.5000000000000000 ) ) ;
#32661=CYLINDRICAL_SURFACE ( 'NONE', #41877, 9.999999999999998224 ) ;
#32664=CARTESIAN_POINT ( 'NONE',  ( -10.81189881249999729, 1.324075727343319199E-15, -50.09375000204835260 ) ) ;
#32666=CARTESIAN_POINT ( 'NONE',  ( 5.405949406249999534, 9.363379034771803333, -161.5937500020484094 ) ) ;
#32672=CARTESIAN_POINT ( 'NONE',  ( -2.121150477449813534E-15, -11.54700538379251284, -90.87499999999997158 ) ) ;
#32673=ORIENTED_EDGE ( 'NONE', *, *, #42320, .F. ) ;
#32674=CARTESIAN_POINT ( 'NONE',  ( 7.644554776091147741E-16, 12.48450537969573659, -121.1562500020483952 ) ) ;
#32675=CARTESIAN_POINT ( 'NONE',  ( 9.999999999999998224, 0.000000000000000000, -134.3750000040967905 ) ) ;
#32680=CARTESIAN_POINT ( 'NONE',  ( -2.293366432827344421E-15, -12.48450537969573659, -57.40625000204838102 ) ) ;
#32698=CARTESIAN_POINT ( 'NONE',  ( 7.070501591499377789E-16, 11.54700538379251284, -25.62499999999997868 ) ) ;
#32701=CARTESIAN_POINT ( 'NONE',  ( -5.405949406250003975, -9.363379034771801557, -147.3437500020483810 ) ) ;
#32702=( BOUNDED_CURVE ( )  B_SPLINE_CURVE ( 2, ( #2997, #38605, #12264, #22209, #29116, #15915, #21993 ),
 .UNSPECIFIED., .F., .F. ) 
 B_SPLINE_CURVE_WITH_KNOTS ( ( 3, 2, 2, 3 ),
 ( 0.1791044776119403437, 0.1803482587064677289, 0.1815920398009950587, 0.1828358208955224162 ),
 .UNSPECIFIED. ) 
 CURVE ( )  GEOMETRIC_REPRESENTATION_ITEM ( )  RATIONAL_B_SPLINE_CURVE ( ( 0.9999999999999940048, 0.8660254037844447028, 1.000000000000000000, 0.8660254037844387076, 1.000000000000000000, 0.8660254037844357100, 1.000000000000003109 ) ) 
 REPRESENTATION_ITEM ( '' )  );
#32703=CARTESIAN_POINT ( 'NONE',  ( -10.81189881249999729, 1.324075727343319199E-15, -167.0937500020484094 ) ) ;
#32705=CARTESIAN_POINT ( 'NONE',  ( -9.999999999999998224, 1.224646799147353059E-15, -185.7500000000000000 ) ) ;
#32710=CARTESIAN_POINT ( 'NONE',  ( -10.81189881249999729, 1.324075727343319199E-15, -183.5937500020483810 ) ) ;
#32712=CARTESIAN_POINT ( 'NONE',  ( 7.644554776091147741E-16, 12.48450537969573659, -62.65625000204838813 ) ) ;
#32714=CARTESIAN_POINT ( 'NONE',  ( -5.000000000000003553, -8.660254037844383745, -111.9999999999999858 ) ) ;
#32716=CARTESIAN_POINT ( 'NONE',  ( -10.81189881249999729, -6.242252689847864744, -140.1562500020484094 ) ) ;
#32717=CARTESIAN_POINT ( 'NONE',  ( 5.405949406249999534, 9.363379034771803333, -157.2812500020484094 ) ) ;
#32719=CARTESIAN_POINT ( 'NONE',  ( 0.000000000000000000, 0.000000000000000000, -99.99999999999998579 ) ) ;
#32720=CARTESIAN_POINT ( 'NONE',  ( -5.405949406249996869, 9.363379034771805109, -89.34375000204838102 ) ) ;
#32723=CARTESIAN_POINT ( 'NONE',  ( 5.405949406249992428, -9.363379034771808662, -187.5937500020483810 ) ) ;
#32727=CARTESIAN_POINT ( 'NONE',  ( 7.644554776091147741E-16, 12.48450537969573659, -83.65625000204838102 ) ) ;
#32729=CARTESIAN_POINT ( 'NONE',  ( 4.999999999999992006, -8.660254037844389075, -62.62500000409676204 ) ) ;
#32730=CARTESIAN_POINT ( 'NONE',  ( -10.81189881249999729, 6.242252689847871849, -20.21875000204836681 ) ) ;
#32733=CARTESIAN_POINT ( 'NONE',  ( 10.81189881249999729, 0.000000000000000000, -15.03125000204835793 ) ) ;
#32741=ORIENTED_EDGE ( 'NONE', *, *, #29386, .F. ) ;
#32744=CARTESIAN_POINT ( 'NONE',  ( -2.293366432827344421E-15, -12.48450537969573659, -102.2187500020483668 ) ) ;
#32745=ORIENTED_EDGE ( 'NONE', *, *, #21998, .F. ) ;
#32746=ORIENTED_EDGE ( 'NONE', *, *, #7691, .T. ) ;
#32753=CARTESIAN_POINT ( 'NONE',  ( -5.000000000000003553, -8.660254037844383745, -121.3750000040967905 ) ) ;
#32755=CARTESIAN_POINT ( 'NONE',  ( -10.81189881249999729, 6.242252689847871849, -158.4062500020483810 ) ) ;
#32757=CARTESIAN_POINT ( 'NONE',  ( -9.999999999999998224, 1.224646799147353059E-15, -178.2500000000000284 ) ) ;
#32761=CARTESIAN_POINT ( 'NONE',  ( 10.81189881249999729, 0.000000000000000000, -77.84375000204838102 ) ) ;
#32763=CARTESIAN_POINT ( 'NONE',  ( 7.644554776091147741E-16, 12.48450537969573659, -85.15625000204838102 ) ) ;
#32766=CARTESIAN_POINT ( 'NONE',  ( 5.405949406249999534, 9.363379034771803333, -169.2812500020484094 ) ) ;
#32767=CARTESIAN_POINT ( 'NONE',  ( 5.405949406249999534, 9.363379034771803333, -176.7812500020484094 ) ) ;
#32768=CARTESIAN_POINT ( 'NONE',  ( -4.999999999999996447, 8.660254037844387298, -154.8750000040967905 ) ) ;
#32770=CARTESIAN_POINT ( 'NONE',  ( 5.405949406249999534, 9.363379034771803333, -4.093750002048368586 ) ) ;
#32771=CARTESIAN_POINT ( 'NONE',  ( 4.999999999999992006, -8.660254037844389075, -156.7500000000000000 ) ) ;
#32772=CARTESIAN_POINT ( 'NONE',  ( 5.405949406249992428, -9.363379034771808662, -117.0937500020483810 ) ) ;
#32774=CARTESIAN_POINT ( 'NONE',  ( 5.405949406249992428, -9.363379034771808662, -13.78125000204835615 ) ) ;
#32777=CARTESIAN_POINT ( 'NONE',  ( -10.81189881249999729, 1.324075727343319199E-15, -110.2812500020483810 ) ) ;
#32779=ORIENTED_EDGE ( 'NONE', *, *, #26106, .F. ) ;
#32780=CARTESIAN_POINT ( 'NONE',  ( 4.999999999999992006, -8.660254037844389075, -86.62500000409677625 ) ) ;
#32782=CARTESIAN_POINT ( 'NONE',  ( -10.81189881249999729, 6.242252689847871849, -41.21875000204835970 ) ) ;
#32783=ORIENTED_EDGE ( 'NONE', *, *, #35462, .F. ) ;
#32786=CARTESIAN_POINT ( 'NONE',  ( -4.999999999999996447, 8.660254037844387298, -10.87500000409674605 ) ) ;
#32793=ADVANCED_FACE ( 'NONE', ( #38701 ), #42135, .F. ) ;
#32794=AXIS2_PLACEMENT_3D ( 'NONE', #27435, #1108, #4990 ) ;
#32796=EDGE_CURVE ( 'NONE', #17140, #26892, #41921, .T. ) ;
#32802=AXIS2_PLACEMENT_3D ( 'NONE', #31105, #20512, #4124 ) ;
#32803=CARTESIAN_POINT ( 'NONE',  ( 0.000000000000000000, 0.000000000000000000, -99.99999999999998579 ) ) ;
#32805=DIRECTION ( 'NONE',  ( 1.000000000000000000, 0.000000000000000000, 0.000000000000000000 ) ) ;
#32806=CARTESIAN_POINT ( 'NONE',  ( 10.81189881249999551, -6.242252689847874514, -178.6562500020484094 ) ) ;
#32811=CARTESIAN_POINT ( 'NONE',  ( 5.405949406249992428, -9.363379034771808662, -102.0937500020483810 ) ) ;
#32813=CARTESIAN_POINT ( 'NONE',  ( -10.81189881249999729, 6.242252689847871849, -111.9062500020483810 ) ) ;
#32815=CARTESIAN_POINT ( 'NONE',  ( 10.81189881249999729, 6.242252689847867408, -118.2187500020483810 ) ) ;
#32818=CARTESIAN_POINT ( 'NONE',  ( -4.999999999999996447, 8.660254037844387298, -141.0000000000000000 ) ) ;
#32819=CARTESIAN_POINT ( 'NONE',  ( -10.00000000000000000, -5.773502691896251982, -2.624999999999960920 ) ) ;
#32823=CARTESIAN_POINT ( 'NONE',  ( 7.070501591499377789E-16, 11.54700538379251284, -180.5000000040967905 ) ) ;
#32825=CARTESIAN_POINT ( 'NONE',  ( -5.405949406249996869, 9.363379034771805109, -32.34375000204836681 ) ) ;
#32827=CARTESIAN_POINT ( 'NONE',  ( -10.81189881249999729, 6.242252689847871849, -141.7187500020483810 ) ) ;
#32829=CARTESIAN_POINT ( 'NONE',  ( 10.81189881249999551, -6.242252689847874514, -36.15625000204835970 ) ) ;
#32832=AXIS2_PLACEMENT_3D ( 'NONE', #14185, #34298, #27168 ) ;
#32833=CARTESIAN_POINT ( 'NONE',  ( 9.999999999999996447, -5.773502691896262640, -68.12499999999998579 ) ) ;
#32834=CARTESIAN_POINT ( 'NONE',  ( 5.405949406249992428, -9.363379034771808662, -133.7812500020483810 ) ) ;
#32837=CARTESIAN_POINT ( 'NONE',  ( 7.070501591499376803E-16, 11.54700538379251284, -142.6250000000000000 ) ) ;
#32838=CARTESIAN_POINT ( 'NONE',  ( 5.000000000000000000, 8.660254037844385522, -111.6250000040967763 ) ) ;
#32839=CARTESIAN_POINT ( 'NONE',  ( -9.999999999999998224, 1.224646799147353059E-15, -100.6250000040967905 ) ) ;
#32840=CARTESIAN_POINT ( 'NONE',  ( -5.405949406250003975, -9.363379034771801557, -63.34375000204836681 ) ) ;
#32841=ORIENTED_EDGE ( 'NONE', *, *, #42516, .T. ) ;
#32845=EDGE_CURVE ( 'NONE', #15525, #36438, #34610, .T. ) ;
#32846=CARTESIAN_POINT ( 'NONE',  ( -9.999999999999998224, 1.224646799147353059E-15, -157.6250000040967905 ) ) ;
#32847=CARTESIAN_POINT ( 'NONE',  ( 4.999999999999992006, -8.660254037844389075, -40.12500000409676915 ) ) ;
#32850=CARTESIAN_POINT ( 'NONE',  ( -4.999999999999996447, 8.660254037844387298, -166.5000000000000000 ) ) ;
#32854=( BOUNDED_CURVE ( )  B_SPLINE_CURVE ( 2, ( #16582, #33240, #3666, #39899, #6475, #16794, #9494 ),
 .UNSPECIFIED., .F., .F. ) 
 B_SPLINE_CURVE_WITH_KNOTS ( ( 3, 2, 2, 3 ),
 ( 0.3507462686567164867, 0.3519900497512438720, 0.3532338308457712572, 0.3544776119402986980 ),
 .UNSPECIFIED. ) 
 CURVE ( )  GEOMETRIC_REPRESENTATION_ITEM ( )  RATIONAL_B_SPLINE_CURVE ( ( 0.9999999999999940048, 0.8660254037844447028, 1.000000000000000000, 0.8660254037844387076, 1.000000000000000000, 0.8660254037844207220, 1.000000000000017986 ) ) 
 REPRESENTATION_ITEM ( '' )  );
#32864=CARTESIAN_POINT ( 'NONE',  ( -2.293366432827344421E-15, -12.48450537969573659, -124.7187500020483668 ) ) ;
#32865=CARTESIAN_POINT ( 'NONE',  ( 5.405949406249999534, 9.363379034771803333, -136.2812500020483810 ) ) ;
#32867=CARTESIAN_POINT ( 'NONE',  ( 5.405949406249999534, 9.363379034771803333, -137.5937500020483810 ) ) ;
#32869=CARTESIAN_POINT ( 'NONE',  ( 9.999999999999998224, 0.000000000000000000, -141.8750000040967905 ) ) ;
#32870=CARTESIAN_POINT ( 'NONE',  ( 4.999999999999992006, -8.660254037844389075, -164.2500000000000000 ) ) ;
#32871=CARTESIAN_POINT ( 'NONE',  ( -9.999999999999998224, 1.224646799147353059E-15, -132.1250000040967620 ) ) ;
#32874=CARTESIAN_POINT ( 'NONE',  ( 5.405949406249999534, 9.363379034771803333, -56.59375000204835970 ) ) ;
#32876=CARTESIAN_POINT ( 'NONE',  ( 5.405949406249999534, 9.363379034771803333, -160.0937500020484094 ) ) ;
#32879=CYLINDRICAL_SURFACE ( 'NONE', #40323, 9.999999999999998224 ) ;
#32881=CARTESIAN_POINT ( 'NONE',  ( 10.00000000000000000, 5.773502691896255534, -93.37499999999997158 ) ) ;
#32882=VERTEX_POINT ( 'NONE', #9344 ) ;
#32883=CARTESIAN_POINT ( 'NONE',  ( -5.405949406249996869, 9.363379034771805109, -109.0312500020483810 ) ) ;
#32884=CARTESIAN_POINT ( 'NONE',  ( 4.999999999999992006, -8.660254037844389075, -134.6250000040967620 ) ) ;
#32885=CYLINDRICAL_SURFACE ( 'NONE', #11178, 9.999999999999998224 ) ;
#32889=CARTESIAN_POINT ( 'NONE',  ( -5.405949406249996869, 9.363379034771805109, -58.03125000204836681 ) ) ;
#32896=CARTESIAN_POINT ( 'NONE',  ( 31.99999999999997158, 0.000000000000000000, -180.0000000000000000 ) ) ;
#32898=ORIENTED_EDGE ( 'NONE', *, *, #23304, .T. ) ;
#32908=CARTESIAN_POINT ( 'NONE',  ( -5.000000000000003553, -8.660254037844383745, -29.49999999999997158 ) ) ;
#32912=CARTESIAN_POINT ( 'NONE',  ( -10.81189881249999729, 1.324075727343319199E-15, -149.0937500020483810 ) ) ;
#32913=CARTESIAN_POINT ( 'NONE',  ( -5.405949406250003975, -9.363379034771801557, -163.8437500020484094 ) ) ;
#32914=CARTESIAN_POINT ( 'NONE',  ( 5.000000000000000000, 8.660254037844385522, -123.6250000040967905 ) ) ;
#32915=CARTESIAN_POINT ( 'NONE',  ( 7.070501591499377789E-16, 11.54700538379251284, -189.1250000000000000 ) ) ;
#32920=CARTESIAN_POINT ( 'NONE',  ( -2.293366432827344421E-15, -12.48450537969573659, -184.7187500020484094 ) ) ;
#32922=CARTESIAN_POINT ( 'NONE',  ( -2.293366432827344421E-15, -12.48450537969573659, -61.90625000204838813 ) ) ;
#32924=CARTESIAN_POINT ( 'NONE',  ( -2.121150477449813534E-15, -11.54700538379251284, -116.3749999999999858 ) ) ;
#32927=CARTESIAN_POINT ( 'NONE',  ( 5.405949406249992428, -9.363379034771808662, -142.7812500020483810 ) ) ;
#32928=CARTESIAN_POINT ( 'NONE',  ( -5.405949406249996869, 9.363379034771805109, -158.5312500020484094 ) ) ;
#32930=CARTESIAN_POINT ( 'NONE',  ( 9.999999999999998224, 0.000000000000000000, -125.0000000000000000 ) ) ;
#32931=CARTESIAN_POINT ( 'NONE',  ( -10.81189881249999729, 1.324075727343319199E-15, -93.59375000204838102 ) ) ;
#32933=VERTEX_POINT ( 'NONE', #22726 ) ;
#32935=CARTESIAN_POINT ( 'NONE',  ( -10.81189881249999907, -6.242252689847864744, -187.9687500020484094 ) ) ;
#32940=CARTESIAN_POINT ( 'NONE',  ( -10.81189881249999907, -6.242252689847864744, -86.15625000204836681 ) ) ;
#32942=CARTESIAN_POINT ( 'NONE',  ( -2.121150477449813534E-15, -11.54700538379251284, -58.25000000409676915 ) ) ;
#32943=CARTESIAN_POINT ( 'NONE',  ( -5.405949406249996869, 9.363379034771805109, -15.84375000204835082 ) ) ;
#32946=CARTESIAN_POINT ( 'NONE',  ( -2.293366432827344421E-15, -12.48450537969573659, -15.40625000204837214 ) ) ;
#32950=CARTESIAN_POINT ( 'NONE',  ( -9.999999999999998224, 1.224646799147353059E-15, -135.1250000040967620 ) ) ;
#32954=ORIENTED_EDGE ( 'NONE', *, *, #3225, .T. ) ;
#32956=CARTESIAN_POINT ( 'NONE',  ( 5.405949406249999534, 9.363379034771803333, -100.0937500020483810 ) ) ;
#32966=AXIS2_PLACEMENT_3D ( 'NONE', #16700, #26021, #20166 ) ;
#32971=CARTESIAN_POINT ( 'NONE',  ( 10.81189881249999729, 0.000000000000000000, -153.0312500020484094 ) ) ;
#32977=CARTESIAN_POINT ( 'NONE',  ( -5.405949406250003975, -9.363379034771801557, -76.84375000204838102 ) ) ;
#32978=CARTESIAN_POINT ( 'NONE',  ( 5.405949406249999534, 9.363379034771803333, -83.78125000204838102 ) ) ;
#32981=CARTESIAN_POINT ( 'NONE',  ( 5.405949406249992428, -9.363379034771808662, -165.2812500020484094 ) ) ;
#32982=CARTESIAN_POINT ( 'NONE',  ( -5.405949406249996869, 9.363379034771805109, -182.5312500020484094 ) ) ;
#32983=CARTESIAN_POINT ( 'NONE',  ( 5.000000000000000000, 8.660254037844385522, -155.1250000040967905 ) ) ;
#32985=CARTESIAN_POINT ( 'NONE',  ( 5.405949406249999534, 9.363379034771803333, -7.093750002048371250 ) ) ;
#32986=CYLINDRICAL_SURFACE ( 'NONE', #15783, 9.999999999999998224 ) ;
#32987=CARTESIAN_POINT ( 'NONE',  ( 5.405949406249999534, 9.363379034771803333, -115.0937500020483810 ) ) ;
#32988=EDGE_CURVE ( 'NONE', #6419, #21319, #24409, .T. ) ;
#32990=CARTESIAN_POINT ( 'NONE',  ( 10.81189881249999551, -6.242252689847874514, -13.65625000204837036 ) ) ;
#32993=CARTESIAN_POINT ( 'NONE',  ( -10.81189881249999907, -6.242252689847864744, -105.6562500020483952 ) ) ;
#32996=CARTESIAN_POINT ( 'NONE',  ( 9.999999999999998224, 0.000000000000000000, -86.37500000409677625 ) ) ;
#32998=CARTESIAN_POINT ( 'NONE',  ( 7.644554776091147741E-16, 12.48450537969573659, -39.96875000204835970 ) ) ;
#33004=CARTESIAN_POINT ( 'NONE',  ( -2.121150477449813534E-15, -11.54700538379251284, -8.750000004096758488 ) ) ;
#33007=ORIENTED_EDGE ( 'NONE', *, *, #34654, .F. ) ;
#33014=VERTEX_POINT ( 'NONE', #26596 ) ;
#33017=CARTESIAN_POINT ( 'NONE',  ( -5.405949406249996869, 9.363379034771805109, -184.0312500020484094 ) ) ;
#33021=CARTESIAN_POINT ( 'NONE',  ( -2.293366432827344421E-15, -12.48450537969573659, -102.2187500020483952 ) ) ;
#33023=CARTESIAN_POINT ( 'NONE',  ( 5.405949406249992428, -9.363379034771808662, -111.2812500020483810 ) ) ;
#33025=CARTESIAN_POINT ( 'NONE',  ( 5.405949406249999534, 9.363379034771803333, -115.0937500020483810 ) ) ;
#33029=CARTESIAN_POINT ( 'NONE',  ( -5.000000000000003553, -8.660254037844383745, -133.0000000000000000 ) ) ;
#33030=CARTESIAN_POINT ( 'NONE',  ( 9.999999999999998224, 0.000000000000000000, -6.499999999999977796 ) ) ;
#33032=AXIS2_PLACEMENT_3D ( 'NONE', #36632, #614, #4683 ) ;
#33034=CARTESIAN_POINT ( 'NONE',  ( 5.000000000000000000, 8.660254037844385522, -180.6250000040967905 ) ) ;
#33036=CARTESIAN_POINT ( 'NONE',  ( -10.81189881249999907, -6.242252689847864744, -28.96875000204835260 ) ) ;
#33037=CARTESIAN_POINT ( 'NONE',  ( 9.999999999999998224, 0.000000000000000000, -149.3750000040967905 ) ) ;
#33038=CARTESIAN_POINT ( 'NONE',  ( 10.81189881249999907, 6.242252689847868297, -140.7187500020483810 ) ) ;
#33039=EDGE_CURVE ( 'NONE', #1917, #31885, #17429, .T. ) ;
#33041=CARTESIAN_POINT ( 'NONE',  ( 10.81189881249999729, 0.000000000000000000, -36.03125000204837391 ) ) ;
#33042=DIRECTION ( 'NONE',  ( -0.000000000000000000, -0.000000000000000000, -1.000000000000000000 ) ) ;
#33044=CARTESIAN_POINT ( 'NONE',  ( -2.121150477449813534E-15, -11.54700538379251284, -63.87499999999999289 ) ) ;
#33045=CARTESIAN_POINT ( 'NONE',  ( -5.405949406250003975, -9.363379034771801557, -129.5312500020484094 ) ) ;
#33049=CARTESIAN_POINT ( 'NONE',  ( -4.999999999999996447, 8.660254037844387298, -142.5000000000000000 ) ) ;
#33050=CARTESIAN_POINT ( 'NONE',  ( 4.999999999999992006, -8.660254037844389075, -107.6250000040967763 ) ) ;
#33052=CARTESIAN_POINT ( 'NONE',  ( 5.405949406249992428, -9.363379034771808662, -63.09375000204836681 ) ) ;
#33053=ORIENTED_EDGE ( 'NONE', *, *, #27535, .T. ) ;
#33058=CARTESIAN_POINT ( 'NONE',  ( -9.999999999999998224, 5.773502691896259087, -34.75000000409674783 ) ) ;
#33059=CARTESIAN_POINT ( 'NONE',  ( 9.999999999999998224, 0.000000000000000000, -117.8750000040967905 ) ) ;
#33061=EDGE_CURVE ( 'NONE', #30831, #16772, #6114, .T. ) ;
#33064=ORIENTED_EDGE ( 'NONE', *, *, #15100, .F. ) ;
#33066=EDGE_CURVE ( 'NONE', #36083, #35300, #20258, .T. ) ;
#33070=CARTESIAN_POINT ( 'NONE',  ( -9.999999999999998224, 1.224646799147353059E-15, -168.1250000040967905 ) ) ;
#33074=CARTESIAN_POINT ( 'NONE',  ( 10.81189881249999551, -6.242252689847874514, -124.4687500020483952 ) ) ;
#33075=CARTESIAN_POINT ( 'NONE',  ( -10.81189881249999729, 6.242252689847871849, -129.9062500020483810 ) ) ;
#33078=CARTESIAN_POINT ( 'NONE',  ( 10.81189881249999729, 6.242252689847867408, -142.2187500020483810 ) ) ;
#33081=CARTESIAN_POINT ( 'NONE',  ( 9.999999999999998224, 0.000000000000000000, -165.5000000000000000 ) ) ;
#33082=CARTESIAN_POINT ( 'NONE',  ( 0.000000000000000000, 0.000000000000000000, -99.99999999999998579 ) ) ;
#33085=CARTESIAN_POINT ( 'NONE',  ( 5.405949406249992428, -9.363379034771808662, -52.59375000204835260 ) ) ;
#33086=DIRECTION ( 'NONE',  ( -0.000000000000000000, -0.000000000000000000, -1.000000000000000000 ) ) ;
#33087=CARTESIAN_POINT ( 'NONE',  ( -5.405949406249996869, 9.363379034771805109, -162.8437500020484094 ) ) ;
#33093=CARTESIAN_POINT ( 'NONE',  ( -5.000000000000003553, -8.660254037844383745, -90.99999999999998579 ) ) ;
#33094=ADVANCED_FACE ( 'NONE', ( #3506 ), #26386, .F. ) ;
#33096=( BOUNDED_CURVE ( )  B_SPLINE_CURVE ( 2, ( #17446, #14198, #13984, #34093, #30642, #31074, #27181 ),
 .UNSPECIFIED., .F., .F. ) 
 B_SPLINE_CURVE_WITH_KNOTS ( ( 3, 2, 2, 3 ),
 ( 0.2276119402985075368, 0.2288557213930349221, 0.2300995024875622796, 0.2313432835820896372 ),
 .UNSPECIFIED. ) 
 CURVE ( )  GEOMETRIC_REPRESENTATION_ITEM ( )  RATIONAL_B_SPLINE_CURVE ( ( 0.9999999999999910072, 0.8660254037844477004, 1.000000000000000000, 0.8660254037844387076, 1.000000000000000000, 0.8660254037844297148, 1.000000000000008882 ) ) 
 REPRESENTATION_ITEM ( '' )  );
#33097=CARTESIAN_POINT ( 'NONE',  ( -10.81189881249999729, 6.242252689847871849, -111.9062500020483810 ) ) ;
#33098=CARTESIAN_POINT ( 'NONE',  ( 9.999999999999998224, 0.000000000000000000, -128.3750000040967905 ) ) ;
#33106=CARTESIAN_POINT ( 'NONE',  ( -10.81189881249999729, 6.242252689847871849, -53.40625000204837391 ) ) ;
#33108=DIRECTION ( 'NONE',  ( -0.000000000000000000, -0.000000000000000000, -1.000000000000000000 ) ) ;
#33113=VERTEX_POINT ( 'NONE', #7816 ) ;
#33114=LINE ( 'NONE', #13225, #38992 ) ;
#33115=EDGE_CURVE ( 'NONE', #14748, #32646, #23249, .T. ) ;
#33120=ORIENTED_EDGE ( 'NONE', *, *, #12971, .F. ) ;
#33127=CARTESIAN_POINT ( 'NONE',  ( 9.999999999999998224, 0.000000000000000000, -28.99999999999997158 ) ) ;
#33130=CARTESIAN_POINT ( 'NONE',  ( 10.81189881249999907, 6.242252689847868297, -149.7187500020483810 ) ) ;
#33131=CARTESIAN_POINT ( 'NONE',  ( 10.81189881249999551, -6.242252689847874514, -161.9687500020484094 ) ) ;
#33134=CARTESIAN_POINT ( 'NONE',  ( -5.000000000000003553, -8.660254037844383745, -185.5000000000000000 ) ) ;
#33136=CARTESIAN_POINT ( 'NONE',  ( -4.999999999999996447, 8.660254037844387298, -138.0000000000000000 ) ) ;
#33139=CARTESIAN_POINT ( 'NONE',  ( 10.81189881249999551, -6.242252689847874514, -185.9687500020484094 ) ) ;
#33142=CARTESIAN_POINT ( 'NONE',  ( 7.644554776091147741E-16, 12.48450537969573659, -53.65625000204838102 ) ) ;
#33144=CARTESIAN_POINT ( 'NONE',  ( 7.070501591499377789E-16, 11.54700538379251284, -114.1249999999999858 ) ) ;
#33146=CARTESIAN_POINT ( 'NONE',  ( 10.81189881249999729, 0.000000000000000000, -136.5312500020484094 ) ) ;
#33147=CARTESIAN_POINT ( 'NONE',  ( -2.293366432827344421E-15, -12.48450537969573659, -147.4062500020483810 ) ) ;
#33150=CARTESIAN_POINT ( 'NONE',  ( -2.293366432827344421E-15, -12.48450537969573659, -82.71875000204838102 ) ) ;
#33153=CARTESIAN_POINT ( 'NONE',  ( 5.405949406249992428, -9.363379034771808662, -177.0937500020484094 ) ) ;
#33157=CARTESIAN_POINT ( 'NONE',  ( -10.81189881249999907, -6.242252689847864744, -81.65625000204839523 ) ) ;
#33159=CARTESIAN_POINT ( 'NONE',  ( 9.999999999999998224, 0.000000000000000000, -63.87500000409676915 ) ) ;
#33160=CARTESIAN_POINT ( 'NONE',  ( -10.81189881249999729, 6.242252689847871849, -18.71875000204837036 ) ) ;
#33165=CARTESIAN_POINT ( 'NONE',  ( 10.81189881249999729, 0.000000000000000000, -12.03125000204835438 ) ) ;
#33168=CARTESIAN_POINT ( 'NONE',  ( -9.999999999999998224, 1.224646799147353059E-15, -114.1250000040967763 ) ) ;
#33175=CARTESIAN_POINT ( 'NONE',  ( -2.293366432827344421E-15, -12.48450537969573659, -100.7187500020483952 ) ) ;
#33176=VERTEX_POINT ( 'NONE', #17284 ) ;
#33178=ORIENTED_EDGE ( 'NONE', *, *, #8857, .T. ) ;
#33188=CARTESIAN_POINT ( 'NONE',  ( -4.999999999999996447, 8.660254037844387298, -172.5000000000000284 ) ) ;
#33189=CARTESIAN_POINT ( 'NONE',  ( -10.81189881249999729, 6.242252689847871849, -147.9062500020483810 ) ) ;
#33191=CARTESIAN_POINT ( 'NONE',  ( 9.999999999999479527, 5.773502691896553074, -178.8749999999999716 ) ) ;
#33197=CARTESIAN_POINT ( 'NONE',  ( -5.405949406250003975, -9.363379034771801557, -70.84375000204836681 ) ) ;
#33198=CARTESIAN_POINT ( 'NONE',  ( -5.405949406249996869, 9.363379034771805109, -77.53125000204838102 ) ) ;
#33200=DIRECTION ( 'NONE',  ( -1.000000000000000000, 0.000000000000000000, 0.000000000000000000 ) ) ;
#33201=CARTESIAN_POINT ( 'NONE',  ( -2.293366432827344421E-15, -12.48450537969573659, -162.4062500020483810 ) ) ;
#33202=CARTESIAN_POINT ( 'NONE',  ( -10.81189881249999907, -6.242252689847864744, -168.6562500020483810 ) ) ;
#33204=LINE ( 'NONE', #10088, #7040 ) ;
#33205=CARTESIAN_POINT ( 'NONE',  ( -5.405949406250003975, -9.363379034771801557, -4.843750002048369474 ) ) ;
#33206=CARTESIAN_POINT ( 'NONE',  ( -4.999999999999996447, 8.660254037844387298, -108.3750000040967763 ) ) ;
#33207=CARTESIAN_POINT ( 'NONE',  ( 10.81189881249999551, -6.242252689847874514, -104.9687500020483810 ) ) ;
#33209=CARTESIAN_POINT ( 'NONE',  ( 10.81189881249999551, -6.242252689847874514, -15.15625000204837036 ) ) ;
#33212=CARTESIAN_POINT ( 'NONE',  ( 5.405949406249999534, 9.363379034771803333, -104.7812500020483810 ) ) ;
#33214=ORIENTED_EDGE ( 'NONE', *, *, #3533, .T. ) ;
#33215=CARTESIAN_POINT ( 'NONE',  ( -5.000000000000003553, -8.660254037844383745, -83.87500000409677625 ) ) ;
#33216=CARTESIAN_POINT ( 'NONE',  ( 5.000000000000000000, 8.660254037844385522, -134.1250000040967620 ) ) ;
#33217=CARTESIAN_POINT ( 'NONE',  ( -5.405949406250003975, -9.363379034771801557, -45.34375000204838102 ) ) ;
#33222=CARTESIAN_POINT ( 'NONE',  ( 9.999999999999996447, -5.773502691896262640, -16.00000000409676559 ) ) ;
#33235=AXIS2_PLACEMENT_3D ( 'NONE', #9481, #31958, #22650 ) ;
#33239=FACE_OUTER_BOUND ( 'NONE', #9437, .T. ) ;
#33240=CARTESIAN_POINT ( 'NONE',  ( 9.999999999999742428, 5.773502691896404748, -128.2500000040967905 ) ) ;
#33241=CARTESIAN_POINT ( 'NONE',  ( 5.405949406249992428, -9.363379034771808662, -175.7812500020484094 ) ) ;
#33244=CARTESIAN_POINT ( 'NONE',  ( -5.405949406249996869, 9.363379034771805109, -98.34375000204838102 ) ) ;
#33245=CARTESIAN_POINT ( 'NONE',  ( 9.999999999999227285, 5.773502691896701400, -106.8749999999999432 ) ) ;
#33246=CARTESIAN_POINT ( 'NONE',  ( 10.81189881249999907, 6.242252689847868297, -106.4062500020483952 ) ) ;
#33248=CARTESIAN_POINT ( 'NONE',  ( 10.81189881249999729, 0.000000000000000000, -116.8437500020483810 ) ) ;
#33251=CARTESIAN_POINT ( 'NONE',  ( 9.999999999999998224, 0.000000000000000000, -122.0000000000000000 ) ) ;
#33253=CARTESIAN_POINT ( 'NONE',  ( -4.999999999999996447, 8.660254037844387298, -133.5000000000000000 ) ) ;
#33254=CARTESIAN_POINT ( 'NONE',  ( 9.999999999999998224, 0.000000000000000000, -1.999999999999974021 ) ) ;
#33257=CARTESIAN_POINT ( 'NONE',  ( -5.000000000000003553, -8.660254037844383745, -182.8750000040967905 ) ) ;
#33259=CARTESIAN_POINT ( 'NONE',  ( 5.405949406249999534, 9.363379034771803333, -28.09375000204836326 ) ) ;
#33261=CARTESIAN_POINT ( 'NONE',  ( -10.81189881249999729, 6.242252689847871849, -137.2187500020483810 ) ) ;
#33263=CARTESIAN_POINT ( 'NONE',  ( 10.81189881249999907, 6.242252689847868297, -37.40625000204836681 ) ) ;
#33265=CARTESIAN_POINT ( 'NONE',  ( -9.999999999999998224, 5.773502691896259087, -58.37499999999998579 ) ) ;
#33266=CARTESIAN_POINT ( 'NONE',  ( 10.81189881249999729, 0.000000000000000000, -129.0312500020484094 ) ) ;
#33269=CARTESIAN_POINT ( 'NONE',  ( -2.121150477449813534E-15, -11.54700538379251284, -131.3750000000000000 ) ) ;
#33270=CARTESIAN_POINT ( 'NONE',  ( -10.00000000000000000, -5.773502691896251982, -106.5000000040967763 ) ) ;
#33272=CARTESIAN_POINT ( 'NONE',  ( 5.405949406249999534, 9.363379034771803333, -68.59375000204836681 ) ) ;
#33273=EDGE_LOOP ( 'NONE', ( #18267, #24254 ) ) ;
#33275=VECTOR ( 'NONE', #30509, 1000.000000000000000 ) ;
#33279=CARTESIAN_POINT ( 'NONE',  ( -9.999999999999998224, 1.224646799147353059E-15, -34.62500000409676915 ) ) ;
#33285=EDGE_CURVE ( 'NONE', #17480, #19924, #7876, .T. ) ;
#33286=VERTEX_POINT ( 'NONE', #24006 ) ;
#33287=CARTESIAN_POINT ( 'NONE',  ( 9.999999999999998224, 0.000000000000000000, -126.8750000040967905 ) ) ;
#33292=CARTESIAN_POINT ( 'NONE',  ( -4.999999999999996447, 8.660254037844387298, -144.3750000040967905 ) ) ;
#33296=DIRECTION ( 'NONE',  ( -1.000000000000000000, 0.000000000000000000, 0.000000000000000000 ) ) ;
#33297=CARTESIAN_POINT ( 'NONE',  ( 7.644554776091147741E-16, 12.48450537969573659, -123.9687500020483952 ) ) ;
#33298=CARTESIAN_POINT ( 'NONE',  ( -2.293366432827344421E-15, -12.48450537969573659, -135.4062500020483810 ) ) ;
#33300=CARTESIAN_POINT ( 'NONE',  ( 10.81189881249999551, -6.242252689847874514, -136.4687500020483810 ) ) ;
#33303=CARTESIAN_POINT ( 'NONE',  ( 10.00000000000000000, 5.773502691896255534, -153.3750000000000000 ) ) ;
#33308=CARTESIAN_POINT ( 'NONE',  ( 7.644554776091147741E-16, 12.48450537969573659, -51.96875000204836681 ) ) ;
#33310=CARTESIAN_POINT ( 'NONE',  ( -10.81189881249999729, 1.324075727343319199E-15, -162.5937500020484094 ) ) ;
#33314=CARTESIAN_POINT ( 'NONE',  ( -4.999999999999996447, 8.660254037844387298, -79.49999999999998579 ) ) ;
#33315=ORIENTED_EDGE ( 'NONE', *, *, #7790, .F. ) ;
#33316=CARTESIAN_POINT ( 'NONE',  ( 7.644554776091147741E-16, 12.48450537969573659, -107.6562500020483810 ) ) ;
#33317=CARTESIAN_POINT ( 'NONE',  ( -10.00000000000000000, -5.773502691896251982, -135.0000000040967905 ) ) ;
#33318=DIRECTION ( 'NONE',  ( -0.000000000000000000, -0.000000000000000000, -1.000000000000000000 ) ) ;
#33322=CARTESIAN_POINT ( 'NONE',  ( 5.405949406249992428, -9.363379034771808662, -54.28125000204836681 ) ) ;
#33328=VERTEX_POINT ( 'NONE', #41011 ) ;
#33331=ORIENTED_EDGE ( 'NONE', *, *, #15733, .F. ) ;
#33343=CARTESIAN_POINT ( 'NONE',  ( -9.999999999999998224, 1.224646799147353059E-15, -134.7499999999999716 ) ) ;
#33348=CARTESIAN_POINT ( 'NONE',  ( -5.405949406250003975, -9.363379034771801557, -153.3437500020483810 ) ) ;
#33349=CARTESIAN_POINT ( 'NONE',  ( -10.81189881249999729, -6.242252689847864744, -163.9687500020483526 ) ) ;
#33350=CARTESIAN_POINT ( 'NONE',  ( 9.999999999999998224, 0.000000000000000000, -123.8750000040967905 ) ) ;
#33351=CARTESIAN_POINT ( 'NONE',  ( 9.999999999999998224, 0.000000000000000000, -126.5000000000000000 ) ) ;
#33352=CARTESIAN_POINT ( 'NONE',  ( 7.070501591499377789E-16, 11.54700538379251284, -178.6250000000000000 ) ) ;
#33357=CARTESIAN_POINT ( 'NONE',  ( -10.81189881249999729, 6.242252689847871849, -186.7187500020483810 ) ) ;
#33360=CARTESIAN_POINT ( 'NONE',  ( 5.405949406249992428, -9.363379034771808662, -54.28125000204836681 ) ) ;
#33362=CARTESIAN_POINT ( 'NONE',  ( 4.999999999999992006, -8.660254037844389075, -119.2500000000000000 ) ) ;
#33363=ORIENTED_EDGE ( 'NONE', *, *, #29132, .T. ) ;
#33364=CARTESIAN_POINT ( 'NONE',  ( -5.405949406249996869, 9.363379034771805109, -134.5312500020484094 ) ) ;
#33365=CARTESIAN_POINT ( 'NONE',  ( -10.81189881249999907, -6.242252689847864744, -146.1562500020484094 ) ) ;
#33369=CARTESIAN_POINT ( 'NONE',  ( 10.81189881249999551, -6.242252689847874514, -80.96875000204838102 ) ) ;
#33372=CARTESIAN_POINT ( 'NONE',  ( 5.405949406249999534, 9.363379034771803333, -184.0937500020483810 ) ) ;
#33376=CARTESIAN_POINT ( 'NONE',  ( -10.81189881249999729, 1.324075727343319199E-15, -80.28125000204838102 ) ) ;
#33378=CARTESIAN_POINT ( 'NONE',  ( -2.121150477449813534E-15, -11.54700538379251284, -55.25000000409677625 ) ) ;
#33379=CARTESIAN_POINT ( 'NONE',  ( 7.644554776091147741E-16, 12.48450537969573659, -8.468750002048359704 ) ) ;
#33382=CARTESIAN_POINT ( 'NONE',  ( 10.81189881249999729, 0.000000000000000000, -7.531250002048350822 ) ) ;
#33389=ORIENTED_EDGE ( 'NONE', *, *, #3031, .F. ) ;
#33390=CARTESIAN_POINT ( 'NONE',  ( 4.999999999999992006, -8.660254037844389075, -160.1250000040967905 ) ) ;
#33391=CARTESIAN_POINT ( 'NONE',  ( 7.644554776091147741E-16, 12.48450537969573659, -102.9687500020483668 ) ) ;
#33393=VERTEX_POINT ( 'NONE', #4945 ) ;
#33398=CARTESIAN_POINT ( 'NONE',  ( -4.999999999999996447, 8.660254037844387298, -43.49999999999998579 ) ) ;
#33402=DIRECTION ( 'NONE',  ( 0.000000000000000000, 0.000000000000000000, 1.000000000000000000 ) ) ;
#33403=CARTESIAN_POINT ( 'NONE',  ( -10.81189881249999907, -6.242252689847864744, -147.6562500020483810 ) ) ;
#33408=CARTESIAN_POINT ( 'NONE',  ( -9.999999999999998224, 1.224646799147353059E-15, -160.6250000040967905 ) ) ;
#33411=CARTESIAN_POINT ( 'NONE',  ( -5.405949406249996869, 9.363379034771805109, -69.84375000204836681 ) ) ;
#33412=CARTESIAN_POINT ( 'NONE',  ( 5.405949406249992428, -9.363379034771808662, -76.78125000204838102 ) ) ;
#33414=CARTESIAN_POINT ( 'NONE',  ( -5.405949406249996869, 9.363379034771805109, -160.0312500020484094 ) ) ;
#33415=CARTESIAN_POINT ( 'NONE',  ( -5.405949406249996869, 9.363379034771805109, -175.0312500020484094 ) ) ;
#33416=DIRECTION ( 'NONE',  ( -0.000000000000000000, -0.000000000000000000, -1.000000000000000000 ) ) ;
#33417=CARTESIAN_POINT ( 'NONE',  ( -2.121150477449813534E-15, -11.54700538379251284, -145.2500000040967905 ) ) ;
#33418=DIRECTION ( 'NONE',  ( -0.000000000000000000, -0.000000000000000000, -1.000000000000000000 ) ) ;
#33419=CARTESIAN_POINT ( 'NONE',  ( -2.293366432827344421E-15, -12.48450537969573659, -105.2187500020483952 ) ) ;
#33421=CARTESIAN_POINT ( 'NONE',  ( 5.405949406249999534, 9.363379034771803333, -4.281250002048375691 ) ) ;
#33424=CARTESIAN_POINT ( 'NONE',  ( -10.81189881249999729, 1.324075727343319199E-15, -96.78125000204839523 ) ) ;
#33427=CARTESIAN_POINT ( 'NONE',  ( 7.070501591499377789E-16, 11.54700538379251284, -74.00000000409677625 ) ) ;
#33429=CARTESIAN_POINT ( 'NONE',  ( -10.81189881249999907, -6.242252689847864744, -31.96875000204834905 ) ) ;
#33432=CARTESIAN_POINT ( 'NONE',  ( 10.81189881249999729, 0.000000000000000000, -39.03125000204838102 ) ) ;
#33436=CARTESIAN_POINT ( 'NONE',  ( -9.999999999999998224, 1.224646799147353059E-15, -10.62500000409674605 ) ) ;
#33440=ORIENTED_EDGE ( 'NONE', *, *, #38704, .T. ) ;
#33442=ORIENTED_EDGE ( 'NONE', *, *, #34658, .T. ) ;
#33452=CARTESIAN_POINT ( 'NONE',  ( 10.81189881249999551, -6.242252689847874514, -175.6562500020484094 ) ) ;
#33453=CARTESIAN_POINT ( 'NONE',  ( 0.000000000000000000, 0.000000000000000000, -169.9999999999999716 ) ) ;
#33455=CARTESIAN_POINT ( 'NONE',  ( 10.81189881249999551, -6.242252689847874514, -89.96875000204838102 ) ) ;
#33457=CARTESIAN_POINT ( 'NONE',  ( 5.405949406249999534, 9.363379034771803333, -98.78125000204839523 ) ) ;
#33459=CARTESIAN_POINT ( 'NONE',  ( 10.81189881249999729, 0.000000000000000000, -112.3437500020483810 ) ) ;
#33464=CARTESIAN_POINT ( 'NONE',  ( 5.405949406249992428, -9.363379034771808662, -196.7812500020484094 ) ) ;
#33467=CARTESIAN_POINT ( 'NONE',  ( 9.999999999999996447, -5.773502691896262640, -175.0000000040968189 ) ) ;
#33469=CARTESIAN_POINT ( 'NONE',  ( 10.81189881249999729, 0.000000000000000000, -19.34375000204835260 ) ) ;
#33471=CARTESIAN_POINT ( 'NONE',  ( -10.81189881249999907, -6.242252689847864744, -129.4687500020483810 ) ) ;
#33473=CARTESIAN_POINT ( 'NONE',  ( -5.405949406249996869, 9.363379034771805109, -25.03125000204836681 ) ) ;
#33474=CARTESIAN_POINT ( 'NONE',  ( 7.070501591499377789E-16, 11.54700538379251284, -58.62499999999997868 ) ) ;
#33475=CARTESIAN_POINT ( 'NONE',  ( 10.81189881249999729, 0.000000000000000000, -135.0312500020484094 ) ) ;
#33479=( BOUNDED_CURVE ( )  B_SPLINE_CURVE ( 2, ( #33343, #36138, #10009, #29883, #39366, #23188, #19937 ),
 .UNSPECIFIED., .F., .F. ) 
 B_SPLINE_CURVE_WITH_KNOTS ( ( 3, 2, 2, 3 ),
 ( 0.3246268656716419510, 0.3258706467661692807, 0.3271144278606965550, 0.3283582089552238847 ),
 .UNSPECIFIED. ) 
 CURVE ( )  GEOMETRIC_REPRESENTATION_ITEM ( )  RATIONAL_B_SPLINE_CURVE ( ( 0.9999999999999820144, 0.8660254037844566932, 1.000000000000000000, 0.8660254037844387076, 1.000000000000000000, 0.8660254037844387076, 1.000000000000000000 ) ) 
 REPRESENTATION_ITEM ( '' )  );
#33480=CARTESIAN_POINT ( 'NONE',  ( -9.999999999999998224, 1.224646799147353059E-15, -131.7499999999999716 ) ) ;
#33481=CARTESIAN_POINT ( 'NONE',  ( -9.999999999999998224, 5.773502691896259087, -111.2500000040967763 ) ) ;
#33483=CARTESIAN_POINT ( 'NONE',  ( 10.81189881249999551, -6.242252689847874514, -59.96875000204837391 ) ) ;
#33487=CYLINDRICAL_SURFACE ( 'NONE', #17283, 9.999999999999998224 ) ;
#33488=CARTESIAN_POINT ( 'NONE',  ( 4.999999999999992006, -8.660254037844389075, -35.62500000409676915 ) ) ;
#33489=CARTESIAN_POINT ( 'NONE',  ( 9.999999999999998224, 0.000000000000000000, -138.5000000000000000 ) ) ;
#33493=VERTEX_POINT ( 'NONE', #1930 ) ;
#33494=ADVANCED_FACE ( 'NONE', ( #26650 ), #26436, .F. ) ;
#33500=CARTESIAN_POINT ( 'NONE',  ( 10.81189881249999729, 0.000000000000000000, -195.0312500020484094 ) ) ;
#33502=CARTESIAN_POINT ( 'NONE',  ( -9.999999999999998224, 1.224646799147353059E-15, -149.7500000000000000 ) ) ;
#33506=CARTESIAN_POINT ( 'NONE',  ( 10.81189881249999907, 6.242252689847868297, -119.7187500020483810 ) ) ;
#33507=CARTESIAN_POINT ( 'NONE',  ( 7.070501591499377789E-16, 11.54700538379251284, -194.0000000040967905 ) ) ;
#33509=CARTESIAN_POINT ( 'NONE',  ( 7.644554776091147741E-16, 12.48450537969573659, -124.1562500020483952 ) ) ;
#33511=CARTESIAN_POINT ( 'NONE',  ( -10.81189881249999729, 6.242252689847871849, -138.7187500020483810 ) ) ;
#33513=CARTESIAN_POINT ( 'NONE',  ( 5.000000000000000000, 8.660254037844385522, -110.1250000040967763 ) ) ;
#33514=CARTESIAN_POINT ( 'NONE',  ( 9.999999999999998224, 0.000000000000000000, -152.0000000000000000 ) ) ;
#33515=CARTESIAN_POINT ( 'NONE',  ( -4.999999999999996447, 8.660254037844387298, -19.49999999999996092 ) ) ;
#33519=CARTESIAN_POINT ( 'NONE',  ( -5.405949406250003975, -9.363379034771801557, -55.84375000204835970 ) ) ;
#33521=CARTESIAN_POINT ( 'NONE',  ( -2.293366432827344421E-15, -12.48450537969573659, -153.2187500020483810 ) ) ;
#33525=CARTESIAN_POINT ( 'NONE',  ( 10.00000000000000000, 5.773502691896255534, -85.87499999999997158 ) ) ;
#33527=EDGE_LOOP ( 'NONE', ( #13973, #21306, #14001, #23612 ) ) ;
#33528=CARTESIAN_POINT ( 'NONE',  ( -5.405949406250003975, -9.363379034771801557, -113.0312500020483952 ) ) ;
#33529=CARTESIAN_POINT ( 'NONE',  ( 5.000000000000000000, 8.660254037844385522, -135.6250000040967620 ) ) ;
#33534=CARTESIAN_POINT ( 'NONE',  ( 5.405949406249992428, -9.363379034771808662, -51.28125000204835970 ) ) ;
#33552=CARTESIAN_POINT ( 'NONE',  ( -2.293366432827344421E-15, -12.48450537969573659, -151.7187500020483810 ) ) ;
#33553=CARTESIAN_POINT ( 'NONE',  ( -10.81189881249999729, -6.242252689847864744, -165.4687500020483526 ) ) ;
#33556=CARTESIAN_POINT ( 'NONE',  ( -9.999999999999998224, 5.773502691896259087, -179.8750000000000000 ) ) ;
#33561=CARTESIAN_POINT ( 'NONE',  ( 7.644554776091147741E-16, 12.48450537969573659, -185.4687500020483810 ) ) ;
#33564=CARTESIAN_POINT ( 'NONE',  ( -10.81189881249999729, 1.324075727343319199E-15, -48.78125000204838813 ) ) ;
#33566=CARTESIAN_POINT ( 'NONE',  ( 9.999999999999998224, 0.000000000000000000, -108.4999999999999858 ) ) ;
#33568=CARTESIAN_POINT ( 'NONE',  ( 10.81189881249999551, -6.242252689847874514, -130.6562500020483810 ) ) ;
#33570=CARTESIAN_POINT ( 'NONE',  ( 10.81189881249999907, 6.242252689847868297, -149.9062500020484094 ) ) ;
#33573=CARTESIAN_POINT ( 'NONE',  ( 10.81189881249999907, 6.242252689847868297, -80.71875000204838102 ) ) ;
#33576=CARTESIAN_POINT ( 'NONE',  ( 10.81189881249999551, -6.242252689847874514, -182.9687500020484094 ) ) ;
#33579=CARTESIAN_POINT ( 'NONE',  ( 4.999999999999992006, -8.660254037844389075, -171.7500000000000000 ) ) ;
#33581=EDGE_CURVE ( 'NONE', #39928, #39100, #32504, .T. ) ;
#33582=CARTESIAN_POINT ( 'NONE',  ( 7.644554776091147741E-16, 12.48450537969573659, -73.15625000204836681 ) ) ;
#33584=CARTESIAN_POINT ( 'NONE',  ( -10.00000000000000000, -5.773502691896251982, -54.00000000409676204 ) ) ;
#33585=CARTESIAN_POINT ( 'NONE',  ( -5.405949406250003975, -9.363379034771801557, -7.843750002048343717 ) ) ;
#33588=CARTESIAN_POINT ( 'NONE',  ( 7.644554776091147741E-16, 12.48450537969573659, -7.156250002048364145 ) ) ;
#33590=DIRECTION ( 'NONE',  ( -1.000000000000000000, 0.000000000000000000, 0.000000000000000000 ) ) ;
#33591=CARTESIAN_POINT ( 'NONE',  ( 0.000000000000000000, 0.000000000000000000, -99.99999999999998579 ) ) ;
#33598=CARTESIAN_POINT ( 'NONE',  ( 9.999999999999998224, 1.224646799147353059E-15, -99.99999999999998579 ) ) ;
#33599=VERTEX_POINT ( 'NONE', #19950 ) ;
#33606=CARTESIAN_POINT ( 'NONE',  ( -9.999999999999998224, 5.773502691896259087, -47.87499999999996447 ) ) ;
#33607=ADVANCED_FACE ( 'NONE', ( #3566 ), #36568, .F. ) ;
#33618=CARTESIAN_POINT ( 'NONE',  ( 10.81189881249999907, 6.242252689847868297, -70.21875000204838102 ) ) ;
#33619=CARTESIAN_POINT ( 'NONE',  ( -10.81189881249999907, -6.242252689847864744, -78.65625000204839523 ) ) ;
#33621=CARTESIAN_POINT ( 'NONE',  ( -10.81189881249999729, 6.242252689847871849, -155.4062500020483810 ) ) ;
#33622=CARTESIAN_POINT ( 'NONE',  ( -10.81189881249999907, -6.242252689847864744, -171.6562500020484094 ) ) ;
#33623=FACE_OUTER_BOUND ( 'NONE', #33273, .T. ) ;
#33624=CARTESIAN_POINT ( 'NONE',  ( 5.000000000000000000, 8.660254037844385522, -108.6250000040967763 ) ) ;
#33625=CARTESIAN_POINT ( 'NONE',  ( -2.293366432827344421E-15, -12.48450537969573659, -102.2187500020483952 ) ) ;
#33628=CARTESIAN_POINT ( 'NONE',  ( 10.81189881249999551, -6.242252689847874514, -3.156250002048361036 ) ) ;
#33630=CARTESIAN_POINT ( 'NONE',  ( -9.999999999999227285, -5.773502691896698735, -133.5000000040967620 ) ) ;
#33631=CARTESIAN_POINT ( 'NONE',  ( -10.81189881249999907, -6.242252689847864744, -104.1562500020483668 ) ) ;
#33633=ADVANCED_FACE ( 'NONE', ( #29896 ), #335, .F. ) ;
#33634=CARTESIAN_POINT ( 'NONE',  ( 4.999999999999992006, -8.660254037844389075, -73.12500000409677625 ) ) ;
#33636=CARTESIAN_POINT ( 'NONE',  ( 10.81189881249999907, 6.242252689847868297, -35.71875000204835970 ) ) ;
#33640=CARTESIAN_POINT ( 'NONE',  ( -5.405949406250003975, -9.363379034771801557, -26.03125000204836681 ) ) ;
#33643=CARTESIAN_POINT ( 'NONE',  ( -10.00000000000000000, -5.773502691896251982, -3.000000004096753603 ) ) ;
#33653=EDGE_CURVE ( 'NONE', #19199, #30761, #23887, .T. ) ;
#33661=CARTESIAN_POINT ( 'NONE',  ( -2.293366432827344421E-15, -12.48450537969573659, -175.9062500020483810 ) ) ;
#33664=CARTESIAN_POINT ( 'NONE',  ( -2.293366432827344421E-15, -12.48450537969573659, -96.21875000204839523 ) ) ;
#33665=CARTESIAN_POINT ( 'NONE',  ( -2.293366432827344421E-15, -12.48450537969573659, -198.2187500020484379 ) ) ;
#33666=CARTESIAN_POINT ( 'NONE',  ( 5.405949406249992428, -9.363379034771808662, -103.7812500020483810 ) ) ;
#33668=CARTESIAN_POINT ( 'NONE',  ( -2.293366432827344421E-15, -12.48450537969573659, -106.7187500020483668 ) ) ;
#33671=CARTESIAN_POINT ( 'NONE',  ( -10.81189881249999729, 6.242252689847871849, -192.9062500020484094 ) ) ;
#33674=CARTESIAN_POINT ( 'NONE',  ( 4.999999999999992006, -8.660254037844389075, -170.6250000040968189 ) ) ;
#33676=CARTESIAN_POINT ( 'NONE',  ( 10.81189881249999551, -6.242252689847874514, -23.96875000204837391 ) ) ;
#33677=CARTESIAN_POINT ( 'NONE',  ( 10.81189881249999907, 6.242252689847868297, -131.7187500020483810 ) ) ;
#33679=CARTESIAN_POINT ( 'NONE',  ( -5.405949406250003975, -9.363379034771801557, -30.53125000204837036 ) ) ;
#33681=( BOUNDED_CURVE ( )  B_SPLINE_CURVE ( 2, ( #32606, #13559, #3030, #16797, #29996, #442, #36042 ),
 .UNSPECIFIED., .F., .F. ) 
 B_SPLINE_CURVE_WITH_KNOTS ( ( 3, 2, 2, 3 ),
 ( 0.2164179104477612636, 0.2176616915422886489, 0.2189054726368160064, 0.2201492537313433639 ),
 .UNSPECIFIED. ) 
 CURVE ( )  GEOMETRIC_REPRESENTATION_ITEM ( )  RATIONAL_B_SPLINE_CURVE ( ( 0.9999999999999910072, 0.8660254037844477004, 1.000000000000000000, 0.8660254037844387076, 1.000000000000000000, 0.8660254037844297148, 1.000000000000008882 ) ) 
 REPRESENTATION_ITEM ( '' )  );
#33683=CARTESIAN_POINT ( 'NONE',  ( -9.999999999999998224, 1.224646799147353059E-15, -62.74999999999997158 ) ) ;
#33684=CARTESIAN_POINT ( 'NONE',  ( -5.405949406249996869, 9.363379034771805109, -122.5312500020483952 ) ) ;
#33688=CARTESIAN_POINT ( 'NONE',  ( -9.999999999999998224, 1.224646799147353059E-15, -102.1250000040967905 ) ) ;
#33690=CARTESIAN_POINT ( 'NONE',  ( -10.81189881249999907, -6.242252689847864744, -61.96875000204838102 ) ) ;
#33694=CARTESIAN_POINT ( 'NONE',  ( 9.999999999999996447, -5.773502691896262640, -25.00000000409677625 ) ) ;
#33706=CARTESIAN_POINT ( 'NONE',  ( -10.81189881249999729, 1.324075727343319199E-15, -195.7812500020484094 ) ) ;
#33712=CARTESIAN_POINT ( 'NONE',  ( -5.405949406250003975, -9.363379034771801557, -114.3437500020483810 ) ) ;
#33713=CARTESIAN_POINT ( 'NONE',  ( 10.00000000000000000, 5.773502691896255534, -192.7500000040968189 ) ) ;
#33714=CARTESIAN_POINT ( 'NONE',  ( 5.405949406249992428, -9.363379034771808662, -121.7812500020483952 ) ) ;
#33716=CARTESIAN_POINT ( 'NONE',  ( -10.81189881249999729, 6.242252689847871849, -126.7187500020483810 ) ) ;
#33717=CARTESIAN_POINT ( 'NONE',  ( -9.999999999999872102, -5.773502691896326589, -166.5000000040967905 ) ) ;
#33721=CARTESIAN_POINT ( 'NONE',  ( 7.070501591499377789E-16, 11.54700538379251284, -154.6250000000000284 ) ) ;
#33722=CARTESIAN_POINT ( 'NONE',  ( 10.00000000000000000, 5.773502691896255534, -18.37499999999997513 ) ) ;
#33727=CARTESIAN_POINT ( 'NONE',  ( 5.405949406249992428, -9.363379034771808662, -46.59375000204838102 ) ) ;
#33729=CARTESIAN_POINT ( 'NONE',  ( -5.405949406250003975, -9.363379034771801557, -156.3437500020483810 ) ) ;
#33732=CARTESIAN_POINT ( 'NONE',  ( 8.154330677275039463, 6.787768574218738138, -180.0000000000000000 ) ) ;
#33733=CARTESIAN_POINT ( 'NONE',  ( 5.000000000000000000, 8.660254037844385522, -81.24999999999998579 ) ) ;
#33737=CARTESIAN_POINT ( 'NONE',  ( 10.81189881249999551, -6.242252689847874514, -109.6562500020483810 ) ) ;
#33738=CARTESIAN_POINT ( 'NONE',  ( -9.999999999999998224, 1.224646799147353059E-15, -121.6250000040967905 ) ) ;
#33742=CARTESIAN_POINT ( 'NONE',  ( 10.81189881249999907, 6.242252689847868297, -53.90625000204838102 ) ) ;
#33744=CARTESIAN_POINT ( 'NONE',  ( -9.999999999999227285, -5.773502691896698735, -136.1249999999999716 ) ) ;
#33747=CARTESIAN_POINT ( 'NONE',  ( 9.999999999999479527, 5.773502691896553074, -109.8749999999999716 ) ) ;
#33748=ORIENTED_EDGE ( 'NONE', *, *, #33039, .T. ) ;
#33749=CARTESIAN_POINT ( 'NONE',  ( 9.999999999999998224, 0.000000000000000000, -164.3750000040967905 ) ) ;
#33750=ORIENTED_EDGE ( 'NONE', *, *, #5122, .F. ) ;
#33755=ORIENTED_EDGE ( 'NONE', *, *, #36279, .F. ) ;
#33763=CARTESIAN_POINT ( 'NONE',  ( -2.293366432827344421E-15, -12.48450537969573659, -138.2187500020483810 ) ) ;
#33764=CARTESIAN_POINT ( 'NONE',  ( 10.81189881249999729, 0.000000000000000000, -163.3437500020484094 ) ) ;
#33767=CARTESIAN_POINT ( 'NONE',  ( 9.999999999999996447, -5.773502691896262640, -179.1250000000000284 ) ) ;
#33772=CARTESIAN_POINT ( 'NONE',  ( 9.999999999999998224, 0.000000000000000000, -123.8750000040967905 ) ) ;
#33773=CARTESIAN_POINT ( 'NONE',  ( -2.293366432827344421E-15, -12.48450537969573659, -175.7187500020483810 ) ) ;
#33776=CARTESIAN_POINT ( 'NONE',  ( -5.405949406250003975, -9.363379034771801557, -51.53125000204835970 ) ) ;
#33778=CARTESIAN_POINT ( 'NONE',  ( -4.999999999999996447, 8.660254037844387298, -107.9999999999999858 ) ) ;
#33780=CARTESIAN_POINT ( 'NONE',  ( -5.405949406249996869, 9.363379034771805109, -137.5312500020484094 ) ) ;
#33781=CARTESIAN_POINT ( 'NONE',  ( -9.999999999999998224, 1.224646799147353059E-15, -159.1250000040967905 ) ) ;
#33782=CARTESIAN_POINT ( 'NONE',  ( 10.81189881249999729, 0.000000000000000000, -151.5312500020484094 ) ) ;
#33784=CARTESIAN_POINT ( 'NONE',  ( -2.293366432827344421E-15, -12.48450537969573659, -85.71875000204838102 ) ) ;
#33787=CARTESIAN_POINT ( 'NONE',  ( -5.405949406249996869, 9.363379034771805109, -182.3437500020483810 ) ) ;
#33790=CARTESIAN_POINT ( 'NONE',  ( -9.999999999999872102, -5.773502691896326589, -158.6250000000000284 ) ) ;
#33791=CARTESIAN_POINT ( 'NONE',  ( 10.81189881249999729, 0.000000000000000000, -76.53125000204838102 ) ) ;
#33793=CARTESIAN_POINT ( 'NONE',  ( -5.000000000000003553, -8.660254037844383745, -52.37500000409675494 ) ) ;
#33794=CARTESIAN_POINT ( 'NONE',  ( -10.81189881249999729, 1.324075727343319199E-15, -14.09375000204834905 ) ) ;
#33797=CARTESIAN_POINT ( 'NONE',  ( 5.405949406249992428, -9.363379034771808662, -7.781250002048350822 ) ) ;
#33798=FACE_OUTER_BOUND ( 'NONE', #4441, .T. ) ;
#33799=CARTESIAN_POINT ( 'NONE',  ( -9.999999999999868550, 5.773502691896333694, -175.7500000040967905 ) ) ;
#33801=LINE ( 'NONE', #23664, #1523 ) ;
#33806=ORIENTED_EDGE ( 'NONE', *, *, #23049, .T. ) ;
#33808=CARTESIAN_POINT ( 'NONE',  ( -9.999999999999479527, -5.773502691896549521, -123.0000000040967763 ) ) ;
#33810=ORIENTED_EDGE ( 'NONE', *, *, #21970, .T. ) ;
#33815=ADVANCED_FACE ( 'NONE', ( #3983 ), #34206, .F. ) ;
#33816=CARTESIAN_POINT ( 'NONE',  ( 4.999999999999992006, -8.660254037844389075, -44.24999999999998579 ) ) ;
#33819=CARTESIAN_POINT ( 'NONE',  ( 10.81189881249999551, -6.242252689847874514, -167.9687500020483810 ) ) ;
#33829=CARTESIAN_POINT ( 'NONE',  ( 5.405949406249999534, 9.363379034771803333, -67.09375000204836681 ) ) ;
#33830=CARTESIAN_POINT ( 'NONE',  ( 5.405949406249992428, -9.363379034771808662, -79.78125000204838102 ) ) ;
#33832=CARTESIAN_POINT ( 'NONE',  ( -10.81189881249999729, 1.324075727343319199E-15, -161.2812500020484094 ) ) ;
#33833=CARTESIAN_POINT ( 'NONE',  ( -10.81189881249999729, 6.242252689847871849, -174.9062500020483810 ) ) ;
#33835=CARTESIAN_POINT ( 'NONE',  ( 10.81189881249999729, 0.000000000000000000, -1.343750002048366143 ) ) ;
#33837=CARTESIAN_POINT ( 'NONE',  ( 7.644554776091147741E-16, 12.48450537969573659, -107.4687500020483668 ) ) ;
#33839=CARTESIAN_POINT ( 'NONE',  ( 10.81189881249999729, 0.000000000000000000, -4.531250002048375691 ) ) ;
#33843=CARTESIAN_POINT ( 'NONE',  ( 10.81189881249999551, -6.242252689847874514, -99.15625000204838102 ) ) ;
#33845=( BOUNDED_CURVE ( )  B_SPLINE_CURVE ( 2, ( #10261, #19978, #13695, #17154, #10051, #33799, #23231 ),
 .UNSPECIFIED., .F., .F. ) 
 B_SPLINE_CURVE_WITH_KNOTS ( ( 3, 2, 2, 3 ),
 ( 0.1119402985074627876, 0.1131840796019901035, 0.1144278606965174333, 0.1156716417910447492 ),
 .UNSPECIFIED. ) 
 CURVE ( )  GEOMETRIC_REPRESENTATION_ITEM ( )  RATIONAL_B_SPLINE_CURVE ( ( 0.9999999999999894529, 0.8660254037844491437, 1.000000000000000000, 0.8660254037844387076, 1.000000000000000000, 0.8660254037844417052, 0.9999999999999970024 ) ) 
 REPRESENTATION_ITEM ( '' )  );
#33846=CARTESIAN_POINT ( 'NONE',  ( -2.121150477449813534E-15, -11.54700538379251284, -76.25000000409677625 ) ) ;
#33848=CARTESIAN_POINT ( 'NONE',  ( -10.81189881249999729, 6.242252689847871849, -32.21875000204835260 ) ) ;
#33851=CARTESIAN_POINT ( 'NONE',  ( 7.644554776091147741E-16, 12.48450537969573659, -25.15625000204837747 ) ) ;
#33853=CARTESIAN_POINT ( 'NONE',  ( 9.999999999999742428, 5.773502691896404748, -139.8749999999999716 ) ) ;
#33854=CARTESIAN_POINT ( 'NONE',  ( 4.999999999999992006, -8.660254037844389075, -5.625000004096769146 ) ) ;
#33860=DIRECTION ( 'NONE',  ( -0.000000000000000000, -0.000000000000000000, -1.000000000000000000 ) ) ;
#33861=EDGE_LOOP ( 'NONE', ( #34000, #29383, #32954, #42371 ) ) ;
#33868=EDGE_CURVE ( 'NONE', #23753, #22977, #41759, .T. ) ;
#33869=CARTESIAN_POINT ( 'NONE',  ( 2.194755657887257350, 10.56074294295119387, -99.99999999999997158 ) ) ;
#33872=CARTESIAN_POINT ( 'NONE',  ( -10.81189881249999729, 1.324075727343319199E-15, -174.7812500020484094 ) ) ;
#33878=CARTESIAN_POINT ( 'NONE',  ( -2.293366432827344421E-15, -12.48450537969573659, -94.71875000204838102 ) ) ;
#33879=CARTESIAN_POINT ( 'NONE',  ( 7.644554776091147741E-16, 12.48450537969573659, -198.9687500020484094 ) ) ;
#33880=CARTESIAN_POINT ( 'NONE',  ( -10.81189881249999907, -6.242252689847864744, -104.1562500020483668 ) ) ;
#33882=CARTESIAN_POINT ( 'NONE',  ( 10.81189881249999551, -6.242252689847874514, -107.9687500020483810 ) ) ;
#33885=CARTESIAN_POINT ( 'NONE',  ( -5.405949406250003975, -9.363379034771801557, -179.0312500020483810 ) ) ;
#33886=CARTESIAN_POINT ( 'NONE',  ( 5.405949406249992428, -9.363379034771808662, -195.2812500020484094 ) ) ;
#33889=CARTESIAN_POINT ( 'NONE',  ( 7.070501591499377789E-16, 11.54700538379251284, -171.5000000040967905 ) ) ;
#33891=CARTESIAN_POINT ( 'NONE',  ( 7.644554776091147741E-16, 12.48450537969573659, -23.46875000204837391 ) ) ;
#33893=CARTESIAN_POINT ( 'NONE',  ( 5.405949406249999534, 9.363379034771803333, -131.5937500020483810 ) ) ;
#33895=CARTESIAN_POINT ( 'NONE',  ( -10.81189881249999907, -6.242252689847864744, -29.15625000204835970 ) ) ;
#33898=CARTESIAN_POINT ( 'NONE',  ( -2.121150477449813534E-15, -11.54700538379251284, -59.37499999999998579 ) ) ;
#33899=CARTESIAN_POINT ( 'NONE',  ( 10.81189881249999551, -6.242252689847874514, -126.1562500020483810 ) ) ;
#33904=CARTESIAN_POINT ( 'NONE',  ( 5.000000000000000000, 8.660254037844385522, -96.62500000409677625 ) ) ;
#33905=CARTESIAN_POINT ( 'NONE',  ( -2.121150477449813534E-15, -11.54700538379251284, -113.3749999999999858 ) ) ;
#33906=CARTESIAN_POINT ( 'NONE',  ( -5.405949406250003975, -9.363379034771801557, -58.84375000204835970 ) ) ;
#33908=EDGE_CURVE ( 'NONE', #10539, #24722, #28562, .T. ) ;
#33914=CARTESIAN_POINT ( 'NONE',  ( 7.070501591499377789E-16, 11.54700538379251284, -29.00000000409674783 ) ) ;
#33919=CYLINDRICAL_SURFACE ( 'NONE', #39711, 9.999999999999998224 ) ;
#33920=AXIS2_PLACEMENT_3D ( 'NONE', #41160, #30839, #10751 ) ;
#33923=CARTESIAN_POINT ( 'NONE',  ( -10.81189881249999907, -6.242252689847864744, -197.1562500020484379 ) ) ;
#33930=CARTESIAN_POINT ( 'NONE',  ( 10.81189881249999729, 0.000000000000000000, -116.8437500020483810 ) ) ;
#33931=CARTESIAN_POINT ( 'NONE',  ( -2.293366432827344421E-15, -12.48450537969573659, -0.2187500020483512386 ) ) ;
#33932=CARTESIAN_POINT ( 'NONE',  ( 10.81189881249999907, 6.242252689847868297, -124.4062500020483810 ) ) ;
#33934=CARTESIAN_POINT ( 'NONE',  ( 5.405949406249992428, -9.363379034771808662, -133.5937500020483810 ) ) ;
#33937=CARTESIAN_POINT ( 'NONE',  ( -9.999999999999998224, 1.224646799147353059E-15, -152.7500000000000000 ) ) ;
#33938=CARTESIAN_POINT ( 'NONE',  ( -4.999999999999996447, 8.660254037844387298, -17.99999999999996092 ) ) ;
#33939=AXIS2_PLACEMENT_3D ( 'NONE', #3635, #33416, #19797 ) ;
#33945=CARTESIAN_POINT ( 'NONE',  ( 10.81189881249999729, 0.000000000000000000, -49.34375000204838102 ) ) ;
#33946=CARTESIAN_POINT ( 'NONE',  ( -9.999999999999998224, 1.224646799147353059E-15, -111.1250000040967763 ) ) ;
#33947=CARTESIAN_POINT ( 'NONE',  ( 5.405949406249999534, 9.363379034771803333, -157.0937500020483810 ) ) ;
#33950=CARTESIAN_POINT ( 'NONE',  ( -3.091979570676882449, 9.607409082080529572, -180.0000000000000000 ) ) ;
#33951=CARTESIAN_POINT ( 'NONE',  ( -4.999999999999996447, 8.660254037844387298, -85.49999999999998579 ) ) ;
#33954=CARTESIAN_POINT ( 'NONE',  ( -10.81189881249999729, 1.324075727343319199E-15, -104.2812500020483810 ) ) ;
#33955=CARTESIAN_POINT ( 'NONE',  ( -10.00000000000000000, -5.773502691896251982, -123.0000000040968047 ) ) ;
#33959=CARTESIAN_POINT ( 'NONE',  ( -10.81189881249999729, 6.242252689847871849, -51.90625000204837391 ) ) ;
#33964=CARTESIAN_POINT ( 'NONE',  ( -4.999999999999996447, 8.660254037844387298, -165.3750000040967905 ) ) ;
#33972=( BOUNDED_CURVE ( )  B_SPLINE_CURVE ( 2, ( #15198, #40809, #21180, #13835, #27457, #1131, #37380 ),
 .UNSPECIFIED., .F., .F. ) 
 B_SPLINE_CURVE_WITH_KNOTS ( ( 3, 2, 2, 3 ),
 ( 0.1977611940298507898, 0.1990049751243781750, 0.2002487562189055326, 0.2014925373134328901 ),
 .UNSPECIFIED. ) 
 CURVE ( )  GEOMETRIC_REPRESENTATION_ITEM ( )  RATIONAL_B_SPLINE_CURVE ( ( 0.9999999999999940048, 0.8660254037844447028, 1.000000000000000000, 0.8660254037844387076, 1.000000000000000000, 0.8660254037844327124, 1.000000000000005995 ) ) 
 REPRESENTATION_ITEM ( '' )  );
#33978=CARTESIAN_POINT ( 'NONE',  ( 10.81189881249999729, 0.000000000000000000, -139.3437500020484094 ) ) ;
#33979=CARTESIAN_POINT ( 'NONE',  ( -5.405949406249996869, 9.363379034771805109, -152.3437500020483810 ) ) ;
#33982=FACE_OUTER_BOUND ( 'NONE', #12480, .T. ) ;
#33983=CARTESIAN_POINT ( 'NONE',  ( 9.999999999999998224, 0.000000000000000000, -182.0000000000000000 ) ) ;
#33988=CARTESIAN_POINT ( 'NONE',  ( -10.81189881249999907, -6.242252689847864744, -177.4687500020484094 ) ) ;
#33991=CARTESIAN_POINT ( 'NONE',  ( -9.999999999999998224, 1.224646799147353059E-15, -115.2499999999999858 ) ) ;
#33992=CARTESIAN_POINT ( 'NONE',  ( -5.405949406249996869, 9.363379034771805109, -53.53125000204836681 ) ) ;
#33994=CARTESIAN_POINT ( 'NONE',  ( 9.999999999999998224, 0.000000000000000000, -103.9999999999999858 ) ) ;
#33996=CARTESIAN_POINT ( 'NONE',  ( 10.81189881249999729, 0.000000000000000000, -132.0312500020484094 ) ) ;
#33997=CARTESIAN_POINT ( 'NONE',  ( -4.999999999999996447, 8.660254037844387298, -147.3750000040967905 ) ) ;
#33998=CARTESIAN_POINT ( 'NONE',  ( -5.405949406249996869, 9.363379034771805109, -151.0312500020483810 ) ) ;
#34000=ORIENTED_EDGE ( 'NONE', *, *, #30774, .F. ) ;
#34002=CARTESIAN_POINT ( 'NONE',  ( -10.81189881249999729, 6.242252689847871849, -182.2187500020484379 ) ) ;
#34006=CARTESIAN_POINT ( 'NONE',  ( 7.644554776091147741E-16, 12.48450537969573659, -77.65625000204838102 ) ) ;
#34009=CARTESIAN_POINT ( 'NONE',  ( -4.999999999999996447, 8.660254037844387298, -49.87500000409675494 ) ) ;
#34010=CARTESIAN_POINT ( 'NONE',  ( -2.293366432827344421E-15, -12.48450537969573659, -10.71875000204836148 ) ) ;
#34013=CARTESIAN_POINT ( 'NONE',  ( 10.81189881249999551, -6.242252689847874514, -6.156250002048363257 ) ) ;
#34019=ORIENTED_EDGE ( 'NONE', *, *, #3134, .F. ) ;
#34023=EDGE_CURVE ( 'NONE', #19597, #1644, #26896, .T. ) ;
#34029=EDGE_CURVE ( 'NONE', #18647, #2497, #23339, .T. ) ;
#34030=CARTESIAN_POINT ( 'NONE',  ( -9.999999999999998224, 1.224646799147353059E-15, -44.74999999999998579 ) ) ;
#34032=CARTESIAN_POINT ( 'NONE',  ( 10.81189881249999729, 0.000000000000000000, -163.3437500020484094 ) ) ;
#34033=CARTESIAN_POINT ( 'NONE',  ( -10.81189881249999729, -6.242252689847864744, -174.4687500020483526 ) ) ;
#34034=CARTESIAN_POINT ( 'NONE',  ( 9.999999999999998224, 0.000000000000000000, -179.3750000040967905 ) ) ;
#34036=CARTESIAN_POINT ( 'NONE',  ( 5.000000000000000000, 8.660254037844385522, -126.2499999999999716 ) ) ;
#34039=DIRECTION ( 'NONE',  ( -0.000000000000000000, -0.000000000000000000, -1.000000000000000000 ) ) ;
#34042=CARTESIAN_POINT ( 'NONE',  ( 10.81189881249999551, -6.242252689847874514, -73.46875000204835260 ) ) ;
#34043=CARTESIAN_POINT ( 'NONE',  ( 5.405949406249999534, 9.363379034771803333, -77.78125000204838102 ) ) ;
#34045=CARTESIAN_POINT ( 'NONE',  ( 4.999999999999992006, -8.660254037844389075, -128.2499999999999716 ) ) ;
#34046=CARTESIAN_POINT ( 'NONE',  ( -5.405949406250003975, -9.363379034771801557, -161.0312500020484094 ) ) ;
#34047=CARTESIAN_POINT ( 'NONE',  ( -10.81189881249999907, -6.242252689847864744, -176.1562500020483810 ) ) ;
#34050=CARTESIAN_POINT ( 'NONE',  ( -5.405949406249996869, 9.363379034771805109, -107.3437500020483810 ) ) ;
#34053=CARTESIAN_POINT ( 'NONE',  ( 5.405949406249999534, 9.363379034771803333, -1.281250002048373027 ) ) ;
#34057=CARTESIAN_POINT ( 'NONE',  ( -5.405949406250003975, -9.363379034771801557, -98.03125000204839523 ) ) ;
#34059=CARTESIAN_POINT ( 'NONE',  ( -10.00000000000000000, -5.773502691896251982, -75.00000000409677625 ) ) ;
#34061=CARTESIAN_POINT ( 'NONE',  ( -5.405949406250003975, -9.363379034771801557, -31.84375000204836681 ) ) ;
#34064=CARTESIAN_POINT ( 'NONE',  ( -10.81189881249999729, 6.242252689847871849, -27.90625000204838102 ) ) ;
#34067=CARTESIAN_POINT ( 'NONE',  ( 10.00000000000051159, -5.773502691895965988, -118.0000000040967763 ) ) ;
#34068=CARTESIAN_POINT ( 'NONE',  ( 7.070501591499377789E-16, 11.54700538379251284, -3.500000004096753603 ) ) ;
#34074=ORIENTED_EDGE ( 'NONE', *, *, #38167, .T. ) ;
#34081=CARTESIAN_POINT ( 'NONE',  ( -9.999999999999998224, 1.224646799147353059E-15, -156.1250000040967905 ) ) ;
#34082=CARTESIAN_POINT ( 'NONE',  ( 7.644554776091147741E-16, 12.48450537969573659, -173.6562500020483810 ) ) ;
#34085=CARTESIAN_POINT ( 'NONE',  ( -5.405949406250003975, -9.363379034771801557, -94.84375000204838102 ) ) ;
#34087=CARTESIAN_POINT ( 'NONE',  ( 10.81189881249999729, 0.000000000000000000, -100.5312500020483952 ) ) ;
#34089=CARTESIAN_POINT ( 'NONE',  ( -10.81189881249999729, -6.242252689847864744, -105.4687500020483668 ) ) ;
#34091=( BOUNDED_CURVE ( )  B_SPLINE_CURVE ( 2, ( #14152, #36213, #33624, #17190, #33206, #39864, #10720 ),
 .UNSPECIFIED., .F., .F. ) 
 B_SPLINE_CURVE_WITH_KNOTS ( ( 3, 2, 2, 3 ),
 ( 0.4477611940298508730, 0.4490049751243782028, 0.4502487562189055881, 0.4514925373134329734 ),
 .UNSPECIFIED. ) 
 CURVE ( )  GEOMETRIC_REPRESENTATION_ITEM ( )  RATIONAL_B_SPLINE_CURVE ( ( 0.9999999999999880096, 0.8660254037844506980, 1.000000000000000000, 0.8660254037844387076, 1.000000000000000000, 0.8660254037844267172, 1.000000000000011990 ) ) 
 REPRESENTATION_ITEM ( '' )  );
#34092=CARTESIAN_POINT ( 'NONE',  ( -9.999999999999998224, 1.224646799147353059E-15, -107.7499999999999858 ) ) ;
#34093=CARTESIAN_POINT ( 'NONE',  ( -2.121150477449813534E-15, -11.54700538379251284, -152.7500000040967620 ) ) ;
#34094=CARTESIAN_POINT ( 'NONE',  ( -2.293366432827344421E-15, -12.48450537969573659, -195.4062500020484094 ) ) ;
#34097=CARTESIAN_POINT ( 'NONE',  ( 4.999999999999992006, -8.660254037844389075, -172.1250000040968189 ) ) ;
#34099=CARTESIAN_POINT ( 'NONE',  ( -5.405949406249996869, 9.363379034771805109, -24.84375000204835970 ) ) ;
#34100=CARTESIAN_POINT ( 'NONE',  ( -2.293366432827344421E-15, -12.48450537969573659, -127.7187500020483668 ) ) ;
#34102=CARTESIAN_POINT ( 'NONE',  ( 10.81189881249999729, 0.000000000000000000, -25.53125000204836681 ) ) ;
#34106=CARTESIAN_POINT ( 'NONE',  ( 9.999999999999998224, 0.000000000000000000, -58.99999999999997158 ) ) ;
#34107=CARTESIAN_POINT ( 'NONE',  ( 10.81189881249999907, 6.242252689847868297, -122.9062500020484094 ) ) ;
#34111=CARTESIAN_POINT ( 'NONE',  ( 4.999999999999992006, -8.660254037844389075, -103.1250000040967763 ) ) ;
#34112=CARTESIAN_POINT ( 'NONE',  ( 9.999999999999998224, 0.000000000000000000, -150.8750000040967905 ) ) ;
#34114=CARTESIAN_POINT ( 'NONE',  ( 10.81189881249999551, -6.242252689847874514, -61.46875000204837391 ) ) ;
#34120=EDGE_CURVE ( 'NONE', #30972, #20460, #2672, .T. ) ;
#34122=CARTESIAN_POINT ( 'NONE',  ( 5.000000000000000000, 8.660254037844385522, -32.12500000409676204 ) ) ;
#34123=EDGE_CURVE ( 'NONE', #23080, #35880, #32459, .T. ) ;
#34133=FACE_OUTER_BOUND ( 'NONE', #24208, .T. ) ;
#34137=ADVANCED_FACE ( 'NONE', ( #12573 ), #9559, .F. ) ;
#34138=CARTESIAN_POINT ( 'NONE',  ( 7.644554776091147741E-16, 12.48450537969573659, -197.6562500020484379 ) ) ;
#34145=CARTESIAN_POINT ( 'NONE',  ( -5.405949406250003975, -9.363379034771801557, -115.8437500020483810 ) ) ;
#34146=CARTESIAN_POINT ( 'NONE',  ( -4.999999999999996447, 8.660254037844387298, -195.3750000040967905 ) ) ;
#34147=CARTESIAN_POINT ( 'NONE',  ( -5.405949406250003975, -9.363379034771801557, -126.5312500020483952 ) ) ;
#34149=CARTESIAN_POINT ( 'NONE',  ( 10.81189881249999551, -6.242252689847874514, -131.9687500020483810 ) ) ;
#34150=CARTESIAN_POINT ( 'NONE',  ( -10.00000000000012434, 5.773502691896184480, -163.3750000000000000 ) ) ;
#34152=CARTESIAN_POINT ( 'NONE',  ( -10.00000000000000000, -5.773502691896251982, -154.1250000000000284 ) ) ;
#34153=CARTESIAN_POINT ( 'NONE',  ( 10.00000000000000000, 5.773502691896255534, -16.87499999999997513 ) ) ;
#34156=DIRECTION ( 'NONE',  ( -0.000000000000000000, -0.000000000000000000, -1.000000000000000000 ) ) ;
#34158=CARTESIAN_POINT ( 'NONE',  ( 5.405949406249992428, -9.363379034771808662, -49.59375000204838102 ) ) ;
#34159=CARTESIAN_POINT ( 'NONE',  ( 5.405949406249992428, -9.363379034771808662, -156.0937500020483810 ) ) ;
#34162=EDGE_CURVE ( 'NONE', #6210, #7311, #3456, .T. ) ;
#34164=AXIS2_PLACEMENT_3D ( 'NONE', #36566, #19948, #23844 ) ;
#34165=CARTESIAN_POINT ( 'NONE',  ( 9.999999999999998224, 0.000000000000000000, -82.99999999999997158 ) ) ;
#34168=CARTESIAN_POINT ( 'NONE',  ( 5.405949406249999534, 9.363379034771803333, -104.7812500020483810 ) ) ;
#34169=CARTESIAN_POINT ( 'NONE',  ( 9.999999999999996447, -5.773502691896262640, -127.0000000040967763 ) ) ;
#34174=CARTESIAN_POINT ( 'NONE',  ( 5.405949406249992428, -9.363379034771808662, -48.28125000204838813 ) ) ;
#34197=CARTESIAN_POINT ( 'NONE',  ( 10.81189881249999907, 6.242252689847868297, -142.2187500020484094 ) ) ;
#34198=CARTESIAN_POINT ( 'NONE',  ( -10.81189881249999729, 6.242252689847871849, -150.9062500020484094 ) ) ;
#34199=CARTESIAN_POINT ( 'NONE',  ( 10.81189881249999729, 0.000000000000000000, -151.3437500020483810 ) ) ;
#34202=CARTESIAN_POINT ( 'NONE',  ( -10.00000000000000000, -5.773502691896251982, -182.6250000000000284 ) ) ;
#34204=CYLINDRICAL_SURFACE ( 'NONE', #30708, 9.999999999999998224 ) ;
#34206=CYLINDRICAL_SURFACE ( 'NONE', #35097, 9.999999999999998224 ) ;
#34207=CARTESIAN_POINT ( 'NONE',  ( -10.81189881249999729, 1.324075727343319199E-15, -179.0937500020484094 ) ) ;
#34210=CARTESIAN_POINT ( 'NONE',  ( 7.070501591499376803E-16, 11.54700538379251284, -115.6249999999999858 ) ) ;
#34211=CARTESIAN_POINT ( 'NONE',  ( -2.293366432827344421E-15, -12.48450537969573659, -42.40625000204836681 ) ) ;
#34213=CARTESIAN_POINT ( 'NONE',  ( 7.070501591499377789E-16, 11.54700538379251284, -109.6249999999999858 ) ) ;
#34215=CARTESIAN_POINT ( 'NONE',  ( 10.81189881249999729, 6.242252689847867408, -130.4062500020483810 ) ) ;
#34216=CARTESIAN_POINT ( 'NONE',  ( 9.999999999999998224, 0.000000000000000000, -144.8750000040967905 ) ) ;
#34221=CARTESIAN_POINT ( 'NONE',  ( -10.81189881249999907, -6.242252689847864744, -169.9687500020484094 ) ) ;
#34225=CARTESIAN_POINT ( 'NONE',  ( 10.81189881249999551, -6.242252689847874514, -78.15625000204838102 ) ) ;
#34227=CARTESIAN_POINT ( 'NONE',  ( -2.121150477449813534E-15, -11.54700538379251284, -52.25000000409676915 ) ) ;
#34228=CARTESIAN_POINT ( 'NONE',  ( -10.81189881249999907, -6.242252689847864744, -3.468750002048353931 ) ) ;
#34231=CARTESIAN_POINT ( 'NONE',  ( -9.999999999999998224, 1.224646799147353059E-15, -160.6250000040967905 ) ) ;
#34233=CARTESIAN_POINT ( 'NONE',  ( -9.999999999999998224, 1.224646799147353059E-15, -103.6250000040967763 ) ) ;
#34237=EDGE_CURVE ( 'NONE', #30244, #21752, #25766, .T. ) ;
#34242=EDGE_LOOP ( 'NONE', ( #27260, #38831, #23649, #14283 ) ) ;
#34249=CARTESIAN_POINT ( 'NONE',  ( 10.00000000000000000, 5.773502691896255534, -42.37499999999996447 ) ) ;
#34251=CARTESIAN_POINT ( 'NONE',  ( 10.81189881249999729, 0.000000000000000000, -164.8437500020484094 ) ) ;
#34253=CARTESIAN_POINT ( 'NONE',  ( 0.000000000000000000, 0.000000000000000000, -99.99999999999998579 ) ) ;
#34261=CARTESIAN_POINT ( 'NONE',  ( -5.405949406250003975, -9.363379034771801557, -60.34375000204835970 ) ) ;
#34262=CARTESIAN_POINT ( 'NONE',  ( 10.81189881249999729, 0.000000000000000000, -72.03125000204838102 ) ) ;
#34264=CARTESIAN_POINT ( 'NONE',  ( -9.999999999999998224, 5.773502691896259087, -130.3750000000000000 ) ) ;
#34265=CARTESIAN_POINT ( 'NONE',  ( -10.81189881249999729, 1.324075727343319199E-15, -152.2812500020484094 ) ) ;
#34266=CARTESIAN_POINT ( 'NONE',  ( -10.81189881249999729, 1.324075727343319199E-15, -164.2812500020484094 ) ) ;
#34267=CARTESIAN_POINT ( 'NONE',  ( 4.999999999999992006, -8.660254037844389075, -145.1250000040967905 ) ) ;
#34269=CARTESIAN_POINT ( 'NONE',  ( 5.405949406249999534, 9.363379034771803333, -97.09375000204838102 ) ) ;
#34272=CARTESIAN_POINT ( 'NONE',  ( -10.81189881249999729, 1.324075727343319199E-15, -3.781250002048375247 ) ) ;
#34275=CARTESIAN_POINT ( 'NONE',  ( -5.405949406250003975, -9.363379034771801557, -96.53125000204839523 ) ) ;
#34277=CARTESIAN_POINT ( 'NONE',  ( 5.000000000000000000, 8.660254037844385522, -75.62500000409677625 ) ) ;
#34278=CARTESIAN_POINT ( 'NONE',  ( -9.999999999999998224, 1.224646799147353059E-15, -134.7499999999999716 ) ) ;
#34279=CARTESIAN_POINT ( 'NONE',  ( 10.81189881249999729, 0.000000000000000000, -34.34375000204836681 ) ) ;
#34282=CARTESIAN_POINT ( 'NONE',  ( 10.81189881249999551, -6.242252689847874514, -28.65625000204838102 ) ) ;
#34284=CARTESIAN_POINT ( 'NONE',  ( 5.000000000000000000, 8.660254037844385522, -6.625000004096770923 ) ) ;
#34298=DIRECTION ( 'NONE',  ( 0.000000000000000000, 0.000000000000000000, -1.000000000000000000 ) ) ;
#34300=CARTESIAN_POINT ( 'NONE',  ( -10.81189881249999729, 1.324075727343319199E-15, -164.2812500020484094 ) ) ;
#34302=ADVANCED_FACE ( 'NONE', ( #25974 ), #22519, .F. ) ;
#34305=CARTESIAN_POINT ( 'NONE',  ( -2.293366432827344421E-15, -12.48450537969573659, -97.71875000204838102 ) ) ;
#34307=CARTESIAN_POINT ( 'NONE',  ( 5.405949406249992428, -9.363379034771808662, -195.0937500020484094 ) ) ;
#34308=CARTESIAN_POINT ( 'NONE',  ( -10.81189881249999907, -6.242252689847864744, -96.65625000204839523 ) ) ;
#34310=CARTESIAN_POINT ( 'NONE',  ( 5.405949406249992428, -9.363379034771808662, -105.0937500020483810 ) ) ;
#34314=CARTESIAN_POINT ( 'NONE',  ( 5.405949406249999534, 9.363379034771803333, -196.2812500020484094 ) ) ;
#34316=CARTESIAN_POINT ( 'NONE',  ( -9.999999999999998224, 1.224646799147353059E-15, -171.1250000040968189 ) ) ;
#34318=CARTESIAN_POINT ( 'NONE',  ( 10.81189881249999551, -6.242252689847874514, -22.46875000204837036 ) ) ;
#34320=CARTESIAN_POINT ( 'NONE',  ( -5.405949406250003975, -9.363379034771801557, -129.3437500020484094 ) ) ;
#34322=CARTESIAN_POINT ( 'NONE',  ( 10.81189881249999729, 0.000000000000000000, -28.53125000204837036 ) ) ;
#34324=CARTESIAN_POINT ( 'NONE',  ( -5.000000000000003553, -8.660254037844383745, -48.99999999999998579 ) ) ;
#34325=CARTESIAN_POINT ( 'NONE',  ( -5.405949406249996869, 9.363379034771805109, -125.5312500020483952 ) ) ;
#34327=ORIENTED_EDGE ( 'NONE', *, *, #3505, .T. ) ;
#34328=CARTESIAN_POINT ( 'NONE',  ( 7.070501591499377789E-16, 11.54700538379251284, -102.5000000040967763 ) ) ;
#34331=CARTESIAN_POINT ( 'NONE',  ( 7.644554776091147741E-16, 12.48450537969573659, -54.96875000204836681 ) ) ;
#34338=CARTESIAN_POINT ( 'NONE',  ( -5.000000000000003553, -8.660254037844383745, -29.87500000409676204 ) ) ;
#34342=CARTESIAN_POINT ( 'NONE',  ( 5.000000000000000000, 8.660254037844385522, -129.6250000040967620 ) ) ;
#34345=ORIENTED_EDGE ( 'NONE', *, *, #18012, .T. ) ;
#34346=ORIENTED_EDGE ( 'NONE', *, *, #32330, .T. ) ;
#34348=( BOUNDED_CURVE ( )  B_SPLINE_CURVE ( 2, ( #35225, #27674, #11895, #40812, #37595, #8680, #5221 ),
 .UNSPECIFIED., .F., .F. ) 
 B_SPLINE_CURVE_WITH_KNOTS ( ( 3, 2, 2, 3 ),
 ( 0.1753731343283582433, 0.1766169154228856009, 0.1778606965174129861, 0.1791044776119403437 ),
 .UNSPECIFIED. ) 
 CURVE ( )  GEOMETRIC_REPRESENTATION_ITEM ( )  RATIONAL_B_SPLINE_CURVE ( ( 0.9999999999999970024, 0.8660254037844417052, 1.000000000000000000, 0.8660254037844387076, 1.000000000000000000, 0.8660254037844327124, 1.000000000000005995 ) ) 
 REPRESENTATION_ITEM ( '' )  );
#34350=CARTESIAN_POINT ( 'NONE',  ( 10.81189881249999551, -6.242252689847874514, -186.1562500020484379 ) ) ;
#34359=CARTESIAN_POINT ( 'NONE',  ( 5.405949406249992428, -9.363379034771808662, -114.0937500020483810 ) ) ;
#34360=CARTESIAN_POINT ( 'NONE',  ( -4.999999999999996447, 8.660254037844387298, -193.8750000040967905 ) ) ;
#34361=CARTESIAN_POINT ( 'NONE',  ( 10.81189881249999729, 0.000000000000000000, -126.0312500020483952 ) ) ;
#34363=CARTESIAN_POINT ( 'NONE',  ( -2.293366432827344421E-15, -12.48450537969573659, -133.7187500020483810 ) ) ;
#34364=CARTESIAN_POINT ( 'NONE',  ( 9.999999999999994671, -5.773502691896262640, -166.0000000040967905 ) ) ;
#34366=CARTESIAN_POINT ( 'NONE',  ( -4.999999999999996447, 8.660254037844387298, -145.5000000000000000 ) ) ;
#34367=CARTESIAN_POINT ( 'NONE',  ( -9.999999999999998224, 5.773502691896259087, -20.87499999999997868 ) ) ;
#34370=CARTESIAN_POINT ( 'NONE',  ( -2.121150477449813534E-15, -11.54700538379251284, -170.3750000000000000 ) ) ;
#34372=CARTESIAN_POINT ( 'NONE',  ( -2.293366432827344421E-15, -12.48450537969573659, -43.71875000204835970 ) ) ;
#34374=CARTESIAN_POINT ( 'NONE',  ( 10.81189881249999551, -6.242252689847874514, -154.4687500020484094 ) ) ;
#34377=CARTESIAN_POINT ( 'NONE',  ( 5.502678791411631742, 8.887464070476337241, -179.9999999999999432 ) ) ;
#34378=CARTESIAN_POINT ( 'NONE',  ( 9.999999999999996447, -5.773502691896262640, -74.12499999999997158 ) ) ;
#34380=VERTEX_POINT ( 'NONE', #4368 ) ;
#34381=CARTESIAN_POINT ( 'NONE',  ( -10.81189881249999729, 1.324075727343319199E-15, -101.2812500020483952 ) ) ;
#34382=CARTESIAN_POINT ( 'NONE',  ( -2.121150477449813534E-15, -11.54700538379251284, -122.7500000040967905 ) ) ;
#34386=CARTESIAN_POINT ( 'NONE',  ( -10.81189881249999729, 1.324075727343319199E-15, -45.78125000204838813 ) ) ;
#34392=ORIENTED_EDGE ( 'NONE', *, *, #18399, .T. ) ;
#34406=CARTESIAN_POINT ( 'NONE',  ( -10.81189881249999907, -6.242252689847864744, -142.9687500020484094 ) ) ;
#34407=CARTESIAN_POINT ( 'NONE',  ( -5.405949406249996869, 9.363379034771805109, -151.0312500020483810 ) ) ;
#34408=CARTESIAN_POINT ( 'NONE',  ( 5.405949406249992428, -9.363379034771808662, -151.5937500020483810 ) ) ;
#34409=EDGE_CURVE ( 'NONE', #42377, #5520, #21099, .T. ) ;
#34412=CARTESIAN_POINT ( 'NONE',  ( -5.000000000000003553, -8.660254037844383745, -167.5000000000000000 ) ) ;
#34413=EDGE_CURVE ( 'NONE', #41597, #1789, #25537, .T. ) ;
#34418=CARTESIAN_POINT ( 'NONE',  ( 10.81189881249999729, 0.000000000000000000, -178.3437500020483810 ) ) ;
#34421=DIRECTION ( 'NONE',  ( -0.000000000000000000, -0.000000000000000000, -1.000000000000000000 ) ) ;
#34422=CARTESIAN_POINT ( 'NONE',  ( -5.405949406249996869, 9.363379034771805109, -44.53125000204838102 ) ) ;
#34424=CARTESIAN_POINT ( 'NONE',  ( -9.999999999999998224, 5.773502691896259087, -110.8749999999999858 ) ) ;
#34426=CARTESIAN_POINT ( 'NONE',  ( 5.405949406249992428, -9.363379034771808662, -127.7812500020483810 ) ) ;
#34427=CARTESIAN_POINT ( 'NONE',  ( 10.00000000000000000, 5.773502691896255534, -144.7500000040967905 ) ) ;
#34432=CARTESIAN_POINT ( 'NONE',  ( 5.405949406249999534, 9.363379034771803333, -172.0937500020484094 ) ) ;
#34436=CARTESIAN_POINT ( 'NONE',  ( 5.405949406249992428, -9.363379034771808662, -69.28125000204838102 ) ) ;
#34439=CARTESIAN_POINT ( 'NONE',  ( 4.999999999999992006, -8.660254037844389075, -46.12500000409677625 ) ) ;
#34441=CARTESIAN_POINT ( 'NONE',  ( -5.405949406249996869, 9.363379034771805109, -2.343750002048366810 ) ) ;
#34448=( BOUNDED_CURVE ( )  B_SPLINE_CURVE ( 2, ( #36813, #26888, #27105, #30356, #3600, #6614, #40043 ),
 .UNSPECIFIED., .F., .F. ) 
 B_SPLINE_CURVE_WITH_KNOTS ( ( 3, 2, 2, 3 ),
 ( 0.1044776119402986148, 0.1057213930348259306, 0.1069651741293532465, 0.1082089552238805485 ),
 .UNSPECIFIED. ) 
 CURVE ( )  GEOMETRIC_REPRESENTATION_ITEM ( )  RATIONAL_B_SPLINE_CURVE ( ( 0.9999999999999880096, 0.8660254037844506980, 1.000000000000000000, 0.8660254037844387076, 1.000000000000000000, 0.8660254037844431485, 0.9999999999999955591 ) ) 
 REPRESENTATION_ITEM ( '' )  );
#34449=DIRECTION ( 'NONE',  ( -0.000000000000000000, -0.000000000000000000, -1.000000000000000000 ) ) ;
#34454=ORIENTED_EDGE ( 'NONE', *, *, #16750, .F. ) ;
#34458=AXIS2_PLACEMENT_3D ( 'NONE', #26886, #156, #33590 ) ;
#34461=CARTESIAN_POINT ( 'NONE',  ( -9.999999999999998224, 5.773502691896259087, -34.37499999999996447 ) ) ;
#34463=CARTESIAN_POINT ( 'NONE',  ( 10.81189881249999551, -6.242252689847874514, -166.4687500020484094 ) ) ;
#34464=CARTESIAN_POINT ( 'NONE',  ( 5.405949406249999534, 9.363379034771803333, -178.0937500020484094 ) ) ;
#34470=CARTESIAN_POINT ( 'NONE',  ( 9.999999999999998224, 0.000000000000000000, -111.4999999999999858 ) ) ;
#34473=CARTESIAN_POINT ( 'NONE',  ( 10.81189881249999907, 6.242252689847868297, -62.71875000204838102 ) ) ;
#34474=CARTESIAN_POINT ( 'NONE',  ( 10.81189881249999907, 6.242252689847868297, -71.90625000204836681 ) ) ;
#34476=CARTESIAN_POINT ( 'NONE',  ( 7.070501591499377789E-16, 11.54700538379251284, -129.1250000000000000 ) ) ;
#34478=CARTESIAN_POINT ( 'NONE',  ( 10.81189881249999729, 6.242252689847867408, -149.9062500020484094 ) ) ;
#34479=CARTESIAN_POINT ( 'NONE',  ( 10.81189881249999729, 0.000000000000000000, -163.5312500020484094 ) ) ;
#34482=CARTESIAN_POINT ( 'NONE',  ( -10.00000000000025580, 5.773502691896109873, -159.2500000040968189 ) ) ;
#34483=CARTESIAN_POINT ( 'NONE',  ( 7.644554776091147741E-16, 12.48450537969573659, -99.96875000204839523 ) ) ;
#34486=CARTESIAN_POINT ( 'NONE',  ( -10.81189881249999729, 6.242252689847871849, -195.7187500020484379 ) ) ;
#34488=CARTESIAN_POINT ( 'NONE',  ( 3.754465651702444173, -9.907696901662989220, -180.0000000000000000 ) ) ;
#34489=CARTESIAN_POINT ( 'NONE',  ( 5.405949406249999534, 9.363379034771803333, -94.28125000204838102 ) ) ;
#34492=CARTESIAN_POINT ( 'NONE',  ( 9.999999999999996447, -5.773502691896262640, -65.50000000409677625 ) ) ;
#34493=CARTESIAN_POINT ( 'NONE',  ( -10.81189881249999907, -6.242252689847864744, -28.96875000204835260 ) ) ;
#34497=CARTESIAN_POINT ( 'NONE',  ( 10.81189881249999551, -6.242252689847874514, -31.65625000204835615 ) ) ;
#34500=CARTESIAN_POINT ( 'NONE',  ( 9.999999999999998224, 0.000000000000000000, -5.375000004096769146 ) ) ;
#34501=CARTESIAN_POINT ( 'NONE',  ( 4.999999999999992006, -8.660254037844389075, -138.7499999999999716 ) ) ;
#34508=CARTESIAN_POINT ( 'NONE',  ( 9.999999999999998224, 0.000000000000000000, -170.3750000040968189 ) ) ;
#34515=CARTESIAN_POINT ( 'NONE',  ( 4.999999999999992006, -8.660254037844389075, -128.6250000040967620 ) ) ;
#34516=LINE ( 'NONE', #31281, #4001 ) ;
#34517=CARTESIAN_POINT ( 'NONE',  ( 7.644554776091147741E-16, 12.48450537969573659, -167.6562500020483810 ) ) ;
#34521=CARTESIAN_POINT ( 'NONE',  ( 7.644554776091147741E-16, 12.48450537969573659, -84.96875000204835260 ) ) ;
#34523=CARTESIAN_POINT ( 'NONE',  ( 10.81189881249999551, -6.242252689847874514, -196.4687500020484094 ) ) ;
#34524=CARTESIAN_POINT ( 'NONE',  ( -2.293366432827344421E-15, -12.48450537969573659, -94.90625000204838102 ) ) ;
#34527=CARTESIAN_POINT ( 'NONE',  ( -5.405949406249996869, 9.363379034771805109, -176.5312500020483810 ) ) ;
#34528=CARTESIAN_POINT ( 'NONE',  ( 10.81189881249999729, 0.000000000000000000, -190.5312500020484094 ) ) ;
#34530=CARTESIAN_POINT ( 'NONE',  ( -2.121150477449813534E-15, -11.54700538379251284, -166.2500000040968189 ) ) ;
#34532=CARTESIAN_POINT ( 'NONE',  ( 5.405949406249999534, 9.363379034771803333, -10.09375000204834549 ) ) ;
#34534=CARTESIAN_POINT ( 'NONE',  ( -5.405949406250003975, -9.363379034771801557, -123.3437500020483952 ) ) ;
#34536=CARTESIAN_POINT ( 'NONE',  ( 10.81189881249999551, -6.242252689847874514, -22.65625000204837747 ) ) ;
#34538=CARTESIAN_POINT ( 'NONE',  ( 4.999999999999992006, -8.660254037844389075, -51.74999999999996447 ) ) ;
#34539=CARTESIAN_POINT ( 'NONE',  ( 10.81189881249999729, 0.000000000000000000, -112.5312500020483952 ) ) ;
#34541=ORIENTED_EDGE ( 'NONE', *, *, #14180, .T. ) ;
#34542=CARTESIAN_POINT ( 'NONE',  ( -2.121150477449813534E-15, -11.54700538379251284, -97.25000000409679046 ) ) ;
#34545=CARTESIAN_POINT ( 'NONE',  ( -10.81189881249999729, 1.324075727343319199E-15, -47.09375000204838102 ) ) ;
#34546=EDGE_LOOP ( 'NONE', ( #208, #30936, #19272, #39666 ) ) ;
#34551=CARTESIAN_POINT ( 'NONE',  ( -4.999999999999996447, 8.660254037844387298, -27.37500000409676204 ) ) ;
#34553=CARTESIAN_POINT ( 'NONE',  ( -9.999999999999998224, 1.224646799147353059E-15, -167.7500000000000000 ) ) ;
#34555=LINE ( 'NONE', #12078, #16225 ) ;
#34556=ORIENTED_EDGE ( 'NONE', *, *, #26106, .T. ) ;
#34559=ORIENTED_EDGE ( 'NONE', *, *, #20347, .F. ) ;
#34563=CARTESIAN_POINT ( 'NONE',  ( -9.999999999999868550, 5.773502691896333694, -174.2500000040967905 ) ) ;
#34565=CARTESIAN_POINT ( 'NONE',  ( -5.405949406250003975, -9.363379034771801557, -185.0312500020484094 ) ) ;
#34570=CARTESIAN_POINT ( 'NONE',  ( -5.405949406250003975, -9.363379034771801557, -111.3437500020483810 ) ) ;
#34572=CARTESIAN_POINT ( 'NONE',  ( 10.81189881249999551, -6.242252689847874514, -112.6562500020483810 ) ) ;
#34574=CARTESIAN_POINT ( 'NONE',  ( 5.405949406249992428, -9.363379034771808662, -127.5937500020483668 ) ) ;
#34578=CARTESIAN_POINT ( 'NONE',  ( 9.999999999999998224, 0.000000000000000000, -147.5000000000000000 ) ) ;
#34579=CARTESIAN_POINT ( 'NONE',  ( 9.999999999999998224, 0.000000000000000000, -9.499999999999953815 ) ) ;
#34585=CARTESIAN_POINT ( 'NONE',  ( 10.81189881249999729, 0.000000000000000000, -41.84375000204837391 ) ) ;
#34587=CARTESIAN_POINT ( 'NONE',  ( -5.405949406250003975, -9.363379034771801557, -144.3437500020483810 ) ) ;
#34590=CARTESIAN_POINT ( 'NONE',  ( 9.999999999999996447, -5.773502691896262640, -78.62499999999998579 ) ) ;
#34592=VERTEX_POINT ( 'NONE', #30914 ) ;
#34593=CARTESIAN_POINT ( 'NONE',  ( 10.81189881249999729, 6.242252689847867408, -100.4062500020483952 ) ) ;
#34594=CARTESIAN_POINT ( 'NONE',  ( 5.000000000000000000, 8.660254037844385522, -126.6250000040967620 ) ) ;
#34595=CARTESIAN_POINT ( 'NONE',  ( -5.000000000000003553, -8.660254037844383745, -143.8750000040967905 ) ) ;
#34596=CARTESIAN_POINT ( 'NONE',  ( 10.81189881249999551, -6.242252689847874514, -79.46875000204838102 ) ) ;
#34599=CARTESIAN_POINT ( 'NONE',  ( 9.999999999999742428, 5.773502691896404748, -130.8749999999999716 ) ) ;
#34600=CARTESIAN_POINT ( 'NONE',  ( -10.81189881249999729, 1.324075727343319199E-15, -47.28125000204838813 ) ) ;
#34607=CARTESIAN_POINT ( 'NONE',  ( 9.999999999999998224, 0.000000000000000000, -173.3750000040968189 ) ) ;
#34610=( BOUNDED_CURVE ( )  B_SPLINE_CURVE ( 2, ( #35265, #5699, #8503, #21655, #19057, #28147, #18194 ),
 .UNSPECIFIED., .F., .T. ) 
 B_SPLINE_CURVE_WITH_KNOTS ( ( 3, 2, 2, 3 ),
 ( 0.3582089552238806873, 0.3594527363184080726, 0.3606965174129355134, 0.3619402985074628432 ),
 .UNSPECIFIED. ) 
 CURVE ( )  GEOMETRIC_REPRESENTATION_ITEM ( )  RATIONAL_B_SPLINE_CURVE ( ( 0.9999999999999880096, 0.8660254037844506980, 1.000000000000000000, 0.8660254037844387076, 1.000000000000000000, 0.8660254037844207220, 1.000000000000017986 ) ) 
 REPRESENTATION_ITEM ( '' )  );
#34619=CARTESIAN_POINT ( 'NONE',  ( 5.405949406249999534, 9.363379034771803333, -136.0937500020483810 ) ) ;
#34620=CARTESIAN_POINT ( 'NONE',  ( -5.405949406249996869, 9.363379034771805109, -146.5312500020483810 ) ) ;
#34621=CARTESIAN_POINT ( 'NONE',  ( 5.405949406249999534, 9.363379034771803333, -154.0937500020483810 ) ) ;
#34624=CARTESIAN_POINT ( 'NONE',  ( 4.999999999999992006, -8.660254037844389075, -170.2500000000000000 ) ) ;
#34626=CARTESIAN_POINT ( 'NONE',  ( -9.999999999999998224, 0.000000000000000000, -99.99999999999998579 ) ) ;
#34628=CARTESIAN_POINT ( 'NONE',  ( -9.281563073697167709, 5.229554528500406363, -100.0000000000000000 ) ) ;
#34629=CARTESIAN_POINT ( 'NONE',  ( -10.81189881249999729, 6.242252689847871849, -176.2187500020483810 ) ) ;
#34633=CARTESIAN_POINT ( 'NONE',  ( 7.644554776091147741E-16, 12.48450537969573659, -43.15625000204837391 ) ) ;
#34635=CARTESIAN_POINT ( 'NONE',  ( -2.121150477449813534E-15, -11.54700538379251284, -96.87500000000000000 ) ) ;
#34638=CARTESIAN_POINT ( 'NONE',  ( 10.81189881249999729, 0.000000000000000000, -129.0312500020484094 ) ) ;
#34639=CARTESIAN_POINT ( 'NONE',  ( -5.000000000000003553, -8.660254037844383745, -151.3750000040967905 ) ) ;
#34640=CARTESIAN_POINT ( 'NONE',  ( 9.999999999999994671, -5.773502691896262640, -167.1250000000000000 ) ) ;
#34643=CARTESIAN_POINT ( 'NONE',  ( 7.644554776091147741E-16, 12.48450537969573659, -171.9687500020483810 ) ) ;
#34647=CARTESIAN_POINT ( 'NONE',  ( 10.81189881249999551, -6.242252689847874514, -66.15625000204839523 ) ) ;
#34648=CARTESIAN_POINT ( 'NONE',  ( 5.000000000000000000, 8.660254037844385522, -41.12500000409677625 ) ) ;
#34649=CARTESIAN_POINT ( 'NONE',  ( -10.81189881249999729, 1.324075727343319199E-15, -2.093750002048366810 ) ) ;
#34652=AXIS2_PLACEMENT_3D ( 'NONE', #19183, #22643, #5397 ) ;
#34654=EDGE_CURVE ( 'NONE', #33286, #2320, #16450, .T. ) ;
#34656=DIRECTION ( 'NONE',  ( -1.000000000000000000, 0.000000000000000000, 0.000000000000000000 ) ) ;
#34658=EDGE_CURVE ( 'NONE', #13418, #7848, #34348, .T. ) ;
#34668=ORIENTED_EDGE ( 'NONE', *, *, #19927, .F. ) ;
#34673=ORIENTED_EDGE ( 'NONE', *, *, #38372, .T. ) ;
#34674=CARTESIAN_POINT ( 'NONE',  ( -9.999999999999998224, 1.224646799147353059E-15, -148.2500000000000000 ) ) ;
#34675=CARTESIAN_POINT ( 'NONE',  ( 4.999999999999992006, -8.660254037844389075, -38.24999999999997868 ) ) ;
#34679=CARTESIAN_POINT ( 'NONE',  ( -10.81189881249999907, -6.242252689847864744, -165.4687500020484094 ) ) ;
#34682=CARTESIAN_POINT ( 'NONE',  ( 0.000000000000000000, 0.000000000000000000, -99.99999999999998579 ) ) ;
#34684=CARTESIAN_POINT ( 'NONE',  ( -4.999999999999996447, 8.660254037844387298, -195.0000000000000000 ) ) ;
#34689=CARTESIAN_POINT ( 'NONE',  ( 10.81189881249999551, -6.242252689847874514, -58.46875000204837391 ) ) ;
#34690=CARTESIAN_POINT ( 'NONE',  ( -5.405949406250003975, -9.363379034771801557, -71.03125000204838102 ) ) ;
#34692=CARTESIAN_POINT ( 'NONE',  ( 10.00000000000000000, 5.773502691896255534, -120.3749999999999858 ) ) ;
#34693=CARTESIAN_POINT ( 'NONE',  ( -10.81189881249999729, 6.242252689847871849, -149.4062500020484094 ) ) ;
#34694=CARTESIAN_POINT ( 'NONE',  ( -2.293366432827344421E-15, -12.48450537969573659, -162.4062500020483810 ) ) ;
#34697=CARTESIAN_POINT ( 'NONE',  ( -2.293366432827344421E-15, -12.48450537969573659, -100.7187500020483952 ) ) ;
#34700=CARTESIAN_POINT ( 'NONE',  ( -10.81189881249999729, 1.324075727343319199E-15, -198.5937500020484094 ) ) ;
#34702=ADVANCED_FACE ( 'NONE', ( #38027 ), #14699, .F. ) ;
#34704=CARTESIAN_POINT ( 'NONE',  ( 5.405949406249999534, 9.363379034771803333, -91.28125000204838102 ) ) ;
#34706=CARTESIAN_POINT ( 'NONE',  ( -10.00000000000000000, -5.773502691896251982, -67.50000000409679046 ) ) ;
#34708=CARTESIAN_POINT ( 'NONE',  ( 10.81189881249999729, 0.000000000000000000, -25.34375000204835970 ) ) ;
#34711=CARTESIAN_POINT ( 'NONE',  ( 10.81189881249999551, -6.242252689847874514, -24.15625000204837747 ) ) ;
#34714=DIRECTION ( 'NONE',  ( -1.000000000000000000, 0.000000000000000000, 0.000000000000000000 ) ) ;
#34730=( BOUNDED_CURVE ( )  B_SPLINE_CURVE ( 2, ( #3018, #16141, #22437, #18773, #42272, #25688, #35406 ),
 .UNSPECIFIED., .F., .F. ) 
 B_SPLINE_CURVE_WITH_KNOTS ( ( 3, 2, 2, 3 ),
 ( 0.2350746268656717097, 0.2363184079601990950, 0.2375621890547264525, 0.2388059701492538378 ),
 .UNSPECIFIED. ) 
 CURVE ( )  GEOMETRIC_REPRESENTATION_ITEM ( )  RATIONAL_B_SPLINE_CURVE ( ( 0.9999999999999940048, 0.8660254037844447028, 1.000000000000000000, 0.8660254037844387076, 1.000000000000000000, 0.8660254037844267172, 1.000000000000011990 ) ) 
 REPRESENTATION_ITEM ( '' )  );
#34732=CARTESIAN_POINT ( 'NONE',  ( 10.81189881249999907, 6.242252689847868297, -166.4062500020483810 ) ) ;
#34735=CARTESIAN_POINT ( 'NONE',  ( 10.81189881249999907, 6.242252689847868297, -86.71875000204836681 ) ) ;
#34737=CARTESIAN_POINT ( 'NONE',  ( 10.81189881249999551, -6.242252689847874514, -190.4687500020484094 ) ) ;
#34738=CARTESIAN_POINT ( 'NONE',  ( -10.81189881249999907, -6.242252689847864744, -95.15625000204839523 ) ) ;
#34743=CARTESIAN_POINT ( 'NONE',  ( 10.81189881249999551, -6.242252689847874514, -177.1562500020484094 ) ) ;
#34744=CARTESIAN_POINT ( 'NONE',  ( -5.405949406249996869, 9.363379034771805109, -190.0312500020484094 ) ) ;
#34746=CARTESIAN_POINT ( 'NONE',  ( 10.00000000000000000, 5.773502691896255534, -167.2500000040968189 ) ) ;
#34748=CARTESIAN_POINT ( 'NONE',  ( -10.81189881249999907, -6.242252689847864744, -15.46875000204836503 ) ) ;
#34750=CARTESIAN_POINT ( 'NONE',  ( 10.81189881249999729, 0.000000000000000000, -121.3437500020483952 ) ) ;
#34752=CARTESIAN_POINT ( 'NONE',  ( 5.405949406249992428, -9.363379034771808662, -18.28125000204835970 ) ) ;
#34755=CARTESIAN_POINT ( 'NONE',  ( 7.070501591499377789E-16, 11.54700538379251284, -49.62499999999997158 ) ) ;
#34756=CARTESIAN_POINT ( 'NONE',  ( -2.293366432827344421E-15, -12.48450537969573659, -118.9062500020483952 ) ) ;
#34758=VERTEX_POINT ( 'NONE', #41239 ) ;
#34759=CARTESIAN_POINT ( 'NONE',  ( -10.00000000000000000, -5.773502691896251982, -96.00000000409679046 ) ) ;
#34761=CARTESIAN_POINT ( 'NONE',  ( 7.644554776091147741E-16, 12.48450537969573659, -53.46875000204836681 ) ) ;
#34762=ORIENTED_EDGE ( 'NONE', *, *, #34409, .T. ) ;
#34768=CARTESIAN_POINT ( 'NONE',  ( 7.070501591499377789E-16, 11.54700538379251284, -20.00000000409676559 ) ) ;
#34772=LINE ( 'NONE', #1966, #34878 ) ;
#34773=ORIENTED_EDGE ( 'NONE', *, *, #21970, .F. ) ;
#34777=ORIENTED_EDGE ( 'NONE', *, *, #27718, .F. ) ;
#34778=ORIENTED_EDGE ( 'NONE', *, *, #15100, .T. ) ;
#34779=DIRECTION ( 'NONE',  ( -1.000000000000000000, 0.000000000000000000, 0.000000000000000000 ) ) ;
#34782=CARTESIAN_POINT ( 'NONE',  ( -10.81189881249999729, 1.324075727343319199E-15, -188.2812500020484094 ) ) ;
#34786=CARTESIAN_POINT ( 'NONE',  ( 10.81189881249999907, 6.242252689847868297, -110.7187500020483810 ) ) ;
#34788=CARTESIAN_POINT ( 'NONE',  ( -2.293366432827344421E-15, -12.48450537969573659, -115.9062500020483810 ) ) ;
#34790=CARTESIAN_POINT ( 'NONE',  ( -10.81189881249999729, 1.324075727343319199E-15, -119.0937500020483810 ) ) ;
#34791=EDGE_CURVE ( 'NONE', #24289, #15832, #13389, .T. ) ;
#34794=CARTESIAN_POINT ( 'NONE',  ( 9.999999999999996447, -5.773502691896262640, -144.6250000000000000 ) ) ;
#34795=CARTESIAN_POINT ( 'NONE',  ( 9.999999999999998224, 0.000000000000000000, -12.49999999999995559 ) ) ;
#34798=CARTESIAN_POINT ( 'NONE',  ( 9.999999999999996447, -5.773502691896262640, -190.0000000040968189 ) ) ;
#34800=CARTESIAN_POINT ( 'NONE',  ( -5.405949406250003975, -9.363379034771801557, -40.84375000204837391 ) ) ;
#34802=CARTESIAN_POINT ( 'NONE',  ( 10.81189881249999551, -6.242252689847874514, -143.9687500020483810 ) ) ;
#34804=CARTESIAN_POINT ( 'NONE',  ( 9.999999999999998224, 0.000000000000000000, -144.8750000040967905 ) ) ;
#34805=CARTESIAN_POINT ( 'NONE',  ( -5.000000000000003553, -8.660254037844383745, -74.49999999999998579 ) ) ;
#34806=CARTESIAN_POINT ( 'NONE',  ( 5.405949406249999534, 9.363379034771803333, -140.7812500020483810 ) ) ;
#34809=CARTESIAN_POINT ( 'NONE',  ( -10.81189881249999729, 6.242252689847871849, -101.4062500020483952 ) ) ;
#34810=CARTESIAN_POINT ( 'NONE',  ( -2.121150477449813534E-15, -11.54700538379251284, -113.7500000040967905 ) ) ;
#34812=CARTESIAN_POINT ( 'NONE',  ( -10.81189881249999729, 1.324075727343319199E-15, -72.59375000204838102 ) ) ;
#34815=CARTESIAN_POINT ( 'NONE',  ( -5.405949406249996869, 9.363379034771805109, -44.53125000204838102 ) ) ;
#34818=EDGE_CURVE ( 'NONE', #25640, #23180, #450, .T. ) ;
#34822=CARTESIAN_POINT ( 'NONE',  ( 9.999999999999866773, -5.773502691896336358, -173.5000000040967905 ) ) ;
#34823=VERTEX_POINT ( 'NONE', #22903 ) ;
#34833=CARTESIAN_POINT ( 'NONE',  ( 10.81189881249999729, 0.000000000000000000, -134.8437500020484094 ) ) ;
#34835=CARTESIAN_POINT ( 'NONE',  ( 10.81189881249999907, 6.242252689847868297, -143.9062500020484094 ) ) ;
#34836=CARTESIAN_POINT ( 'NONE',  ( -10.81189881249999729, -6.242252689847864744, -151.9687500020484094 ) ) ;
#34838=CARTESIAN_POINT ( 'NONE',  ( 9.999999999999998224, 0.000000000000000000, -173.0000000000000284 ) ) ;
#34842=CARTESIAN_POINT ( 'NONE',  ( -7.718883402056913923, -6.624744321260780389, -100.0000000000000284 ) ) ;
#34843=EDGE_CURVE ( 'NONE', #31374, #530, #35735, .T. ) ;
#34844=CARTESIAN_POINT ( 'NONE',  ( -5.405949406249996869, 9.363379034771805109, -173.3437500020484094 ) ) ;
#34847=DIRECTION ( 'NONE',  ( -0.000000000000000000, -0.000000000000000000, -1.000000000000000000 ) ) ;
#34848=CARTESIAN_POINT ( 'NONE',  ( -2.293366432827344421E-15, -12.48450537969573659, -46.90625000204837391 ) ) ;
#34850=CARTESIAN_POINT ( 'NONE',  ( 7.070501591499377789E-16, 11.54700538379251284, -96.12500000000000000 ) ) ;
#34853=CARTESIAN_POINT ( 'NONE',  ( -5.405949406249996869, 9.363379034771805109, -127.0312500020483952 ) ) ;
#34854=CARTESIAN_POINT ( 'NONE',  ( -2.121150477449813534E-15, -11.54700538379251284, -146.7500000040968189 ) ) ;
#34857=VERTEX_POINT ( 'NONE', #32413 ) ;
#34858=CARTESIAN_POINT ( 'NONE',  ( -10.81189881249999907, -6.242252689847864744, -171.4687500020484094 ) ) ;
#34862=CARTESIAN_POINT ( 'NONE',  ( 10.81189881249999907, 6.242252689847868297, -65.90625000204839523 ) ) ;
#34864=CARTESIAN_POINT ( 'NONE',  ( -9.999999999999998224, 1.224646799147353059E-15, -42.12500000409677625 ) ) ;
#34865=CARTESIAN_POINT ( 'NONE',  ( 7.644554776091147741E-16, 12.48450537969573659, -0.9687500020483519325 ) ) ;
#34878=VECTOR ( 'NONE', #18349, 1000.000000000000000 ) ;
#34879=VERTEX_POINT ( 'NONE', #38661 ) ;
#34886=CARTESIAN_POINT ( 'NONE',  ( 9.999999999999998224, 0.000000000000000000, -34.99999999999997868 ) ) ;
#34889=CARTESIAN_POINT ( 'NONE',  ( -2.293366432827344421E-15, -12.48450537969573659, -157.7187500020484094 ) ) ;
#34893=CARTESIAN_POINT ( 'NONE',  ( -5.000000000000003553, -8.660254037844383745, -191.5000000000000000 ) ) ;
#34900=CARTESIAN_POINT ( 'NONE',  ( -10.81189881249999729, 1.324075727343319199E-15, -68.28125000204838102 ) ) ;
#34902=CARTESIAN_POINT ( 'NONE',  ( 9.999999999999998224, 0.000000000000000000, -120.5000000000000000 ) ) ;
#34903=CARTESIAN_POINT ( 'NONE',  ( -2.293366432827344421E-15, -12.48450537969573659, -151.9062500020483810 ) ) ;
#34904=CARTESIAN_POINT ( 'NONE',  ( 5.405949406249992428, -9.363379034771808662, -163.7812500020484094 ) ) ;
#34907=CARTESIAN_POINT ( 'NONE',  ( -10.81189881249999729, 6.242252689847871849, -99.71875000204839523 ) ) ;
#34910=CARTESIAN_POINT ( 'NONE',  ( 5.405949406249999534, 9.363379034771803333, -199.0937500020484094 ) ) ;
#34914=CARTESIAN_POINT ( 'NONE',  ( 5.405949406249992428, -9.363379034771808662, -96.28125000204838102 ) ) ;
#34916=CARTESIAN_POINT ( 'NONE',  ( 9.999999999999996447, -5.773502691896262640, -71.50000000409676204 ) ) ;
#34918=CARTESIAN_POINT ( 'NONE',  ( 5.405949406249992428, -9.363379034771808662, -28.59375000204836326 ) ) ;
#34919=ORIENTED_EDGE ( 'NONE', *, *, #39416, .T. ) ;
#34921=CARTESIAN_POINT ( 'NONE',  ( -10.81189881249999729, 1.324075727343319199E-15, -18.78125000204835970 ) ) ;
#34924=EDGE_CURVE ( 'NONE', #34758, #15268, #9257, .T. ) ;
#34933=EDGE_CURVE ( 'NONE', #18938, #28436, #40120, .T. ) ;
#34940=CARTESIAN_POINT ( 'NONE',  ( 8.145196138936681152, 6.643413332909280378, -99.99999999999997158 ) ) ;
#34942=CARTESIAN_POINT ( 'NONE',  ( -2.293366432827344421E-15, -12.48450537969573659, -163.9062500020483810 ) ) ;
#34947=CARTESIAN_POINT ( 'NONE',  ( 7.644554776091147741E-16, 12.48450537969573659, -83.46875000204838102 ) ) ;
#34949=CARTESIAN_POINT ( 'NONE',  ( 10.81189881249999729, 0.000000000000000000, -193.3437500020484094 ) ) ;
#34950=CARTESIAN_POINT ( 'NONE',  ( -2.293366432827344421E-15, -12.48450537969573659, -93.40625000204839523 ) ) ;
#34953=ADVANCED_FACE ( 'NONE', ( #875 ), #30230, .F. ) ;
#34954=CARTESIAN_POINT ( 'NONE',  ( -9.999999999999998224, 1.224646799147353059E-15, -151.2500000000000000 ) ) ;
#34955=CARTESIAN_POINT ( 'NONE',  ( 10.81189881249999729, 6.242252689847867408, -176.9062500020484094 ) ) ;
#34956=CARTESIAN_POINT ( 'NONE',  ( 5.405949406249992428, -9.363379034771808662, -184.7812500020484094 ) ) ;
#34959=CARTESIAN_POINT ( 'NONE',  ( -9.999999999999998224, 5.773502691896259087, -160.7500000040967620 ) ) ;
#34961=CARTESIAN_POINT ( 'NONE',  ( 10.81189881249999907, 6.242252689847868297, -13.21875000204836148 ) ) ;
#34963=CARTESIAN_POINT ( 'NONE',  ( 10.81189881249999907, 6.242252689847868297, -119.7187500020483810 ) ) ;
#34965=CARTESIAN_POINT ( 'NONE',  ( 5.405949406249999534, 9.363379034771803333, -20.78125000204836326 ) ) ;
#34968=CARTESIAN_POINT ( 'NONE',  ( 7.070501591499377789E-16, 11.54700538379251284, -51.12499999999997868 ) ) ;
#34969=CARTESIAN_POINT ( 'NONE',  ( -10.81189881249999729, 6.242252689847871849, -117.9062500020483952 ) ) ;
#34972=CARTESIAN_POINT ( 'NONE',  ( 5.000000000000000000, 8.660254037844385522, -90.62500000409677625 ) ) ;
#34975=CARTESIAN_POINT ( 'NONE',  ( 5.405949406249992428, -9.363379034771808662, -54.09375000204835970 ) ) ;
#34980=CARTESIAN_POINT ( 'NONE',  ( -9.999999999999998224, 5.773502691896259087, -16.75000000409676559 ) ) ;
#34981=ADVANCED_FACE ( 'NONE', ( #23322 ), #13575, .F. ) ;
#34986=ORIENTED_EDGE ( 'NONE', *, *, #10314, .T. ) ;
#34992=ORIENTED_EDGE ( 'NONE', *, *, #28859, .F. ) ;
#34996=CARTESIAN_POINT ( 'NONE',  ( -5.405949406250003975, -9.363379034771801557, -186.5312500020484094 ) ) ;
#34999=CARTESIAN_POINT ( 'NONE',  ( -10.81189881249999729, 1.324075727343319199E-15, -107.0937500020483810 ) ) ;
#35001=CARTESIAN_POINT ( 'NONE',  ( 5.405949406249992428, -9.363379034771808662, -115.7812500020483952 ) ) ;
#35003=CARTESIAN_POINT ( 'NONE',  ( -10.81189881249999729, 1.324075727343319199E-15, -125.0937500020483668 ) ) ;
#35005=DIRECTION ( 'NONE',  ( -0.000000000000000000, -0.000000000000000000, -1.000000000000000000 ) ) ;
#35006=CARTESIAN_POINT ( 'NONE',  ( -10.00000000000000000, -5.773502691896251982, -148.1249999999999716 ) ) ;
#35007=CARTESIAN_POINT ( 'NONE',  ( -2.121150477449813534E-15, -11.54700538379251284, -15.87499999999997335 ) ) ;
#35010=CARTESIAN_POINT ( 'NONE',  ( -10.00000000000000000, -5.773502691896251982, -189.0000000040967905 ) ) ;
#35013=CARTESIAN_POINT ( 'NONE',  ( 5.405949406249999534, 9.363379034771803333, -41.59375000204837391 ) ) ;
#35015=CARTESIAN_POINT ( 'NONE',  ( -5.405949406250003975, -9.363379034771801557, -142.8437500020483810 ) ) ;
#35018=CARTESIAN_POINT ( 'NONE',  ( -4.999999999999996447, 8.660254037844387298, -73.49999999999998579 ) ) ;
#35019=CARTESIAN_POINT ( 'NONE',  ( 5.405949406249992428, -9.363379034771808662, -144.2812500020483810 ) ) ;
#35022=CARTESIAN_POINT ( 'NONE',  ( -9.999999999999998224, 5.773502691896259087, -117.2500000040967763 ) ) ;
#35024=CARTESIAN_POINT ( 'NONE',  ( -10.81189881249999907, -6.242252689847864744, -72.46875000204835260 ) ) ;
#35026=ADVANCED_FACE ( 'NONE', ( #27188 ), #40332, .F. ) ;
#35029=CARTESIAN_POINT ( 'NONE',  ( 10.81189881249999729, 0.000000000000000000, -45.03125000204838102 ) ) ;
#35038=AXIS2_PLACEMENT_3D ( 'NONE', #26431, #23632, #19520 ) ;
#35039=ORIENTED_EDGE ( 'NONE', *, *, #17227, .F. ) ;
#35047=CARTESIAN_POINT ( 'NONE',  ( -10.81189881249999729, 1.324075727343319199E-15, -135.5937500020483810 ) ) ;
#35048=CARTESIAN_POINT ( 'NONE',  ( 10.81189881249999729, 0.000000000000000000, -144.0312500020483810 ) ) ;
#35049=CARTESIAN_POINT ( 'NONE',  ( -10.81189881249999729, 1.324075727343319199E-15, -143.0937500020483810 ) ) ;
#35052=CARTESIAN_POINT ( 'NONE',  ( 7.070501591499377789E-16, 11.54700538379251284, -174.1250000000000000 ) ) ;
#35056=CARTESIAN_POINT ( 'NONE',  ( -5.378272834344112852, -8.460370942358581559, -99.99999999999998579 ) ) ;
#35057=CARTESIAN_POINT ( 'NONE',  ( 5.405949406249999534, 9.363379034771803333, -169.0937500020484094 ) ) ;
#35061=CARTESIAN_POINT ( 'NONE',  ( -10.81189881249999907, -6.242252689847864744, -44.15625000204837391 ) ) ;
#35063=CARTESIAN_POINT ( 'NONE',  ( 9.999999999999998224, 0.000000000000000000, -99.49999999999998579 ) ) ;
#35066=CARTESIAN_POINT ( 'NONE',  ( -10.81189881249999729, 1.324075727343319199E-15, -128.2812500020483810 ) ) ;
#35067=CARTESIAN_POINT ( 'NONE',  ( -10.00000000000000000, -5.773502691896251982, -136.5000000040967905 ) ) ;
#35072=AXIS2_PLACEMENT_3D ( 'NONE', #12617, #13455, #39173 ) ;
#35073=( BOUNDED_CURVE ( )  B_SPLINE_CURVE ( 2, ( #39014, #22833, #12877, #16537, #35996, #29519, #3402 ),
 .UNSPECIFIED., .F., .F. ) 
 B_SPLINE_CURVE_WITH_KNOTS ( ( 3, 2, 2, 3 ),
 ( 0.3880597014925373789, 0.3893034825870647087, 0.3905472636815920939, 0.3917910447761194792 ),
 .UNSPECIFIED. ) 
 CURVE ( )  GEOMETRIC_REPRESENTATION_ITEM ( )  RATIONAL_B_SPLINE_CURVE ( ( 0.9999999999999940048, 0.8660254037844447028, 1.000000000000000000, 0.8660254037844387076, 1.000000000000000000, 0.8660254037844327124, 1.000000000000005995 ) ) 
 REPRESENTATION_ITEM ( '' )  );
#35074=CARTESIAN_POINT ( 'NONE',  ( -9.999999999999612754, -5.773502691896474914, -155.6249999999999716 ) ) ;
#35075=CARTESIAN_POINT ( 'NONE',  ( -10.81189881249999729, 1.324075727343319199E-15, -65.28125000204838102 ) ) ;
#35078=CARTESIAN_POINT ( 'NONE',  ( 9.999999999999998224, 0.000000000000000000, -162.5000000000000000 ) ) ;
#35080=EDGE_CURVE ( 'NONE', #1591, #36081, #4103, .T. ) ;
#35081=ORIENTED_EDGE ( 'NONE', *, *, #11491, .F. ) ;
#35086=ORIENTED_EDGE ( 'NONE', *, *, #30941, .F. ) ;
#35087=CARTESIAN_POINT ( 'NONE',  ( -2.121150477449813534E-15, -11.54700538379251284, -178.2500000040968189 ) ) ;
#35091=FACE_OUTER_BOUND ( 'NONE', #5538, .T. ) ;
#35096=CARTESIAN_POINT ( 'NONE',  ( 5.000000000000000000, 8.660254037844385522, -36.24999999999997868 ) ) ;
#35097=AXIS2_PLACEMENT_3D ( 'NONE', #27077, #8080, #40220 ) ;
#35100=CARTESIAN_POINT ( 'NONE',  ( 10.81189881249999729, 0.000000000000000000, -157.3437500020483810 ) ) ;
#35101=CARTESIAN_POINT ( 'NONE',  ( 7.644554776091147741E-16, 12.48450537969573659, -171.9687500020483810 ) ) ;
#35102=CARTESIAN_POINT ( 'NONE',  ( 9.999999999999998224, 0.000000000000000000, -129.5000000000000000 ) ) ;
#35104=CARTESIAN_POINT ( 'NONE',  ( -5.000000000000003553, -8.660254037844383745, -194.5000000000000000 ) ) ;
#35105=AXIS2_PLACEMENT_3D ( 'NONE', #34253, #1875, #8558 ) ;
#35110=CARTESIAN_POINT ( 'NONE',  ( 7.644554776091147741E-16, 12.48450537969573659, -70.15625000204839523 ) ) ;
#35112=CARTESIAN_POINT ( 'NONE',  ( -9.999999999999998224, 1.224646799147353059E-15, -125.7499999999999716 ) ) ;
#35113=( BOUNDED_CURVE ( )  B_SPLINE_CURVE ( 2, ( #17386, #21062, #1229 ),
 .UNSPECIFIED., .F., .F. ) 
 B_SPLINE_CURVE_WITH_KNOTS ( ( 3, 3 ),
 ( 0.4962686567164180107, 0.4975124378109453960 ),
 .UNSPECIFIED. ) 
 CURVE ( )  GEOMETRIC_REPRESENTATION_ITEM ( )  RATIONAL_B_SPLINE_CURVE ( ( 0.9999999999999880096, 0.8660254037844387076, 1.000000000000011990 ) ) 
 REPRESENTATION_ITEM ( '' )  );
#35114=EDGE_LOOP ( 'NONE', ( #765, #11259, #36239, #4537 ) ) ;
#35115=CARTESIAN_POINT ( 'NONE',  ( -5.405949406249996869, 9.363379034771805109, -148.0312500020483810 ) ) ;
#35116=CARTESIAN_POINT ( 'NONE',  ( 7.644554776091147741E-16, 12.48450537969573659, -161.6562500020484379 ) ) ;
#35119=CARTESIAN_POINT ( 'NONE',  ( -10.81189881249999729, 1.324075727343319199E-15, -95.09375000204838102 ) ) ;
#35122=CARTESIAN_POINT ( 'NONE',  ( 5.405949406249999534, 9.363379034771803333, -194.5937500020484094 ) ) ;
#35124=CARTESIAN_POINT ( 'NONE',  ( 8.340417757194298787, -6.866608375281687771, -180.0000000000000284 ) ) ;
#35125=CARTESIAN_POINT ( 'NONE',  ( -9.999999999999998224, 1.224646799147353059E-15, -145.2500000000000000 ) ) ;
#35126=CARTESIAN_POINT ( 'NONE',  ( 7.644554776091147741E-16, 12.48450537969573659, -94.15625000204839523 ) ) ;
#35129=CARTESIAN_POINT ( 'NONE',  ( -2.121150477449813534E-15, -11.54700538379251284, -67.25000000409679046 ) ) ;
#35130=DIRECTION ( 'NONE',  ( -0.000000000000000000, -0.000000000000000000, -1.000000000000000000 ) ) ;
#35131=CARTESIAN_POINT ( 'NONE',  ( -2.293366432827344421E-15, -12.48450537969573659, -28.71875000204834905 ) ) ;
#35134=CARTESIAN_POINT ( 'NONE',  ( 5.405949406249992428, -9.363379034771808662, -22.78125000204836326 ) ) ;
#35136=CARTESIAN_POINT ( 'NONE',  ( 9.999999999999998224, 0.000000000000000000, -132.5000000000000000 ) ) ;
#35137=CARTESIAN_POINT ( 'NONE',  ( 5.000000000000000000, 8.660254037844385522, 0.8749999959032361829 ) ) ;
#35142=CARTESIAN_POINT ( 'NONE',  ( 5.000000000000000000, 8.660254037844385522, -170.1250000040968189 ) ) ;
#35153=CARTESIAN_POINT ( 'NONE',  ( -10.81189881249999729, 6.242252689847871849, -161.4062500020483810 ) ) ;
#35155=CARTESIAN_POINT ( 'NONE',  ( -10.00000000000000000, -5.773502691896252870, -172.5000000040967905 ) ) ;
#35158=CARTESIAN_POINT ( 'NONE',  ( -10.81189881249999729, 1.324075727343319199E-15, -83.09375000204836681 ) ) ;
#35159=CARTESIAN_POINT ( 'NONE',  ( 10.81189881249999551, -6.242252689847874514, -191.9687500020484379 ) ) ;
#35160=CARTESIAN_POINT ( 'NONE',  ( -5.405949406249996869, 9.363379034771805109, -89.53125000204838102 ) ) ;
#35164=CARTESIAN_POINT ( 'NONE',  ( -2.293366432827344421E-15, -12.48450537969573659, -172.9062500020484379 ) ) ;
#35165=CARTESIAN_POINT ( 'NONE',  ( -10.81189881249999729, 1.324075727343319199E-15, -188.2812500020484094 ) ) ;
#35168=CARTESIAN_POINT ( 'NONE',  ( 9.999999999999996447, -5.773502691896262640, -163.0000000040967905 ) ) ;
#35170=CARTESIAN_POINT ( 'NONE',  ( -10.81189881249999729, 1.324075727343319199E-15, -17.09375000204835260 ) ) ;
#35172=CARTESIAN_POINT ( 'NONE',  ( -2.293366432827344421E-15, -12.48450537969573659, -124.7187500020483668 ) ) ;
#35174=CARTESIAN_POINT ( 'NONE',  ( -5.405949406249996869, 9.363379034771805109, -19.03125000204835970 ) ) ;
#35177=CARTESIAN_POINT ( 'NONE',  ( -5.405949406249996869, 9.363379034771805109, -113.5312500020483952 ) ) ;
#35180=CARTESIAN_POINT ( 'NONE',  ( 9.999999999999996447, -5.773502691896262640, -89.50000000409676204 ) ) ;
#35182=CARTESIAN_POINT ( 'NONE',  ( 10.81189881249999907, 6.242252689847868297, -53.71875000204837391 ) ) ;
#35187=CARTESIAN_POINT ( 'NONE',  ( -2.121150477449813534E-15, -11.54700538379251284, -19.25000000409676559 ) ) ;
#35190=VERTEX_POINT ( 'NONE', #13788 ) ;
#35205=CARTESIAN_POINT ( 'NONE',  ( -5.405949406249996869, 9.363379034771805109, -190.0312500020484094 ) ) ;
#35210=CARTESIAN_POINT ( 'NONE',  ( -2.293366432827344421E-15, -12.48450537969573659, -108.2187500020483668 ) ) ;
#35211=CARTESIAN_POINT ( 'NONE',  ( -2.121150477449813534E-15, -11.54700538379251284, -149.7500000040968189 ) ) ;
#35212=CARTESIAN_POINT ( 'NONE',  ( -10.81189881249999729, 6.242252689847871849, -117.9062500020483952 ) ) ;
#35214=CARTESIAN_POINT ( 'NONE',  ( -5.405949406250003975, -9.363379034771801557, -124.8437500020483810 ) ) ;
#35217=CARTESIAN_POINT ( 'NONE',  ( -10.00000000000000000, -5.773502691896251982, -143.6250000000000000 ) ) ;
#35218=CARTESIAN_POINT ( 'NONE',  ( -9.999999999999998224, 1.224646799147353059E-15, -16.24999999999995737 ) ) ;
#35222=CARTESIAN_POINT ( 'NONE',  ( 5.000000000000000000, 8.660254037844385522, -188.1250000040967905 ) ) ;
#35224=CARTESIAN_POINT ( 'NONE',  ( -5.405949406250003975, -9.363379034771801557, -36.34375000204836681 ) ) ;
#35225=CARTESIAN_POINT ( 'NONE',  ( -9.999999999999998224, 1.224646799147353059E-15, -163.6250000040967905 ) ) ;
#35226=CARTESIAN_POINT ( 'NONE',  ( -10.81189881249999907, -6.242252689847864744, -148.9687500020484094 ) ) ;
#35228=CARTESIAN_POINT ( 'NONE',  ( -2.121150477449813534E-15, -11.54700538379251284, -101.7500000040967763 ) ) ;
#35229=CARTESIAN_POINT ( 'NONE',  ( 5.000000000000000000, 8.660254037844385522, -78.24999999999998579 ) ) ;
#35230=CARTESIAN_POINT ( 'NONE',  ( -5.405949406250003975, -9.363379034771801557, -137.0312500020484094 ) ) ;
#35234=CARTESIAN_POINT ( 'NONE',  ( -9.999999999999998224, 5.773502691896259087, -114.2500000040967905 ) ) ;
#35236=CARTESIAN_POINT ( 'NONE',  ( -2.293366432827344421E-15, -12.48450537969573659, -73.71875000204835260 ) ) ;
#35242=CARTESIAN_POINT ( 'NONE',  ( -5.405949406249996869, 9.363379034771805109, -40.03125000204838102 ) ) ;
#35248=CARTESIAN_POINT ( 'NONE',  ( -2.121150477449813534E-15, -11.54700538379251284, -173.7500000040968189 ) ) ;
#35261=CARTESIAN_POINT ( 'NONE',  ( 5.405949406249992428, -9.363379034771808662, -133.5937500020483810 ) ) ;
#35262=CARTESIAN_POINT ( 'NONE',  ( 5.405949406249999534, 9.363379034771803333, -140.7812500020483810 ) ) ;
#35264=CARTESIAN_POINT ( 'NONE',  ( 7.644554776091147741E-16, 12.48450537969573659, -146.4687500020484094 ) ) ;
#35265=CARTESIAN_POINT ( 'NONE',  ( 9.999999999999998224, 0.000000000000000000, -128.0000000000000000 ) ) ;
#35267=CARTESIAN_POINT ( 'NONE',  ( 5.000000000000000000, 8.660254037844385522, -174.2500000000000284 ) ) ;
#35272=CARTESIAN_POINT ( 'NONE',  ( -10.44810905595974759, 0.3217275869905217300, -99.99999999999998579 ) ) ;
#35273=CARTESIAN_POINT ( 'NONE',  ( -2.293366432827344421E-15, -12.48450537969573659, -172.7187500020484094 ) ) ;
#35277=CARTESIAN_POINT ( 'NONE',  ( -5.405949406250003975, -9.363379034771801557, -33.53125000204837391 ) ) ;
#35279=CARTESIAN_POINT ( 'NONE',  ( 9.999999999999996447, -5.773502691896262640, -98.12499999999998579 ) ) ;
#35281=CARTESIAN_POINT ( 'NONE',  ( 5.405949406249999534, 9.363379034771803333, -115.2812500020483952 ) ) ;
#35282=CARTESIAN_POINT ( 'NONE',  ( -10.00000000000000000, -5.773502691896251982, -139.5000000040967905 ) ) ;
#35287=CARTESIAN_POINT ( 'NONE',  ( -5.405949406249996869, 9.363379034771805109, -56.53125000204836681 ) ) ;
#35292=CARTESIAN_POINT ( 'NONE',  ( -2.121150477449813534E-15, -11.54700538379251284, -106.2500000040967905 ) ) ;
#35295=DIRECTION ( 'NONE',  ( -0.000000000000000000, -0.000000000000000000, -1.000000000000000000 ) ) ;
#35300=VERTEX_POINT ( 'NONE', #27619 ) ;
#35301=CARTESIAN_POINT ( 'NONE',  ( -5.000000000000003553, -8.660254037844383745, -100.3750000040967905 ) ) ;
#35308=ORIENTED_EDGE ( 'NONE', *, *, #38704, .F. ) ;
#35309=CARTESIAN_POINT ( 'NONE',  ( -5.000000000000003553, -8.660254037844383745, -112.3750000040967763 ) ) ;
#35310=CARTESIAN_POINT ( 'NONE',  ( -9.999999999999998224, 1.224646799147353059E-15, -37.24999999999997868 ) ) ;
#35313=CARTESIAN_POINT ( 'NONE',  ( 7.644554776091147741E-16, 12.48450537969573659, -156.9687500020484094 ) ) ;
#35315=CARTESIAN_POINT ( 'NONE',  ( -5.405949406249996869, 9.363379034771805109, -173.3437500020484094 ) ) ;
#35317=CARTESIAN_POINT ( 'NONE',  ( -4.999999999999996447, 8.660254037844387298, -132.0000000000000000 ) ) ;
#35318=CARTESIAN_POINT ( 'NONE',  ( -9.999999999999998224, 5.773502691896259087, -193.3750000000000000 ) ) ;
#35323=( BOUNDED_CURVE ( )  B_SPLINE_CURVE ( 2, ( #7111, #36669, #12920, #13134, #35836, #16157, #3447 ),
 .UNSPECIFIED., .F., .F. ) 
 B_SPLINE_CURVE_WITH_KNOTS ( ( 3, 2, 2, 3 ),
 ( 0.2574626865671643117, 0.2587064676616916414, 0.2599502487562190267, 0.2611940298507463565 ),
 .UNSPECIFIED. ) 
 CURVE ( )  GEOMETRIC_REPRESENTATION_ITEM ( )  RATIONAL_B_SPLINE_CURVE ( ( 0.9999999999999880096, 0.8660254037844506980, 1.000000000000000000, 0.8660254037844387076, 1.000000000000000000, 0.8660254037844267172, 1.000000000000011990 ) ) 
 REPRESENTATION_ITEM ( '' )  );
#35324=CARTESIAN_POINT ( 'NONE',  ( -2.293366432827344421E-15, -12.48450537969573659, -60.40625000204838813 ) ) ;
#35326=CARTESIAN_POINT ( 'NONE',  ( -10.00000000000000000, -5.773502691896251982, -124.1250000000000000 ) ) ;
#35329=CARTESIAN_POINT ( 'NONE',  ( -5.405949406249996869, 9.363379034771805109, -139.0312500020484094 ) ) ;
#35330=CARTESIAN_POINT ( 'NONE',  ( -5.405949406249996869, 9.363379034771805109, -160.0312500020484094 ) ) ;
#35332=CARTESIAN_POINT ( 'NONE',  ( 7.070501591499376803E-16, 11.54700538379251284, -105.1249999999999858 ) ) ;
#35333=CARTESIAN_POINT ( 'NONE',  ( 7.644554776091147741E-16, 12.48450537969573659, -86.46875000204838102 ) ) ;
#35336=CARTESIAN_POINT ( 'NONE',  ( -5.405949406250003975, -9.363379034771801557, -0.5312500020483723606 ) ) ;
#35338=CARTESIAN_POINT ( 'NONE',  ( -2.121150477449813534E-15, -11.54700538379251284, -117.8749999999999858 ) ) ;
#35339=CARTESIAN_POINT ( 'NONE',  ( -10.81189881249999907, -6.242252689847864744, -95.15625000204839523 ) ) ;
#35341=CARTESIAN_POINT ( 'NONE',  ( 5.000000000000000000, 8.660254037844385522, -71.12500000409677625 ) ) ;
#35343=CARTESIAN_POINT ( 'NONE',  ( -2.293366432827344421E-15, -12.48450537969573659, -22.71875000204837391 ) ) ;
#35344=CARTESIAN_POINT ( 'NONE',  ( -10.00000000000051337, 5.773502691895962435, -100.3750000000000000 ) ) ;
#35346=CARTESIAN_POINT ( 'NONE',  ( -10.81189881249999729, 6.242252689847871849, -21.90625000204837391 ) ) ;
#35355=CARTESIAN_POINT ( 'NONE',  ( -4.999999999999996447, 8.660254037844387298, -115.8750000040967905 ) ) ;
#35356=ORIENTED_EDGE ( 'NONE', *, *, #29665, .F. ) ;
#35367=CARTESIAN_POINT ( 'NONE',  ( 5.405949406249992428, -9.363379034771808662, -159.2812500020484094 ) ) ;
#35372=CARTESIAN_POINT ( 'NONE',  ( -10.81189881249999907, -6.242252689847864744, -81.46875000204838102 ) ) ;
#35373=CARTESIAN_POINT ( 'NONE',  ( -10.81189881249999729, 6.242252689847871849, -92.40625000204838102 ) ) ;
#35376=( BOUNDED_CURVE ( )  B_SPLINE_CURVE ( 2, ( #3218, #3647, #3425, #23277, #42685, #16563, #3855 ),
 .UNSPECIFIED., .F., .F. ) 
 B_SPLINE_CURVE_WITH_KNOTS ( ( 3, 2, 2, 3 ),
 ( 0.2873134328358210032, 0.2885572139303483885, 0.2898009950248757183, 0.2910447761194031036 ),
 .UNSPECIFIED. ) 
 CURVE ( )  GEOMETRIC_REPRESENTATION_ITEM ( )  RATIONAL_B_SPLINE_CURVE ( ( 0.9999999999999880096, 0.8660254037844506980, 1.000000000000000000, 0.8660254037844387076, 1.000000000000000000, 0.8660254037844267172, 1.000000000000011990 ) ) 
 REPRESENTATION_ITEM ( '' )  );
#35378=CARTESIAN_POINT ( 'NONE',  ( 10.81189881249999729, 6.242252689847867408, -172.4062500020484094 ) ) ;
#35379=CARTESIAN_POINT ( 'NONE',  ( -5.405949406250003975, -9.363379034771801557, -189.5312500020484094 ) ) ;
#35381=CARTESIAN_POINT ( 'NONE',  ( -9.999999999999998224, 1.224646799147353059E-15, -168.1250000040967905 ) ) ;
#35383=CARTESIAN_POINT ( 'NONE',  ( -2.293366432827344421E-15, -12.48450537969573659, -10.71875000204836148 ) ) ;
#35385=CARTESIAN_POINT ( 'NONE',  ( 5.405949406249992428, -9.363379034771808662, -118.5937500020483810 ) ) ;
#35388=CARTESIAN_POINT ( 'NONE',  ( 10.81189881249999551, -6.242252689847874514, -16.65625000204837391 ) ) ;
#35391=CARTESIAN_POINT ( 'NONE',  ( -10.81189881249999729, 1.324075727343319199E-15, -116.2812500020483952 ) ) ;
#35394=CARTESIAN_POINT ( 'NONE',  ( 4.999999999999992006, -8.660254037844389075, -92.62500000409677625 ) ) ;
#35397=CARTESIAN_POINT ( 'NONE',  ( 10.81189881249999907, 6.242252689847868297, -52.21875000204837391 ) ) ;
#35398=VERTEX_POINT ( 'NONE', #40968 ) ;
#35402=CARTESIAN_POINT ( 'NONE',  ( 10.00000000000000000, 5.773502691896255534, -21.75000000409676915 ) ) ;
#35405=ORIENTED_EDGE ( 'NONE', *, *, #27279, .F. ) ;
#35406=CARTESIAN_POINT ( 'NONE',  ( 9.999999999999998224, 0.000000000000000000, -152.0000000000000000 ) ) ;
#35407=VERTEX_POINT ( 'NONE', #37973 ) ;
#35416=CARTESIAN_POINT ( 'NONE',  ( 10.81189881249999729, 0.000000000000000000, -177.0312500020483810 ) ) ;
#35420=CARTESIAN_POINT ( 'NONE',  ( 10.81189881249999551, -6.242252689847874514, -107.9687500020483810 ) ) ;
#35422=CARTESIAN_POINT ( 'NONE',  ( 7.644554776091147741E-16, 12.48450537969573659, -113.6562500020483952 ) ) ;
#35424=CARTESIAN_POINT ( 'NONE',  ( -5.405949406249996869, 9.363379034771805109, -120.8437500020483952 ) ) ;
#35426=CARTESIAN_POINT ( 'NONE',  ( 7.070501591499376803E-16, 11.54700538379251284, -157.6250000000000284 ) ) ;
#35427=CARTESIAN_POINT ( 'NONE',  ( -5.000000000000003553, -8.660254037844383745, -137.5000000000000000 ) ) ;
#35428=CARTESIAN_POINT ( 'NONE',  ( 4.999999999999992006, -8.660254037844389075, -11.24999999999995381 ) ) ;
#35431=CARTESIAN_POINT ( 'NONE',  ( 4.999999999999992006, -8.660254037844389075, -187.1250000040967905 ) ) ;
#35433=CARTESIAN_POINT ( 'NONE',  ( 10.81189881249999551, -6.242252689847874514, -38.96875000204835970 ) ) ;
#35435=CARTESIAN_POINT ( 'NONE',  ( 5.405949406249992428, -9.363379034771808662, -150.0937500020483810 ) ) ;
#35436=ADVANCED_FACE ( 'NONE', ( #28054 ), #5385, .F. ) ;
#35440=CARTESIAN_POINT ( 'NONE',  ( 9.999999999999998224, 0.000000000000000000, -64.99999999999997158 ) ) ;
#35441=CARTESIAN_POINT ( 'NONE',  ( -10.81189881249999729, 1.324075727343319199E-15, -138.7812500020483810 ) ) ;
#35446=CARTESIAN_POINT ( 'NONE',  ( -9.999999999999998224, 1.224646799147353059E-15, -115.6250000040967905 ) ) ;
#35448=CARTESIAN_POINT ( 'NONE',  ( 7.644554776091147741E-16, 12.48450537969573659, -74.46875000204838102 ) ) ;
#35453=CARTESIAN_POINT ( 'NONE',  ( 7.070501591499376803E-16, 11.54700538379251284, -119.0000000040967763 ) ) ;
#35455=CARTESIAN_POINT ( 'NONE',  ( -10.81189881249999729, 6.242252689847871849, -38.40625000204835970 ) ) ;
#35459=CARTESIAN_POINT ( 'NONE',  ( 10.00000000000012257, -5.773502691896187144, -164.5000000040967905 ) ) ;
#35461=ORIENTED_EDGE ( 'NONE', *, *, #11998, .F. ) ;
#35462=EDGE_CURVE ( 'NONE', #24467, #27698, #25282, .T. ) ;
#35472=CARTESIAN_POINT ( 'NONE',  ( -9.999999999999998224, 1.224646799147353059E-15, -147.1250000040967905 ) ) ;
#35473=CARTESIAN_POINT ( 'NONE',  ( -5.405949406250003975, -9.363379034771801557, -133.8437500020484094 ) ) ;
#35474=CARTESIAN_POINT ( 'NONE',  ( -5.405949406250003975, -9.363379034771801557, -144.5312500020483810 ) ) ;
#35476=CARTESIAN_POINT ( 'NONE',  ( -10.81189881249999729, 1.324075727343319199E-15, -147.5937500020483810 ) ) ;
#35479=CARTESIAN_POINT ( 'NONE',  ( 5.000000000000000000, 8.660254037844385522, -162.2500000000000000 ) ) ;
#35481=CARTESIAN_POINT ( 'NONE',  ( 4.999999999999992006, -8.660254037844389075, -114.7499999999999858 ) ) ;
#35483=CARTESIAN_POINT ( 'NONE',  ( 10.81189881249999907, 6.242252689847868297, -64.21875000204838102 ) ) ;
#35485=CARTESIAN_POINT ( 'NONE',  ( -10.81189881249999729, 1.324075727343319199E-15, -171.5937500020484094 ) ) ;
#35489=CARTESIAN_POINT ( 'NONE',  ( 5.405949406249992428, -9.363379034771808662, -37.78125000204838102 ) ) ;
#35491=CARTESIAN_POINT ( 'NONE',  ( 9.999999999999996447, -5.773502691896262640, -96.62500000000000000 ) ) ;
#35493=EDGE_CURVE ( 'NONE', #7848, #33176, #32702, .T. ) ;
#35495=CARTESIAN_POINT ( 'NONE',  ( -2.293366432827344421E-15, -12.48450537969573659, -115.9062500020483952 ) ) ;
#35496=CARTESIAN_POINT ( 'NONE',  ( 7.070501591499377789E-16, 11.54700538379251284, -137.0000000040967905 ) ) ;
#35497=CARTESIAN_POINT ( 'NONE',  ( -10.00000000000012434, 5.773502691896184480, -158.8750000000000000 ) ) ;
#35501=CARTESIAN_POINT ( 'NONE',  ( 7.644554776091147741E-16, 12.48450537969573659, -59.65625000204838102 ) ) ;
#35503=CARTESIAN_POINT ( 'NONE',  ( 9.999999999999479527, 5.773502691896553074, -147.7500000040967620 ) ) ;
#35505=CARTESIAN_POINT ( 'NONE',  ( -2.121150477449813534E-15, -11.54700538379251284, -162.8750000000000000 ) ) ;
#35507=ORIENTED_EDGE ( 'NONE', *, *, #22283, .T. ) ;
#35512=EDGE_LOOP ( 'NONE', ( #42067, #11322, #40940, #27966 ) ) ;
#35515=VERTEX_POINT ( 'NONE', #25873 ) ;
#35523=CARTESIAN_POINT ( 'NONE',  ( 9.999999999999998224, 0.000000000000000000, -30.49999999999997158 ) ) ;
#35526=CARTESIAN_POINT ( 'NONE',  ( 5.405949406249992428, -9.363379034771808662, -154.5937500020483810 ) ) ;
#35527=CARTESIAN_POINT ( 'NONE',  ( 5.405949406249999534, 9.363379034771803333, -167.5937500020484094 ) ) ;
#35529=CYLINDRICAL_SURFACE ( 'NONE', #30894, 9.999999999999998224 ) ;
#35530=CARTESIAN_POINT ( 'NONE',  ( -2.121150477449813534E-15, -11.54700538379251284, -192.8750000000000284 ) ) ;
#35535=CARTESIAN_POINT ( 'NONE',  ( -10.81189881249999729, 6.242252689847871849, -60.90625000204837391 ) ) ;
#35537=CARTESIAN_POINT ( 'NONE',  ( 10.00000000000000000, 5.773502691896255534, -121.8750000000000000 ) ) ;
#35539=CARTESIAN_POINT ( 'NONE',  ( -5.405949406249996869, 9.363379034771805109, -143.5312500020483810 ) ) ;
#35540=CARTESIAN_POINT ( 'NONE',  ( -2.293366432827344421E-15, -12.48450537969573659, -157.9062500020483810 ) ) ;
#35543=CARTESIAN_POINT ( 'NONE',  ( -10.81189881249999729, 6.242252689847871849, -93.71875000204838102 ) ) ;
#35546=CARTESIAN_POINT ( 'NONE',  ( 5.405949406249999534, 9.363379034771803333, -187.0937500020483810 ) ) ;
#35549=CARTESIAN_POINT ( 'NONE',  ( 10.00000000000051159, -5.773502691895965988, -123.6250000000000142 ) ) ;
#35550=CARTESIAN_POINT ( 'NONE',  ( 10.81189881249999729, 0.000000000000000000, -87.03125000204838102 ) ) ;
#35553=CARTESIAN_POINT ( 'NONE',  ( 10.00000000000000000, 5.773502691896255534, -56.25000000409676915 ) ) ;
#35555=CARTESIAN_POINT ( 'NONE',  ( 5.405949406249992428, -9.363379034771808662, -15.09375000204835082 ) ) ;
#35556=ORIENTED_EDGE ( 'NONE', *, *, #24377, .F. ) ;
#35559=CARTESIAN_POINT ( 'NONE',  ( 10.81189881249999729, 0.000000000000000000, -18.03125000204835970 ) ) ;
#35562=CARTESIAN_POINT ( 'NONE',  ( 7.070501591499377789E-16, 11.54700538379251284, 0.9999999959032501717 ) ) ;
#35568=CARTESIAN_POINT ( 'NONE',  ( 7.070501591499376803E-16, 11.54700538379251284, -116.0000000040967905 ) ) ;
#35576=VECTOR ( 'NONE', #35130, 1000.000000000000000 ) ;
#35578=CARTESIAN_POINT ( 'NONE',  ( -10.81189881249999907, -6.242252689847864744, -159.6562500020484094 ) ) ;
#35585=CARTESIAN_POINT ( 'NONE',  ( 7.644554776091147741E-16, 12.48450537969573659, -74.46875000204838102 ) ) ;
#35586=CARTESIAN_POINT ( 'NONE',  ( 10.81189881249999907, 6.242252689847868297, -83.90625000204836681 ) ) ;
#35589=CARTESIAN_POINT ( 'NONE',  ( 10.81189881249999551, -6.242252689847874514, -163.6562500020484094 ) ) ;
#35590=CARTESIAN_POINT ( 'NONE',  ( 5.405949406249992428, -9.363379034771808662, -178.7812500020484094 ) ) ;
#35592=CARTESIAN_POINT ( 'NONE',  ( 7.070501591499377789E-16, 11.54700538379251284, -159.5000000040967905 ) ) ;
#35594=CARTESIAN_POINT ( 'NONE',  ( 10.81189881249999907, 6.242252689847868297, -5.718750002048356151 ) ) ;
#35596=CARTESIAN_POINT ( 'NONE',  ( 10.81189881249999729, 0.000000000000000000, -110.8437500020483810 ) ) ;
#35598=CARTESIAN_POINT ( 'NONE',  ( 7.644554776091147741E-16, 12.48450537969573659, -8.656250002048365033 ) ) ;
#35601=CARTESIAN_POINT ( 'NONE',  ( -5.405949406250003975, -9.363379034771801557, -108.5312500020483810 ) ) ;
#35603=EDGE_LOOP ( 'NONE', ( #37336, #16097, #7052, #25982 ) ) ;
#35605=CARTESIAN_POINT ( 'NONE',  ( -9.999999999999998224, 1.224646799147353059E-15, -93.12500000409677625 ) ) ;
#35606=FACE_OUTER_BOUND ( 'NONE', #1369, .T. ) ;
#35607=CARTESIAN_POINT ( 'NONE',  ( -2.293366432827344421E-15, -12.48450537969573659, -43.71875000204835970 ) ) ;
#35608=ORIENTED_EDGE ( 'NONE', *, *, #34791, .F. ) ;
#35612=CARTESIAN_POINT ( 'NONE',  ( -9.999999999999998224, 1.224646799147353059E-15, -19.62500000409675494 ) ) ;
#35615=ORIENTED_EDGE ( 'NONE', *, *, #22537, .F. ) ;
#35622=EDGE_LOOP ( 'NONE', ( #25309, #17425, #38033, #10306 ) ) ;
#35624=DIRECTION ( 'NONE',  ( -1.000000000000000000, 0.000000000000000000, 0.000000000000000000 ) ) ;
#35628=CARTESIAN_POINT ( 'NONE',  ( 10.81189881249999907, 6.242252689847868297, -176.9062500020484094 ) ) ;
#35630=CARTESIAN_POINT ( 'NONE',  ( 35.00000000000000711, 4.286263797015737285E-15, -169.9999999999999716 ) ) ;
#35632=CARTESIAN_POINT ( 'NONE',  ( 5.405949406249999534, 9.363379034771803333, -103.0937500020483810 ) ) ;
#35634=CARTESIAN_POINT ( 'NONE',  ( -10.81189881249999729, 6.242252689847871849, -110.4062500020483810 ) ) ;
#35636=CARTESIAN_POINT ( 'NONE',  ( 5.405949406249992428, -9.363379034771808662, -118.5937500020483810 ) ) ;
#35639=CARTESIAN_POINT ( 'NONE',  ( 9.999999999999996447, -5.773502691896262640, -135.6250000000000000 ) ) ;
#35640=CARTESIAN_POINT ( 'NONE',  ( 10.00000000000000000, 5.773502691896255534, -4.874999999999962697 ) ) ;
#35643=CARTESIAN_POINT ( 'NONE',  ( -10.00000000000000000, -5.773502691896251982, -187.5000000040967905 ) ) ;
#35645=CARTESIAN_POINT ( 'NONE',  ( 7.644554776091147741E-16, 12.48450537969573659, -39.96875000204835970 ) ) ;
#35646=CARTESIAN_POINT ( 'NONE',  ( 7.070501591499376803E-16, 11.54700538379251284, -149.0000000040967905 ) ) ;
#35647=CARTESIAN_POINT ( 'NONE',  ( -10.81189881249999729, 1.324075727343319199E-15, -135.5937500020483810 ) ) ;
#35650=CARTESIAN_POINT ( 'NONE',  ( 5.000000000000000000, 8.660254037844385522, -67.74999999999997158 ) ) ;
#35651=CARTESIAN_POINT ( 'NONE',  ( 10.81189881249999551, -6.242252689847874514, -136.6562500020484094 ) ) ;
#35653=ORIENTED_EDGE ( 'NONE', *, *, #17595, .T. ) ;
#35655=CARTESIAN_POINT ( 'NONE',  ( -2.121150477449813534E-15, -11.54700538379251284, -116.7500000040967905 ) ) ;
#35657=CARTESIAN_POINT ( 'NONE',  ( 10.81189881249999907, 6.242252689847868297, -73.21875000204836681 ) ) ;
#35662=CARTESIAN_POINT ( 'NONE',  ( 10.00000000000000000, 5.773502691896255534, -47.25000000409676204 ) ) ;
#35663=CARTESIAN_POINT ( 'NONE',  ( 5.405949406249992428, -9.363379034771808662, -33.28125000204837391 ) ) ;
#35673=EDGE_CURVE ( 'NONE', #35190, #24289, #34091, .T. ) ;
#35678=AXIS2_PLACEMENT_3D ( 'NONE', #21976, #5155, #12457 ) ;
#35681=CARTESIAN_POINT ( 'NONE',  ( -9.999999999999998224, 1.224646799147353059E-15, -176.7500000000000284 ) ) ;
#35682=CARTESIAN_POINT ( 'NONE',  ( 10.81189881249999551, -6.242252689847874514, -128.9687500020483810 ) ) ;
#35683=CARTESIAN_POINT ( 'NONE',  ( -10.81189881249999729, 1.324075727343319199E-15, -135.7812500020483810 ) ) ;
#35685=CARTESIAN_POINT ( 'NONE',  ( 5.405949406249992428, -9.363379034771808662, -150.0937500020483810 ) ) ;
#35687=CARTESIAN_POINT ( 'NONE',  ( 7.070501591499376803E-16, 11.54700538379251284, -141.5000000040967905 ) ) ;
#35688=CARTESIAN_POINT ( 'NONE',  ( 10.00000000000000000, 5.773502691896255534, -166.8750000000000000 ) ) ;
#35691=CARTESIAN_POINT ( 'NONE',  ( -5.405949406249996869, 9.363379034771805109, -57.84375000204835970 ) ) ;
#35692=DIRECTION ( 'NONE',  ( -0.000000000000000000, -0.000000000000000000, -1.000000000000000000 ) ) ;
#35693=CARTESIAN_POINT ( 'NONE',  ( 5.405949406249992428, -9.363379034771808662, -169.5937500020484094 ) ) ;
#35699=CARTESIAN_POINT ( 'NONE',  ( 9.999999999999996447, -5.773502691896262640, -93.62499999999998579 ) ) ;
#35701=CARTESIAN_POINT ( 'NONE',  ( 5.405949406249999534, 9.363379034771803333, -121.2812500020483952 ) ) ;
#35702=CARTESIAN_POINT ( 'NONE',  ( 9.999999999999996447, -5.773502691896262640, -142.0000000040967905 ) ) ;
#35706=CARTESIAN_POINT ( 'NONE',  ( 10.00000000000025402, -5.773502691896113426, -159.6250000000000284 ) ) ;
#35707=CARTESIAN_POINT ( 'NONE',  ( 5.405949406249999534, 9.363379034771803333, -62.78125000204837391 ) ) ;
#35708=CARTESIAN_POINT ( 'NONE',  ( -22.00000000000000711, 0.000000000000000000, -99.99999999999998579 ) ) ;
#35722=ORIENTED_EDGE ( 'NONE', *, *, #7691, .F. ) ;
#35728=EDGE_CURVE ( 'NONE', #27698, #17741, #3637, .T. ) ;
#35729=CARTESIAN_POINT ( 'NONE',  ( 9.999999999999998224, 0.000000000000000000, -138.5000000000000000 ) ) ;
#35730=CARTESIAN_POINT ( 'NONE',  ( -9.999999999999998224, 1.224646799147353059E-15, -31.24999999999997158 ) ) ;
#35734=CARTESIAN_POINT ( 'NONE',  ( -5.405949406250003975, -9.363379034771801557, -156.3437500020483810 ) ) ;
#35735=( BOUNDED_CURVE ( )  B_SPLINE_CURVE ( 2, ( #22685, #15550, #42511, #12528, #13151, #23108, #25513 ),
 .UNSPECIFIED., .F., .F. ) 
 B_SPLINE_CURVE_WITH_KNOTS ( ( 3, 2, 2, 3 ),
 ( 0.4664179104477613191, 0.4676616915422886489, 0.4689054726368160342, 0.4701492537313434195 ),
 .UNSPECIFIED. ) 
 CURVE ( )  GEOMETRIC_REPRESENTATION_ITEM ( )  RATIONAL_B_SPLINE_CURVE ( ( 0.9999999999999880096, 0.8660254037844506980, 1.000000000000000000, 0.8660254037844387076, 1.000000000000000000, 0.8660254037844267172, 1.000000000000011990 ) ) 
 REPRESENTATION_ITEM ( '' )  );
#35736=CARTESIAN_POINT ( 'NONE',  ( -5.405949406250003975, -9.363379034771801557, -171.3437500020484094 ) ) ;
#35737=CARTESIAN_POINT ( 'NONE',  ( 0.000000000000000000, 0.000000000000000000, -99.99999999999998579 ) ) ;
#35738=CARTESIAN_POINT ( 'NONE',  ( 9.999999999999998224, 0.000000000000000000, -168.5000000000000000 ) ) ;
#35739=CARTESIAN_POINT ( 'NONE',  ( 9.999999999999998224, 0.000000000000000000, -188.0000000000000000 ) ) ;
#35745=VECTOR ( 'NONE', #22305, 1000.000000000000000 ) ;
#35746=CARTESIAN_POINT ( 'NONE',  ( 5.405949406249999534, 9.363379034771803333, -59.78125000204836681 ) ) ;
#35748=CARTESIAN_POINT ( 'NONE',  ( -10.00000000000000000, -5.773502691896251982, -118.1250000000000142 ) ) ;
#35749=EDGE_CURVE ( 'NONE', #8116, #9826, #30177, .T. ) ;
#35751=CARTESIAN_POINT ( 'NONE',  ( 10.81189881249999729, 0.000000000000000000, -142.5312500020483810 ) ) ;
#35752=CARTESIAN_POINT ( 'NONE',  ( 10.81189881249999551, -6.242252689847874514, -159.1562500020484094 ) ) ;
#35754=CARTESIAN_POINT ( 'NONE',  ( 9.999999999999998224, 0.000000000000000000, -179.0000000000000000 ) ) ;
#35755=CARTESIAN_POINT ( 'NONE',  ( -5.405949406250003975, -9.363379034771801557, -88.84375000204838102 ) ) ;
#35758=CARTESIAN_POINT ( 'NONE',  ( 5.405949406249992428, -9.363379034771808662, -192.0937500020484094 ) ) ;
#35760=CARTESIAN_POINT ( 'NONE',  ( 9.999999999999998224, 1.224646799147353059E-15, -99.99999999999998579 ) ) ;
#35762=CARTESIAN_POINT ( 'NONE',  ( 7.644554776091147741E-16, 12.48450537969573659, -85.15625000204838102 ) ) ;
#35764=CARTESIAN_POINT ( 'NONE',  ( 9.999999999999996447, -5.773502691896262640, -64.00000000409677625 ) ) ;
#35765=CARTESIAN_POINT ( 'NONE',  ( -5.405949406250003975, -9.363379034771801557, -16.84375000204835260 ) ) ;
#35766=CARTESIAN_POINT ( 'NONE',  ( 5.000000000000000000, 8.660254037844385522, -100.7499999999999858 ) ) ;
#35768=CARTESIAN_POINT ( 'NONE',  ( -2.293366432827344421E-15, -12.48450537969573659, -12.40625000204836859 ) ) ;
#35777=AXIS2_PLACEMENT_3D ( 'NONE', #8837, #8198, #21347 ) ;
#35787=CARTESIAN_POINT ( 'NONE',  ( 9.999999999999998224, 0.000000000000000000, -125.0000000000000000 ) ) ;
#35788=FACE_BOUND ( 'NONE', #8985, .T. ) ;
#35789=CARTESIAN_POINT ( 'NONE',  ( -10.81189881249999729, 1.324075727343319199E-15, -158.2812500020484094 ) ) ;
#35796=CARTESIAN_POINT ( 'NONE',  ( 10.81189881249999551, -6.242252689847874514, -77.96875000204838102 ) ) ;
#35797=CARTESIAN_POINT ( 'NONE',  ( 10.81189881249999551, -6.242252689847874514, -85.65625000204838102 ) ) ;
#35800=CARTESIAN_POINT ( 'NONE',  ( -10.81189881249999729, -6.242252689847864744, -168.6562500020484094 ) ) ;
#35801=CARTESIAN_POINT ( 'NONE',  ( 7.644554776091147741E-16, 12.48450537969573659, -179.6562500020484094 ) ) ;
#35802=CARTESIAN_POINT ( 'NONE',  ( -2.121150477449813534E-15, -11.54700538379251284, -155.7500000040967620 ) ) ;
#35804=CARTESIAN_POINT ( 'NONE',  ( -2.293366432827344421E-15, -12.48450537969573659, -9.218750002048359704 ) ) ;
#35806=CARTESIAN_POINT ( 'NONE',  ( -5.405949406249996869, 9.363379034771805109, -114.8437500020483810 ) ) ;
#35808=CARTESIAN_POINT ( 'NONE',  ( -10.81189881249999907, -6.242252689847864744, -14.15625000204837036 ) ) ;
#35811=CARTESIAN_POINT ( 'NONE',  ( -10.81189881249999729, 6.242252689847871849, -105.9062500020483810 ) ) ;
#35813=EDGE_LOOP ( 'NONE', ( #349, #9056, #37, #5450 ) ) ;
#35814=CARTESIAN_POINT ( 'NONE',  ( 9.999999999999996447, -5.773502691896262640, -85.00000000409677625 ) ) ;
#35815=CARTESIAN_POINT ( 'NONE',  ( -35.00000000000000711, 0.000000000000000000, -176.9999999999999432 ) ) ;
#35816=CARTESIAN_POINT ( 'NONE',  ( 10.81189881249999907, 6.242252689847868297, -43.21875000204835970 ) ) ;
#35821=CARTESIAN_POINT ( 'NONE',  ( 10.00000000000000000, 5.773502691896255534, -11.25000000409676204 ) ) ;
#35822=CARTESIAN_POINT ( 'NONE',  ( 4.999999999999992006, -8.660254037844389075, -119.6250000040967905 ) ) ;
#35824=ORIENTED_EDGE ( 'NONE', *, *, #13545, .F. ) ;
#35826=( BOUNDED_CURVE ( )  B_SPLINE_CURVE ( 2, ( #12378, #35503, #25573, #14976, #28390, #1850, #15611 ),
 .UNSPECIFIED., .F., .F. ) 
 B_SPLINE_CURVE_WITH_KNOTS ( ( 3, 2, 2, 3 ),
 ( 0.2537313432835822113, 0.2549751243781095411, 0.2562189054726369264, 0.2574626865671643117 ),
 .UNSPECIFIED. ) 
 CURVE ( )  GEOMETRIC_REPRESENTATION_ITEM ( )  RATIONAL_B_SPLINE_CURVE ( ( 0.9999999999999880096, 0.8660254037844506980, 1.000000000000000000, 0.8660254037844387076, 1.000000000000000000, 0.8660254037844267172, 1.000000000000011990 ) ) 
 REPRESENTATION_ITEM ( '' )  );
#35831=ORIENTED_EDGE ( 'NONE', *, *, #38942, .T. ) ;
#35834=CARTESIAN_POINT ( 'NONE',  ( -2.293366432827344421E-15, -12.48450537969573659, -180.4062500020484379 ) ) ;
#35836=CARTESIAN_POINT ( 'NONE',  ( 4.999999999999992006, -8.660254037844389075, -146.6250000040967905 ) ) ;
#35839=CARTESIAN_POINT ( 'NONE',  ( 10.81189881249999551, -6.242252689847874514, -103.4687500020483810 ) ) ;
#35841=CARTESIAN_POINT ( 'NONE',  ( 5.405949406249999534, 9.363379034771803333, -109.2812500020483810 ) ) ;
#35843=CARTESIAN_POINT ( 'NONE',  ( -10.81189881249999729, -6.242252689847864744, -117.4687500020483810 ) ) ;
#35846=CARTESIAN_POINT ( 'NONE',  ( 5.000000000000000000, 8.660254037844385522, -138.2499999999999716 ) ) ;
#35847=CARTESIAN_POINT ( 'NONE',  ( -9.999999999999998224, 5.773502691896259087, -5.874999999999963585 ) ) ;
#35850=CARTESIAN_POINT ( 'NONE',  ( 9.999999999999998224, 0.000000000000000000, -176.3750000040967905 ) ) ;
#35852=CARTESIAN_POINT ( 'NONE',  ( 10.81189881249999551, -6.242252689847874514, -31.46875000204835260 ) ) ;
#35854=CARTESIAN_POINT ( 'NONE',  ( 10.81189881249999907, 6.242252689847868297, -139.2187500020484094 ) ) ;
#35857=CARTESIAN_POINT ( 'NONE',  ( -9.999999999999998224, 5.773502691896259087, -70.37499999999998579 ) ) ;
#35858=CARTESIAN_POINT ( 'NONE',  ( 7.644554776091147741E-16, 12.48450537969573659, -136.1562500020483810 ) ) ;
#35863=CARTESIAN_POINT ( 'NONE',  ( -4.999999999999996447, 8.660254037844387298, -106.8750000040967763 ) ) ;
#35865=CARTESIAN_POINT ( 'NONE',  ( -5.405949406249996869, 9.363379034771805109, -65.34375000204836681 ) ) ;
#35870=CARTESIAN_POINT ( 'NONE',  ( 7.070501591499377789E-16, 11.54700538379251284, -44.00000000409676204 ) ) ;
#35871=CARTESIAN_POINT ( 'NONE',  ( -10.81189881249999729, 6.242252689847871849, -39.90625000204836681 ) ) ;
#35876=CARTESIAN_POINT ( 'NONE',  ( 7.070501591499376803E-16, 11.54700538379251284, -150.5000000040968189 ) ) ;
#35880=VERTEX_POINT ( 'NONE', #29750 ) ;
#35886=CARTESIAN_POINT ( 'NONE',  ( -2.121150477449813534E-15, -11.54700538379251284, -119.3749999999999858 ) ) ;
#35887=CARTESIAN_POINT ( 'NONE',  ( 5.405949406249992428, -9.363379034771808662, -123.0937500020483952 ) ) ;
#35888=CARTESIAN_POINT ( 'NONE',  ( 10.81189881249999729, 0.000000000000000000, -129.0312500020484094 ) ) ;
#35890=CARTESIAN_POINT ( 'NONE',  ( 7.644554776091147741E-16, 12.48450537969573659, -147.9687500020484094 ) ) ;
#35891=CARTESIAN_POINT ( 'NONE',  ( -2.121150477449813534E-15, -11.54700538379251284, -125.7500000040967763 ) ) ;
#35893=CARTESIAN_POINT ( 'NONE',  ( 4.999999999999992006, -8.660254037844389075, -161.2500000000000000 ) ) ;
#35898=CARTESIAN_POINT ( 'NONE',  ( -10.81189881249999729, 1.324075727343319199E-15, -54.59375000204835970 ) ) ;
#35899=DIRECTION ( 'NONE',  ( -1.000000000000000000, 0.000000000000000000, 0.000000000000000000 ) ) ;
#35900=CARTESIAN_POINT ( 'NONE',  ( 5.405949406249992428, -9.363379034771808662, -160.5937500020484094 ) ) ;
#35903=CARTESIAN_POINT ( 'NONE',  ( 0.000000000000000000, 0.000000000000000000, -99.99999999999998579 ) ) ;
#35905=CARTESIAN_POINT ( 'NONE',  ( 5.000000000000000000, 8.660254037844385522, -93.24999999999998579 ) ) ;
#35907=CARTESIAN_POINT ( 'NONE',  ( 7.644554776091147741E-16, 12.48450537969573659, -116.6562500020483952 ) ) ;
#35908=CARTESIAN_POINT ( 'NONE',  ( -9.999999999999998224, 5.773502691896259087, -136.7500000040967905 ) ) ;
#35912=ADVANCED_FACE ( 'NONE', ( #20439 ), #32986, .F. ) ;
#35913=DIRECTION ( 'NONE',  ( -0.000000000000000000, -0.000000000000000000, -1.000000000000000000 ) ) ;
#35914=CARTESIAN_POINT ( 'NONE',  ( 5.405949406249999534, 9.363379034771803333, -58.28125000204836681 ) ) ;
#35929=CARTESIAN_POINT ( 'NONE',  ( -10.00000000000000000, -5.773502691896251982, -32.62499999999995737 ) ) ;
#35933=CARTESIAN_POINT ( 'NONE',  ( -5.405949406250003975, -9.363379034771801557, -151.8437500020483810 ) ) ;
#35934=CARTESIAN_POINT ( 'NONE',  ( -5.405949406250003975, -9.363379034771801557, -168.3437500020484094 ) ) ;
#35937=CARTESIAN_POINT ( 'NONE',  ( -4.999999999999996447, 8.660254037844387298, -186.0000000000000000 ) ) ;
#35942=CARTESIAN_POINT ( 'NONE',  ( 5.405949406249999534, 9.363379034771803333, -184.0937500020483810 ) ) ;
#35944=CARTESIAN_POINT ( 'NONE',  ( 5.405949406249999534, 9.363379034771803333, -64.28125000204836681 ) ) ;
#35946=CARTESIAN_POINT ( 'NONE',  ( -2.121150477449813534E-15, -11.54700538379251284, -113.3749999999999858 ) ) ;
#35948=ORIENTED_EDGE ( 'NONE', *, *, #1695, .F. ) ;
#35949=CARTESIAN_POINT ( 'NONE',  ( -10.81189881249999729, 6.242252689847871849, -141.9062500020484094 ) ) ;
#35950=CARTESIAN_POINT ( 'NONE',  ( 10.81189881249999551, -6.242252689847874514, -157.6562500020484094 ) ) ;
#35954=CARTESIAN_POINT ( 'NONE',  ( 10.81189881249999729, 0.000000000000000000, -92.84375000204838102 ) ) ;
#35957=CARTESIAN_POINT ( 'NONE',  ( 7.644554776091147741E-16, 12.48450537969573659, -189.9687500020484094 ) ) ;
#35963=CARTESIAN_POINT ( 'NONE',  ( -2.293366432827344421E-15, -12.48450537969573659, -82.90625000204838102 ) ) ;
#35966=CARTESIAN_POINT ( 'NONE',  ( -4.999999999999996447, 8.660254037844387298, -61.87500000409676204 ) ) ;
#35967=CARTESIAN_POINT ( 'NONE',  ( -10.81189881249999907, -6.242252689847864744, -19.96875000204837036 ) ) ;
#35970=CIRCLE ( 'NONE', #41472, 35.00000000000000711 ) ;
#35971=CARTESIAN_POINT ( 'NONE',  ( 10.81189881249999729, 0.000000000000000000, -9.031250002048352599 ) ) ;
#35979=CARTESIAN_POINT ( 'NONE',  ( -5.000000000000003553, -8.660254037844383745, -160.3750000040967905 ) ) ;
#35980=EDGE_CURVE ( 'NONE', #31308, #32304, #9505, .T. ) ;
#35981=CARTESIAN_POINT ( 'NONE',  ( 5.405949406249999534, 9.363379034771803333, -103.0937500020483810 ) ) ;
#35994=CARTESIAN_POINT ( 'NONE',  ( 7.644554776091147741E-16, 12.48450537969573659, -154.1562500020484094 ) ) ;
#35996=CARTESIAN_POINT ( 'NONE',  ( -4.999999999999996447, 8.660254037844387298, -121.5000000000000000 ) ) ;
#36001=CARTESIAN_POINT ( 'NONE',  ( -5.405949406249996869, 9.363379034771805109, -75.84375000204838102 ) ) ;
#36002=CARTESIAN_POINT ( 'NONE',  ( 7.644554776091147741E-16, 12.48450537969573659, -83.65625000204838102 ) ) ;
#36004=CARTESIAN_POINT ( 'NONE',  ( 5.405949406249999534, 9.363379034771803333, -163.2812500020484094 ) ) ;
#36005=CARTESIAN_POINT ( 'NONE',  ( 10.81189881249999551, -6.242252689847874514, -177.1562500020484094 ) ) ;
#36006=CARTESIAN_POINT ( 'NONE',  ( 9.999999999999998224, 0.000000000000000000, -153.8750000040967905 ) ) ;
#36008=CARTESIAN_POINT ( 'NONE',  ( 10.81189881249999729, 0.000000000000000000, -5.843750002048370362 ) ) ;
#36010=CARTESIAN_POINT ( 'NONE',  ( 10.81189881249999907, 6.242252689847868297, -116.7187500020483810 ) ) ;
#36012=CARTESIAN_POINT ( 'NONE',  ( 5.405949406249992428, -9.363379034771808662, -12.28125000204835438 ) ) ;
#36015=CARTESIAN_POINT ( 'NONE',  ( -5.405949406249996869, 9.363379034771805109, -110.5312500020483810 ) ) ;
#36019=CARTESIAN_POINT ( 'NONE',  ( -10.00000000000000000, -5.773502691896251982, -81.00000000409677625 ) ) ;
#36021=CARTESIAN_POINT ( 'NONE',  ( -5.405949406250003975, -9.363379034771801557, -42.34375000204837391 ) ) ;
#36025=CARTESIAN_POINT ( 'NONE',  ( 9.999999999999998224, 0.000000000000000000, -14.37500000409674961 ) ) ;
#36030=EDGE_LOOP ( 'NONE', ( #37461, #3334, #33214, #28512 ) ) ;
#36038=DIRECTION ( 'NONE',  ( -1.000000000000000000, 0.000000000000000000, 0.000000000000000000 ) ) ;
#36040=CARTESIAN_POINT ( 'NONE',  ( 10.81189881249999729, 0.000000000000000000, -181.5312500020483810 ) ) ;
#36042=CARTESIAN_POINT ( 'NONE',  ( -9.999999999999998224, 1.224646799147353059E-15, -154.6250000040967905 ) ) ;
#36044=CARTESIAN_POINT ( 'NONE',  ( 10.81189881249999729, 0.000000000000000000, -104.8437500020483810 ) ) ;
#36046=CARTESIAN_POINT ( 'NONE',  ( 10.81189881249999729, 0.000000000000000000, -109.5312500020483810 ) ) ;
#36048=CARTESIAN_POINT ( 'NONE',  ( -10.81189881249999729, 6.242252689847871849, -117.7187500020483952 ) ) ;
#36051=CARTESIAN_POINT ( 'NONE',  ( 9.999999999999996447, -5.773502691896262640, -141.6250000000000000 ) ) ;
#36052=CARTESIAN_POINT ( 'NONE',  ( 10.00000000000000000, 5.773502691896255534, -6.374999999999963585 ) ) ;
#36056=CARTESIAN_POINT ( 'NONE',  ( 9.999999999999996447, -5.773502691896262640, -181.0000000040968189 ) ) ;
#36058=CARTESIAN_POINT ( 'NONE',  ( -5.405949406250003975, -9.363379034771801557, -30.34375000204836326 ) ) ;
#36060=CARTESIAN_POINT ( 'NONE',  ( -10.81189881249999729, 1.324075727343319199E-15, -141.5937500020483810 ) ) ;
#36063=CARTESIAN_POINT ( 'NONE',  ( -2.121150477449813534E-15, -11.54700538379251284, -69.87500000000000000 ) ) ;
#36064=CARTESIAN_POINT ( 'NONE',  ( 5.405949406249999534, 9.363379034771803333, -134.7812500020483810 ) ) ;
#36067=CARTESIAN_POINT ( 'NONE',  ( 9.999999999999998224, 0.000000000000000000, -108.8750000040967763 ) ) ;
#36068=CARTESIAN_POINT ( 'NONE',  ( -9.999999999999998224, 1.224646799147353059E-15, -113.7499999999999858 ) ) ;
#36069=CARTESIAN_POINT ( 'NONE',  ( 10.81189881249999907, 6.242252689847868297, -64.21875000204838102 ) ) ;
#36070=ORIENTED_EDGE ( 'NONE', *, *, #10961, .T. ) ;
#36074=CARTESIAN_POINT ( 'NONE',  ( -2.121150477449813534E-15, -11.54700538379251284, -131.7500000040967905 ) ) ;
#36075=CARTESIAN_POINT ( 'NONE',  ( -10.00000000000000000, -5.773502691896251982, -33.00000000409675494 ) ) ;
#36076=CARTESIAN_POINT ( 'NONE',  ( 7.070501591499376803E-16, 11.54700538379251284, -117.5000000040967905 ) ) ;
#36078=ADVANCED_FACE ( 'NONE', ( #14592, #27568 ), #7717, .F. ) ;
#36080=CARTESIAN_POINT ( 'NONE',  ( 5.000000000000000000, 8.660254037844385522, -150.6250000040967905 ) ) ;
#36081=VERTEX_POINT ( 'NONE', #40917 ) ;
#36082=EDGE_LOOP ( 'NONE', ( #12911, #28296, #40514, #21901 ) ) ;
#36083=VERTEX_POINT ( 'NONE', #15236 ) ;
#36085=CARTESIAN_POINT ( 'NONE',  ( 9.999999999999998224, 0.000000000000000000, -103.9999999999999858 ) ) ;
#36088=CARTESIAN_POINT ( 'NONE',  ( -4.999999999999996447, 8.660254037844387298, -111.3750000040967763 ) ) ;
#36091=FACE_OUTER_BOUND ( 'NONE', #16575, .T. ) ;
#36092=CARTESIAN_POINT ( 'NONE',  ( 7.644554776091147741E-16, 12.48450537969573659, -126.9687500020483668 ) ) ;
#36093=CARTESIAN_POINT ( 'NONE',  ( -5.405949406250003975, -9.363379034771801557, -131.0312500020484094 ) ) ;
#36096=CARTESIAN_POINT ( 'NONE',  ( -5.405949406249996869, 9.363379034771805109, -141.8437500020483810 ) ) ;
#36099=CARTESIAN_POINT ( 'NONE',  ( 9.999999999999996447, -5.773502691896262640, -165.6250000000000000 ) ) ;
#36103=CARTESIAN_POINT ( 'NONE',  ( -10.81189881249999729, 6.242252689847871849, -56.21875000204837391 ) ) ;
#36104=CARTESIAN_POINT ( 'NONE',  ( 9.999999999999866773, -5.773502691896336358, -174.6249999999999716 ) ) ;
#36105=CARTESIAN_POINT ( 'NONE',  ( -10.81189881249999729, 1.324075727343319199E-15, -159.5937500020484094 ) ) ;
#36110=CARTESIAN_POINT ( 'NONE',  ( -2.121150477449813534E-15, -11.54700538379251284, -87.87499999999997158 ) ) ;
#36113=CARTESIAN_POINT ( 'NONE',  ( 10.81189881249999729, 0.000000000000000000, -120.0312500020483952 ) ) ;
#36114=CARTESIAN_POINT ( 'NONE',  ( -9.999999999999998224, 1.224646799147353059E-15, -133.6250000040967620 ) ) ;
#36119=CARTESIAN_POINT ( 'NONE',  ( -2.293366432827344421E-15, -12.48450537969573659, -60.40625000204838813 ) ) ;
#36126=CARTESIAN_POINT ( 'NONE',  ( -9.999999999999998224, 1.224646799147353059E-15, -173.7500000000000284 ) ) ;
#36138=CARTESIAN_POINT ( 'NONE',  ( -9.999999999999227285, -5.773502691896698735, -134.6249999999999716 ) ) ;
#36140=CARTESIAN_POINT ( 'NONE',  ( 9.999999999999998224, 0.000000000000000000, -25.99999999999996803 ) ) ;
#36143=CARTESIAN_POINT ( 'NONE',  ( 10.81189881249999729, 0.000000000000000000, -151.3437500020483810 ) ) ;
#36144=CARTESIAN_POINT ( 'NONE',  ( -2.293366432827344421E-15, -12.48450537969573659, -163.7187500020483810 ) ) ;
#36146=CARTESIAN_POINT ( 'NONE',  ( -9.999999999999998224, 5.773502691896259087, -190.3750000000000000 ) ) ;
#36151=CARTESIAN_POINT ( 'NONE',  ( 10.81189881249999551, -6.242252689847874514, -184.4687500020483810 ) ) ;
#36153=CARTESIAN_POINT ( 'NONE',  ( 10.81189881249999907, 6.242252689847868297, -59.90625000204838102 ) ) ;
#36155=CARTESIAN_POINT ( 'NONE',  ( -10.00000000000000000, -5.773502691896251982, -116.6249999999999858 ) ) ;
#36157=CARTESIAN_POINT ( 'NONE',  ( -10.81189881249999729, 1.324075727343319199E-15, -144.7812500020483810 ) ) ;
#36158=CARTESIAN_POINT ( 'NONE',  ( -10.81189881249999729, 1.324075727343319199E-15, -153.7812500020484094 ) ) ;
#36160=FACE_OUTER_BOUND ( 'NONE', #16412, .T. ) ;
#36161=CARTESIAN_POINT ( 'NONE',  ( -2.293366432827344421E-15, -12.48450537969573659, -90.21875000204838102 ) ) ;
#36162=ORIENTED_EDGE ( 'NONE', *, *, #42434, .T. ) ;
#36164=CARTESIAN_POINT ( 'NONE',  ( 10.81189881249999729, 0.000000000000000000, -188.8437500020483810 ) ) ;
#36166=CARTESIAN_POINT ( 'NONE',  ( 9.999999999999998224, 0.000000000000000000, -168.8750000040967905 ) ) ;
#36168=CARTESIAN_POINT ( 'NONE',  ( -5.405949406250003975, -9.363379034771801557, -84.53125000204838102 ) ) ;
#36170=CARTESIAN_POINT ( 'NONE',  ( 5.000000000000000000, 8.660254037844385522, -60.62500000409676204 ) ) ;
#36171=CARTESIAN_POINT ( 'NONE',  ( 10.81189881249999907, 6.242252689847868297, -20.71875000204837036 ) ) ;
#36173=CARTESIAN_POINT ( 'NONE',  ( 7.644554776091147741E-16, 12.48450537969573659, -11.65625000204836859 ) ) ;
#36176=DIRECTION ( 'NONE',  ( -0.000000000000000000, -0.000000000000000000, -1.000000000000000000 ) ) ;
#36180=VERTEX_POINT ( 'NONE', #38770 ) ;
#36192=EDGE_CURVE ( 'NONE', #530, #13652, #40359, .T. ) ;
#36196=CARTESIAN_POINT ( 'NONE',  ( 5.000000000000000000, 8.660254037844385522, -172.7500000000000284 ) ) ;
#36197=CARTESIAN_POINT ( 'NONE',  ( 7.644554776091147741E-16, 12.48450537969573659, -155.6562500020484094 ) ) ;
#36203=CARTESIAN_POINT ( 'NONE',  ( -2.293366432827344421E-15, -12.48450537969573659, -79.71875000204838102 ) ) ;
#36205=CARTESIAN_POINT ( 'NONE',  ( 10.81189881249999729, 0.000000000000000000, -81.03125000204839523 ) ) ;
#36208=CARTESIAN_POINT ( 'NONE',  ( 10.81189881249999729, 6.242252689847867408, -163.4062500020483810 ) ) ;
#36209=CARTESIAN_POINT ( 'NONE',  ( 5.405949406249999534, 9.363379034771803333, -184.2812500020484094 ) ) ;
#36210=CARTESIAN_POINT ( 'NONE',  ( 10.00000000000000000, 5.773502691896255534, -155.2500000040967905 ) ) ;
#36212=CARTESIAN_POINT ( 'NONE',  ( -2.293366432827344421E-15, -12.48450537969573659, -4.718750002048355263 ) ) ;
#36213=CARTESIAN_POINT ( 'NONE',  ( 9.999999999999479527, 5.773502691896553074, -108.7500000040967620 ) ) ;
#36214=CARTESIAN_POINT ( 'NONE',  ( -5.405949406249996869, 9.363379034771805109, -111.8437500020483810 ) ) ;
#36216=CARTESIAN_POINT ( 'NONE',  ( 5.405949406249999534, 9.363379034771803333, -10.28125000204835260 ) ) ;
#36220=CARTESIAN_POINT ( 'NONE',  ( 5.405949406249999534, 9.363379034771803333, -107.7812500020483810 ) ) ;
#36223=CARTESIAN_POINT ( 'NONE',  ( 9.999999999999998224, 0.000000000000000000, -80.37500000409677625 ) ) ;
#36225=CARTESIAN_POINT ( 'NONE',  ( 10.81189881249999729, 0.000000000000000000, -44.84375000204837391 ) ) ;
#36226=ORIENTED_EDGE ( 'NONE', *, *, #3031, .T. ) ;
#36232=CARTESIAN_POINT ( 'NONE',  ( -9.999999999999998224, 1.224646799147353059E-15, -15.12500000409674961 ) ) ;
#36236=ORIENTED_EDGE ( 'NONE', *, *, #27718, .T. ) ;
#36239=ORIENTED_EDGE ( 'NONE', *, *, #36721, .T. ) ;
#36240=AXIS2_PLACEMENT_3D ( 'NONE', #39304, #12749, #29185 ) ;
#36248=DIRECTION ( 'NONE',  ( 0.000000000000000000, 0.000000000000000000, -1.000000000000000000 ) ) ;
#36249=ADVANCED_FACE ( 'NONE', ( #25612 ), #5542, .F. ) ;
#36250=CARTESIAN_POINT ( 'NONE',  ( -5.405949406249996869, 9.363379034771805109, -181.0312500020483810 ) ) ;
#36251=DIRECTION ( 'NONE',  ( 1.000000000000000000, 0.000000000000000000, 0.000000000000000000 ) ) ;
#36255=CARTESIAN_POINT ( 'NONE',  ( -2.293366432827344421E-15, -12.48450537969573659, -99.21875000204839523 ) ) ;
#36257=CARTESIAN_POINT ( 'NONE',  ( 10.81189881249999551, -6.242252689847874514, -105.1562500020483810 ) ) ;
#36259=CARTESIAN_POINT ( 'NONE',  ( 5.405949406249999534, 9.363379034771803333, -113.5937500020483810 ) ) ;
#36263=CARTESIAN_POINT ( 'NONE',  ( -9.999999999999998224, 5.773502691896259087, -139.3750000000000000 ) ) ;
#36264=CARTESIAN_POINT ( 'NONE',  ( -5.000000000000003553, -8.660254037844383745, -6.999999999999978684 ) ) ;
#36267=CARTESIAN_POINT ( 'NONE',  ( -2.121150477449813534E-15, -11.54700538379251284, -179.7500000040967905 ) ) ;
#36269=CARTESIAN_POINT ( 'NONE',  ( -10.81189881249999729, 1.324075727343319199E-15, -27.59375000204836326 ) ) ;
#36270=CARTESIAN_POINT ( 'NONE',  ( -9.999999999999998224, 1.224646799147353059E-15, -142.6250000040967905 ) ) ;
#36271=CARTESIAN_POINT ( 'NONE',  ( 7.644554776091147741E-16, 12.48450537969573659, -135.9687500020483810 ) ) ;
#36273=CARTESIAN_POINT ( 'NONE',  ( -10.81189881249999729, 6.242252689847871849, -36.90625000204835970 ) ) ;
#36274=CYLINDRICAL_SURFACE ( 'NONE', #21749, 9.999999999999998224 ) ;
#36275=AXIS2_PLACEMENT_3D ( 'NONE', #32803, #23517, #7321 ) ;
#36276=CARTESIAN_POINT ( 'NONE',  ( 9.999999999999998224, 0.000000000000000000, -70.99999999999998579 ) ) ;
#36277=CARTESIAN_POINT ( 'NONE',  ( 10.81189881249999551, -6.242252689847874514, -135.1562500020484094 ) ) ;
#36279=EDGE_CURVE ( 'NONE', #11060, #32933, #6486, .T. ) ;
#36280=VERTEX_POINT ( 'NONE', #19321 ) ;
#36281=CARTESIAN_POINT ( 'NONE',  ( 5.000000000000000000, 8.660254037844385522, -142.7500000000000000 ) ) ;
#36282=CARTESIAN_POINT ( 'NONE',  ( -5.000000000000003553, -8.660254037844383745, -107.8750000040967763 ) ) ;
#36283=CARTESIAN_POINT ( 'NONE',  ( 5.000000000000000000, 8.660254037844385522, -162.2500000000000000 ) ) ;
#36284=CARTESIAN_POINT ( 'NONE',  ( -10.81189881249999907, -6.242252689847864744, -66.46875000204838102 ) ) ;
#36289=CARTESIAN_POINT ( 'NONE',  ( 7.070501591499376803E-16, 11.54700538379251284, -125.0000000040967763 ) ) ;
#36290=CARTESIAN_POINT ( 'NONE',  ( 10.00000000000000000, 5.773502691896255534, -36.75000000409675494 ) ) ;
#36291=CARTESIAN_POINT ( 'NONE',  ( 5.000000000000000000, 8.660254037844385522, -117.6250000040967905 ) ) ;
#36299=CARTESIAN_POINT ( 'NONE',  ( -9.999999999999998224, 1.224646799147353059E-15, -104.7499999999999858 ) ) ;
#36306=CARTESIAN_POINT ( 'NONE',  ( -2.293366432827344421E-15, -12.48450537969573659, -129.2187500020483810 ) ) ;
#36307=CARTESIAN_POINT ( 'NONE',  ( 5.405949406249992428, -9.363379034771808662, -129.2812500020483810 ) ) ;
#36309=CARTESIAN_POINT ( 'NONE',  ( 5.405949406249999534, 9.363379034771803333, -142.0937500020483810 ) ) ;
#36310=DIRECTION ( 'NONE',  ( -0.000000000000000000, -0.000000000000000000, -1.000000000000000000 ) ) ;
#36311=CARTESIAN_POINT ( 'NONE',  ( -2.121150477449813534E-15, -11.54700538379251284, -161.3750000000000000 ) ) ;
#36316=CARTESIAN_POINT ( 'NONE',  ( 10.81189881249999907, 6.242252689847868297, -56.71875000204838813 ) ) ;
#36317=DIRECTION ( 'NONE',  ( -1.000000000000000000, 0.000000000000000000, 0.000000000000000000 ) ) ;
#36318=CARTESIAN_POINT ( 'NONE',  ( 10.81189881249999729, 0.000000000000000000, -158.8437500020483810 ) ) ;
#36321=DIRECTION ( 'NONE',  ( -0.000000000000000000, -0.000000000000000000, -1.000000000000000000 ) ) ;
#36323=CARTESIAN_POINT ( 'NONE',  ( -9.999999999999998224, 1.224646799147353059E-15, -91.24999999999998579 ) ) ;
#36325=CARTESIAN_POINT ( 'NONE',  ( 10.81189881249999551, -6.242252689847874514, -112.6562500020483952 ) ) ;
#36326=CARTESIAN_POINT ( 'NONE',  ( 5.000000000000000000, 8.660254037844385522, -132.6250000040967620 ) ) ;
#36327=CARTESIAN_POINT ( 'NONE',  ( 4.999999999999992006, -8.660254037844389075, -177.7500000000000284 ) ) ;
#36330=DIRECTION ( 'NONE',  ( -1.000000000000000000, 0.000000000000000000, 0.000000000000000000 ) ) ;
#36331=CARTESIAN_POINT ( 'NONE',  ( 10.81189881249999551, -6.242252689847874514, -54.15625000204837391 ) ) ;
#36336=CARTESIAN_POINT ( 'NONE',  ( -9.999999999999998224, 1.224646799147353059E-15, -171.1250000040968189 ) ) ;
#36337=VERTEX_POINT ( 'NONE', #18694 ) ;
#36340=VERTEX_POINT ( 'NONE', #31890 ) ;
#36344=ORIENTED_EDGE ( 'NONE', *, *, #303, .F. ) ;
#36350=CARTESIAN_POINT ( 'NONE',  ( -2.121150477449813534E-15, -11.54700538379251284, -24.87499999999997868 ) ) ;
#36353=CARTESIAN_POINT ( 'NONE',  ( -5.405949406250003975, -9.363379034771801557, -148.8437500020483810 ) ) ;
#36354=CARTESIAN_POINT ( 'NONE',  ( 5.405949406249992428, -9.363379034771808662, -162.0937500020484094 ) ) ;
#36356=CARTESIAN_POINT ( 'NONE',  ( 5.000000000000000000, 8.660254037844385522, -102.6250000040967905 ) ) ;
#36357=CARTESIAN_POINT ( 'NONE',  ( 4.999999999999992006, -8.660254037844389075, -188.2500000000000000 ) ) ;
#36359=CARTESIAN_POINT ( 'NONE',  ( 10.00000000000000000, 5.773502691896255534, -138.3750000000000000 ) ) ;
#36362=CARTESIAN_POINT ( 'NONE',  ( -10.81189881249999907, -6.242252689847864744, -186.4687500020484094 ) ) ;
#36365=CARTESIAN_POINT ( 'NONE',  ( 10.81189881249999907, 6.242252689847868297, -50.90625000204837391 ) ) ;
#36367=CARTESIAN_POINT ( 'NONE',  ( 10.00000000000000000, 5.773502691896255534, -115.8749999999999858 ) ) ;
#36369=CARTESIAN_POINT ( 'NONE',  ( 5.405949406249992428, -9.363379034771808662, -136.7812500020483810 ) ) ;
#36370=CARTESIAN_POINT ( 'NONE',  ( 7.644554776091147741E-16, 12.48450537969573659, -145.1562500020484094 ) ) ;
#36373=CARTESIAN_POINT ( 'NONE',  ( -10.81189881249999907, -6.242252689847864744, -84.46875000204836681 ) ) ;
#36377=CARTESIAN_POINT ( 'NONE',  ( -10.81189881249999729, 6.242252689847871849, -185.2187500020483810 ) ) ;
#36379=VECTOR ( 'NONE', #17750, 1000.000000000000000 ) ;
#36383=CARTESIAN_POINT ( 'NONE',  ( -5.405949406250003975, -9.363379034771801557, -81.53125000204839523 ) ) ;
#36385=CARTESIAN_POINT ( 'NONE',  ( -9.999999999999998224, 5.773502691896259087, -63.25000000409678336 ) ) ;
#36386=CARTESIAN_POINT ( 'NONE',  ( 10.81189881249999551, -6.242252689847874514, -19.46875000204836681 ) ) ;
#36389=CARTESIAN_POINT ( 'NONE',  ( 5.405949406249992428, -9.363379034771808662, -13.78125000204835615 ) ) ;
#36391=CARTESIAN_POINT ( 'NONE',  ( -9.999999999999998224, 1.224646799147353059E-15, -148.6250000040967905 ) ) ;
#36392=LINE ( 'NONE', #158, #13889 ) ;
#36400=ORIENTED_EDGE ( 'NONE', *, *, #32796, .F. ) ;
#36406=VECTOR ( 'NONE', #20160, 1000.000000000000000 ) ;
#36411=CARTESIAN_POINT ( 'NONE',  ( 10.81189881249999907, 6.242252689847868297, -149.9062500020484094 ) ) ;
#36415=CARTESIAN_POINT ( 'NONE',  ( 5.000000000000000000, 8.660254037844385522, -141.2500000000000000 ) ) ;
#36418=CARTESIAN_POINT ( 'NONE',  ( -10.81189881249999729, 6.242252689847871849, -66.71875000204838102 ) ) ;
#36419=CARTESIAN_POINT ( 'NONE',  ( -10.81189881249999729, 6.242252689847871849, -80.40625000204839523 ) ) ;
#36422=CARTESIAN_POINT ( 'NONE',  ( 10.81189881249999551, -6.242252689847874514, -169.6562500020484094 ) ) ;
#36423=CARTESIAN_POINT ( 'NONE',  ( 7.644554776091147741E-16, 12.48450537969573659, -184.1562500020484094 ) ) ;
#36424=CYLINDRICAL_SURFACE ( 'NONE', #14591, 9.999999999999998224 ) ;
#36425=CARTESIAN_POINT ( 'NONE',  ( -10.81189881249999729, 1.324075727343319199E-15, -3.593750002048368142 ) ) ;
#36427=CARTESIAN_POINT ( 'NONE',  ( 5.405949406249999534, 9.363379034771803333, -113.5937500020483810 ) ) ;
#36429=CARTESIAN_POINT ( 'NONE',  ( -10.81189881249999907, -6.242252689847864744, -15.65625000204837214 ) ) ;
#36432=CARTESIAN_POINT ( 'NONE',  ( 7.644554776091147741E-16, 12.48450537969573659, -106.1562500020483952 ) ) ;
#36435=CARTESIAN_POINT ( 'NONE',  ( -10.00000000000000000, -5.773502691896251982, -84.00000000409677625 ) ) ;
#36437=CARTESIAN_POINT ( 'NONE',  ( 5.405949406249999534, 9.363379034771803333, -44.59375000204837391 ) ) ;
#36438=VERTEX_POINT ( 'NONE', #16281 ) ;
#36444=CARTESIAN_POINT ( 'NONE',  ( 5.000000000000000000, 8.660254037844385522, -14.12500000409674961 ) ) ;
#36449=ORIENTED_EDGE ( 'NONE', *, *, #5790, .F. ) ;
#36458=CARTESIAN_POINT ( 'NONE',  ( 5.405949406249992428, -9.363379034771808662, -174.2812500020484094 ) ) ;
#36461=CARTESIAN_POINT ( 'NONE',  ( -10.81189881249999907, -6.242252689847864744, -99.46875000204838102 ) ) ;
#36463=CARTESIAN_POINT ( 'NONE',  ( 5.405949406249999534, 9.363379034771803333, -106.2812500020483810 ) ) ;
#36465=CARTESIAN_POINT ( 'NONE',  ( -2.293366432827344421E-15, -12.48450537969573659, -115.7187500020483668 ) ) ;
#36468=CARTESIAN_POINT ( 'NONE',  ( -9.999999999999227285, -5.773502691896698735, -114.0000000040967478 ) ) ;
#36469=CARTESIAN_POINT ( 'NONE',  ( 5.000000000000000000, 8.660254037844385522, -129.2499999999999716 ) ) ;
#36470=CARTESIAN_POINT ( 'NONE',  ( 7.070501591499377789E-16, 11.54700538379251284, -1.624999999999959810 ) ) ;
#36474=CARTESIAN_POINT ( 'NONE',  ( -9.999999999999998224, 5.773502691896259087, -180.2500000040967905 ) ) ;
#36476=CARTESIAN_POINT ( 'NONE',  ( 7.644554776091147741E-16, 12.48450537969573659, -27.96875000204837747 ) ) ;
#36478=CARTESIAN_POINT ( 'NONE',  ( -2.293366432827344421E-15, -12.48450537969573659, -136.7187500020483810 ) ) ;
#36480=CARTESIAN_POINT ( 'NONE',  ( -5.405949406250003975, -9.363379034771801557, -35.03125000204837391 ) ) ;
#36481=CARTESIAN_POINT ( 'NONE',  ( 10.00000000000000000, 5.773502691896255534, -63.37499999999998579 ) ) ;
#36482=CARTESIAN_POINT ( 'NONE',  ( -10.81189881249999907, -6.242252689847864744, -131.1562500020483810 ) ) ;
#36487=CARTESIAN_POINT ( 'NONE',  ( 9.999999999999996447, -5.773502691896262640, -107.5000000040967763 ) ) ;
#36488=CARTESIAN_POINT ( 'NONE',  ( -10.81189881249999729, 6.242252689847871849, -66.71875000204838102 ) ) ;
#36495=CARTESIAN_POINT ( 'NONE',  ( 7.070501591499377789E-16, 11.54700538379251284, -33.50000000409675494 ) ) ;
#36496=EDGE_CURVE ( 'NONE', #35398, #17462, #32467, .T. ) ;
#36502=EDGE_LOOP ( 'NONE', ( #13916, #12603, #12444, #37981 ) ) ;
#36503=ORIENTED_EDGE ( 'NONE', *, *, #13828, .T. ) ;
#36507=EDGE_CURVE ( 'NONE', #23032, #42377, #16922, .T. ) ;
#36514=CARTESIAN_POINT ( 'NONE',  ( -10.81189881249999729, 6.242252689847871849, -122.2187500020483810 ) ) ;
#36515=CARTESIAN_POINT ( 'NONE',  ( -10.81189881249999729, 1.324075727343319199E-15, -132.7812500020483810 ) ) ;
#36517=CARTESIAN_POINT ( 'NONE',  ( 10.81189881249999729, 0.000000000000000000, -139.3437500020484094 ) ) ;
#36519=CARTESIAN_POINT ( 'NONE',  ( -9.999999999999998224, 5.773502691896259087, -155.8749999999999716 ) ) ;
#36523=CARTESIAN_POINT ( 'NONE',  ( -2.293366432827344421E-15, -12.48450537969573659, -54.21875000204837391 ) ) ;
#36525=CARTESIAN_POINT ( 'NONE',  ( 10.81189881249999907, 6.242252689847868297, -160.2187500020483810 ) ) ;
#36530=CARTESIAN_POINT ( 'NONE',  ( 10.00000000000000000, 5.773502691896255534, -91.87499999999998579 ) ) ;
#36532=CARTESIAN_POINT ( 'NONE',  ( 5.405949406249999534, 9.363379034771803333, -109.2812500020483810 ) ) ;
#36533=CARTESIAN_POINT ( 'NONE',  ( -2.121150477449813534E-15, -11.54700538379251284, -131.7500000040967905 ) ) ;
#36534=CYLINDRICAL_SURFACE ( 'NONE', #11889, 9.999999999999998224 ) ;
#36539=CARTESIAN_POINT ( 'NONE',  ( 5.405949406249999534, 9.363379034771803333, -49.28125000204838813 ) ) ;
#36545=DIRECTION ( 'NONE',  ( 0.7071067811865451302, 0.000000000000000000, 0.7071067811865500152 ) ) ;
#36557=AXIS2_PLACEMENT_3D ( 'NONE', #5502, #8743, #18651 ) ;
#36560=CARTESIAN_POINT ( 'NONE',  ( 5.405949406249999534, 9.363379034771803333, -149.5937500020483810 ) ) ;
#36561=CARTESIAN_POINT ( 'NONE',  ( 5.405949406249992428, -9.363379034771808662, -160.5937500020484094 ) ) ;
#36562=CARTESIAN_POINT ( 'NONE',  ( -4.999999999999996447, 8.660254037844387298, -106.8750000040967763 ) ) ;
#36564=CARTESIAN_POINT ( 'NONE',  ( 9.999999999999998224, 0.000000000000000000, -179.0000000000000000 ) ) ;
#36566=CARTESIAN_POINT ( 'NONE',  ( 0.000000000000000000, 0.000000000000000000, -99.99999999999998579 ) ) ;
#36568=CYLINDRICAL_SURFACE ( 'NONE', #32966, 9.999999999999998224 ) ;
#36569=CARTESIAN_POINT ( 'NONE',  ( 5.405949406249999534, 9.363379034771803333, -185.5937500020483810 ) ) ;
#36572=CARTESIAN_POINT ( 'NONE',  ( 10.81189881249999551, -6.242252689847874514, -54.15625000204837391 ) ) ;
#36574=CARTESIAN_POINT ( 'NONE',  ( 5.000000000000000000, 8.660254037844385522, -115.7499999999999858 ) ) ;
#36575=ORIENTED_EDGE ( 'NONE', *, *, #7506, .T. ) ;
#36576=CARTESIAN_POINT ( 'NONE',  ( 10.81189881249999729, 0.000000000000000000, -133.5312500020484094 ) ) ;
#36577=CARTESIAN_POINT ( 'NONE',  ( -10.81189881249999729, 1.324075727343319199E-15, -147.7812500020483810 ) ) ;
#36579=CARTESIAN_POINT ( 'NONE',  ( 10.00000000000025402, -5.773502691896113426, -125.1249999999999574 ) ) ;
#36580=CARTESIAN_POINT ( 'NONE',  ( -10.81189881249999907, -6.242252689847864744, -82.96875000204836681 ) ) ;
#36583=CARTESIAN_POINT ( 'NONE',  ( 10.81189881249999907, 6.242252689847868297, -176.7187500020483810 ) ) ;
#36585=CARTESIAN_POINT ( 'NONE',  ( -10.00000000000000000, -5.773502691896252870, -172.1250000000000284 ) ) ;
#36587=CARTESIAN_POINT ( 'NONE',  ( -5.405949406249996869, 9.363379034771805109, -76.03125000204838102 ) ) ;
#36589=CARTESIAN_POINT ( 'NONE',  ( 9.999999999999998224, 0.000000000000000000, -53.37500000409675494 ) ) ;
#36590=CARTESIAN_POINT ( 'NONE',  ( -10.81189881249999729, 6.242252689847871849, -8.218750002048357928 ) ) ;
#36591=CARTESIAN_POINT ( 'NONE',  ( -9.999999999999998224, 1.224646799147353059E-15, -133.6250000040967620 ) ) ;
#36594=CARTESIAN_POINT ( 'NONE',  ( 10.81189881249999551, -6.242252689847874514, -4.656250002048361480 ) ) ;
#36595=CARTESIAN_POINT ( 'NONE',  ( -9.999999999999998224, 1.224646799147353059E-15, -107.7499999999999858 ) ) ;
#36597=CARTESIAN_POINT ( 'NONE',  ( 9.999999999999998224, 1.224646799147353059E-15, -99.99999999999998579 ) ) ;
#36599=( BOUNDED_CURVE ( )  B_SPLINE_CURVE ( 2, ( #25584, #22126, #35301, #38738, #22338, #577, #4011 ),
 .UNSPECIFIED., .F., .F. ) 
 B_SPLINE_CURVE_WITH_KNOTS ( ( 3, 2, 2, 3 ),
 ( 0.4888059701492538101, 0.4900497512437811398, 0.4912935323383084696, 0.4919154229045888393 ),
 .UNSPECIFIED. ) 
 CURVE ( )  GEOMETRIC_REPRESENTATION_ITEM ( )  RATIONAL_B_SPLINE_CURVE ( ( 0.9999999999999940048, 0.8660254037844447028, 1.000000000000000000, 0.8660254037844387076, 1.000000000000000000, 0.9330126998438240671, 0.9330127018922194093 ) ) 
 REPRESENTATION_ITEM ( '' )  );
#36604=CARTESIAN_POINT ( 'NONE',  ( -10.81189881249999729, 6.242252689847871849, -101.2187500020483810 ) ) ;
#36611=CARTESIAN_POINT ( 'NONE',  ( 7.070501591499377789E-16, 11.54700538379251284, -42.12499999999997158 ) ) ;
#36614=ADVANCED_FACE ( 'NONE', ( #36160 ), #6593, .F. ) ;
#36617=CARTESIAN_POINT ( 'NONE',  ( 7.644554776091147741E-16, 12.48450537969573659, -145.1562500020484094 ) ) ;
#36625=CARTESIAN_POINT ( 'NONE',  ( -5.405949406249996869, 9.363379034771805109, -68.34375000204836681 ) ) ;
#36626=CARTESIAN_POINT ( 'NONE',  ( 10.81189881249999729, 0.000000000000000000, -73.53125000204838102 ) ) ;
#36628=CARTESIAN_POINT ( 'NONE',  ( 7.644554776091147741E-16, 12.48450537969573659, -161.6562500020484094 ) ) ;
#36629=CARTESIAN_POINT ( 'NONE',  ( 7.644554776091147741E-16, 12.48450537969573659, -170.6562500020484094 ) ) ;
#36630=CIRCLE ( 'NONE', #42138, 9.999999999999998224 ) ;
#36632=CARTESIAN_POINT ( 'NONE',  ( 0.000000000000000000, 0.000000000000000000, -99.99999999999998579 ) ) ;
#36634=CARTESIAN_POINT ( 'NONE',  ( -10.81189881249999729, 6.242252689847871849, -104.2187500020483810 ) ) ;
#36636=CARTESIAN_POINT ( 'NONE',  ( 10.81189881249999729, 0.000000000000000000, -7.531250002048350822 ) ) ;
#36638=CARTESIAN_POINT ( 'NONE',  ( 9.999999999999998224, 0.000000000000000000, -119.3750000040967905 ) ) ;
#36639=CARTESIAN_POINT ( 'NONE',  ( -2.293366432827344421E-15, -12.48450537969573659, -96.40625000204839523 ) ) ;
#36642=ADVANCED_FACE ( 'NONE', ( #36928 ), #17061, .F. ) ;
#36643=CARTESIAN_POINT ( 'NONE',  ( 7.070501591499377789E-16, 11.54700538379251284, -81.50000000409677625 ) ) ;
#36644=CARTESIAN_POINT ( 'NONE',  ( -9.999999999999998224, 0.000000000000000000, -99.99999999999998579 ) ) ;
#36645=CARTESIAN_POINT ( 'NONE',  ( 5.405949406249999534, 9.363379034771803333, -34.09375000204836681 ) ) ;
#36646=ORIENTED_EDGE ( 'NONE', *, *, #20111, .F. ) ;
#36648=ADVANCED_FACE ( 'NONE', ( #11018 ), #30817, .T. ) ;
#36649=CARTESIAN_POINT ( 'NONE',  ( -10.81189881249999729, 1.324075727343319199E-15, -38.28125000204838102 ) ) ;
#36652=CARTESIAN_POINT ( 'NONE',  ( 7.070501591499377789E-16, 11.54700538379251284, -12.50000000409676026 ) ) ;
#36653=ADVANCED_FACE ( 'NONE', ( #7929 ), #30388, .F. ) ;
#36668=CARTESIAN_POINT ( 'NONE',  ( 5.405949406249992428, -9.363379034771808662, -169.7812500020484094 ) ) ;
#36669=CARTESIAN_POINT ( 'NONE',  ( -9.999999999999479527, -5.773502691896549521, -147.0000000040967620 ) ) ;
#36670=ADVANCED_FACE ( 'NONE', ( #20438 ), #17189, .F. ) ;
#36672=CARTESIAN_POINT ( 'NONE',  ( -5.405949406250003975, -9.363379034771801557, -90.34375000204838102 ) ) ;
#36673=DIRECTION ( 'NONE',  ( 1.000000000000000000, 0.000000000000000000, 0.000000000000000000 ) ) ;
#36674=CARTESIAN_POINT ( 'NONE',  ( -10.81189881249999729, 6.242252689847871849, -101.4062500020483952 ) ) ;
#36676=CARTESIAN_POINT ( 'NONE',  ( 10.81189881249999729, 0.000000000000000000, -113.8437500020483810 ) ) ;
#36680=CARTESIAN_POINT ( 'NONE',  ( -4.999999999999996447, 8.660254037844387298, -132.3750000040967905 ) ) ;
#36681=CARTESIAN_POINT ( 'NONE',  ( -2.293366432827344421E-15, -12.48450537969573659, -198.4062500020484094 ) ) ;
#36684=CARTESIAN_POINT ( 'NONE',  ( -5.000000000000003553, -8.660254037844383745, -172.3750000040968189 ) ) ;
#36686=CARTESIAN_POINT ( 'NONE',  ( 10.81189881249999551, -6.242252689847874514, -19.46875000204836681 ) ) ;
#36688=CARTESIAN_POINT ( 'NONE',  ( -10.81189881249999729, 1.324075727343319199E-15, -126.5937500020483668 ) ) ;
#36690=CARTESIAN_POINT ( 'NONE',  ( 10.81189881249999551, -6.242252689847874514, -39.15625000204835970 ) ) ;
#36693=CARTESIAN_POINT ( 'NONE',  ( 7.070501591499377789E-16, 11.54700538379251284, -60.12499999999997868 ) ) ;
#36694=CARTESIAN_POINT ( 'NONE',  ( -5.405949406249996869, 9.363379034771805109, -133.0312500020484094 ) ) ;
#36697=CARTESIAN_POINT ( 'NONE',  ( -9.999999999999998224, 5.773502691896259087, -109.7500000040967763 ) ) ;
#36698=CARTESIAN_POINT ( 'NONE',  ( 9.999999999999479527, 5.773502691896553074, -101.2500000040967763 ) ) ;
#36699=CARTESIAN_POINT ( 'NONE',  ( 10.81189881249999907, 6.242252689847868297, -62.71875000204838102 ) ) ;
#36705=CARTESIAN_POINT ( 'NONE',  ( -4.999999999999996447, 8.660254037844387298, -39.37500000409676915 ) ) ;
#36708=CARTESIAN_POINT ( 'NONE',  ( -4.999999999999996447, 8.660254037844387298, -129.3750000040967905 ) ) ;
#36711=CARTESIAN_POINT ( 'NONE',  ( 9.999999999999998224, 0.000000000000000000, -155.3750000040967905 ) ) ;
#36714=CARTESIAN_POINT ( 'NONE',  ( 7.644554776091147741E-16, 12.48450537969573659, -199.1562500020484094 ) ) ;
#36718=EDGE_CURVE ( 'NONE', #17318, #11384, #7109, .T. ) ;
#36721=EDGE_CURVE ( 'NONE', #31616, #33286, #23695, .T. ) ;
#36722=CARTESIAN_POINT ( 'NONE',  ( -5.405949406250003975, -9.363379034771801557, -120.3437500020483952 ) ) ;
#36723=CARTESIAN_POINT ( 'NONE',  ( -9.999999999999998224, 5.773502691896259087, -198.2500000040968189 ) ) ;
#36724=CARTESIAN_POINT ( 'NONE',  ( 5.405949406249992428, -9.363379034771808662, -123.2812500020483952 ) ) ;
#36726=CARTESIAN_POINT ( 'NONE',  ( -2.293366432827344421E-15, -12.48450537969573659, -138.2187500020483810 ) ) ;
#36728=( BOUNDED_CURVE ( )  B_SPLINE_CURVE ( 2, ( #12514, #9917, #29152, #32188, #19210, #42496, #19003 ),
 .UNSPECIFIED., .F., .F. ) 
 B_SPLINE_CURVE_WITH_KNOTS ( ( 3, 2, 2, 3 ),
 ( 0.2798507462686568026, 0.2810945273631841879, 0.2823383084577115731, 0.2835820895522389029 ),
 .UNSPECIFIED. ) 
 CURVE ( )  GEOMETRIC_REPRESENTATION_ITEM ( )  RATIONAL_B_SPLINE_CURVE ( ( 0.9999999999999880096, 0.8660254037844506980, 1.000000000000000000, 0.8660254037844387076, 1.000000000000000000, 0.8660254037844267172, 1.000000000000011990 ) ) 
 REPRESENTATION_ITEM ( '' )  );
#36730=CARTESIAN_POINT ( 'NONE',  ( 4.999999999999992006, -8.660254037844389075, -152.2500000000000000 ) ) ;
#36735=CARTESIAN_POINT ( 'NONE',  ( 10.81189881249999551, -6.242252689847874514, -50.96875000204836681 ) ) ;
#36737=CARTESIAN_POINT ( 'NONE',  ( -10.81189881249999729, 6.242252689847871849, -159.7187500020483526 ) ) ;
#36741=CARTESIAN_POINT ( 'NONE',  ( -5.000000000000003553, -8.660254037844383745, -86.49999999999998579 ) ) ;
#36744=( BOUNDED_CURVE ( )  B_SPLINE_CURVE ( 2, ( #20930, #24617, #10998, #30664, #40770, #1092, #34112 ),
 .UNSPECIFIED., .F., .F. ) 
 B_SPLINE_CURVE_WITH_KNOTS ( ( 3, 2, 2, 3 ),
 ( 0.2350746268656717097, 0.2363184079601990950, 0.2375621890547264525, 0.2388059701492538378 ),
 .UNSPECIFIED. ) 
 CURVE ( )  GEOMETRIC_REPRESENTATION_ITEM ( )  RATIONAL_B_SPLINE_CURVE ( ( 0.9999999999999940048, 0.8660254037844447028, 1.000000000000000000, 0.8660254037844387076, 1.000000000000000000, 0.8660254037844267172, 1.000000000000011990 ) ) 
 REPRESENTATION_ITEM ( '' )  );
#36745=CARTESIAN_POINT ( 'NONE',  ( 5.405949406249992428, -9.363379034771808662, -106.7812500020483810 ) ) ;
#36746=CARTESIAN_POINT ( 'NONE',  ( -2.121150477449813534E-15, -11.54700538379251284, -133.2500000040967905 ) ) ;
#36747=CARTESIAN_POINT ( 'NONE',  ( -2.121150477449813534E-15, -11.54700538379251284, -111.8749999999999858 ) ) ;
#36749=ADVANCED_FACE ( 'NONE', ( #33623, #1246 ), #821, .F. ) ;
#36751=CARTESIAN_POINT ( 'NONE',  ( 7.644554776091147741E-16, 12.48450537969573659, -50.65625000204837391 ) ) ;
#36757=CARTESIAN_POINT ( 'NONE',  ( 10.00000000000012790, 5.773502691896179151, -174.3750000000000000 ) ) ;
#36773=CARTESIAN_POINT ( 'NONE',  ( 5.405949406249999534, 9.363379034771803333, -152.5937500020483810 ) ) ;
#36774=CARTESIAN_POINT ( 'NONE',  ( -10.81189881249999729, -6.242252689847864744, -159.4687500020484094 ) ) ;
#36778=CARTESIAN_POINT ( 'NONE',  ( -9.999999999999998224, 5.773502691896259087, -176.8750000000000000 ) ) ;
#36781=CARTESIAN_POINT ( 'NONE',  ( 7.070501591499376803E-16, 11.54700538379251284, -138.1250000000000000 ) ) ;
#36784=CARTESIAN_POINT ( 'NONE',  ( -10.81189881249999729, 1.324075727343319199E-15, -185.0937500020483810 ) ) ;
#36787=CARTESIAN_POINT ( 'NONE',  ( -10.81189881249999729, 6.242252689847871849, -53.40625000204837391 ) ) ;
#36789=CARTESIAN_POINT ( 'NONE',  ( -10.00000000000000000, -5.773502691896251982, -107.6249999999999858 ) ) ;
#36790=VERTEX_POINT ( 'NONE', #38547 ) ;
#36791=CARTESIAN_POINT ( 'NONE',  ( -10.81189881249999729, 1.324075727343319199E-15, -131.2812500020483810 ) ) ;
#36792=CARTESIAN_POINT ( 'NONE',  ( -5.405949406249996869, 9.363379034771805109, -148.0312500020483810 ) ) ;
#36794=CARTESIAN_POINT ( 'NONE',  ( 5.405949406249999534, 9.363379034771803333, -79.09375000204838102 ) ) ;
#36797=CARTESIAN_POINT ( 'NONE',  ( 10.81189881249999729, 0.000000000000000000, -182.8437500020483810 ) ) ;
#36799=CARTESIAN_POINT ( 'NONE',  ( -9.999999999999998224, 1.224646799147353059E-15, -172.2500000000000000 ) ) ;
#36800=FACE_OUTER_BOUND ( 'NONE', #8121, .T. ) ;
#36801=CARTESIAN_POINT ( 'NONE',  ( -5.405949406249996869, 9.363379034771805109, -79.03125000204838102 ) ) ;
#36804=CARTESIAN_POINT ( 'NONE',  ( 10.00000000000000000, 5.773502691896255534, -54.75000000409676915 ) ) ;
#36805=CARTESIAN_POINT ( 'NONE',  ( -10.81189881249999729, 6.242252689847871849, -6.718750002048357040 ) ) ;
#36808=CARTESIAN_POINT ( 'NONE',  ( -10.81189881249999729, 1.324075727343319199E-15, -3.781250002048375247 ) ) ;
#36813=CARTESIAN_POINT ( 'NONE',  ( 9.999999999999998224, 0.000000000000000000, -177.8750000040967905 ) ) ;
#36824=CARTESIAN_POINT ( 'NONE',  ( 9.999999999999998224, 0.000000000000000000, -46.99999999999998579 ) ) ;
#36833=CARTESIAN_POINT ( 'NONE',  ( 9.999999999999998224, 0.000000000000000000, -141.5000000000000000 ) ) ;
#36836=CARTESIAN_POINT ( 'NONE',  ( 10.81189881249999729, 0.000000000000000000, -68.84375000204836681 ) ) ;
#36837=CARTESIAN_POINT ( 'NONE',  ( 10.81189881249999907, 6.242252689847868297, -73.40625000204836681 ) ) ;
#36839=CARTESIAN_POINT ( 'NONE',  ( -5.405949406249996869, 9.363379034771805109, -155.5312500020484094 ) ) ;
#36840=CARTESIAN_POINT ( 'NONE',  ( -2.293366432827344421E-15, -12.48450537969573659, -169.9062500020483810 ) ) ;
#36843=CARTESIAN_POINT ( 'NONE',  ( 10.81189881249999907, 6.242252689847868297, -1.218750002048352155 ) ) ;
#36845=CARTESIAN_POINT ( 'NONE',  ( 10.81189881249999907, 6.242252689847868297, -103.2187500020483810 ) ) ;
#36848=CARTESIAN_POINT ( 'NONE',  ( 10.81189881249999551, -6.242252689847874514, -1.656250002048359482 ) ) ;
#36851=CARTESIAN_POINT ( 'NONE',  ( -10.81189881249999729, 1.324075727343319199E-15, -101.2812500020483952 ) ) ;
#36854=CARTESIAN_POINT ( 'NONE',  ( -2.121150477449813534E-15, -11.54700538379251284, -73.25000000409674783 ) ) ;
#36856=CARTESIAN_POINT ( 'NONE',  ( 5.405949406249992428, -9.363379034771808662, -33.09375000204836681 ) ) ;
#36859=CARTESIAN_POINT ( 'NONE',  ( 5.405949406249992428, -9.363379034771808662, -28.78125000204837036 ) ) ;
#36862=CARTESIAN_POINT ( 'NONE',  ( 10.00000000000000000, 5.773502691896255534, -3.750000004096754047 ) ) ;
#36863=EDGE_CURVE ( 'NONE', #33393, #36337, #21722, .T. ) ;
#36879=CARTESIAN_POINT ( 'NONE',  ( 10.81189881249999551, -6.242252689847874514, -174.1562500020484094 ) ) ;
#36882=CARTESIAN_POINT ( 'NONE',  ( -10.81189881249999729, 6.242252689847871849, -92.21875000204838102 ) ) ;
#36883=CARTESIAN_POINT ( 'NONE',  ( -10.81189881249999907, -6.242252689847864744, -198.4687500020484379 ) ) ;
#36884=CARTESIAN_POINT ( 'NONE',  ( 5.405949406249999534, 9.363379034771803333, -101.7812500020483952 ) ) ;
#36886=CARTESIAN_POINT ( 'NONE',  ( 7.644554776091147741E-16, 12.48450537969573659, -104.4687500020483668 ) ) ;
#36888=ADVANCED_FACE ( 'NONE', ( #5115 ), #41348, .F. ) ;
#36892=CARTESIAN_POINT ( 'NONE',  ( 7.644554776091147741E-16, 12.48450537969573659, -193.1562500020484094 ) ) ;
#36895=CARTESIAN_POINT ( 'NONE',  ( 10.00000000000000000, 5.773502691896255534, -168.7500000040967905 ) ) ;
#36897=CARTESIAN_POINT ( 'NONE',  ( -10.81189881249999729, 1.324075727343319199E-15, -21.59375000204835615 ) ) ;
#36899=CARTESIAN_POINT ( 'NONE',  ( 5.405949406249999534, 9.363379034771803333, -133.0937500020483810 ) ) ;
#36901=CARTESIAN_POINT ( 'NONE',  ( -10.81189881249999907, -6.242252689847864744, -24.65625000204838102 ) ) ;
#36903=CARTESIAN_POINT ( 'NONE',  ( -4.999999999999996447, 8.660254037844387298, -62.99999999999997158 ) ) ;
#36904=CARTESIAN_POINT ( 'NONE',  ( 10.81189881249999551, -6.242252689847874514, -123.1562500020483952 ) ) ;
#36908=CARTESIAN_POINT ( 'NONE',  ( -9.999999999999998224, 5.773502691896259087, -96.25000000409677625 ) ) ;
#36910=CARTESIAN_POINT ( 'NONE',  ( 10.81189881249999729, 0.000000000000000000, -55.34375000204835970 ) ) ;
#36911=VERTEX_POINT ( 'NONE', #4903 ) ;
#36915=DIRECTION ( 'NONE',  ( -0.000000000000000000, -0.000000000000000000, -1.000000000000000000 ) ) ;
#36916=CARTESIAN_POINT ( 'NONE',  ( -2.121150477449813534E-15, -11.54700538379251284, -37.25000000409675494 ) ) ;
#36922=LINE ( 'NONE', #37353, #12124 ) ;
#36923=VERTEX_POINT ( 'NONE', #22157 ) ;
#36928=FACE_OUTER_BOUND ( 'NONE', #29031, .T. ) ;
#36935=CARTESIAN_POINT ( 'NONE',  ( 7.644554776091147741E-16, 12.48450537969573659, -119.4687500020483952 ) ) ;
#36936=CARTESIAN_POINT ( 'NONE',  ( 9.999999999999996447, -5.773502691896262640, -197.5000000040968189 ) ) ;
#36938=CARTESIAN_POINT ( 'NONE',  ( -10.81189881249999729, 1.324075727343319199E-15, -122.2812500020483952 ) ) ;
#36940=CARTESIAN_POINT ( 'NONE',  ( 5.405949406249999534, 9.363379034771803333, -136.0937500020483810 ) ) ;
#36941=CARTESIAN_POINT ( 'NONE',  ( -4.999999999999996447, 8.660254037844387298, -163.5000000000000000 ) ) ;
#36943=CARTESIAN_POINT ( 'NONE',  ( 9.999999999999998224, 0.000000000000000000, -156.5000000000000000 ) ) ;
#36944=CARTESIAN_POINT ( 'NONE',  ( 4.999999999999992006, -8.660254037844389075, -18.74999999999996092 ) ) ;
#36947=CARTESIAN_POINT ( 'NONE',  ( 10.00000000000012257, -5.773502691896187144, -170.1250000000000000 ) ) ;
#36949=CARTESIAN_POINT ( 'NONE',  ( -10.81189881249999729, 6.242252689847871849, -45.71875000204836681 ) ) ;
#36950=CARTESIAN_POINT ( 'NONE',  ( 4.999999999999992006, -8.660254037844389075, -110.6250000040967763 ) ) ;
#36951=CARTESIAN_POINT ( 'NONE',  ( 10.81189881249999729, 0.000000000000000000, -155.8437500020483810 ) ) ;
#36954=CARTESIAN_POINT ( 'NONE',  ( 0.2237483581476167049, 10.23237876573678307, -180.0000000000000000 ) ) ;
#36955=CARTESIAN_POINT ( 'NONE',  ( 5.000000000000000000, 8.660254037844385522, -82.74999999999997158 ) ) ;
#36958=CARTESIAN_POINT ( 'NONE',  ( -10.81189881249999729, 1.324075727343319199E-15, -110.2812500020483810 ) ) ;
#36959=CARTESIAN_POINT ( 'NONE',  ( 5.000000000000000000, 8.660254037844385522, -131.1250000040967620 ) ) ;
#36962=DIRECTION ( 'NONE',  ( -0.000000000000000000, -0.000000000000000000, -1.000000000000000000 ) ) ;
#36963=CARTESIAN_POINT ( 'NONE',  ( -5.405949406250003975, -9.363379034771801557, -50.03125000204838813 ) ) ;
#36975=ORIENTED_EDGE ( 'NONE', *, *, #41196, .T. ) ;
#36987=CARTESIAN_POINT ( 'NONE',  ( -10.81189881249999729, 1.324075727343319199E-15, -138.5937500020483810 ) ) ;
#36988=CARTESIAN_POINT ( 'NONE',  ( 10.81189881249999729, 6.242252689847867408, -158.7187500020484094 ) ) ;
#36992=CARTESIAN_POINT ( 'NONE',  ( 10.00000000000000000, 5.773502691896255534, -180.3750000000000284 ) ) ;
#36996=CARTESIAN_POINT ( 'NONE',  ( -9.999999999999998224, 1.224646799147353059E-15, -124.6250000040967763 ) ) ;
#36997=CARTESIAN_POINT ( 'NONE',  ( -2.293366432827344421E-15, -12.48450537969573659, -180.2187500020484094 ) ) ;
#37000=CARTESIAN_POINT ( 'NONE',  ( 10.81189881249999907, 6.242252689847868297, -49.40625000204837391 ) ) ;
#37002=CARTESIAN_POINT ( 'NONE',  ( 10.00000000000000000, 5.773502691896255534, -111.3749999999999858 ) ) ;
#37004=CARTESIAN_POINT ( 'NONE',  ( -10.81189881249999729, -6.242252689847864744, -132.6562500020483810 ) ) ;
#37005=CARTESIAN_POINT ( 'NONE',  ( 9.999999999999996447, -5.773502691896262640, -155.5000000040968189 ) ) ;
#37006=CARTESIAN_POINT ( 'NONE',  ( 7.644554776091147741E-16, 12.48450537969573659, -151.1562500020484094 ) ) ;
#37008=CARTESIAN_POINT ( 'NONE',  ( 10.81189881249999907, 6.242252689847868297, -85.21875000204836681 ) ) ;
#37011=CARTESIAN_POINT ( 'NONE',  ( 10.81189881249999729, 0.000000000000000000, -181.3437500020483810 ) ) ;
#37014=CARTESIAN_POINT ( 'NONE',  ( -9.999999999999998224, 1.224646799147353059E-15, -133.2499999999999716 ) ) ;
#37015=CARTESIAN_POINT ( 'NONE',  ( 10.81189881249999907, 6.242252689847868297, -77.90625000204836681 ) ) ;
#37017=CARTESIAN_POINT ( 'NONE',  ( -9.999999999999998224, 1.224646799147353059E-15, -52.62500000409675494 ) ) ;
#37018=CARTESIAN_POINT ( 'NONE',  ( 5.405949406249999534, 9.363379034771803333, -7.093750002048371250 ) ) ;
#37021=CARTESIAN_POINT ( 'NONE',  ( 10.81189881249999907, 6.242252689847868297, -4.406250002048361480 ) ) ;
#37023=CARTESIAN_POINT ( 'NONE',  ( -9.999999999999998224, 1.224646799147353059E-15, -161.7500000000000000 ) ) ;
#37039=CARTESIAN_POINT ( 'NONE',  ( -9.999999999999998224, 1.224646799147353059E-15, -122.7500000000000000 ) ) ;
#37040=CARTESIAN_POINT ( 'NONE',  ( 9.999999999999996447, -5.773502691896262640, -45.62499999999996447 ) ) ;
#37042=CARTESIAN_POINT ( 'NONE',  ( -5.405949406250003975, -9.363379034771801557, -165.3437500020484094 ) ) ;
#37045=CARTESIAN_POINT ( 'NONE',  ( 7.070501591499376803E-16, 11.54700538379251284, -147.1250000000000000 ) ) ;
#37046=CARTESIAN_POINT ( 'NONE',  ( -4.999999999999996447, 8.660254037844387298, -126.0000000000000000 ) ) ;
#37049=CARTESIAN_POINT ( 'NONE',  ( 9.999999999999998224, 0.000000000000000000, -161.3750000040967905 ) ) ;
#37052=CARTESIAN_POINT ( 'NONE',  ( 10.81189881249999551, -6.242252689847874514, -65.96875000204838102 ) ) ;
#37053=CARTESIAN_POINT ( 'NONE',  ( 5.405949406249999534, 9.363379034771803333, -76.28125000204838102 ) ) ;
#37055=CARTESIAN_POINT ( 'NONE',  ( 10.81189881249999729, 6.242252689847867408, -157.4062500020483810 ) ) ;
#37056=CARTESIAN_POINT ( 'NONE',  ( -10.81189881249999729, 6.242252689847871849, -168.9062500020483810 ) ) ;
#37057=CARTESIAN_POINT ( 'NONE',  ( 9.999999999999998224, 0.000000000000000000, -144.8750000040967905 ) ) ;
#37058=CARTESIAN_POINT ( 'NONE',  ( -5.405949406250003975, -9.363379034771801557, -102.3437500020483810 ) ) ;
#37061=CARTESIAN_POINT ( 'NONE',  ( -10.81189881249999729, 1.324075727343319199E-15, -5.281250002048376579 ) ) ;
#37064=CARTESIAN_POINT ( 'NONE',  ( 5.405949406249992428, -9.363379034771808662, -100.7812500020483952 ) ) ;
#37066=CARTESIAN_POINT ( 'NONE',  ( -2.121150477449813534E-15, -11.54700538379251284, -74.75000000409677625 ) ) ;
#37068=CARTESIAN_POINT ( 'NONE',  ( -10.81189881249999729, 6.242252689847871849, -36.71875000204835260 ) ) ;
#37069=VERTEX_POINT ( 'NONE', #20630 ) ;
#37071=CARTESIAN_POINT ( 'NONE',  ( -5.405949406249996869, 9.363379034771805109, -29.53125000204837036 ) ) ;
#37074=CARTESIAN_POINT ( 'NONE',  ( -9.999999999999998224, 5.773502691896259087, -3.250000004096753603 ) ) ;
#37078=VERTEX_POINT ( 'NONE', #12708 ) ;
#37080=VECTOR ( 'NONE', #3495, 1000.000000000000000 ) ;
#37090=CARTESIAN_POINT ( 'NONE',  ( 10.81189881249999907, 6.242252689847868297, -170.9062500020484094 ) ) ;
#37093=CARTESIAN_POINT ( 'NONE',  ( 10.81189881249999729, 0.000000000000000000, -91.34375000204838102 ) ) ;
#37095=CARTESIAN_POINT ( 'NONE',  ( 7.644554776091147741E-16, 12.48450537969573659, -103.1562500020483952 ) ) ;
#37097=CARTESIAN_POINT ( 'NONE',  ( -10.81189881249999729, -6.242252689847864744, -108.4687500020483810 ) ) ;
#37101=CARTESIAN_POINT ( 'NONE',  ( -5.405949406250003975, -9.363379034771801557, -198.5312500020484094 ) ) ;
#37104=CARTESIAN_POINT ( 'NONE',  ( -5.000000000000003553, -8.660254037844383745, -170.8750000040968189 ) ) ;
#37106=CARTESIAN_POINT ( 'NONE',  ( 5.405949406249992428, -9.363379034771808662, -18.09375000204835260 ) ) ;
#37107=CARTESIAN_POINT ( 'NONE',  ( 0.000000000000000000, 0.000000000000000000, -99.99999999999998579 ) ) ;
#37108=CARTESIAN_POINT ( 'NONE',  ( -2.293366432827344421E-15, -12.48450537969573659, -129.2187500020483810 ) ) ;
#37110=CARTESIAN_POINT ( 'NONE',  ( 10.81189881249999551, -6.242252689847874514, -28.65625000204838102 ) ) ;
#37113=CARTESIAN_POINT ( 'NONE',  ( -2.121150477449813534E-15, -11.54700538379251284, -60.87499999999998579 ) ) ;
#37114=CARTESIAN_POINT ( 'NONE',  ( 5.405949406249999534, 9.363379034771803333, -125.7812500020483668 ) ) ;
#37118=CARTESIAN_POINT ( 'NONE',  ( -9.999999999999998224, 1.224646799147353059E-15, -97.62500000409677625 ) ) ;
#37120=CARTESIAN_POINT ( 'NONE',  ( -5.405949406250003975, -9.363379034771801557, -61.84375000204836681 ) ) ;
#37125=CARTESIAN_POINT ( 'NONE',  ( -10.00000000000000000, -5.773502691896251982, -28.50000000409674783 ) ) ;
#37127=CARTESIAN_POINT ( 'NONE',  ( 9.999999999999998224, 0.000000000000000000, -146.3750000040967905 ) ) ;
#37132=DIRECTION ( 'NONE',  ( -0.000000000000000000, -0.000000000000000000, -1.000000000000000000 ) ) ;
#37135=CARTESIAN_POINT ( 'NONE',  ( 10.81189881249999729, 0.000000000000000000, -196.5312500020484094 ) ) ;
#37141=CARTESIAN_POINT ( 'NONE',  ( 7.644554776091147741E-16, 12.48450537969573659, -120.9687500020483952 ) ) ;
#37142=CARTESIAN_POINT ( 'NONE',  ( -9.999999999999998224, 5.773502691896259087, -196.7500000040968189 ) ) ;
#37143=CARTESIAN_POINT ( 'NONE',  ( 5.405949406249999534, 9.363379034771803333, -121.2812500020483952 ) ) ;
#37145=CARTESIAN_POINT ( 'NONE',  ( -10.81189881249999729, 1.324075727343319199E-15, -131.0937500020483810 ) ) ;
#37147=CARTESIAN_POINT ( 'NONE',  ( 9.999999999999998224, 0.000000000000000000, -164.0000000000000000 ) ) ;
#37150=CARTESIAN_POINT ( 'NONE',  ( -9.999999999999998224, 1.224646799147353059E-15, -157.2500000000000000 ) ) ;
#37151=CARTESIAN_POINT ( 'NONE',  ( 7.070501591499377789E-16, 11.54700538379251284, -18.12499999999997513 ) ) ;
#37155=CARTESIAN_POINT ( 'NONE',  ( -10.81189881249999907, -6.242252689847864744, -42.46875000204835970 ) ) ;
#37157=CARTESIAN_POINT ( 'NONE',  ( 5.405949406249992428, -9.363379034771808662, -151.5937500020483810 ) ) ;
#37161=CARTESIAN_POINT ( 'NONE',  ( -5.000000000000003553, -8.660254037844383745, -80.49999999999998579 ) ) ;
#37163=ORIENTED_EDGE ( 'NONE', *, *, #3272, .T. ) ;
#37164=CARTESIAN_POINT ( 'NONE',  ( 10.81189881249999729, 0.000000000000000000, -108.0312500020483810 ) ) ;
#37165=CARTESIAN_POINT ( 'NONE',  ( -5.000000000000003553, -8.660254037844383745, -127.3750000040967905 ) ) ;
#37166=FACE_OUTER_BOUND ( 'NONE', #35512, .T. ) ;
#37168=CYLINDRICAL_SURFACE ( 'NONE', #4216, 9.999999999999998224 ) ;
#37169=CARTESIAN_POINT ( 'NONE',  ( 7.644554776091147741E-16, 12.48450537969573659, -53.65625000204838102 ) ) ;
#37174=CARTESIAN_POINT ( 'NONE',  ( 9.999999999999998224, 0.000000000000000000, -120.8750000040967905 ) ) ;
#37176=CARTESIAN_POINT ( 'NONE',  ( -10.00000000000012434, 5.773502691896184480, -163.7500000040967905 ) ) ;
#37179=ORIENTED_EDGE ( 'NONE', *, *, #33285, .F. ) ;
#37182=( BOUNDED_CURVE ( )  B_SPLINE_CURVE ( 2, ( #37615, #20560, #13858, #14718, #24038, #21420, #27692 ),
 .UNSPECIFIED., .F., .F. ) 
 B_SPLINE_CURVE_WITH_KNOTS ( ( 3, 2, 2, 3 ),
 ( 0.1119402985074627876, 0.1131840796019901035, 0.1144278606965174333, 0.1156716417910447492 ),
 .UNSPECIFIED. ) 
 CURVE ( )  GEOMETRIC_REPRESENTATION_ITEM ( )  RATIONAL_B_SPLINE_CURVE ( ( 0.9999999999999894529, 0.8660254037844491437, 1.000000000000000000, 0.8660254037844387076, 1.000000000000000000, 0.8660254037844417052, 0.9999999999999970024 ) ) 
 REPRESENTATION_ITEM ( '' )  );
#37191=CARTESIAN_POINT ( 'NONE',  ( 5.405949406249999534, 9.363379034771803333, -140.5937500020483810 ) ) ;
#37192=CARTESIAN_POINT ( 'NONE',  ( -5.405949406249996869, 9.363379034771805109, -156.8437500020483810 ) ) ;
#37194=CARTESIAN_POINT ( 'NONE',  ( -9.999999999999998224, 1.224646799147353059E-15, -139.6250000040967905 ) ) ;
#37195=CARTESIAN_POINT ( 'NONE',  ( -9.999999999999998224, 5.773502691896259087, -182.8750000000000000 ) ) ;
#37198=CARTESIAN_POINT ( 'NONE',  ( -4.208742559982952436, 9.984557306008309041, -99.99999999999995737 ) ) ;
#37201=EDGE_CURVE ( 'NONE', #22477, #34879, #7269, .T. ) ;
#37202=CARTESIAN_POINT ( 'NONE',  ( -10.81189881249999729, 6.242252689847871849, -179.2187500020483810 ) ) ;
#37206=CARTESIAN_POINT ( 'NONE',  ( 5.405949406249999534, 9.363379034771803333, -52.28125000204835970 ) ) ;
#37208=CARTESIAN_POINT ( 'NONE',  ( -2.121150477449813534E-15, -11.54700538379251284, -104.3749999999999716 ) ) ;
#37210=CARTESIAN_POINT ( 'NONE',  ( -5.405949406249996869, 9.363379034771805109, -136.0312500020484094 ) ) ;
#37211=CARTESIAN_POINT ( 'NONE',  ( -10.00000000000000000, -5.773502691896251982, -145.5000000040967905 ) ) ;
#37212=CARTESIAN_POINT ( 'NONE',  ( 7.644554776091147741E-16, 12.48450537969573659, -146.6562500020484379 ) ) ;
#37216=CARTESIAN_POINT ( 'NONE',  ( 10.81189881249999551, -6.242252689847874514, -184.4687500020483810 ) ) ;
#37220=CARTESIAN_POINT ( 'NONE',  ( -10.81189881249999907, -6.242252689847864744, -78.65625000204839523 ) ) ;
#37222=CARTESIAN_POINT ( 'NONE',  ( -10.00000000000000000, -5.773502691896251982, -51.00000000409676915 ) ) ;
#37223=CARTESIAN_POINT ( 'NONE',  ( -2.293366432827344421E-15, -12.48450537969573659, -12.21875000204836148 ) ) ;
#37226=CARTESIAN_POINT ( 'NONE',  ( -5.405949406250003975, -9.363379034771801557, -8.031250002048350822 ) ) ;
#37231=( BOUNDED_CURVE ( )  B_SPLINE_CURVE ( 2, ( #28441, #41577, #42626, #19330, #22798, #35549, #32315 ),
 .UNSPECIFIED., .F., .F. ) 
 B_SPLINE_CURVE_WITH_KNOTS ( ( 3, 2, 2, 3 ),
 ( 0.3768656716417911334, 0.3781094527363185187, 0.3793532338308459040, 0.3805970149253732338 ),
 .UNSPECIFIED. ) 
 CURVE ( )  GEOMETRIC_REPRESENTATION_ITEM ( )  RATIONAL_B_SPLINE_CURVE ( ( 0.9999999999999880096, 0.8660254037844506980, 1.000000000000000000, 0.8660254037844387076, 1.000000000000000000, 0.8660254037844267172, 1.000000000000011990 ) ) 
 REPRESENTATION_ITEM ( '' )  );
#37236=CARTESIAN_POINT ( 'NONE',  ( -9.999999999999998224, 1.224646799147353059E-15, -123.1250000040967905 ) ) ;
#37245=CARTESIAN_POINT ( 'NONE',  ( 10.00000000000000000, 5.773502691896255534, -48.37499999999997158 ) ) ;
#37247=CARTESIAN_POINT ( 'NONE',  ( 7.644554776091147741E-16, 12.48450537969573659, -168.9687500020483810 ) ) ;
#37248=CARTESIAN_POINT ( 'NONE',  ( -10.81189881249999729, 6.242252689847871849, -176.2187500020483810 ) ) ;
#37250=CARTESIAN_POINT ( 'NONE',  ( -10.00000000000000000, -5.773502691896252870, -168.0000000040968189 ) ) ;
#37251=CARTESIAN_POINT ( 'NONE',  ( 7.070501591499377789E-16, 11.54700538379251284, -199.6250000000000000 ) ) ;
#37257=ADVANCED_FACE ( 'NONE', ( #22663 ), #6269, .F. ) ;
#37258=CARTESIAN_POINT ( 'NONE',  ( 10.81189881249999729, 0.000000000000000000, -73.34375000204838102 ) ) ;
#37260=CARTESIAN_POINT ( 'NONE',  ( 10.81189881249999907, 6.242252689847868297, -79.40625000204839523 ) ) ;
#37262=CARTESIAN_POINT ( 'NONE',  ( -9.999999999999998224, 5.773502691896259087, -134.8750000000000000 ) ) ;
#37264=CARTESIAN_POINT ( 'NONE',  ( -10.81189881249999729, 1.324075727343319199E-15, -155.2812500020484094 ) ) ;
#37265=CARTESIAN_POINT ( 'NONE',  ( 10.81189881249999551, -6.242252689847874514, -171.1562500020484094 ) ) ;
#37269=CARTESIAN_POINT ( 'NONE',  ( -10.81189881249999729, 1.324075727343319199E-15, -105.5937500020483810 ) ) ;
#37270=CARTESIAN_POINT ( 'NONE',  ( -4.999999999999996447, 8.660254037844387298, -156.0000000000000000 ) ) ;
#37272=CARTESIAN_POINT ( 'NONE',  ( 5.405949406249992428, -9.363379034771808662, -1.781250002048373471 ) ) ;
#37276=CARTESIAN_POINT ( 'NONE',  ( -10.81189881249999907, -6.242252689847864744, -102.6562500020483952 ) ) ;
#37278=CARTESIAN_POINT ( 'NONE',  ( -9.999999999999998224, 5.773502691896259087, -72.25000000409676204 ) ) ;
#37280=CARTESIAN_POINT ( 'NONE',  ( 5.405949406249999534, 9.363379034771803333, -35.59375000204836681 ) ) ;
#37283=CARTESIAN_POINT ( 'NONE',  ( -10.81189881249999729, 6.242252689847871849, -30.90625000204835615 ) ) ;
#37287=CARTESIAN_POINT ( 'NONE',  ( 9.999999999999998224, 0.000000000000000000, -2.375000004096766482 ) ) ;
#37289=EDGE_CURVE ( 'NONE', #35300, #5570, #13131, .T. ) ;
#37296=EDGE_LOOP ( 'NONE', ( #39361, #4874, #21963, #11812 ) ) ;
#37297=ORIENTED_EDGE ( 'NONE', *, *, #16335, .T. ) ;
#37306=CARTESIAN_POINT ( 'NONE',  ( 5.000000000000000000, 8.660254037844385522, -156.6250000040967905 ) ) ;
#37307=CARTESIAN_POINT ( 'NONE',  ( -10.81189881249999907, -6.242252689847864744, -173.1562500020484094 ) ) ;
#37312=CARTESIAN_POINT ( 'NONE',  ( 7.644554776091147741E-16, 12.48450537969573659, -93.96875000204838102 ) ) ;
#37315=CARTESIAN_POINT ( 'NONE',  ( 10.81189881249999729, 0.000000000000000000, -97.53125000204839523 ) ) ;
#37317=CARTESIAN_POINT ( 'NONE',  ( 10.81189881249999729, 0.000000000000000000, -106.3437500020483810 ) ) ;
#37321=CARTESIAN_POINT ( 'NONE',  ( 10.00000000000000000, 5.773502691896255534, -0.3749999999999586997 ) ) ;
#37324=CARTESIAN_POINT ( 'NONE',  ( -9.999999999999998224, 1.224646799147353059E-15, -174.1250000040968189 ) ) ;
#37326=CARTESIAN_POINT ( 'NONE',  ( -10.81189881249999729, 6.242252689847871849, -23.21875000204837036 ) ) ;
#37328=CARTESIAN_POINT ( 'NONE',  ( -5.405949406249996869, 9.363379034771805109, -128.3437500020484094 ) ) ;
#37330=CARTESIAN_POINT ( 'NONE',  ( -5.405949406249996869, 9.363379034771805109, -28.03125000204837036 ) ) ;
#37332=CARTESIAN_POINT ( 'NONE',  ( -4.999999999999996447, 8.660254037844387298, -157.8750000040967905 ) ) ;
#37333=CARTESIAN_POINT ( 'NONE',  ( -5.000000000000003553, -8.660254037844383745, -59.49999999999997158 ) ) ;
#37334=CARTESIAN_POINT ( 'NONE',  ( -10.81189881249999907, -6.242252689847864744, -125.1562500020483810 ) ) ;
#37336=ORIENTED_EDGE ( 'NONE', *, *, #22114, .F. ) ;
#37338=DIRECTION ( 'NONE',  ( -0.000000000000000000, -0.000000000000000000, -1.000000000000000000 ) ) ;
#37339=CARTESIAN_POINT ( 'NONE',  ( 7.070501591499377789E-16, 11.54700538379251284, -99.50000000409677625 ) ) ;
#37342=CARTESIAN_POINT ( 'NONE',  ( -2.293366432827344421E-15, -12.48450537969573659, -58.71875000204837391 ) ) ;
#37348=DIRECTION ( 'NONE',  ( -1.000000000000000000, 0.000000000000000000, 0.000000000000000000 ) ) ;
#37349=CARTESIAN_POINT ( 'NONE',  ( 10.00000000000000000, 5.773502691896255534, -26.25000000409677270 ) ) ;
#37350=AXIS2_PLACEMENT_3D ( 'NONE', #14880, #28075, #11644 ) ;
#37353=CARTESIAN_POINT ( 'NONE',  ( -9.999999999999998224, 0.000000000000000000, -99.99999999999998579 ) ) ;
#37354=ORIENTED_EDGE ( 'NONE', *, *, #41980, .F. ) ;
#37362=CARTESIAN_POINT ( 'NONE',  ( -2.293366432827344421E-15, -12.48450537969573659, -196.9062500020484094 ) ) ;
#37364=CARTESIAN_POINT ( 'NONE',  ( -4.999999999999996447, 8.660254037844387298, -150.0000000000000000 ) ) ;
#37368=CARTESIAN_POINT ( 'NONE',  ( -2.293366432827344421E-15, -12.48450537969573659, -115.7187500020483952 ) ) ;
#37369=CARTESIAN_POINT ( 'NONE',  ( 10.81189881249999907, 6.242252689847868297, 0.2812499979516491777 ) ) ;
#37370=CARTESIAN_POINT ( 'NONE',  ( 7.644554776091147741E-16, 12.48450537969573659, -127.1562500020483952 ) ) ;
#37372=CARTESIAN_POINT ( 'NONE',  ( 5.405949406249992428, -9.363379034771808662, -129.0937500020483810 ) ) ;
#37374=CARTESIAN_POINT ( 'NONE',  ( -4.999999999999996447, 8.660254037844387298, -109.8750000040967763 ) ) ;
#37375=CARTESIAN_POINT ( 'NONE',  ( 5.000000000000000000, 8.660254037844385522, -156.2500000000000000 ) ) ;
#37376=CARTESIAN_POINT ( 'NONE',  ( -5.000000000000003553, -8.660254037844383745, -17.49999999999996092 ) ) ;
#37380=CARTESIAN_POINT ( 'NONE',  ( 9.999999999999998224, 0.000000000000000000, -158.3750000040967905 ) ) ;
#37382=CARTESIAN_POINT ( 'NONE',  ( 10.81189881249999907, 6.242252689847868297, -46.21875000204837391 ) ) ;
#37383=CARTESIAN_POINT ( 'NONE',  ( -5.000000000000003553, -8.660254037844383745, -110.8750000040967763 ) ) ;
#37384=CARTESIAN_POINT ( 'NONE',  ( -10.81189881249999907, -6.242252689847864744, -150.4687500020484094 ) ) ;
#37388=CARTESIAN_POINT ( 'NONE',  ( 4.999999999999992006, -8.660254037844389075, -80.24999999999998579 ) ) ;
#37391=CARTESIAN_POINT ( 'NONE',  ( 5.405949406249992428, -9.363379034771808662, -105.2812500020483810 ) ) ;
#37392=CARTESIAN_POINT ( 'NONE',  ( 10.00000000000000000, 5.773502691896255534, -126.7500000040967905 ) ) ;
#37393=CARTESIAN_POINT ( 'NONE',  ( -2.121150477449813534E-15, -11.54700538379251284, -154.2500000040968189 ) ) ;
#37394=EDGE_CURVE ( 'NONE', #17641, #32014, #5476, .T. ) ;
#37397=CARTESIAN_POINT ( 'NONE',  ( -10.81189881249999729, 1.324075727343319199E-15, -44.28125000204838102 ) ) ;
#37405=EDGE_CURVE ( 'NONE', #10629, #21806, #22819, .T. ) ;
#37412=CARTESIAN_POINT ( 'NONE',  ( 9.999999999999742428, 5.773502691896404748, -153.7500000040967620 ) ) ;
#37417=CARTESIAN_POINT ( 'NONE',  ( -5.405949406249996869, 9.363379034771805109, -141.8437500020483810 ) ) ;
#37418=CARTESIAN_POINT ( 'NONE',  ( -2.293366432827344421E-15, -12.48450537969573659, -145.9062500020484094 ) ) ;
#37419=CARTESIAN_POINT ( 'NONE',  ( 10.81189881249999551, -6.242252689847874514, -152.9687500020484094 ) ) ;
#37421=CARTESIAN_POINT ( 'NONE',  ( 7.070501591499377789E-16, 11.54700538379251284, -180.1250000000000000 ) ) ;
#37426=CARTESIAN_POINT ( 'NONE',  ( -2.293366432827344421E-15, -12.48450537969573659, -181.7187500020484094 ) ) ;
#37430=CARTESIAN_POINT ( 'NONE',  ( 10.81189881249999907, 6.242252689847868297, -44.90625000204836681 ) ) ;
#37432=CARTESIAN_POINT ( 'NONE',  ( 7.070501591499377789E-16, 11.54700538379251284, -105.1249999999999858 ) ) ;
#37435=CARTESIAN_POINT ( 'NONE',  ( -10.81189881249999729, -6.242252689847864744, -129.6562500020483810 ) ) ;
#37436=CARTESIAN_POINT ( 'NONE',  ( 7.070501591499377789E-16, 11.54700538379251284, -150.5000000040968189 ) ) ;
#37438=ORIENTED_EDGE ( 'NONE', *, *, #25324, .F. ) ;
#37440=CARTESIAN_POINT ( 'NONE',  ( 10.81189881249999729, 0.000000000000000000, -184.3437500020483810 ) ) ;
#37444=CARTESIAN_POINT ( 'NONE',  ( -2.293366432827344421E-15, -12.48450537969573659, -78.40625000204838102 ) ) ;
#37446=CARTESIAN_POINT ( 'NONE',  ( -9.999999999999998224, 5.773502691896259087, -48.25000000409676915 ) ) ;
#37447=CARTESIAN_POINT ( 'NONE',  ( 5.405949406249999534, 9.363379034771803333, -8.593750002048345493 ) ) ;
#37450=CARTESIAN_POINT ( 'NONE',  ( -10.81189881249999729, 1.324075727343319199E-15, -5.281250002048376579 ) ) ;
#37451=CARTESIAN_POINT ( 'NONE',  ( 0.000000000000000000, 0.000000000000000000, -99.99999999999998579 ) ) ;
#37454=DIRECTION ( 'NONE',  ( -0.000000000000000000, -0.000000000000000000, -1.000000000000000000 ) ) ;
#37457=ORIENTED_EDGE ( 'NONE', *, *, #11998, .T. ) ;
#37459=FACE_OUTER_BOUND ( 'NONE', #18925, .T. ) ;
#37461=ORIENTED_EDGE ( 'NONE', *, *, #36863, .F. ) ;
#37467=CARTESIAN_POINT ( 'NONE',  ( 5.000000000000000000, 8.660254037844385522, -40.74999999999997868 ) ) ;
#37469=CARTESIAN_POINT ( 'NONE',  ( 10.81189881249999551, -6.242252689847874514, -169.4687500020483810 ) ) ;
#37470=CARTESIAN_POINT ( 'NONE',  ( -2.293366432827344421E-15, -12.48450537969573659, -175.7187500020483810 ) ) ;
#37479=CARTESIAN_POINT ( 'NONE',  ( 5.405949406249999534, 9.363379034771803333, -61.09375000204836681 ) ) ;
#37480=CARTESIAN_POINT ( 'NONE',  ( 10.81189881249999907, 6.242252689847868297, -65.90625000204839523 ) ) ;
#37482=CARTESIAN_POINT ( 'NONE',  ( -10.00000000000000000, -5.773502691896251982, -131.6250000000000000 ) ) ;
#37484=CARTESIAN_POINT ( 'NONE',  ( 5.405949406249999534, 9.363379034771803333, -160.2812500020484094 ) ) ;
#37485=CARTESIAN_POINT ( 'NONE',  ( 7.644554776091147741E-16, 12.48450537969573659, -169.1562500020484094 ) ) ;
#37486=CARTESIAN_POINT ( 'NONE',  ( 5.405949406249999534, 9.363379034771803333, -1.093750002048365921 ) ) ;
#37487=CARTESIAN_POINT ( 'NONE',  ( -5.405949406250003975, -9.363379034771801557, -106.8437500020483810 ) ) ;
#37490=CARTESIAN_POINT ( 'NONE',  ( 10.81189881249999551, -6.242252689847874514, -7.656250002048365921 ) ) ;
#37492=CARTESIAN_POINT ( 'NONE',  ( -9.999999999999998224, 1.224646799147353059E-15, -133.6250000040967620 ) ) ;
#37493=CARTESIAN_POINT ( 'NONE',  ( 5.405949406249999534, 9.363379034771803333, -97.28125000204839523 ) ) ;
#37495=( BOUNDED_CURVE ( )  B_SPLINE_CURVE ( 2, ( #37049, #20430, #20002, #4250, #23474, #4034, #33408 ),
 .UNSPECIFIED., .F., .F. ) 
 B_SPLINE_CURVE_WITH_KNOTS ( ( 3, 2, 2, 3 ),
 ( 0.1865671641791045166, 0.1878109452736318741, 0.1890547263681592594, 0.1902985074626866169 ),
 .UNSPECIFIED. ) 
 CURVE ( )  GEOMETRIC_REPRESENTATION_ITEM ( )  RATIONAL_B_SPLINE_CURVE ( ( 0.9999999999999970024, 0.8660254037844417052, 1.000000000000000000, 0.8660254037844387076, 1.000000000000000000, 0.8660254037844327124, 1.000000000000005995 ) ) 
 REPRESENTATION_ITEM ( '' )  );
#37496=CARTESIAN_POINT ( 'NONE',  ( 5.000000000000000000, 8.660254037844385522, -78.62500000409677625 ) ) ;
#37497=CARTESIAN_POINT ( 'NONE',  ( 5.000000000000000000, 8.660254037844385522, -135.2499999999999716 ) ) ;
#37498=CARTESIAN_POINT ( 'NONE',  ( -5.405949406250003975, -9.363379034771801557, -36.34375000204836681 ) ) ;
#37501=CARTESIAN_POINT ( 'NONE',  ( -10.81189881249999729, 1.324075727343319199E-15, -24.78125000204836681 ) ) ;
#37504=CARTESIAN_POINT ( 'NONE',  ( 9.999999999999996447, -5.773502691896262640, -7.000000004096756712 ) ) ;
#37508=CARTESIAN_POINT ( 'NONE',  ( 9.999999999999998224, 0.000000000000000000, -120.5000000000000000 ) ) ;
#37510=ORIENTED_EDGE ( 'NONE', *, *, #36192, .F. ) ;
#37511=DIRECTION ( 'NONE',  ( -1.000000000000000000, 0.000000000000000000, 0.000000000000000000 ) ) ;
#37520=CARTESIAN_POINT ( 'NONE',  ( -5.000000000000003553, -8.660254037844383745, -128.8750000040967905 ) ) ;
#37521=CARTESIAN_POINT ( 'NONE',  ( 5.000000000000000000, 8.660254037844385522, -105.6250000040967763 ) ) ;
#37522=CARTESIAN_POINT ( 'NONE',  ( 10.81189881249999907, 6.242252689847868297, -161.9062500020484094 ) ) ;
#37526=CARTESIAN_POINT ( 'NONE',  ( 10.81189881249999907, 6.242252689847868297, -94.21875000204838102 ) ) ;
#37528=CARTESIAN_POINT ( 'NONE',  ( -2.293366432827344421E-15, -12.48450537969573659, -190.7187500020484094 ) ) ;
#37529=CARTESIAN_POINT ( 'NONE',  ( 5.405949406249992428, -9.363379034771808662, -97.78125000204839523 ) ) ;
#37531=CARTESIAN_POINT ( 'NONE',  ( -10.81189881249999729, 1.324075727343319199E-15, -108.5937500020483810 ) ) ;
#37533=CARTESIAN_POINT ( 'NONE',  ( -9.999999999999998224, 1.224646799147353059E-15, -151.6250000040967905 ) ) ;
#37535=CARTESIAN_POINT ( 'NONE',  ( 5.000000000000000000, 8.660254037844385522, -0.2499999999999724665 ) ) ;
#37537=CARTESIAN_POINT ( 'NONE',  ( -2.121150477449813534E-15, -11.54700538379251284, -172.2500000040968189 ) ) ;
#37539=CARTESIAN_POINT ( 'NONE',  ( 5.405949406249999534, 9.363379034771803333, -23.59375000204835970 ) ) ;
#37541=CARTESIAN_POINT ( 'NONE',  ( 10.81189881249999551, -6.242252689847874514, -131.9687500020483810 ) ) ;
#37543=CARTESIAN_POINT ( 'NONE',  ( -10.81189881249999907, -6.242252689847864744, -32.15625000204835970 ) ) ;
#37547=CARTESIAN_POINT ( 'NONE',  ( -10.00000000000000000, -5.773502691896251982, -53.62499999999997868 ) ) ;
#37548=CARTESIAN_POINT ( 'NONE',  ( -10.81189881249999729, 6.242252689847871849, -126.9062500020483810 ) ) ;
#37551=CARTESIAN_POINT ( 'NONE',  ( -4.999999999999996447, 8.660254037844387298, -97.87500000409677625 ) ) ;
#37554=CARTESIAN_POINT ( 'NONE',  ( 10.81189881249999907, 6.242252689847868297, -55.21875000204836681 ) ) ;
#37560=CARTESIAN_POINT ( 'NONE',  ( -4.999999999999996447, 8.660254037844387298, -24.37500000409675849 ) ) ;
#37565=EDGE_LOOP ( 'NONE', ( #1915, #2697, #9796, #14455 ) ) ;
#37567=EDGE_CURVE ( 'NONE', #29817, #35407, #23381, .T. ) ;
#37570=( BOUNDED_CURVE ( )  B_SPLINE_CURVE ( 2, ( #9657, #22830, #36196, #10075, #33188, #26905, #40061 ),
 .UNSPECIFIED., .F., .F. ) 
 B_SPLINE_CURVE_WITH_KNOTS ( ( 3, 2, 2, 3 ),
 ( 0.1343283582089551953, 0.1355721393034825528, 0.1368159203980099381, 0.1380597014925373234 ),
 .UNSPECIFIED. ) 
 CURVE ( )  GEOMETRIC_REPRESENTATION_ITEM ( )  RATIONAL_B_SPLINE_CURVE ( ( 1.000000000000003109, 0.8660254037844358210, 1.000000000000000000, 0.8660254037844387076, 1.000000000000000000, 0.8660254037844387076, 1.000000000000000000 ) ) 
 REPRESENTATION_ITEM ( '' )  );
#37572=CARTESIAN_POINT ( 'NONE',  ( 7.070501591499376803E-16, 11.54700538379251284, -174.5000000040967905 ) ) ;
#37574=CARTESIAN_POINT ( 'NONE',  ( 7.644554776091147741E-16, 12.48450537969573659, -193.1562500020484094 ) ) ;
#37580=CARTESIAN_POINT ( 'NONE',  ( 5.405949406249999534, 9.363379034771803333, -116.5937500020483810 ) ) ;
#37581=CARTESIAN_POINT ( 'NONE',  ( 4.999999999999992006, -8.660254037844389075, -194.6250000040967905 ) ) ;
#37582=CARTESIAN_POINT ( 'NONE',  ( -10.81189881249999729, 1.324075727343319199E-15, -120.7812500020483952 ) ) ;
#37584=CARTESIAN_POINT ( 'NONE',  ( 5.405949406249999534, 9.363379034771803333, -128.5937500020483810 ) ) ;
#37585=ADVANCED_FACE ( 'NONE', ( #37459 ), #24315, .F. ) ;
#37588=CARTESIAN_POINT ( 'NONE',  ( -9.999999999999998224, 5.773502691896259087, -149.8750000000000000 ) ) ;
#37589=CARTESIAN_POINT ( 'NONE',  ( 9.999999999999998224, 0.000000000000000000, -22.99999999999996447 ) ) ;
#37594=CARTESIAN_POINT ( 'NONE',  ( -5.405949406250003975, -9.363379034771801557, -48.34375000204838102 ) ) ;
#37595=CARTESIAN_POINT ( 'NONE',  ( 4.999999999999992006, -8.660254037844389075, -163.1250000040967905 ) ) ;
#37596=CARTESIAN_POINT ( 'NONE',  ( -10.81189881249999907, -6.242252689847864744, -156.4687500020484379 ) ) ;
#37599=CARTESIAN_POINT ( 'NONE',  ( -1.877755174760191048, 9.997121275661758233, -180.0000000000000284 ) ) ;
#37600=VECTOR ( 'NONE', #37338, 1000.000000000000000 ) ;
#37601=CARTESIAN_POINT ( 'NONE',  ( 10.00000000000000000, 5.773502691896255534, -87.37499999999998579 ) ) ;
#37604=CARTESIAN_POINT ( 'NONE',  ( -10.81189881249999729, -6.242252689847864744, -102.6562500020483952 ) ) ;
#37605=CARTESIAN_POINT ( 'NONE',  ( 4.999999999999992006, -8.660254037844389075, -125.6250000040967620 ) ) ;
#37606=CARTESIAN_POINT ( 'NONE',  ( 10.00000000000051159, -5.773502691895965988, -143.5000000040967905 ) ) ;
#37608=CARTESIAN_POINT ( 'NONE',  ( 7.070501591499376803E-16, 11.54700538379251284, -130.6250000000000000 ) ) ;
#37609=CARTESIAN_POINT ( 'NONE',  ( 7.644554776091147741E-16, 12.48450537969573659, -46.15625000204837391 ) ) ;
#37615=CARTESIAN_POINT ( 'NONE',  ( 9.999999999999998224, 0.000000000000000000, -177.5000000000000000 ) ) ;
#37616=ORIENTED_EDGE ( 'NONE', *, *, #29248, .F. ) ;
#37619=ORIENTED_EDGE ( 'NONE', *, *, #27535, .F. ) ;
#37632=CARTESIAN_POINT ( 'NONE',  ( -5.405949406249996869, 9.363379034771805109, -144.8437500020483810 ) ) ;
#37633=CARTESIAN_POINT ( 'NONE',  ( 10.81189881249999551, -6.242252689847874514, -150.1562500020484094 ) ) ;
#37634=CARTESIAN_POINT ( 'NONE',  ( 10.81189881249999729, 0.000000000000000000, -152.8437500020483810 ) ) ;
#37637=CARTESIAN_POINT ( 'NONE',  ( -10.00000000000000000, -5.773502691896251982, -167.6249999999999716 ) ) ;
#37642=CARTESIAN_POINT ( 'NONE',  ( 10.81189881249999551, -6.242252689847874514, -178.4687500020484094 ) ) ;
#37646=CARTESIAN_POINT ( 'NONE',  ( -10.81189881249999729, 6.242252689847871849, -42.90625000204836681 ) ) ;
#37648=CARTESIAN_POINT ( 'NONE',  ( 5.000000000000000000, 8.660254037844385522, -106.7499999999999858 ) ) ;
#37650=CARTESIAN_POINT ( 'NONE',  ( 7.644554776091147741E-16, 12.48450537969573659, -128.6562500020483810 ) ) ;
#37651=CARTESIAN_POINT ( 'NONE',  ( -5.000000000000003553, -8.660254037844383745, -148.3750000040967905 ) ) ;
#37655=CARTESIAN_POINT ( 'NONE',  ( 7.644554776091147741E-16, 12.48450537969573659, -173.4687500020483810 ) ) ;
#37657=CARTESIAN_POINT ( 'NONE',  ( -9.999999999999998224, 0.000000000000000000, -99.99999999999998579 ) ) ;
#37659=CARTESIAN_POINT ( 'NONE',  ( 10.81189881249999907, 6.242252689847868297, -64.40625000204839523 ) ) ;
#37660=CONICAL_SURFACE ( 'NONE', #32832, 22.00000000000000711, 0.7853981633974466137 ) ;
#37662=CARTESIAN_POINT ( 'NONE',  ( 7.070501591499377789E-16, 11.54700538379251284, -42.50000000409676204 ) ) ;
#37663=CARTESIAN_POINT ( 'NONE',  ( 5.405949406249999534, 9.363379034771803333, -4.093750002048368586 ) ) ;
#37671=LINE ( 'NONE', #21263, #4126 ) ;
#37681=ORIENTED_EDGE ( 'NONE', *, *, #17752, .F. ) ;
#37683=CARTESIAN_POINT ( 'NONE',  ( -9.999999999999998224, 1.224646799147353059E-15, -32.74999999999997158 ) ) ;
#37685=CARTESIAN_POINT ( 'NONE',  ( 10.81189881249999729, 0.000000000000000000, -166.3437500020484094 ) ) ;
#37686=CARTESIAN_POINT ( 'NONE',  ( 10.81189881249999729, 6.242252689847867408, -176.7187500020484094 ) ) ;
#37689=CARTESIAN_POINT ( 'NONE',  ( 9.999999999999994671, -5.773502691896262640, -167.5000000040967905 ) ) ;
#37697=CARTESIAN_POINT ( 'NONE',  ( -10.81189881249999729, 6.242252689847871849, -65.21875000204838102 ) ) ;
#37698=CARTESIAN_POINT ( 'NONE',  ( -10.81189881249999907, -6.242252689847864744, -65.15625000204838102 ) ) ;
#37700=CARTESIAN_POINT ( 'NONE',  ( 4.999999999999992006, -8.660254037844389075, -134.2499999999999716 ) ) ;
#37701=CARTESIAN_POINT ( 'NONE',  ( 10.81189881249999729, 0.000000000000000000, -150.0312500020483810 ) ) ;
#37702=CARTESIAN_POINT ( 'NONE',  ( 5.405949406249999534, 9.363379034771803333, -163.2812500020484094 ) ) ;
#37704=DIRECTION ( 'NONE',  ( -1.000000000000000000, 0.000000000000000000, -0.000000000000000000 ) ) ;
#37705=CARTESIAN_POINT ( 'NONE',  ( -10.81189881249999907, -6.242252689847864744, -99.46875000204838102 ) ) ;
#37708=CARTESIAN_POINT ( 'NONE',  ( 10.81189881249999551, -6.242252689847874514, -194.9687500020484094 ) ) ;
#37711=CARTESIAN_POINT ( 'NONE',  ( 10.81189881249999907, 6.242252689847868297, -91.40625000204836681 ) ) ;
#37713=CARTESIAN_POINT ( 'NONE',  ( 9.999999999999998224, 0.000000000000000000, -74.37500000409677625 ) ) ;
#37715=CARTESIAN_POINT ( 'NONE',  ( -10.81189881249999729, 1.324075727343319199E-15, -29.09375000204836326 ) ) ;
#37718=CARTESIAN_POINT ( 'NONE',  ( -5.405949406250003975, -9.363379034771801557, -24.53125000204836681 ) ) ;
#37721=CARTESIAN_POINT ( 'NONE',  ( 5.000000000000000000, 8.660254037844385522, -8.125000004096744277 ) ) ;
#37729=ORIENTED_EDGE ( 'NONE', *, *, #30982, .T. ) ;
#37734=CYLINDRICAL_SURFACE ( 'NONE', #33920, 9.999999999999998224 ) ;
#37735=CARTESIAN_POINT ( 'NONE',  ( 9.999999999999998224, 0.000000000000000000, -128.3750000040967905 ) ) ;
#37738=CARTESIAN_POINT ( 'NONE',  ( 5.405949406249992428, -9.363379034771808662, -163.7812500020484094 ) ) ;
#37741=CARTESIAN_POINT ( 'NONE',  ( -2.293366432827344421E-15, -12.48450537969573659, -84.21875000204835260 ) ) ;
#37743=CARTESIAN_POINT ( 'NONE',  ( -5.405949406249996869, 9.363379034771805109, -194.3437500020484094 ) ) ;
#37744=CARTESIAN_POINT ( 'NONE',  ( 10.81189881249999907, 6.242252689847868297, -95.90625000204839523 ) ) ;
#37748=CARTESIAN_POINT ( 'NONE',  ( -10.81189881249999729, 1.324075727343319199E-15, -173.2812500020484094 ) ) ;
#37749=CARTESIAN_POINT ( 'NONE',  ( -10.81189881249999729, 6.242252689847871849, -189.9062500020484379 ) ) ;
#37751=CARTESIAN_POINT ( 'NONE',  ( -9.999999999999998224, 1.224646799147353059E-15, -162.1250000040967905 ) ) ;
#37753=CARTESIAN_POINT ( 'NONE',  ( -5.405949406250003975, -9.363379034771801557, -10.84375000204834727 ) ) ;
#37754=CARTESIAN_POINT ( 'NONE',  ( 5.405949406249992428, -9.363379034771808662, -126.0937500020483668 ) ) ;
#37755=ADVANCED_FACE ( 'NONE', ( #27539 ), #17803, .F. ) ;
#37757=CARTESIAN_POINT ( 'NONE',  ( -2.293366432827344421E-15, -12.48450537969573659, -19.90625000204837391 ) ) ;
#37759=CARTESIAN_POINT ( 'NONE',  ( -5.000000000000003553, -8.660254037844383745, -136.3750000040967905 ) ) ;
#37761=CARTESIAN_POINT ( 'NONE',  ( -9.999999999999998224, 5.773502691896259087, -55.37499999999998579 ) ) ;
#37762=CARTESIAN_POINT ( 'NONE',  ( -2.293366432827344421E-15, -12.48450537969573659, -120.4062500020483952 ) ) ;
#37764=EDGE_LOOP ( 'NONE', ( #33748, #1189, #20470, #9820 ) ) ;
#37765=CARTESIAN_POINT ( 'NONE',  ( 9.999999999999998224, 0.000000000000000000, -96.87500000409677625 ) ) ;
#37768=CARTESIAN_POINT ( 'NONE',  ( -2.293366432827344421E-15, -12.48450537969573659, -60.21875000204837391 ) ) ;
#37775=CARTESIAN_POINT ( 'NONE',  ( 7.070501591499377789E-16, 11.54700538379251284, -27.50000000409677270 ) ) ;
#37785=CYLINDRICAL_SURFACE ( 'NONE', #9340, 9.999999999999998224 ) ;
#37788=CARTESIAN_POINT ( 'NONE',  ( 10.81189881249999551, -6.242252689847874514, -187.6562500020484379 ) ) ;
#37794=CARTESIAN_POINT ( 'NONE',  ( 10.81189881249999551, -6.242252689847874514, -112.4687500020483810 ) ) ;
#37796=CARTESIAN_POINT ( 'NONE',  ( -2.293366432827344421E-15, -12.48450537969573659, -112.9062500020483952 ) ) ;
#37798=CARTESIAN_POINT ( 'NONE',  ( -10.81189881249999729, 6.242252689847871849, -132.7187500020483810 ) ) ;
#37801=CARTESIAN_POINT ( 'NONE',  ( 7.070501591499377789E-16, 11.54700538379251284, -147.1250000000000000 ) ) ;
#37802=CARTESIAN_POINT ( 'NONE',  ( 9.999999999999998224, 0.000000000000000000, -19.99999999999996092 ) ) ;
#37807=CARTESIAN_POINT ( 'NONE',  ( -5.405949406250003975, -9.363379034771801557, -45.34375000204838102 ) ) ;
#37809=EDGE_CURVE ( 'NONE', #27414, #21209, #15205, .T. ) ;
#37810=CARTESIAN_POINT ( 'NONE',  ( 5.405949406249992428, -9.363379034771808662, -145.5937500020483810 ) ) ;
#37814=CARTESIAN_POINT ( 'NONE',  ( 9.988285040850783503, 3.942477841776621084, -180.0000000000000568 ) ) ;
#37815=CARTESIAN_POINT ( 'NONE',  ( 10.00000000000000000, 5.773502691896255534, -72.37499999999997158 ) ) ;
#37819=CARTESIAN_POINT ( 'NONE',  ( -10.81189881249999729, -6.242252689847864744, -104.1562500020483952 ) ) ;
#37820=CARTESIAN_POINT ( 'NONE',  ( -9.999999999999998224, 1.224646799147353059E-15, -123.1250000040967905 ) ) ;
#37822=CARTESIAN_POINT ( 'NONE',  ( -10.81189881249999907, -6.242252689847864744, -81.46875000204838102 ) ) ;
#37826=CARTESIAN_POINT ( 'NONE',  ( 10.81189881249999551, -6.242252689847874514, -45.15625000204836681 ) ) ;
#37836=ORIENTED_EDGE ( 'NONE', *, *, #28393, .F. ) ;
#37838=CARTESIAN_POINT ( 'NONE',  ( 10.00000000000012257, -5.773502691896187144, -165.6250000000000000 ) ) ;
#37846=CARTESIAN_POINT ( 'NONE',  ( -5.405949406249996869, 9.363379034771805109, -140.3437500020484094 ) ) ;
#37847=CARTESIAN_POINT ( 'NONE',  ( -2.293366432827344421E-15, -12.48450537969573659, -150.4062500020483810 ) ) ;
#37848=CARTESIAN_POINT ( 'NONE',  ( 10.81189881249999551, -6.242252689847874514, -155.9687500020484094 ) ) ;
#37849=CARTESIAN_POINT ( 'NONE',  ( 9.999999999999998224, 0.000000000000000000, -165.8750000040967905 ) ) ;
#37851=CARTESIAN_POINT ( 'NONE',  ( -2.121150477449813534E-15, -11.54700538379251284, -171.8750000000000284 ) ) ;
#37855=CARTESIAN_POINT ( 'NONE',  ( -10.36423010611328799, -0.9417504169010495474, -99.99999999999998579 ) ) ;
#37856=CARTESIAN_POINT ( 'NONE',  ( -10.81189881249999729, 1.324075727343319199E-15, -177.5937500020484094 ) ) ;
#37859=CARTESIAN_POINT ( 'NONE',  ( 0.000000000000000000, 0.000000000000000000, -99.99999999999998579 ) ) ;
#37860=CARTESIAN_POINT ( 'NONE',  ( 10.81189881249999729, 0.000000000000000000, -42.03125000204838102 ) ) ;
#37862=CARTESIAN_POINT ( 'NONE',  ( 4.999999999999992006, -8.660254037844389075, -99.74999999999998579 ) ) ;
#37864=CARTESIAN_POINT ( 'NONE',  ( -2.293366432827344421E-15, -12.48450537969573659, -123.4062500020483952 ) ) ;
#37865=CARTESIAN_POINT ( 'NONE',  ( -10.00000000000000000, -5.773502691896251982, -151.5000000040967905 ) ) ;
#37869=CARTESIAN_POINT ( 'NONE',  ( 7.644554776091147741E-16, 12.48450537969573659, -174.9687500020484094 ) ) ;
#37871=LINE ( 'NONE', #30983, #21710 ) ;
#37873=CARTESIAN_POINT ( 'NONE',  ( 5.405949406249999534, 9.363379034771803333, -68.78125000204838102 ) ) ;
#37876=CARTESIAN_POINT ( 'NONE',  ( -5.000000000000003553, -8.660254037844383745, -47.87500000409677625 ) ) ;
#37878=CARTESIAN_POINT ( 'NONE',  ( -10.81189881249999729, 6.242252689847871849, -5.218750002048355263 ) ) ;
#37888=ORIENTED_EDGE ( 'NONE', *, *, #9191, .F. ) ;
#37889=DIRECTION ( 'NONE',  ( 1.000000000000000000, 0.000000000000000000, 0.000000000000000000 ) ) ;
#37900=CARTESIAN_POINT ( 'NONE',  ( 5.000000000000000000, 8.660254037844385522, -34.74999999999997868 ) ) ;
#37903=CARTESIAN_POINT ( 'NONE',  ( -10.81189881249999907, -6.242252689847864744, -168.4687500020483526 ) ) ;
#37904=CARTESIAN_POINT ( 'NONE',  ( 10.81189881249999729, 6.242252689847867408, -178.2187500020484094 ) ) ;
#37906=DIRECTION ( 'NONE',  ( -0.000000000000000000, -0.000000000000000000, -1.000000000000000000 ) ) ;
#37907=CARTESIAN_POINT ( 'NONE',  ( -10.00000000000000000, -5.773502691896251982, -199.1250000000000284 ) ) ;
#37912=CARTESIAN_POINT ( 'NONE',  ( -10.81189881249999729, 6.242252689847871849, -60.71875000204838102 ) ) ;
#37913=CARTESIAN_POINT ( 'NONE',  ( -5.405949406250003975, -9.363379034771801557, -72.53125000204838102 ) ) ;
#37915=CARTESIAN_POINT ( 'NONE',  ( -5.000000000000003553, -8.660254037844383745, -121.0000000000000000 ) ) ;
#37916=CARTESIAN_POINT ( 'NONE',  ( -10.81189881249999729, 6.242252689847871849, -150.9062500020484094 ) ) ;
#37917=CARTESIAN_POINT ( 'NONE',  ( 10.81189881249999729, 0.000000000000000000, -162.0312500020484094 ) ) ;
#37920=CARTESIAN_POINT ( 'NONE',  ( 10.81189881249999907, 6.242252689847868297, -94.21875000204838102 ) ) ;
#37921=ORIENTED_EDGE ( 'NONE', *, *, #31149, .T. ) ;
#37923=CARTESIAN_POINT ( 'NONE',  ( -5.405949406250003975, -9.363379034771801557, -198.3437500020484094 ) ) ;
#37925=CARTESIAN_POINT ( 'NONE',  ( -5.604939563500185962, -8.526197496611898075, -180.0000000000000000 ) ) ;
#37926=CARTESIAN_POINT ( 'NONE',  ( -5.405949406250003975, -9.363379034771801557, -90.53125000204838102 ) ) ;
#37928=CARTESIAN_POINT ( 'NONE',  ( -5.000000000000003553, -8.660254037844383745, -71.87500000409677625 ) ) ;
#37930=CARTESIAN_POINT ( 'NONE',  ( -10.81189881249999729, 6.242252689847871849, -29.21875000204834905 ) ) ;
#37933=EDGE_CURVE ( 'NONE', #39083, #342, #42639, .T. ) ;
#37934=CARTESIAN_POINT ( 'NONE',  ( -2.293366432827344421E-15, -12.48450537969573659, -21.40625000204837747 ) ) ;
#37936=CARTESIAN_POINT ( 'NONE',  ( -9.999999999999998224, 1.224646799147353059E-15, -118.6250000040967905 ) ) ;
#37938=CARTESIAN_POINT ( 'NONE',  ( -9.999999999999998224, 1.224646799147353059E-15, -0.1250000040967647053 ) ) ;
#37939=CARTESIAN_POINT ( 'NONE',  ( -9.999999999999998224, 1.224646799147353059E-15, -151.6250000040967905 ) ) ;
#37947=ORIENTED_EDGE ( 'NONE', *, *, #16683, .F. ) ;
#37948=EDGE_CURVE ( 'NONE', #22601, #36180, #36599, .T. ) ;
#37954=CARTESIAN_POINT ( 'NONE',  ( -10.81189881249999907, -6.242252689847864744, -167.1562500020483810 ) ) ;
#37956=VECTOR ( 'NONE', #33860, 1000.000000000000000 ) ;
#37957=VECTOR ( 'NONE', #10624, 1000.000000000000000 ) ;
#37959=CARTESIAN_POINT ( 'NONE',  ( -10.81189881249999729, 6.242252689847871849, -89.21875000204836681 ) ) ;
#37961=CARTESIAN_POINT ( 'NONE',  ( 5.405949406249992428, -9.363379034771808662, -192.0937500020484094 ) ) ;
#37962=CARTESIAN_POINT ( 'NONE',  ( -5.405949406249996869, 9.363379034771805109, -92.53125000204838102 ) ) ;
#37965=CARTESIAN_POINT ( 'NONE',  ( -2.121150477449813534E-15, -11.54700538379251284, -150.8750000000000000 ) ) ;
#37966=CARTESIAN_POINT ( 'NONE',  ( 7.644554776091147741E-16, 12.48450537969573659, -173.6562500020483810 ) ) ;
#37967=CARTESIAN_POINT ( 'NONE',  ( -2.293366432827344421E-15, -12.48450537969573659, -190.9062500020483810 ) ) ;
#37969=EDGE_CURVE ( 'NONE', #24099, #1756, #33845, .T. ) ;
#37970=CARTESIAN_POINT ( 'NONE',  ( -4.999999999999996447, 8.660254037844387298, -162.3750000040967905 ) ) ;
#37972=CARTESIAN_POINT ( 'NONE',  ( 10.81189881249999729, 0.000000000000000000, -10.34375000204834549 ) ) ;
#37973=CARTESIAN_POINT ( 'NONE',  ( 9.999999999999998224, 0.000000000000000000, -122.3750000040967905 ) ) ;
#37974=CARTESIAN_POINT ( 'NONE',  ( 10.81189881249999551, -6.242252689847874514, -121.4687500020484094 ) ) ;
#37976=CARTESIAN_POINT ( 'NONE',  ( 10.81189881249999551, -6.242252689847874514, -21.15625000204837391 ) ) ;
#37978=CARTESIAN_POINT ( 'NONE',  ( -9.999999999999998224, 1.224646799147353059E-15, -50.74999999999996447 ) ) ;
#37979=CARTESIAN_POINT ( 'NONE',  ( -5.405949406249996869, 9.363379034771805109, -119.5312500020483952 ) ) ;
#37981=ORIENTED_EDGE ( 'NONE', *, *, #26060, .F. ) ;
#37983=CARTESIAN_POINT ( 'NONE',  ( -9.999999999999998224, 1.224646799147353059E-15, -96.12500000409677625 ) ) ;
#37986=CARTESIAN_POINT ( 'NONE',  ( 10.81189881249999729, 0.000000000000000000, -46.34375000204838102 ) ) ;
#37992=CARTESIAN_POINT ( 'NONE',  ( -2.121150477449813534E-15, -11.54700538379251284, -25.25000000409676915 ) ) ;
#37997=VERTEX_POINT ( 'NONE', #23875 ) ;
#38001=ADVANCED_FACE ( 'NONE', ( #29712 ), #39828, .F. ) ;
#38003=ORIENTED_EDGE ( 'NONE', *, *, #20808, .T. ) ;
#38004=CARTESIAN_POINT ( 'NONE',  ( 0.000000000000000000, 0.000000000000000000, -99.99999999999998579 ) ) ;
#38007=CARTESIAN_POINT ( 'NONE',  ( -10.81189881249999907, -6.242252689847864744, -189.6562500020484094 ) ) ;
#38011=CARTESIAN_POINT ( 'NONE',  ( 10.81189881249999907, 6.242252689847868297, -113.7187500020483810 ) ) ;
#38013=CARTESIAN_POINT ( 'NONE',  ( -5.405949406249996869, 9.363379034771805109, -118.0312500020483952 ) ) ;
#38015=CARTESIAN_POINT ( 'NONE',  ( 10.81189881249999729, 0.000000000000000000, -124.3437500020483952 ) ) ;
#38016=CIRCLE ( 'NONE', #28350, 9.999999999999998224 ) ;
#38019=CARTESIAN_POINT ( 'NONE',  ( -5.000000000000003553, -8.660254037844383745, -145.0000000000000000 ) ) ;
#38020=CARTESIAN_POINT ( 'NONE',  ( 10.00000000000000000, 5.773502691896255534, -10.87499999999996625 ) ) ;
#38024=CARTESIAN_POINT ( 'NONE',  ( 10.00000000000000000, 5.773502691896255534, -191.2500000040968189 ) ) ;
#38026=CARTESIAN_POINT ( 'NONE',  ( 10.81189881249999907, 6.242252689847868297, -34.21875000204835260 ) ) ;
#38027=FACE_OUTER_BOUND ( 'NONE', #19881, .T. ) ;
#38028=CARTESIAN_POINT ( 'NONE',  ( 7.644554776091147741E-16, 12.48450537969573659, -147.9687500020484094 ) ) ;
#38030=CARTESIAN_POINT ( 'NONE',  ( -9.999999999999998224, 1.224646799147353059E-15, -71.74999999999998579 ) ) ;
#38031=CARTESIAN_POINT ( 'NONE',  ( 10.81189881249999729, 0.000000000000000000, -144.0312500020483810 ) ) ;
#38033=ORIENTED_EDGE ( 'NONE', *, *, #23486, .F. ) ;
#38034=CARTESIAN_POINT ( 'NONE',  ( -10.81189881249999729, 6.242252689847871849, -104.4062500020483810 ) ) ;
#38035=CARTESIAN_POINT ( 'NONE',  ( -10.00000000000000000, -5.773502691896251982, -114.0000000040967905 ) ) ;
#38037=CARTESIAN_POINT ( 'NONE',  ( 10.81189881249999729, 0.000000000000000000, -71.84375000204836681 ) ) ;
#38041=CARTESIAN_POINT ( 'NONE',  ( -2.293366432827344421E-15, -12.48450537969573659, -42.40625000204836681 ) ) ;
#38048=EDGE_LOOP ( 'NONE', ( #18384, #9223, #12593, #39813 ) ) ;
#38049=EDGE_CURVE ( 'NONE', #5023, #26528, #29184, .T. ) ;
#38051=EDGE_CURVE ( 'NONE', #23180, #26892, #30569, .T. ) ;
#38058=CARTESIAN_POINT ( 'NONE',  ( 5.405949406249992428, -9.363379034771808662, -130.5937500020483810 ) ) ;
#38059=CARTESIAN_POINT ( 'NONE',  ( -10.81189881249999729, 1.324075727343319199E-15, -141.7812500020483810 ) ) ;
#38060=CARTESIAN_POINT ( 'NONE',  ( -10.81189881249999729, -6.242252689847864744, -156.4687500020484094 ) ) ;
#38063=CARTESIAN_POINT ( 'NONE',  ( -10.00000000000000000, -5.773502691896251982, -175.1249999999999716 ) ) ;
#38067=CARTESIAN_POINT ( 'NONE',  ( -10.12150904654152761, -2.198084950377523050, -100.0000000000000142 ) ) ;
#38068=CARTESIAN_POINT ( 'NONE',  ( 7.644554776091147741E-16, 12.48450537969573659, -170.4687500020483810 ) ) ;
#38072=CYLINDRICAL_SURFACE ( 'NONE', #3433, 9.999999999999998224 ) ;
#38073=CARTESIAN_POINT ( 'NONE',  ( -10.81189881249999729, 6.242252689847871849, -45.90625000204836681 ) ) ;
#38075=CARTESIAN_POINT ( 'NONE',  ( 4.999999999999992006, -8.660254037844389075, -96.74999999999998579 ) ) ;
#38077=CARTESIAN_POINT ( 'NONE',  ( 5.405949406249992428, -9.363379034771808662, -123.2812500020483952 ) ) ;
#38078=CARTESIAN_POINT ( 'NONE',  ( 9.999999999999996447, -5.773502691896262640, -148.0000000040968189 ) ) ;
#38081=CARTESIAN_POINT ( 'NONE',  ( 10.81189881249999907, 6.242252689847868297, -170.7187500020483810 ) ) ;
#38086=CARTESIAN_POINT ( 'NONE',  ( -5.405949406250003975, -9.363379034771801557, -66.53125000204838102 ) ) ;
#38087=CARTESIAN_POINT ( 'NONE',  ( -2.121150477449813534E-15, -11.54700538379251284, -40.25000000409676204 ) ) ;
#38088=CARTESIAN_POINT ( 'NONE',  ( 10.81189881249999907, 6.242252689847868297, -4.218750002048355263 ) ) ;
#38091=CARTESIAN_POINT ( 'NONE',  ( 9.999999999999998224, 0.000000000000000000, -107.3750000040967763 ) ) ;
#38092=CARTESIAN_POINT ( 'NONE',  ( -10.00000000000051337, 5.773502691895962435, -148.3749999999999716 ) ) ;
#38101=ORIENTED_EDGE ( 'NONE', *, *, #23406, .T. ) ;
#38109=CARTESIAN_POINT ( 'NONE',  ( -9.999999999999998224, 1.224646799147353059E-15, -109.6250000040967763 ) ) ;
#38110=CARTESIAN_POINT ( 'NONE',  ( -5.000000000000003553, -8.660254037844383745, -39.99999999999997868 ) ) ;
#38113=CARTESIAN_POINT ( 'NONE',  ( 5.405949406249999534, 9.363379034771803333, -158.5937500020483810 ) ) ;
#38114=CARTESIAN_POINT ( 'NONE',  ( 10.81189881249999551, -6.242252689847874514, -175.4687500020484094 ) ) ;
#38117=CARTESIAN_POINT ( 'NONE',  ( 5.000000000000000000, 8.660254037844385522, -193.7500000000000000 ) ) ;
#38122=CARTESIAN_POINT ( 'NONE',  ( -2.293366432827344421E-15, -12.48450537969573659, -72.40625000204836681 ) ) ;
#38124=CARTESIAN_POINT ( 'NONE',  ( -10.00000000000000000, -5.773502691896251982, -127.1249999999999858 ) ) ;
#38127=CARTESIAN_POINT ( 'NONE',  ( -10.81189881249999729, -6.242252689847864744, -153.6562500020484094 ) ) ;
#38128=CARTESIAN_POINT ( 'NONE',  ( 10.81189881249999551, -6.242252689847874514, -162.1562500020484379 ) ) ;
#38131=CARTESIAN_POINT ( 'NONE',  ( -2.293366432827344421E-15, -12.48450537969573659, -94.71875000204838102 ) ) ;
#38134=CARTESIAN_POINT ( 'NONE',  ( -10.81189881249999729, 1.324075727343319199E-15, -197.0937500020484094 ) ) ;
#38137=CARTESIAN_POINT ( 'NONE',  ( -9.999999999999998224, 1.224646799147353059E-15, -157.2500000000000000 ) ) ;
#38138=CARTESIAN_POINT ( 'NONE',  ( -5.405949406249996869, 9.363379034771805109, -94.03125000204838102 ) ) ;
#38141=CARTESIAN_POINT ( 'NONE',  ( 10.00000000000000000, 5.773502691896255534, -71.25000000409676204 ) ) ;
#38143=CARTESIAN_POINT ( 'NONE',  ( 10.81189881249999729, 0.000000000000000000, -23.84375000204835970 ) ) ;
#38146=CARTESIAN_POINT ( 'NONE',  ( -5.405949406249996869, 9.363379034771805109, -20.53125000204836326 ) ) ;
#38164=CARTESIAN_POINT ( 'NONE',  ( 7.644554776091147741E-16, 12.48450537969573659, -166.1562500020483810 ) ) ;
#38167=EDGE_CURVE ( 'NONE', #6210, #1756, #1420, .T. ) ;
#38169=CARTESIAN_POINT ( 'NONE',  ( -10.81189881249999729, 6.242252689847871849, -87.71875000204838102 ) ) ;
#38171=CARTESIAN_POINT ( 'NONE',  ( 10.81189881249999729, 0.000000000000000000, -196.3437500020484094 ) ) ;
#38172=CARTESIAN_POINT ( 'NONE',  ( 10.81189881249999551, -6.242252689847874514, -96.15625000204838102 ) ) ;
#38175=CARTESIAN_POINT ( 'NONE',  ( 9.999999999999998224, 0.000000000000000000, -164.3750000040967905 ) ) ;
#38176=CARTESIAN_POINT ( 'NONE',  ( -10.81189881249999729, 1.324075727343319199E-15, -176.2812500020484094 ) ) ;
#38177=CARTESIAN_POINT ( 'NONE',  ( -10.81189881249999729, 1.324075727343319199E-15, -185.2812500020484094 ) ) ;
#38179=CARTESIAN_POINT ( 'NONE',  ( 9.999999999999998224, 0.000000000000000000, -165.8750000040967905 ) ) ;
#38181=CARTESIAN_POINT ( 'NONE',  ( -10.81189881249999907, -6.242252689847864744, -13.96875000204836326 ) ) ;
#38183=CARTESIAN_POINT ( 'NONE',  ( 10.81189881249999907, 6.242252689847868297, -125.7187500020483810 ) ) ;
#38185=CARTESIAN_POINT ( 'NONE',  ( 7.644554776091147741E-16, 12.48450537969573659, -17.65625000204837391 ) ) ;
#38188=CARTESIAN_POINT ( 'NONE',  ( 5.000000000000000000, 8.660254037844385522, -52.74999999999996447 ) ) ;
#38189=CARTESIAN_POINT ( 'NONE',  ( 10.81189881249999551, -6.242252689847874514, -114.1562500020483952 ) ) ;
#38191=EDGE_CURVE ( 'NONE', #1644, #29774, #17301, .T. ) ;
#38193=CARTESIAN_POINT ( 'NONE',  ( -2.121150477449813534E-15, -11.54700538379251284, -91.25000000409677625 ) ) ;
#38194=LINE ( 'NONE', #12687, #32589 ) ;
#38196=CARTESIAN_POINT ( 'NONE',  ( -10.81189881249999729, 1.324075727343319199E-15, -48.59375000204838102 ) ) ;
#38201=CARTESIAN_POINT ( 'NONE',  ( -2.121150477449813534E-15, -11.54700538379251284, -22.25000000409676915 ) ) ;
#38211=VERTEX_POINT ( 'NONE', #40452 ) ;
#38217=CARTESIAN_POINT ( 'NONE',  ( -10.81189881249999907, -6.242252689847864744, -191.1562500020484094 ) ) ;
#38221=CARTESIAN_POINT ( 'NONE',  ( 7.644554776091147741E-16, 12.48450537969573659, -107.4687500020483668 ) ) ;
#38223=CARTESIAN_POINT ( 'NONE',  ( 7.644554776091147741E-16, 12.48450537969573659, -116.6562500020483952 ) ) ;
#38225=CARTESIAN_POINT ( 'NONE',  ( 5.405949406249992428, -9.363379034771808662, -121.5937500020483952 ) ) ;
#38227=CARTESIAN_POINT ( 'NONE',  ( 9.999999999999998224, 0.000000000000000000, -158.0000000000000000 ) ) ;
#38228=CARTESIAN_POINT ( 'NONE',  ( -2.121150477449813534E-15, -11.54700538379251284, -146.3750000000000000 ) ) ;
#38229=CARTESIAN_POINT ( 'NONE',  ( -4.999999999999996447, 8.660254037844387298, -8.999999999999952038 ) ) ;
#38232=CARTESIAN_POINT ( 'NONE',  ( 10.00000000000000000, 5.773502691896255534, -185.2500000040967905 ) ) ;
#38234=CARTESIAN_POINT ( 'NONE',  ( 10.81189881249999907, 6.242252689847868297, -38.71875000204835260 ) ) ;
#38236=CARTESIAN_POINT ( 'NONE',  ( -10.81189881249999729, 1.324075727343319199E-15, -149.0937500020483810 ) ) ;
#38239=CARTESIAN_POINT ( 'NONE',  ( -9.999999999999479527, -5.773502691896549521, -148.1249999999999716 ) ) ;
#38240=CARTESIAN_POINT ( 'NONE',  ( -5.000000000000003553, -8.660254037844383745, -71.49999999999998579 ) ) ;
#38241=CARTESIAN_POINT ( 'NONE',  ( 10.81189881249999551, -6.242252689847874514, -139.6562500020484094 ) ) ;
#38244=CARTESIAN_POINT ( 'NONE',  ( -5.405949406250003975, -9.363379034771801557, -102.5312500020483952 ) ) ;
#38245=CARTESIAN_POINT ( 'NONE',  ( 5.000000000000000000, 8.660254037844385522, -114.6250000040967763 ) ) ;
#38246=CARTESIAN_POINT ( 'NONE',  ( 9.999999999999998224, 0.000000000000000000, -140.0000000000000000 ) ) ;
#38247=CARTESIAN_POINT ( 'NONE',  ( -2.293366432827344421E-15, -12.48450537969573659, -72.21875000204835260 ) ) ;
#38250=CARTESIAN_POINT ( 'NONE',  ( -5.405949406250003975, -9.363379034771801557, -41.03125000204838102 ) ) ;
#38267=CARTESIAN_POINT ( 'NONE',  ( -10.81189881249999729, 6.242252689847871849, -135.7187500020483810 ) ) ;
#38269=CARTESIAN_POINT ( 'NONE',  ( 10.81189881249999907, 6.242252689847868297, -142.4062500020484094 ) ) ;
#38270=CARTESIAN_POINT ( 'NONE',  ( 7.644554776091147741E-16, 12.48450537969573659, -143.4687500020484094 ) ) ;
#38273=CARTESIAN_POINT ( 'NONE',  ( -5.000000000000003553, -8.660254037844383745, -175.0000000000000284 ) ) ;
#38275=CARTESIAN_POINT ( 'NONE',  ( -5.000000000000003553, -8.660254037844383745, -113.8750000040967763 ) ) ;
#38278=CARTESIAN_POINT ( 'NONE',  ( 10.81189881249999729, 0.000000000000000000, -170.8437500020484094 ) ) ;
#38282=CARTESIAN_POINT ( 'NONE',  ( 5.405949406249999534, 9.363379034771803333, -43.28125000204838102 ) ) ;
#38284=CARTESIAN_POINT ( 'NONE',  ( -2.121150477449813534E-15, -11.54700538379251284, -101.3750000000000000 ) ) ;
#38286=AXIS2_PLACEMENT_3D ( 'NONE', #25516, #32204, #2633 ) ;
#38287=CARTESIAN_POINT ( 'NONE',  ( -5.405949406249996869, 9.363379034771805109, -130.0312500020484094 ) ) ;
#38288=CARTESIAN_POINT ( 'NONE',  ( 9.999999999999998224, 0.000000000000000000, -137.3750000040967905 ) ) ;
#38289=CARTESIAN_POINT ( 'NONE',  ( 9.999999999999998224, 0.000000000000000000, -147.5000000000000000 ) ) ;
#38292=CARTESIAN_POINT ( 'NONE',  ( -10.81189881249999729, 1.324075727343319199E-15, -174.5937500020484094 ) ) ;
#38296=CARTESIAN_POINT ( 'NONE',  ( 10.81189881249999907, 6.242252689847868297, -71.90625000204836681 ) ) ;
#38297=CARTESIAN_POINT ( 'NONE',  ( 5.000000000000000000, 8.660254037844385522, -47.12500000409677625 ) ) ;
#38304=CARTESIAN_POINT ( 'NONE',  ( -9.999999999999998224, 1.224646799147353059E-15, -137.7499999999999716 ) ) ;
#38305=VECTOR ( 'NONE', #21379, 1000.000000000000000 ) ;
#38320=CARTESIAN_POINT ( 'NONE',  ( -9.999999999999998224, 5.773502691896259087, -35.87499999999995737 ) ) ;
#38323=CARTESIAN_POINT ( 'NONE',  ( 7.644554776091147741E-16, 12.48450537969573659, -161.4687500020484094 ) ) ;
#38324=CARTESIAN_POINT ( 'NONE',  ( -5.405949406250003975, -9.363379034771801557, -166.8437500020484094 ) ) ;
#38326=CARTESIAN_POINT ( 'NONE',  ( 9.999999999999996447, -5.773502691896262640, -195.6250000000000284 ) ) ;
#38332=CARTESIAN_POINT ( 'NONE',  ( -10.81189881249999729, 1.324075727343319199E-15, -71.28125000204838102 ) ) ;
#38334=CARTESIAN_POINT ( 'NONE',  ( 9.999999999999996447, -5.773502691896262640, -126.6250000000000000 ) ) ;
#38335=ORIENTED_EDGE ( 'NONE', *, *, #32988, .T. ) ;
#38336=CARTESIAN_POINT ( 'NONE',  ( 10.81189881249999729, 0.000000000000000000, -153.0312500020484094 ) ) ;
#38337=CARTESIAN_POINT ( 'NONE',  ( 10.81189881249999729, 0.000000000000000000, -166.5312500020484094 ) ) ;
#38340=CARTESIAN_POINT ( 'NONE',  ( 5.405949406249999534, 9.363379034771803333, -100.0937500020483810 ) ) ;
#38343=CARTESIAN_POINT ( 'NONE',  ( -10.81189881249999729, 6.242252689847871849, -197.2187500020484379 ) ) ;
#38347=LINE ( 'NONE', #1090, #37600 ) ;
#38348=CARTESIAN_POINT ( 'NONE',  ( 10.81189881249999907, 6.242252689847868297, -89.90625000204839523 ) ) ;
#38351=CARTESIAN_POINT ( 'NONE',  ( 4.999999999999992006, -8.660254037844389075, -70.12500000409677625 ) ) ;
#38353=CARTESIAN_POINT ( 'NONE',  ( -10.81189881249999729, 1.324075727343319199E-15, -27.59375000204836326 ) ) ;
#38357=CARTESIAN_POINT ( 'NONE',  ( -5.405949406250003975, -9.363379034771801557, -17.03125000204835970 ) ) ;
#38366=VERTEX_POINT ( 'NONE', #31416 ) ;
#38372=EDGE_CURVE ( 'NONE', #21752, #6776, #4085, .T. ) ;
#38375=CARTESIAN_POINT ( 'NONE',  ( 9.999999999999998224, 0.000000000000000000, -173.3750000040968189 ) ) ;
#38376=( BOUNDED_CURVE ( )  B_SPLINE_CURVE ( 2, ( #1068, #33245, #11189, #17440, #27175, #40528, #16800 ),
 .UNSPECIFIED., .F., .F. ) 
 B_SPLINE_CURVE_WITH_KNOTS ( ( 3, 2, 2, 3 ),
 ( 0.4626865671641792743, 0.4639303482587066596, 0.4651741293532339339, 0.4664179104477613191 ),
 .UNSPECIFIED. ) 
 CURVE ( )  GEOMETRIC_REPRESENTATION_ITEM ( )  RATIONAL_B_SPLINE_CURVE ( ( 0.9999999999999820144, 0.8660254037844566932, 1.000000000000000000, 0.8660254037844387076, 1.000000000000000000, 0.8660254037844267172, 1.000000000000011990 ) ) 
 REPRESENTATION_ITEM ( '' )  );
#38378=CARTESIAN_POINT ( 'NONE',  ( 10.81189881249999907, 6.242252689847868297, -163.4062500020484094 ) ) ;
#38380=DIRECTION ( 'NONE',  ( -0.000000000000000000, -0.000000000000000000, -1.000000000000000000 ) ) ;
#38382=CARTESIAN_POINT ( 'NONE',  ( -5.405949406249996869, 9.363379034771805109, -89.34375000204838102 ) ) ;
#38383=CARTESIAN_POINT ( 'NONE',  ( -5.405949406250003975, -9.363379034771801557, -193.8437500020484094 ) ) ;
#38384=CARTESIAN_POINT ( 'NONE',  ( 5.405949406249999534, 9.363379034771803333, -89.78125000204838102 ) ) ;
#38389=CARTESIAN_POINT ( 'NONE',  ( -10.81189881249999729, 6.242252689847871849, -171.9062500020484094 ) ) ;
#38390=CARTESIAN_POINT ( 'NONE',  ( -10.81189881249999907, -6.242252689847864744, -189.6562500020484094 ) ) ;
#38392=CARTESIAN_POINT ( 'NONE',  ( 4.999999999999992006, -8.660254037844389075, -164.6250000040967905 ) ) ;
#38394=CARTESIAN_POINT ( 'NONE',  ( 5.405949406249999534, 9.363379034771803333, -11.59375000204834727 ) ) ;
#38396=CARTESIAN_POINT ( 'NONE',  ( 7.644554776091147741E-16, 12.48450537969573659, -119.4687500020483952 ) ) ;
#38398=CARTESIAN_POINT ( 'NONE',  ( 10.81189881249999551, -6.242252689847874514, -19.65625000204837747 ) ) ;
#38400=DIRECTION ( 'NONE',  ( -0.000000000000000000, -0.000000000000000000, -1.000000000000000000 ) ) ;
#38401=CARTESIAN_POINT ( 'NONE',  ( -10.81189881249999729, 1.324075727343319199E-15, -114.7812500020483952 ) ) ;
#38404=CARTESIAN_POINT ( 'NONE',  ( -9.999999999999998224, 1.224646799147353059E-15, -88.62500000409677625 ) ) ;
#38407=CARTESIAN_POINT ( 'NONE',  ( -2.293366432827344421E-15, -12.48450537969573659, -48.21875000204836681 ) ) ;
#38408=ORIENTED_EDGE ( 'NONE', *, *, #32845, .F. ) ;
#38413=CARTESIAN_POINT ( 'NONE',  ( 9.999999999999996447, -5.773502691896262640, -17.50000000409676559 ) ) ;
#38417=ORIENTED_EDGE ( 'NONE', *, *, #34413, .F. ) ;
#38425=ORIENTED_EDGE ( 'NONE', *, *, #24323, .F. ) ;
#38429=CARTESIAN_POINT ( 'NONE',  ( -2.293366432827344421E-15, -12.48450537969573659, -187.9062500020484094 ) ) ;
#38432=CARTESIAN_POINT ( 'NONE',  ( -5.405949406250003975, -9.363379034771801557, -108.3437500020483810 ) ) ;
#38433=CARTESIAN_POINT ( 'NONE',  ( -9.999999999999998224, 1.224646799147353059E-15, -150.1250000040967905 ) ) ;
#38434=CARTESIAN_POINT ( 'NONE',  ( 10.81189881249999729, 0.000000000000000000, -114.0312500020483952 ) ) ;
#38436=CARTESIAN_POINT ( 'NONE',  ( 5.405949406249992428, -9.363379034771808662, -126.0937500020483668 ) ) ;
#38438=CARTESIAN_POINT ( 'NONE',  ( -4.999999999999996447, 8.660254037844387298, -148.5000000000000000 ) ) ;
#38439=CARTESIAN_POINT ( 'NONE',  ( 5.000000000000000000, 8.660254037844385522, -12.24999999999995559 ) ) ;
#38442=CARTESIAN_POINT ( 'NONE',  ( -2.121150477449813534E-15, -11.54700538379251284, -187.2500000040967905 ) ) ;
#38445=CARTESIAN_POINT ( 'NONE',  ( 7.644554776091147741E-16, 12.48450537969573659, -36.96875000204835260 ) ) ;
#38447=CARTESIAN_POINT ( 'NONE',  ( 5.405949406249999534, 9.363379034771803333, -145.0937500020483810 ) ) ;
#38450=CARTESIAN_POINT ( 'NONE',  ( -4.999999999999996447, 8.660254037844387298, -136.5000000000000000 ) ) ;
#38451=CARTESIAN_POINT ( 'NONE',  ( -9.999999999999998224, 5.773502691896259087, -76.37499999999998579 ) ) ;
#38452=CARTESIAN_POINT ( 'NONE',  ( -10.81189881249999907, -6.242252689847864744, -141.6562500020483810 ) ) ;
#38456=CARTESIAN_POINT ( 'NONE',  ( 10.00000000000000000, 5.773502691896255534, -117.7500000040967905 ) ) ;
#38458=CARTESIAN_POINT ( 'NONE',  ( -10.81189881249999729, 6.242252689847871849, -74.21875000204836681 ) ) ;
#38461=( BOUNDED_CURVE ( )  B_SPLINE_CURVE ( 2, ( #2866, #15997, #2246, #8916, #5250, #29192, #28567 ),
 .UNSPECIFIED., .F., .F. ) 
 B_SPLINE_CURVE_WITH_KNOTS ( ( 3, 2, 2, 3 ),
 ( 0.3134328358208955390, 0.3146766169154229242, 0.3159203980099503650, 0.3171641791044778058 ),
 .UNSPECIFIED. ) 
 CURVE ( )  GEOMETRIC_REPRESENTATION_ITEM ( )  RATIONAL_B_SPLINE_CURVE ( ( 1.000000000000000000, 0.8660254037844387076, 1.000000000000000000, 0.8660254037844387076, 1.000000000000000000, 0.8660254037844207220, 1.000000000000017986 ) ) 
 REPRESENTATION_ITEM ( '' )  );
#38462=CARTESIAN_POINT ( 'NONE',  ( -9.999999999999872102, -5.773502691896326589, -157.5000000040968189 ) ) ;
#38463=CARTESIAN_POINT ( 'NONE',  ( 10.81189881249999551, -6.242252689847874514, -37.65625000204836681 ) ) ;
#38470=AXIS2_PLACEMENT_3D ( 'NONE', #34682, #20851, #21280 ) ;
#38473=CYLINDRICAL_SURFACE ( 'NONE', #29076, 9.999999999999998224 ) ;
#38480=CARTESIAN_POINT ( 'NONE',  ( -5.405949406249996869, 9.363379034771805109, -134.3437500020484094 ) ) ;
#38481=CARTESIAN_POINT ( 'NONE',  ( 10.81189881249999551, -6.242252689847874514, -136.6562500020484094 ) ) ;
#38483=CARTESIAN_POINT ( 'NONE',  ( 10.81189881249999729, 0.000000000000000000, -146.8437500020483810 ) ) ;
#38486=CARTESIAN_POINT ( 'NONE',  ( 5.000000000000000000, 8.660254037844385522, -172.7500000000000284 ) ) ;
#38488=CARTESIAN_POINT ( 'NONE',  ( 9.999999999999998224, 1.224646799147353059E-15, -99.99999999999998579 ) ) ;
#38491=CARTESIAN_POINT ( 'NONE',  ( -10.81189881249999729, 6.242252689847871849, -173.2187500020483810 ) ) ;
#38495=CARTESIAN_POINT ( 'NONE',  ( 5.405949406249992428, -9.363379034771808662, -34.78125000204837391 ) ) ;
#38497=CARTESIAN_POINT ( 'NONE',  ( 7.070501591499377789E-16, 11.54700538379251284, -99.12500000000000000 ) ) ;
#38500=CARTESIAN_POINT ( 'NONE',  ( -10.81189881249999729, -6.242252689847864744, -116.1562500020483952 ) ) ;
#38501=CARTESIAN_POINT ( 'NONE',  ( 7.070501591499377789E-16, 11.54700538379251284, -140.0000000040968189 ) ) ;
#38506=AXIS2_PLACEMENT_3D ( 'NONE', #10774, #17453, #23963 ) ;
#38507=CARTESIAN_POINT ( 'NONE',  ( -10.81189881249999907, -6.242252689847864744, -65.15625000204838102 ) ) ;
#38528=CARTESIAN_POINT ( 'NONE',  ( 9.999999999999996447, -5.773502691896262640, -33.62499999999995737 ) ) ;
#38531=CARTESIAN_POINT ( 'NONE',  ( 5.405949406249992428, -9.363379034771808662, -157.5937500020483810 ) ) ;
#38532=CARTESIAN_POINT ( 'NONE',  ( 10.81189881249999551, -6.242252689847874514, -166.4687500020483810 ) ) ;
#38535=CARTESIAN_POINT ( 'NONE',  ( -2.121150477449813534E-15, -11.54700538379251284, -195.8750000000000284 ) ) ;
#38536=VECTOR ( 'NONE', #39599, 1000.000000000000000 ) ;
#38541=CARTESIAN_POINT ( 'NONE',  ( 10.81189881249999907, 6.242252689847868297, -64.40625000204839523 ) ) ;
#38543=CARTESIAN_POINT ( 'NONE',  ( 4.999999999999992006, -8.660254037844389075, -120.7500000000000000 ) ) ;
#38544=ORIENTED_EDGE ( 'NONE', *, *, #32330, .F. ) ;
#38545=CARTESIAN_POINT ( 'NONE',  ( -10.81189881249999729, 1.324075727343319199E-15, -141.7812500020483810 ) ) ;
#38546=CARTESIAN_POINT ( 'NONE',  ( 7.644554776091147741E-16, 12.48450537969573659, -164.6562500020484094 ) ) ;
#38547=CARTESIAN_POINT ( 'NONE',  ( 22.00000000000000711, 2.877919977996280320E-15, -99.99999999999998579 ) ) ;
#38549=CARTESIAN_POINT ( 'NONE',  ( 10.81189881249999729, 0.000000000000000000, -88.34375000204838102 ) ) ;
#38550=EDGE_LOOP ( 'NONE', ( #21630, #32071, #12292, #26985, #7468, #31217, #36503, #28614, #8652, #7181, #24956, #15320, #20514, #25049, #40152, #29937, #297, #13756, #26581, #887, #3101, #35831, #20945, #22425, #33442, #5621, #41957, #21696, #32841, #7256, #18277, #30887, #34556, #37729, #34919, #28641, #24524, #28497, #14765, #42329, #34392, #2389, #23287, #31639, #10582, #31621, #38899, #26371, #8214, #38900, #10908, #39840, #26477, #637, #21597, #17844, #25404, #34673, #40977, #42228, #37457, #31948, #30287, #11648, #42212, #24515, #19185, #37163, #20777, #14394, #14177, #26320, #37921, #9999, #38335, #11273, #3119, #17467, #946, #21697, #18479, #18655, #29085, #41643, #36975, #31666, #1051, #36162, #13433, #36236, #9256, #8476, #19823, #1699, #34762, #5400, #8367, #17693, #13436, #34346, #19410, #16342, #25791, #13018, #18882, #1576, #14827, #18133, #142, #1745 ) ) ;
#38552=CARTESIAN_POINT ( 'NONE',  ( 10.81189881249999907, 6.242252689847868297, -193.2187500020484094 ) ) ;
#38556=CARTESIAN_POINT ( 'NONE',  ( 10.81189881249999729, 0.000000000000000000, -96.03125000204838102 ) ) ;
#38558=CARTESIAN_POINT ( 'NONE',  ( -9.999999999999998224, 1.224646799147353059E-15, -67.62500000409676204 ) ) ;
#38560=CARTESIAN_POINT ( 'NONE',  ( -10.81189881249999729, 1.324075727343319199E-15, -23.09375000204835615 ) ) ;
#38563=CARTESIAN_POINT ( 'NONE',  ( -10.81189881249999729, 6.242252689847871849, -20.40625000204837391 ) ) ;
#38565=CARTESIAN_POINT ( 'NONE',  ( -10.00000000000076916, 5.773502691895813221, -136.7500000040967620 ) ) ;
#38570=VECTOR ( 'NONE', #14173, 1000.000000000000000 ) ;
#38576=AXIS2_PLACEMENT_3D ( 'NONE', #14528, #34847, #9147 ) ;
#38581=CARTESIAN_POINT ( 'NONE',  ( 6.703084383986223749, 8.205311082841122428, -100.0000000000000000 ) ) ;
#38587=CARTESIAN_POINT ( 'NONE',  ( 5.405949406249999534, 9.363379034771803333, -152.7812500020484094 ) ) ;
#38593=CARTESIAN_POINT ( 'NONE',  ( 5.405949406249999534, 9.363379034771803333, -82.09375000204836681 ) ) ;
#38594=CARTESIAN_POINT ( 'NONE',  ( -10.81189881249999729, 6.242252689847871849, -95.40625000204838102 ) ) ;
#38598=CARTESIAN_POINT ( 'NONE',  ( -2.293366432827344421E-15, -12.48450537969573659, -175.9062500020484379 ) ) ;
#38599=CARTESIAN_POINT ( 'NONE',  ( 7.644554776091147741E-16, 12.48450537969573659, -190.1562500020484094 ) ) ;
#38602=CARTESIAN_POINT ( 'NONE',  ( 9.999999999999996447, -5.773502691896262640, -164.5000000040967905 ) ) ;
#38604=CARTESIAN_POINT ( 'NONE',  ( 7.644554776091147741E-16, 12.48450537969573659, -12.96875000204836503 ) ) ;
#38605=CARTESIAN_POINT ( 'NONE',  ( 9.999999999999742428, 5.773502691896404748, -162.7500000040968189 ) ) ;
#38606=CARTESIAN_POINT ( 'NONE',  ( -5.405949406250003975, -9.363379034771801557, -118.8437500020483810 ) ) ;
#38608=CARTESIAN_POINT ( 'NONE',  ( -10.81189881249999907, -6.242252689847864744, -17.15625000204837391 ) ) ;
#38611=DIRECTION ( 'NONE',  ( -1.000000000000000000, 0.000000000000000000, 0.000000000000000000 ) ) ;
#38612=CARTESIAN_POINT ( 'NONE',  ( -10.81189881249999729, 1.324075727343319199E-15, -119.2812500020483952 ) ) ;
#38615=CARTESIAN_POINT ( 'NONE',  ( -9.999999999999998224, 5.773502691896259087, -90.25000000409676204 ) ) ;
#38618=CARTESIAN_POINT ( 'NONE',  ( 10.81189881249999907, 6.242252689847868297, -47.71875000204835970 ) ) ;
#38625=CARTESIAN_POINT ( 'NONE',  ( -2.121150477449813534E-15, -11.54700538379251284, -23.75000000409676915 ) ) ;
#38631=ORIENTED_EDGE ( 'NONE', *, *, #19278, .F. ) ;
#38639=CARTESIAN_POINT ( 'NONE',  ( 9.999999999999998224, 0.000000000000000000, -125.3750000040967905 ) ) ;
#38644=CARTESIAN_POINT ( 'NONE',  ( -2.293366432827344421E-15, -12.48450537969573659, -190.9062500020483810 ) ) ;
#38647=CARTESIAN_POINT ( 'NONE',  ( -2.293366432827344421E-15, -12.48450537969573659, -111.2187500020483668 ) ) ;
#38649=CARTESIAN_POINT ( 'NONE',  ( -5.405949406250003975, -9.363379034771801557, -116.0312500020483952 ) ) ;
#38651=CARTESIAN_POINT ( 'NONE',  ( -5.405949406250003975, -9.363379034771801557, -120.3437500020483952 ) ) ;
#38654=CARTESIAN_POINT ( 'NONE',  ( -10.00000000000000000, -5.773502691896251982, -137.6250000000000000 ) ) ;
#38655=CARTESIAN_POINT ( 'NONE',  ( -10.00000000000000000, -5.773502691896251982, -14.62499999999996980 ) ) ;
#38658=CARTESIAN_POINT ( 'NONE',  ( -5.000000000000003553, -8.660254037844383745, -191.8750000040967905 ) ) ;
#38660=CARTESIAN_POINT ( 'NONE',  ( 7.644554776091147741E-16, 12.48450537969573659, -35.46875000204835260 ) ) ;
#38661=CARTESIAN_POINT ( 'NONE',  ( 9.999999999999998224, 0.000000000000000000, -111.8750000040967763 ) ) ;
#38662=CARTESIAN_POINT ( 'NONE',  ( -10.81189881249999729, 6.242252689847871849, -144.7187500020483810 ) ) ;
#38664=CARTESIAN_POINT ( 'NONE',  ( 9.999999999999998224, 0.000000000000000000, -146.0000000000000000 ) ) ;
#38665=CARTESIAN_POINT ( 'NONE',  ( -10.00000000000000000, -5.773502691896251982, -65.62499999999998579 ) ) ;
#38666=CARTESIAN_POINT ( 'NONE',  ( 7.644554776091147741E-16, 12.48450537969573659, -139.1562500020483810 ) ) ;
#38671=CARTESIAN_POINT ( 'NONE',  ( -10.00000000000000000, -5.773502691896251982, -115.5000000040967905 ) ) ;
#38673=CARTESIAN_POINT ( 'NONE',  ( 10.81189881249999729, 0.000000000000000000, -73.34375000204838102 ) ) ;
#38678=CARTESIAN_POINT ( 'NONE',  ( 4.999999999999992006, -8.660254037844389075, -131.6250000040967620 ) ) ;
#38679=CARTESIAN_POINT ( 'NONE',  ( 10.81189881249999907, 6.242252689847868297, -38.90625000204836681 ) ) ;
#38685=ORIENTED_EDGE ( 'NONE', *, *, #19874, .T. ) ;
#38697=CARTESIAN_POINT ( 'NONE',  ( 7.644554776091147741E-16, 12.48450537969573659, -132.9687500020483810 ) ) ;
#38698=CARTESIAN_POINT ( 'NONE',  ( 10.81189881249999551, -6.242252689847874514, -139.6562500020484094 ) ) ;
#38700=CARTESIAN_POINT ( 'NONE',  ( -10.81189881249999729, 1.324075727343319199E-15, -146.0937500020483810 ) ) ;
#38701=FACE_OUTER_BOUND ( 'NONE', #33861, .T. ) ;
#38703=CARTESIAN_POINT ( 'NONE',  ( 10.00000000000000000, 5.773502691896255534, -165.3749999999999716 ) ) ;
#38704=EDGE_CURVE ( 'NONE', #17267, #5246, #16458, .T. ) ;
#38706=CARTESIAN_POINT ( 'NONE',  ( -9.999999999999998224, 1.224646799147353059E-15, -114.1250000040967763 ) ) ;
#38708=CARTESIAN_POINT ( 'NONE',  ( -5.405949406249996869, 9.363379034771805109, -65.34375000204836681 ) ) ;
#38710=CARTESIAN_POINT ( 'NONE',  ( 10.81189881249999907, 6.242252689847868297, -172.2187500020483810 ) ) ;
#38715=CARTESIAN_POINT ( 'NONE',  ( 5.405949406249992428, -9.363379034771808662, -39.28125000204838102 ) ) ;
#38717=CARTESIAN_POINT ( 'NONE',  ( 5.000000000000000000, 8.660254037844385522, -99.24999999999998579 ) ) ;
#38719=CARTESIAN_POINT ( 'NONE',  ( 10.81189881249999551, -6.242252689847874514, -118.6562500020483952 ) ) ;
#38720=CARTESIAN_POINT ( 'NONE',  ( -2.121150477449813534E-15, -11.54700538379251284, -139.2500000040967905 ) ) ;
#38724=CARTESIAN_POINT ( 'NONE',  ( -9.999999999999742428, -5.773502691896402084, -160.1250000000000284 ) ) ;
#38725=CARTESIAN_POINT ( 'NONE',  ( 10.81189881249999729, 0.000000000000000000, -60.03125000204836681 ) ) ;
#38728=FACE_OUTER_BOUND ( 'NONE', #15831, .T. ) ;
#38738=CARTESIAN_POINT ( 'NONE',  ( -2.121150477449813534E-15, -11.54700538379251284, -100.2500000040967905 ) ) ;
#38742=LINE ( 'NONE', #11976, #14836 ) ;
#38747=CARTESIAN_POINT ( 'NONE',  ( -5.000000000000003553, -8.660254037844383745, -30.99999999999997158 ) ) ;
#38750=CARTESIAN_POINT ( 'NONE',  ( 10.81189881249999551, -6.242252689847874514, -155.9687500020484094 ) ) ;
#38753=CARTESIAN_POINT ( 'NONE',  ( 10.81189881249999729, 0.000000000000000000, -170.8437500020484094 ) ) ;
#38756=CARTESIAN_POINT ( 'NONE',  ( 9.999999999999998224, 0.000000000000000000, -126.5000000000000000 ) ) ;
#38757=CARTESIAN_POINT ( 'NONE',  ( -5.000000000000003553, -8.660254037844383745, -199.0000000000000000 ) ) ;
#38762=CARTESIAN_POINT ( 'NONE',  ( -2.293366432827344421E-15, -12.48450537969573659, -63.40625000204838813 ) ) ;
#38764=CARTESIAN_POINT ( 'NONE',  ( 9.999999999999996447, -5.773502691896262640, -125.1249999999999858 ) ) ;
#38766=CARTESIAN_POINT ( 'NONE',  ( -5.405949406250003975, -9.363379034771801557, -144.5312500020483810 ) ) ;
#38767=CARTESIAN_POINT ( 'NONE',  ( 5.405949406249992428, -9.363379034771808662, -156.2812500020484094 ) ) ;
#38770=CARTESIAN_POINT ( 'NONE',  ( 8.660254119780192994, -4.999999858083012505, -99.99999999999998579 ) ) ;
#38771=CARTESIAN_POINT ( 'NONE',  ( 10.81189881249999551, -6.242252689847874514, -89.96875000204838102 ) ) ;
#38774=CARTESIAN_POINT ( 'NONE',  ( 7.644554776091147741E-16, 12.48450537969573659, -186.9687500020483810 ) ) ;
#38778=CARTESIAN_POINT ( 'NONE',  ( -5.405949406249996869, 9.363379034771805109, -85.03125000204838102 ) ) ;
#38780=CARTESIAN_POINT ( 'NONE',  ( 9.999999999999996447, -5.773502691896262640, -56.50000000409677625 ) ) ;
#38782=CARTESIAN_POINT ( 'NONE',  ( -2.293366432827344421E-15, -12.48450537969573659, -16.71875000204836681 ) ) ;
#38785=CARTESIAN_POINT ( 'NONE',  ( 5.405949406249992428, -9.363379034771808662, -18.28125000204835970 ) ) ;
#38789=FACE_OUTER_BOUND ( 'NONE', #21688, .T. ) ;
#38802=CARTESIAN_POINT ( 'NONE',  ( 9.865189697491926424, 3.226167097173905152, -100.0000000000000000 ) ) ;
#38803=CARTESIAN_POINT ( 'NONE',  ( -9.999999999999998224, 1.224646799147353059E-15, -127.6250000040967620 ) ) ;
#38805=CARTESIAN_POINT ( 'NONE',  ( 10.81189881249999729, 0.000000000000000000, -159.0312500020484094 ) ) ;
#38810=CARTESIAN_POINT ( 'NONE',  ( 5.405949406249999534, 9.363379034771803333, -76.09375000204838102 ) ) ;
#38811=CARTESIAN_POINT ( 'NONE',  ( -10.81189881249999907, -6.242252689847864744, -83.15625000204836681 ) ) ;
#38814=CARTESIAN_POINT ( 'NONE',  ( 10.81189881249999729, 6.242252689847867408, -164.9062500020484094 ) ) ;
#38815=CARTESIAN_POINT ( 'NONE',  ( -10.81189881249999729, 1.324075727343319199E-15, -179.2812500020484094 ) ) ;
#38817=CARTESIAN_POINT ( 'NONE',  ( -5.000000000000003553, -8.660254037844383745, -155.8750000040967905 ) ) ;
#38819=CARTESIAN_POINT ( 'NONE',  ( 10.81189881249999907, 6.242252689847868297, -4.218750002048355263 ) ) ;
#38820=CARTESIAN_POINT ( 'NONE',  ( -5.405949406250003975, -9.363379034771801557, -111.3437500020483810 ) ) ;
#38822=CARTESIAN_POINT ( 'NONE',  ( 10.81189881249999907, 6.242252689847868297, -8.906250002048366810 ) ) ;
#38825=CARTESIAN_POINT ( 'NONE',  ( 5.405949406249992428, -9.363379034771808662, -112.7812500020483952 ) ) ;
#38827=ORIENTED_EDGE ( 'NONE', *, *, #37201, .T. ) ;
#38828=CARTESIAN_POINT ( 'NONE',  ( -2.121150477449813534E-15, -11.54700538379251284, -89.75000000409677625 ) ) ;
#38829=CARTESIAN_POINT ( 'NONE',  ( 10.00000000000051159, -5.773502691895965988, -101.1249999999999858 ) ) ;
#38830=CARTESIAN_POINT ( 'NONE',  ( -5.405949406249996869, 9.363379034771805109, -47.34375000204838102 ) ) ;
#38831=ORIENTED_EDGE ( 'NONE', *, *, #31492, .T. ) ;
#38833=EDGE_CURVE ( 'NONE', #3790, #34380, #11499, .T. ) ;
#38836=CARTESIAN_POINT ( 'NONE',  ( 9.999999999999998224, 0.000000000000000000, -17.37500000409675138 ) ) ;
#38837=EDGE_CURVE ( 'NONE', #7311, #10904, #20334, .T. ) ;
#38840=ORIENTED_EDGE ( 'NONE', *, *, #34933, .T. ) ;
#38852=CARTESIAN_POINT ( 'NONE',  ( 10.81189881249999729, 0.000000000000000000, -180.0312500020483810 ) ) ;
#38857=CARTESIAN_POINT ( 'NONE',  ( -5.405949406250003975, -9.363379034771801557, -105.3437500020483810 ) ) ;
#38858=CARTESIAN_POINT ( 'NONE',  ( -5.405949406250003975, -9.363379034771801557, -111.5312500020483810 ) ) ;
#38860=CARTESIAN_POINT ( 'NONE',  ( 5.405949406249999534, 9.363379034771803333, -122.5937500020483952 ) ) ;
#38862=CARTESIAN_POINT ( 'NONE',  ( -9.999999999999998224, 1.224646799147353059E-15, -170.7500000000000000 ) ) ;
#38863=CARTESIAN_POINT ( 'NONE',  ( 7.070501591499377789E-16, 11.54700538379251284, -142.6250000000000000 ) ) ;
#38864=CARTESIAN_POINT ( 'NONE',  ( -9.999999999999998224, 1.224646799147353059E-15, -2.749999999999974687 ) ) ;
#38867=CARTESIAN_POINT ( 'NONE',  ( 9.999999999999996447, -5.773502691896262640, -188.5000000040968189 ) ) ;
#38869=CARTESIAN_POINT ( 'NONE',  ( -5.405949406250003975, -9.363379034771801557, -34.84375000204836681 ) ) ;
#38870=CARTESIAN_POINT ( 'NONE',  ( 5.000000000000000000, 8.660254037844385522, -149.1250000040967905 ) ) ;
#38871=CARTESIAN_POINT ( 'NONE',  ( -5.405949406249996869, 9.363379034771805109, -137.3437500020484094 ) ) ;
#38873=CARTESIAN_POINT ( 'NONE',  ( -2.121150477449813534E-15, -11.54700538379251284, -147.8750000000000000 ) ) ;
#38874=CARTESIAN_POINT ( 'NONE',  ( -5.000000000000003553, -8.660254037844383745, -65.49999999999997158 ) ) ;
#38875=CARTESIAN_POINT ( 'NONE',  ( 5.405949406249992428, -9.363379034771808662, -136.7812500020483810 ) ) ;
#38879=CARTESIAN_POINT ( 'NONE',  ( -10.00000000000025580, 5.773502691896109873, -120.2500000040967905 ) ) ;
#38880=CARTESIAN_POINT ( 'NONE',  ( -9.999999999999998224, 1.224646799147353059E-15, -120.1250000040967905 ) ) ;
#38882=CARTESIAN_POINT ( 'NONE',  ( -5.405949406249996869, 9.363379034771805109, -72.84375000204838102 ) ) ;
#38887=CARTESIAN_POINT ( 'NONE',  ( -22.00000000000000711, 0.000000000000000000, -99.99999999999998579 ) ) ;
#38888=CARTESIAN_POINT ( 'NONE',  ( -10.81189881249999907, -6.242252689847864744, -38.15625000204835970 ) ) ;
#38890=( BOUNDED_CURVE ( )  B_SPLINE_CURVE ( 2, ( #27521, #33790, #987, #13686, #16930, #14105, #20185 ),
 .UNSPECIFIED., .F., .F. ) 
 B_SPLINE_CURVE_WITH_KNOTS ( ( 3, 2, 2, 3 ),
 ( 0.2052238805970149627, 0.2064676616915423202, 0.2077114427860697055, 0.2089552238805970630 ),
 .UNSPECIFIED. ) 
 CURVE ( )  GEOMETRIC_REPRESENTATION_ITEM ( )  RATIONAL_B_SPLINE_CURVE ( ( 0.9999999999999970024, 0.8660254037844417052, 1.000000000000000000, 0.8660254037844387076, 1.000000000000000000, 0.8660254037844327124, 1.000000000000005995 ) ) 
 REPRESENTATION_ITEM ( '' )  );
#38891=CARTESIAN_POINT ( 'NONE',  ( -9.999999999999998224, 1.224646799147353059E-15, -175.6250000040968189 ) ) ;
#38896=CARTESIAN_POINT ( 'NONE',  ( -9.999999999999998224, 1.224646799147353059E-15, -121.2500000000000000 ) ) ;
#38897=ORIENTED_EDGE ( 'NONE', *, *, #3505, .F. ) ;
#38898=( BOUNDED_CURVE ( )  B_SPLINE_CURVE ( 2, ( #1144, #11474, #5026, #37393, #4799, #27684, #14489 ),
 .UNSPECIFIED., .F., .F. ) 
 B_SPLINE_CURVE_WITH_KNOTS ( ( 3, 2, 2, 3 ),
 ( 0.2201492537313433639, 0.2213930348258707215, 0.2226368159203980790, 0.2238805970149254365 ),
 .UNSPECIFIED. ) 
 CURVE ( )  GEOMETRIC_REPRESENTATION_ITEM ( )  RATIONAL_B_SPLINE_CURVE ( ( 0.9999999999999910072, 0.8660254037844477004, 1.000000000000000000, 0.8660254037844387076, 1.000000000000000000, 0.8660254037844327124, 1.000000000000005995 ) ) 
 REPRESENTATION_ITEM ( '' )  );
#38899=ORIENTED_EDGE ( 'NONE', *, *, #5364, .T. ) ;
#38900=ORIENTED_EDGE ( 'NONE', *, *, #30852, .T. ) ;
#38902=CARTESIAN_POINT ( 'NONE',  ( -9.999999999999998224, 1.224646799147353059E-15, -177.1250000040968189 ) ) ;
#38908=CARTESIAN_POINT ( 'NONE',  ( 10.00000000000051159, -5.773502691895965988, -176.1250000000000000 ) ) ;
#38909=CARTESIAN_POINT ( 'NONE',  ( 7.644554776091147741E-16, 12.48450537969573659, -129.9687500020483810 ) ) ;
#38910=CARTESIAN_POINT ( 'NONE',  ( -10.81189881249999907, -6.242252689847864744, -141.6562500020483810 ) ) ;
#38912=CARTESIAN_POINT ( 'NONE',  ( 10.81189881249999551, -6.242252689847874514, -148.4687500020484094 ) ) ;
#38915=CARTESIAN_POINT ( 'NONE',  ( 4.999999999999992006, -8.660254037844389075, -167.2500000000000000 ) ) ;
#38918=CARTESIAN_POINT ( 'NONE',  ( 5.405949406249999534, 9.363379034771803333, -58.09375000204835970 ) ) ;
#38919=CARTESIAN_POINT ( 'NONE',  ( 9.999999999999998224, 1.224646799147353059E-15, -99.99999999999998579 ) ) ;
#38920=CARTESIAN_POINT ( 'NONE',  ( -10.81189881249999729, 6.242252689847871849, -168.7187500020483810 ) ) ;
#38925=CARTESIAN_POINT ( 'NONE',  ( -4.999999999999996447, 8.660254037844387298, -94.49999999999998579 ) ) ;
#38927=CARTESIAN_POINT ( 'NONE',  ( -5.405949406249996869, 9.363379034771805109, -115.0312500020483952 ) ) ;
#38928=CARTESIAN_POINT ( 'NONE',  ( -10.00000000000000000, -5.773502691896251982, -144.0000000040967905 ) ) ;
#38929=CARTESIAN_POINT ( 'NONE',  ( -4.999999999999996447, 8.660254037844387298, -159.0000000000000000 ) ) ;
#38933=CARTESIAN_POINT ( 'NONE',  ( -2.293366432827344421E-15, -12.48450537969573659, -58.90625000204838102 ) ) ;
#38942=EDGE_CURVE ( 'NONE', #32646, #28517, #12884, .T. ) ;
#38947=ORIENTED_EDGE ( 'NONE', *, *, #13590, .T. ) ;
#38955=CARTESIAN_POINT ( 'NONE',  ( -10.00000000000000000, -5.773502691896251982, -26.62499999999998224 ) ) ;
#38959=CARTESIAN_POINT ( 'NONE',  ( 7.644554776091147741E-16, 12.48450537969573659, -155.4687500020484094 ) ) ;
#38960=CARTESIAN_POINT ( 'NONE',  ( -10.81189881249999729, 6.242252689847871849, -168.7187500020483810 ) ) ;
#38963=CARTESIAN_POINT ( 'NONE',  ( 9.999999999999998224, 0.000000000000000000, -183.5000000000000000 ) ) ;
#38968=CARTESIAN_POINT ( 'NONE',  ( -5.405949406249996869, 9.363379034771805109, -58.03125000204836681 ) ) ;
#38970=CARTESIAN_POINT ( 'NONE',  ( -4.999999999999996447, 8.660254037844387298, -112.4999999999999858 ) ) ;
#38972=CARTESIAN_POINT ( 'NONE',  ( 5.405949406249999534, 9.363379034771803333, -143.7812500020483810 ) ) ;
#38973=CARTESIAN_POINT ( 'NONE',  ( -5.405949406249996869, 9.363379034771805109, -154.0312500020484094 ) ) ;
#38976=CARTESIAN_POINT ( 'NONE',  ( -10.81189881249999729, 6.242252689847871849, -90.71875000204838102 ) ) ;
#38977=ORIENTED_EDGE ( 'NONE', *, *, #23293, .F. ) ;
#38979=CARTESIAN_POINT ( 'NONE',  ( -10.81189881249999907, -6.242252689847864744, -189.4687500020484094 ) ) ;
#38982=CARTESIAN_POINT ( 'NONE',  ( 10.81189881249999907, 6.242252689847868297, -85.40625000204839523 ) ) ;
#38985=CARTESIAN_POINT ( 'NONE',  ( -10.00000000000000000, -5.773502691896251982, -63.00000000409677625 ) ) ;
#38986=CARTESIAN_POINT ( 'NONE',  ( 7.644554776091147741E-16, 12.48450537969573659, -14.46875000204836503 ) ) ;
#38989=CARTESIAN_POINT ( 'NONE',  ( -10.81189881249999729, 1.324075727343319199E-15, -12.78125000204835615 ) ) ;
#38992=VECTOR ( 'NONE', #99, 1000.000000000000000 ) ;
#39010=CARTESIAN_POINT ( 'NONE',  ( -9.999999999999998224, 1.224646799147353059E-15, -124.2500000000000000 ) ) ;
#39011=PLANE ( 'NONE',  #41161 ) ;
#39012=CARTESIAN_POINT ( 'NONE',  ( 10.81189881249999729, 0.000000000000000000, -156.0312500020484094 ) ) ;
#39014=CARTESIAN_POINT ( 'NONE',  ( 9.999999999999998224, 0.000000000000000000, -122.0000000000000000 ) ) ;
#39019=CARTESIAN_POINT ( 'NONE',  ( 7.644554776091147741E-16, 12.48450537969573659, -78.96875000204839523 ) ) ;
#39020=CARTESIAN_POINT ( 'NONE',  ( 7.644554776091147741E-16, 12.48450537969573659, -88.15625000204838102 ) ) ;
#39023=CARTESIAN_POINT ( 'NONE',  ( -5.405949406250003975, -9.363379034771801557, -165.5312500020484094 ) ) ;
#39024=CARTESIAN_POINT ( 'NONE',  ( -5.405949406250003975, -9.363379034771801557, -183.5312500020484094 ) ) ;
#39025=CARTESIAN_POINT ( 'NONE',  ( -9.999999999999998224, 5.773502691896259087, -159.2500000040967905 ) ) ;
#39027=CARTESIAN_POINT ( 'NONE',  ( -10.81189881249999907, -6.242252689847864744, -1.968750002048352599 ) ) ;
#39029=CARTESIAN_POINT ( 'NONE',  ( -10.81189881249999907, -6.242252689847864744, -112.9687500020483810 ) ) ;
#39031=CARTESIAN_POINT ( 'NONE',  ( -2.293366432827344421E-15, -12.48450537969573659, -15.40625000204837214 ) ) ;
#39033=CARTESIAN_POINT ( 'NONE',  ( 0.000000000000000000, 0.000000000000000000, -99.99999999999998579 ) ) ;
#39034=CARTESIAN_POINT ( 'NONE',  ( -2.293366432827344421E-15, -12.48450537969573659, -111.4062500020483952 ) ) ;
#39037=CARTESIAN_POINT ( 'NONE',  ( -9.999999999999998224, 5.773502691896259087, -81.25000000409677625 ) ) ;
#39039=CARTESIAN_POINT ( 'NONE',  ( -10.81189881249999729, 6.242252689847871849, -42.71875000204835970 ) ) ;
#39043=CARTESIAN_POINT ( 'NONE',  ( 5.000000000000000000, 8.660254037844385522, -23.12500000409675849 ) ) ;
#39044=FACE_OUTER_BOUND ( 'NONE', #11738, .T. ) ;
#39052=EDGE_LOOP ( 'NONE', ( #23292, #26582, #6668, #34992 ) ) ;
#39056=CARTESIAN_POINT ( 'NONE',  ( 5.405949406249999534, 9.363379034771803333, -181.2812500020483810 ) ) ;
#39061=CARTESIAN_POINT ( 'NONE',  ( -5.405949406249996869, 9.363379034771805109, -102.8437500020483810 ) ) ;
#39063=CARTESIAN_POINT ( 'NONE',  ( -10.81189881249999907, -6.242252689847864744, -111.6562500020483952 ) ) ;
#39065=CARTESIAN_POINT ( 'NONE',  ( -10.81189881249999729, 1.324075727343319199E-15, -111.5937500020483810 ) ) ;
#39068=CARTESIAN_POINT ( 'NONE',  ( -9.999999999999998224, 1.224646799147353059E-15, -137.7499999999999716 ) ) ;
#39069=CARTESIAN_POINT ( 'NONE',  ( -9.999999999999998224, 1.224646799147353059E-15, -7.249999999999978684 ) ) ;
#39073=CARTESIAN_POINT ( 'NONE',  ( 4.999999999999992006, -8.660254037844389075, -176.6250000040968189 ) ) ;
#39075=CARTESIAN_POINT ( 'NONE',  ( 7.644554776091147741E-16, 12.48450537969573659, -26.46875000204837391 ) ) ;
#39076=CARTESIAN_POINT ( 'NONE',  ( -10.00000000000051337, 5.773502691895962435, -116.8749999999999858 ) ) ;
#39077=CARTESIAN_POINT ( 'NONE',  ( 7.644554776091147741E-16, 12.48450537969573659, -134.4687500020483810 ) ) ;
#39079=CARTESIAN_POINT ( 'NONE',  ( 7.070501591499376803E-16, 11.54700538379251284, -111.1249999999999858 ) ) ;
#39080=CARTESIAN_POINT ( 'NONE',  ( -10.00000000000000000, -5.773502691896251982, -68.62499999999998579 ) ) ;
#39081=CARTESIAN_POINT ( 'NONE',  ( -10.81189881249999729, 6.242252689847871849, -129.9062500020483810 ) ) ;
#39083=VERTEX_POINT ( 'NONE', #1152 ) ;
#39084=CARTESIAN_POINT ( 'NONE',  ( -9.999999999999998224, 1.224646799147353059E-15, -120.1250000040967905 ) ) ;
#39085=CARTESIAN_POINT ( 'NONE',  ( 10.00000000000000000, 5.773502691896255534, -104.2500000040967763 ) ) ;
#39086=CARTESIAN_POINT ( 'NONE',  ( 9.999999999999872102, 5.773502691896329253, -169.8750000000000000 ) ) ;
#39087=CARTESIAN_POINT ( 'NONE',  ( -10.81189881249999907, -6.242252689847864744, -67.96875000204838102 ) ) ;
#39093=CARTESIAN_POINT ( 'NONE',  ( 4.999999999999992006, -8.660254037844389075, -47.62500000409677625 ) ) ;
#39094=CARTESIAN_POINT ( 'NONE',  ( 7.644554776091147741E-16, 12.48450537969573659, -38.65625000204836681 ) ) ;
#39099=ORIENTED_EDGE ( 'NONE', *, *, #29386, .T. ) ;
#39100=VERTEX_POINT ( 'NONE', #37174 ) ;
#39101=VERTEX_POINT ( 'NONE', #14275 ) ;
#39102=DIRECTION ( 'NONE',  ( -1.000000000000000000, 0.000000000000000000, 0.000000000000000000 ) ) ;
#39107=EDGE_CURVE ( 'NONE', #34857, #27421, #26643, .T. ) ;
#39112=CARTESIAN_POINT ( 'NONE',  ( -10.81189881249999729, 1.324075727343319199E-15, -126.5937500020483668 ) ) ;
#39113=CARTESIAN_POINT ( 'NONE',  ( 10.81189881249999907, 6.242252689847868297, -130.4062500020483810 ) ) ;
#39116=CARTESIAN_POINT ( 'NONE',  ( -2.293366432827344421E-15, -12.48450537969573659, -145.7187500020484094 ) ) ;
#39118=CARTESIAN_POINT ( 'NONE',  ( 8.614196012144985204, -6.533971456632194474, -180.0000000000000000 ) ) ;
#39119=CARTESIAN_POINT ( 'NONE',  ( 5.000000000000000000, 8.660254037844385522, -141.6250000040967905 ) ) ;
#39120=CARTESIAN_POINT ( 'NONE',  ( -9.999999999999998224, 1.224646799147353059E-15, -166.2500000000000000 ) ) ;
#39124=CARTESIAN_POINT ( 'NONE',  ( 10.81189881249999907, 6.242252689847868297, -52.21875000204837391 ) ) ;
#39125=CARTESIAN_POINT ( 'NONE',  ( 0.000000000000000000, 0.000000000000000000, -99.99999999999998579 ) ) ;
#39126=CARTESIAN_POINT ( 'NONE',  ( 10.81189881249999729, 0.000000000000000000, -161.8437500020484094 ) ) ;
#39130=FACE_OUTER_BOUND ( 'NONE', #18970, .T. ) ;
#39132=CARTESIAN_POINT ( 'NONE',  ( -4.999999999999996447, 8.660254037844387298, -92.99999999999998579 ) ) ;
#39135=CARTESIAN_POINT ( 'NONE',  ( -10.81189881249999729, 6.242252689847871849, -120.9062500020483952 ) ) ;
#39136=CARTESIAN_POINT ( 'NONE',  ( 9.999999999999996447, -5.773502691896262640, -137.5000000040967905 ) ) ;
#39140=EDGE_CURVE ( 'NONE', #28517, #9895, #31072, .T. ) ;
#39142=CARTESIAN_POINT ( 'NONE',  ( -5.405949406250003975, -9.363379034771801557, -57.53125000204836681 ) ) ;
#39147=AXIS2_PLACEMENT_3D ( 'NONE', #10440, #39374, #39794 ) ;
#39161=CARTESIAN_POINT ( 'NONE',  ( 9.999999999999998224, 1.224646799147353059E-15, -99.99999999999998579 ) ) ;
#39162=CARTESIAN_POINT ( 'NONE',  ( -2.121150477449813534E-15, -11.54700538379251284, -30.87499999999995737 ) ) ;
#39165=CARTESIAN_POINT ( 'NONE',  ( 10.81189881249999907, 6.242252689847868297, -146.7187500020484094 ) ) ;
#39166=CARTESIAN_POINT ( 'NONE',  ( -5.405949406249996869, 9.363379034771805109, -171.8437500020484094 ) ) ;
#39168=CARTESIAN_POINT ( 'NONE',  ( -2.121150477449813534E-15, -11.54700538379251284, -161.7500000040968189 ) ) ;
#39169=CARTESIAN_POINT ( 'NONE',  ( -2.121150477449813534E-15, -11.54700538379251284, -189.8750000000000000 ) ) ;
#39173=DIRECTION ( 'NONE',  ( -1.000000000000000000, 0.000000000000000000, 0.000000000000000000 ) ) ;
#39174=CARTESIAN_POINT ( 'NONE',  ( -2.293366432827344421E-15, -12.48450537969573659, -189.2187500020484094 ) ) ;
#39177=CARTESIAN_POINT ( 'NONE',  ( -5.405949406250003975, -9.363379034771801557, -63.53125000204837391 ) ) ;
#39179=CARTESIAN_POINT ( 'NONE',  ( -5.000000000000003553, -8.660254037844383745, -113.4999999999999858 ) ) ;
#39180=ORIENTED_EDGE ( 'NONE', *, *, #38049, .T. ) ;
#39181=CARTESIAN_POINT ( 'NONE',  ( 10.81189881249999729, 6.242252689847867408, -143.9062500020484094 ) ) ;
#39182=CARTESIAN_POINT ( 'NONE',  ( 7.644554776091147741E-16, 12.48450537969573659, -158.6562500020484094 ) ) ;
#39185=CARTESIAN_POINT ( 'NONE',  ( -10.00000000000019362, -5.773502691896140959, -179.6250000000000568 ) ) ;
#39186=CARTESIAN_POINT ( 'NONE',  ( 7.644554776091147741E-16, 12.48450537969573659, -93.96875000204838102 ) ) ;
#39189=CARTESIAN_POINT ( 'NONE',  ( 10.81189881249999907, 6.242252689847868297, -188.7187500020484094 ) ) ;
#39193=CARTESIAN_POINT ( 'NONE',  ( 5.405949406249999534, 9.363379034771803333, -86.78125000204838102 ) ) ;
#39195=CARTESIAN_POINT ( 'NONE',  ( 10.00000000000000000, 5.773502691896255534, -63.75000000409677625 ) ) ;
#39196=CARTESIAN_POINT ( 'NONE',  ( -10.81189881249999907, -6.242252689847864744, -18.46875000204836681 ) ) ;
#39199=CARTESIAN_POINT ( 'NONE',  ( -10.81189881249999729, 1.324075727343319199E-15, -9.781250002048352599 ) ) ;
#39201=CARTESIAN_POINT ( 'NONE',  ( 10.00000000000000000, 5.773502691896255534, -137.2500000040967905 ) ) ;
#39211=ORIENTED_EDGE ( 'NONE', *, *, #7629, .F. ) ;
#39221=CARTESIAN_POINT ( 'NONE',  ( -5.405949406250003975, -9.363379034771801557, -158.0312500020484094 ) ) ;
#39223=CARTESIAN_POINT ( 'NONE',  ( -9.999999999999804601, 5.773502691896371886, -178.3750000000000284 ) ) ;
#39227=CARTESIAN_POINT ( 'NONE',  ( -10.81189881249999907, -6.242252689847864744, -78.46875000204838102 ) ) ;
#39228=CARTESIAN_POINT ( 'NONE',  ( 7.644554776091147741E-16, 12.48450537969573659, -86.65625000204838102 ) ) ;
#39231=CARTESIAN_POINT ( 'NONE',  ( 7.644554776091147741E-16, 12.48450537969573659, -163.1562500020483810 ) ) ;
#39232=CARTESIAN_POINT ( 'NONE',  ( -5.405949406250003975, -9.363379034771801557, -177.5312500020483810 ) ) ;
#39233=EDGE_CURVE ( 'NONE', #32014, #11758, #41254, .T. ) ;
#39234=CARTESIAN_POINT ( 'NONE',  ( 9.999999999999996447, -5.773502691896262640, -160.0000000040968189 ) ) ;
#39235=CARTESIAN_POINT ( 'NONE',  ( 7.644554776091147741E-16, 12.48450537969573659, -6.968750002048357040 ) ) ;
#39237=CARTESIAN_POINT ( 'NONE',  ( -5.405949406250003975, -9.363379034771801557, -117.3437500020483810 ) ) ;
#39239=CARTESIAN_POINT ( 'NONE',  ( -2.293366432827344421E-15, -12.48450537969573659, -12.40625000204836859 ) ) ;
#39242=CARTESIAN_POINT ( 'NONE',  ( -5.405949406249996869, 9.363379034771805109, -104.5312500020483810 ) ) ;
#39245=CARTESIAN_POINT ( 'NONE',  ( -9.999999999999998224, 5.773502691896259087, -82.75000000409676204 ) ) ;
#39246=DIRECTION ( 'NONE',  ( -0.000000000000000000, -0.000000000000000000, -1.000000000000000000 ) ) ;
#39247=CARTESIAN_POINT ( 'NONE',  ( 5.405949406249992428, -9.363379034771808662, -42.09375000204837391 ) ) ;
#39252=CARTESIAN_POINT ( 'NONE',  ( -4.999999999999996447, 8.660254037844387298, -13.87500000409674961 ) ) ;
#39266=CARTESIAN_POINT ( 'NONE',  ( 0.000000000000000000, 0.000000000000000000, -103.0000000000000000 ) ) ;
#39267=CARTESIAN_POINT ( 'NONE',  ( 7.644554776091147741E-16, 12.48450537969573659, -182.6562500020484094 ) ) ;
#39270=CIRCLE ( 'NONE', #17226, 9.999999999999998224 ) ;
#39272=CARTESIAN_POINT ( 'NONE',  ( -10.81189881249999907, -6.242252689847864744, -102.4687500020483810 ) ) ;
#39274=CARTESIAN_POINT ( 'NONE',  ( -10.81189881249999729, 1.324075727343319199E-15, -105.7812500020483810 ) ) ;
#39276=CARTESIAN_POINT ( 'NONE',  ( -5.405949406250003975, -9.363379034771801557, -112.8437500020483810 ) ) ;
#39280=CARTESIAN_POINT ( 'NONE',  ( 9.999999999999996447, -5.773502691896262640, -143.1250000000000000 ) ) ;
#39281=CARTESIAN_POINT ( 'NONE',  ( 4.999999999999992006, -8.660254037844389075, -8.249999999999952038 ) ) ;
#39284=CARTESIAN_POINT ( 'NONE',  ( -4.999999999999996447, 8.660254037844387298, -181.8750000040967905 ) ) ;
#39286=CARTESIAN_POINT ( 'NONE',  ( -10.81189881249999907, -6.242252689847864744, -25.96875000204837391 ) ) ;
#39287=CARTESIAN_POINT ( 'NONE',  ( 5.405949406249992428, -9.363379034771808662, -136.5937500020483810 ) ) ;
#39290=CARTESIAN_POINT ( 'NONE',  ( -10.00000000000000000, -5.773502691896251982, -64.12499999999998579 ) ) ;
#39291=CARTESIAN_POINT ( 'NONE',  ( -10.81189881249999729, 1.324075727343319199E-15, -135.7812500020483810 ) ) ;
#39294=CARTESIAN_POINT ( 'NONE',  ( 9.999999999999998224, 0.000000000000000000, -143.0000000000000000 ) ) ;
#39295=CARTESIAN_POINT ( 'NONE',  ( -5.000000000000003553, -8.660254037844383745, -109.3750000040967763 ) ) ;
#39296=CARTESIAN_POINT ( 'NONE',  ( 5.405949406249999534, 9.363379034771803333, -67.09375000204836681 ) ) ;
#39301=CARTESIAN_POINT ( 'NONE',  ( 9.999999999999998224, 0.000000000000000000, -156.8750000040967905 ) ) ;
#39302=CARTESIAN_POINT ( 'NONE',  ( -10.00000000000000000, -5.773502691896251982, -36.00000000409675494 ) ) ;
#39303=CARTESIAN_POINT ( 'NONE',  ( -10.81189881249999729, 1.324075727343319199E-15, -36.78125000204837391 ) ) ;
#39304=CARTESIAN_POINT ( 'NONE',  ( 0.000000000000000000, 0.000000000000000000, -99.99999999999998579 ) ) ;
#39310=ORIENTED_EDGE ( 'NONE', *, *, #36863, .T. ) ;
#39315=CARTESIAN_POINT ( 'NONE',  ( -10.00000000000076916, 5.773502691895813221, -111.2500000040967620 ) ) ;
#39318=CARTESIAN_POINT ( 'NONE',  ( -5.405949406249996869, 9.363379034771805109, -126.8437500020483952 ) ) ;
#39319=CARTESIAN_POINT ( 'NONE',  ( -2.293366432827344421E-15, -12.48450537969573659, -132.4062500020483810 ) ) ;
#39321=CARTESIAN_POINT ( 'NONE',  ( -2.293366432827344421E-15, -12.48450537969573659, -139.7187500020483810 ) ) ;
#39322=DIRECTION ( 'NONE',  ( -0.000000000000000000, -0.000000000000000000, -1.000000000000000000 ) ) ;
#39324=CARTESIAN_POINT ( 'NONE',  ( -4.999999999999996447, 8.660254037844387298, -163.5000000000000000 ) ) ;
#39329=CARTESIAN_POINT ( 'NONE',  ( 5.405949406249992428, -9.363379034771808662, -54.09375000204835970 ) ) ;
#39331=CARTESIAN_POINT ( 'NONE',  ( 10.81189881249999907, 6.242252689847868297, -163.2187500020483810 ) ) ;
#39337=CARTESIAN_POINT ( 'NONE',  ( 9.999999999999998224, 0.000000000000000000, -91.99999999999998579 ) ) ;
#39339=CARTESIAN_POINT ( 'NONE',  ( -5.405949406250003975, -9.363379034771801557, -116.0312500020483952 ) ) ;
#39340=CARTESIAN_POINT ( 'NONE',  ( -5.000000000000003553, -8.660254037844383745, -134.8750000040967905 ) ) ;
#39344=CARTESIAN_POINT ( 'NONE',  ( -5.405949406250003975, -9.363379034771801557, -62.03125000204837391 ) ) ;
#39349=CARTESIAN_POINT ( 'NONE',  ( 9.999999999999998224, 0.000000000000000000, -171.8750000040968189 ) ) ;
#39360=ORIENTED_EDGE ( 'NONE', *, *, #23820, .F. ) ;
#39361=ORIENTED_EDGE ( 'NONE', *, *, #7748, .T. ) ;
#39366=CARTESIAN_POINT ( 'NONE',  ( 4.999999999999992006, -8.660254037844389075, -134.2499999999999716 ) ) ;
#39367=CARTESIAN_POINT ( 'NONE',  ( 9.999999999999996447, -5.773502691896262640, -26.12499999999998224 ) ) ;
#39371=CARTESIAN_POINT ( 'NONE',  ( 10.81189881249999551, -6.242252689847874514, -151.4687500020483810 ) ) ;
#39372=CARTESIAN_POINT ( 'NONE',  ( -5.405949406250003975, -9.363379034771801557, -162.3437500020484094 ) ) ;
#39374=DIRECTION ( 'NONE',  ( -0.000000000000000000, -0.000000000000000000, -1.000000000000000000 ) ) ;
#39375=CARTESIAN_POINT ( 'NONE',  ( 10.00000000000000000, 5.773502691896255534, -184.8750000000000000 ) ) ;
#39380=CARTESIAN_POINT ( 'NONE',  ( -10.81189881249999729, 6.242252689847871849, -182.2187500020484379 ) ) ;
#39384=CARTESIAN_POINT ( 'NONE',  ( -10.81189881249999729, 1.324075727343319199E-15, -59.28125000204836681 ) ) ;
#39386=CARTESIAN_POINT ( 'NONE',  ( 7.070501591499377789E-16, 11.54700538379251284, -117.1249999999999858 ) ) ;
#39388=CARTESIAN_POINT ( 'NONE',  ( -10.81189881249999729, -6.242252689847864744, -141.6562500020484094 ) ) ;
#39389=CARTESIAN_POINT ( 'NONE',  ( -5.405949406250003975, -9.363379034771801557, -156.5312500020484094 ) ) ;
#39393=CARTESIAN_POINT ( 'NONE',  ( 5.405949406249999534, 9.363379034771803333, -86.59375000204836681 ) ) ;
#39396=CARTESIAN_POINT ( 'NONE',  ( 10.81189881249999729, 0.000000000000000000, -191.8437500020484094 ) ) ;
#39400=CARTESIAN_POINT ( 'NONE',  ( -10.81189881249999907, -6.242252689847864744, -84.65625000204836681 ) ) ;
#39402=CARTESIAN_POINT ( 'NONE',  ( 9.999999999999998224, 0.000000000000000000, -62.37500000409676204 ) ) ;
#39403=CARTESIAN_POINT ( 'NONE',  ( -5.405949406249996869, 9.363379034771805109, -17.34375000204835260 ) ) ;
#39407=CARTESIAN_POINT ( 'NONE',  ( 10.81189881249999551, -6.242252689847874514, -12.15625000204836859 ) ) ;
#39412=CARTESIAN_POINT ( 'NONE',  ( -6.652853726956784897, 8.522716305231336165, -100.0000000000000142 ) ) ;
#39413=ADVANCED_FACE ( 'NONE', ( #16782 ), #17000, .F. ) ;
#39416=EDGE_CURVE ( 'NONE', #28218, #20460, #18954, .T. ) ;
#39420=CARTESIAN_POINT ( 'NONE',  ( 5.405949406249992428, -9.363379034771808662, -102.0937500020483810 ) ) ;
#39431=CARTESIAN_POINT ( 'NONE',  ( 9.999999999999998224, 1.224646799147353059E-15, -99.99999999999998579 ) ) ;
#39433=CARTESIAN_POINT ( 'NONE',  ( 10.81189881249999551, -6.242252689847874514, -156.1562500020484094 ) ) ;
#39439=CARTESIAN_POINT ( 'NONE',  ( -10.81189881249999729, 1.324075727343319199E-15, -78.59375000204838102 ) ) ;
#39440=CARTESIAN_POINT ( 'NONE',  ( 5.405949406249999534, 9.363379034771803333, -88.28125000204838102 ) ) ;
#39443=CARTESIAN_POINT ( 'NONE',  ( 10.81189881249999551, -6.242252689847874514, -168.1562500020484094 ) ) ;
#39444=CARTESIAN_POINT ( 'NONE',  ( 5.405949406249999534, 9.363379034771803333, -181.2812500020483810 ) ) ;
#39445=CARTESIAN_POINT ( 'NONE',  ( 10.00000000000000000, 5.773502691896255534, -158.2500000040967905 ) ) ;
#39447=CARTESIAN_POINT ( 'NONE',  ( 10.81189881249999551, -6.242252689847874514, -4.468750002048355263 ) ) ;
#39449=CARTESIAN_POINT ( 'NONE',  ( 7.644554776091147741E-16, 12.48450537969573659, -111.9687500020483952 ) ) ;
#39451=CARTESIAN_POINT ( 'NONE',  ( -10.81189881249999729, 6.242252689847871849, -11.40625000204836859 ) ) ;
#39454=CARTESIAN_POINT ( 'NONE',  ( 7.644554776091147741E-16, 12.48450537969573659, -107.6562500020483810 ) ) ;
#39458=CARTESIAN_POINT ( 'NONE',  ( 10.00000000000000000, 5.773502691896255534, -87.75000000409677625 ) ) ;
#39460=CARTESIAN_POINT ( 'NONE',  ( -10.81189881249999907, -6.242252689847864744, -40.96875000204835260 ) ) ;
#39465=CARTESIAN_POINT ( 'NONE',  ( -10.00000000000000000, -5.773502691896251982, -9.000000004096758488 ) ) ;
#39469=DIRECTION ( 'NONE',  ( -0.000000000000000000, -0.000000000000000000, -1.000000000000000000 ) ) ;
#39473=EDGE_CURVE ( 'NONE', #8961, #20303, #17540, .T. ) ;
#39479=CARTESIAN_POINT ( 'NONE',  ( -5.405949406250003975, -9.363379034771801557, -180.5312500020483810 ) ) ;
#39481=CYLINDRICAL_SURFACE ( 'NONE', #7319, 35.00000000000000711 ) ;
#39483=CARTESIAN_POINT ( 'NONE',  ( 10.81189881249999729, 0.000000000000000000, -101.8437500020483810 ) ) ;
#39485=CARTESIAN_POINT ( 'NONE',  ( 5.405949406249992428, -9.363379034771808662, -105.2812500020483810 ) ) ;
#39487=CARTESIAN_POINT ( 'NONE',  ( 10.81189881249999729, 6.242252689847867408, -115.2187500020483810 ) ) ;
#39491=CARTESIAN_POINT ( 'NONE',  ( -10.00000000000000000, -5.773502691896251982, -139.1250000000000000 ) ) ;
#39492=CARTESIAN_POINT ( 'NONE',  ( 10.00000000000000000, 5.773502691896255534, -1.874999999999960254 ) ) ;
#39495=CARTESIAN_POINT ( 'NONE',  ( 9.999999999999998224, 0.000000000000000000, -180.8750000040967905 ) ) ;
#39497=CARTESIAN_POINT ( 'NONE',  ( 10.81189881249999729, 0.000000000000000000, -28.34375000204836326 ) ) ;
#39499=CARTESIAN_POINT ( 'NONE',  ( 5.405949406249999534, 9.363379034771803333, -139.0937500020483810 ) ) ;
#39501=CARTESIAN_POINT ( 'NONE',  ( -5.405949406249996869, 9.363379034771805109, -34.03125000204837391 ) ) ;
#39502=LINE ( 'NONE', #30017, #14127 ) ;
#39503=CARTESIAN_POINT ( 'NONE',  ( 4.999999999999992006, -8.660254037844389075, -71.24999999999998579 ) ) ;
#39504=CARTESIAN_POINT ( 'NONE',  ( 10.81189881249999551, -6.242252689847874514, -130.6562500020484094 ) ) ;
#39506=ORIENTED_EDGE ( 'NONE', *, *, #2632, .F. ) ;
#39509=CARTESIAN_POINT ( 'NONE',  ( 7.070501591499377789E-16, 11.54700538379251284, -110.0000000040968047 ) ) ;
#39510=CARTESIAN_POINT ( 'NONE',  ( 7.070501591499376803E-16, 11.54700538379251284, -162.1250000000000284 ) ) ;
#39511=CARTESIAN_POINT ( 'NONE',  ( -10.81189881249999907, -6.242252689847864744, -69.46875000204838102 ) ) ;
#39512=ORIENTED_EDGE ( 'NONE', *, *, #25059, .F. ) ;
#39517=CARTESIAN_POINT ( 'NONE',  ( 7.070501591499377789E-16, 11.54700538379251284, -38.00000000409675494 ) ) ;
#39523=EDGE_CURVE ( 'NONE', #19597, #32882, #20671, .T. ) ;
#39534=CARTESIAN_POINT ( 'NONE',  ( -10.81189881249999729, 6.242252689847871849, -126.7187500020483952 ) ) ;
#39535=CARTESIAN_POINT ( 'NONE',  ( -2.293366432827344421E-15, -12.48450537969573659, -133.9062500020483810 ) ) ;
#39537=CARTESIAN_POINT ( 'NONE',  ( -10.81189881249999729, -6.242252689847864744, -139.9687500020483810 ) ) ;
#39538=CARTESIAN_POINT ( 'NONE',  ( -5.000000000000003553, -8.660254037844383745, -125.8750000040967905 ) ) ;
#39540=CARTESIAN_POINT ( 'NONE',  ( 10.00000000000000000, 5.773502691896255534, -160.8750000000000000 ) ) ;
#39543=CARTESIAN_POINT ( 'NONE',  ( -10.81189881249999907, -6.242252689847864744, -57.46875000204836681 ) ) ;
#39544=CARTESIAN_POINT ( 'NONE',  ( 4.999999999999992006, -8.660254037844389075, -174.7500000000000284 ) ) ;
#39545=CARTESIAN_POINT ( 'NONE',  ( -5.405949406249996869, 9.363379034771805109, -165.8437500020484094 ) ) ;
#39550=CARTESIAN_POINT ( 'NONE',  ( -2.121150477449813534E-15, -11.54700538379251284, -95.37500000000000000 ) ) ;
#39551=EDGE_LOOP ( 'NONE', ( #22436, #29191, #5307, #26979 ) ) ;
#39552=CARTESIAN_POINT ( 'NONE',  ( -10.81189881249999729, -6.242252689847864744, -113.1562500020483952 ) ) ;
#39553=CARTESIAN_POINT ( 'NONE',  ( -4.999999999999996447, 8.660254037844387298, -129.3750000040967905 ) ) ;
#39554=LINE ( 'NONE', #16873, #33275 ) ;
#39558=CARTESIAN_POINT ( 'NONE',  ( 5.405949406249999534, 9.363379034771803333, -56.78125000204836681 ) ) ;
#39563=CARTESIAN_POINT ( 'NONE',  ( 10.00000000000012790, 5.773502691896179151, -171.7500000040967620 ) ) ;
#39571=ORIENTED_EDGE ( 'NONE', *, *, #39107, .F. ) ;
#39576=CARTESIAN_POINT ( 'NONE',  ( -9.999999999999998224, 1.224646799147353059E-15, -25.24999999999996803 ) ) ;
#39579=CARTESIAN_POINT ( 'NONE',  ( 10.81189881249999907, 6.242252689847868297, -151.2187500020483810 ) ) ;
#39580=CARTESIAN_POINT ( 'NONE',  ( 10.81189881249999551, -6.242252689847874514, -163.4687500020483810 ) ) ;
#39581=CARTESIAN_POINT ( 'NONE',  ( -9.999999999999998224, 1.224646799147353059E-15, -123.1250000040967905 ) ) ;
#39583=CARTESIAN_POINT ( 'NONE',  ( 4.999999999999992006, -8.660254037844389075, -189.7500000000000000 ) ) ;
#39588=CARTESIAN_POINT ( 'NONE',  ( 5.405949406249992428, -9.363379034771808662, -187.5937500020483810 ) ) ;
#39592=CARTESIAN_POINT ( 'NONE',  ( 7.644554776091147741E-16, 12.48450537969573659, -49.15625000204837391 ) ) ;
#39594=CARTESIAN_POINT ( 'NONE',  ( -5.000000000000003553, -8.660254037844383745, -116.4999999999999858 ) ) ;
#39596=CARTESIAN_POINT ( 'NONE',  ( 10.81189881249999551, -6.242252689847874514, -133.6562500020483810 ) ) ;
#39597=CARTESIAN_POINT ( 'NONE',  ( 10.81189881249999729, 0.000000000000000000, -145.5312500020483810 ) ) ;
#39599=DIRECTION ( 'NONE',  ( -0.000000000000000000, -0.000000000000000000, -1.000000000000000000 ) ) ;
#39600=CARTESIAN_POINT ( 'NONE',  ( -2.293366432827344421E-15, -12.48450537969573659, -78.21875000204838102 ) ) ;
#39603=CARTESIAN_POINT ( 'NONE',  ( 5.405949406249992428, -9.363379034771808662, -186.0937500020483810 ) ) ;
#39606=CARTESIAN_POINT ( 'NONE',  ( 7.070501591499376803E-16, 11.54700538379251284, -140.0000000040967905 ) ) ;
#39607=CARTESIAN_POINT ( 'NONE',  ( 5.405949406249999534, 9.363379034771803333, -83.78125000204838102 ) ) ;
#39609=CARTESIAN_POINT ( 'NONE',  ( 7.070501591499377789E-16, 11.54700538379251284, -59.00000000409677625 ) ) ;
#39610=CARTESIAN_POINT ( 'NONE',  ( -10.81189881249999729, 1.324075727343319199E-15, -15.59375000204835082 ) ) ;
#39613=CARTESIAN_POINT ( 'NONE',  ( -5.405949406249996869, 9.363379034771805109, -11.53125000204835438 ) ) ;
#39614=CARTESIAN_POINT ( 'NONE',  ( -5.000000000000003553, -8.660254037844383745, -148.3750000040967905 ) ) ;
#39615=LINE ( 'NONE', #36597, #24972 ) ;
#39619=DIRECTION ( 'NONE',  ( -0.000000000000000000, -0.000000000000000000, -1.000000000000000000 ) ) ;
#39634=CARTESIAN_POINT ( 'NONE',  ( 5.405949406249999534, 9.363379034771803333, -151.2812500020484094 ) ) ;
#39642=CARTESIAN_POINT ( 'NONE',  ( -10.81189881249999729, 1.324075727343319199E-15, -74.09375000204838102 ) ) ;
#39643=CARTESIAN_POINT ( 'NONE',  ( -10.81189881249999729, 6.242252689847871849, -83.40625000204836681 ) ) ;
#39645=EDGE_CURVE ( 'NONE', #39928, #40993, #8260, .T. ) ;
#39646=FACE_OUTER_BOUND ( 'NONE', #55, .T. ) ;
#39647=CARTESIAN_POINT ( 'NONE',  ( -10.81189881249999729, -6.242252689847864744, -167.1562500020484094 ) ) ;
#39648=CARTESIAN_POINT ( 'NONE',  ( 10.81189881249999729, 0.000000000000000000, -180.0312500020483810 ) ) ;
#39649=CARTESIAN_POINT ( 'NONE',  ( -5.000000000000003553, -8.660254037844383745, -157.3750000040967905 ) ) ;
#39650=CYLINDRICAL_SURFACE ( 'NONE', #25650, 9.999999999999998224 ) ;
#39651=CARTESIAN_POINT ( 'NONE',  ( 7.644554776091147741E-16, 12.48450537969573659, -3.968750002048354819 ) ) ;
#39653=CARTESIAN_POINT ( 'NONE',  ( -2.293366432827344421E-15, -12.48450537969573659, -117.2187500020483952 ) ) ;
#39655=CARTESIAN_POINT ( 'NONE',  ( -10.81189881249999729, 1.324075727343319199E-15, -11.28125000204835438 ) ) ;
#39660=CARTESIAN_POINT ( 'NONE',  ( -10.81189881249999729, 6.242252689847871849, -108.9062500020483810 ) ) ;
#39662=EDGE_LOOP ( 'NONE', ( #28063, #9698, #20355, #19745, #29129, #8641, #31109, #17515, #21480, #15231, #13551, #37510, #21811, #31456, #16715, #18775, #24469, #39571, #28329, #28463, #9792, #10424, #849, #31218, #11058, #23719, #36646, #855, #38425, #2861, #2244, #8389, #19651, #7661, #41694, #15471, #26443, #30521, #14537, #32745, #12390, #38408, #28160, #15099, #4284, #29444, #556, #8688, #33750, #1864, #5514, #38631, #31358, #19039, #41856, #15616, #31313, #42593, #16565, #1040, #38417, #23085, #21644, #12654, #35556, #13379, #40255, #39211, #35081, #20335, #27434, #5082, #1860, #18132, #17961, #31327, #12441, #1619, #26325, #24471, #32783, #6208, #10372, #35039, #37438, #3997, #19862, #17201, #33331, #37179, #9799, #1375, #12322, #7313, #16094, #11703, #22692, #28760, #14502, #8600, #13338, #1373, #19231, #10958, #28239, #5063, #4604, #38897, #6939, #32511, #33755 ) ) ;
#39663=CARTESIAN_POINT ( 'NONE',  ( -4.999999999999996447, 8.660254037844387298, -87.37500000409677625 ) ) ;
#39664=CARTESIAN_POINT ( 'NONE',  ( 9.999999999999998224, 0.000000000000000000, -117.5000000000000000 ) ) ;
#39665=CARTESIAN_POINT ( 'NONE',  ( 10.81189881249999551, -6.242252689847874514, -44.96875000204835970 ) ) ;
#39666=ORIENTED_EDGE ( 'NONE', *, *, #35493, .F. ) ;
#39670=CARTESIAN_POINT ( 'NONE',  ( 9.999999999999998224, 0.000000000000000000, -8.375000004096744277 ) ) ;
#39675=ORIENTED_EDGE ( 'NONE', *, *, #21969, .F. ) ;
#39676=CARTESIAN_POINT ( 'NONE',  ( 24.99999999999999645, 3.061616997868382648E-15, -103.0000000000000000 ) ) ;
#39688=CARTESIAN_POINT ( 'NONE',  ( -10.81189881249999729, 6.242252689847871849, -179.4062500020484094 ) ) ;
#39691=CARTESIAN_POINT ( 'NONE',  ( 7.644554776091147741E-16, 12.48450537969573659, -99.96875000204839523 ) ) ;
#39693=CARTESIAN_POINT ( 'NONE',  ( -10.81189881249999729, 1.324075727343319199E-15, -110.2812500020483810 ) ) ;
#39695=CARTESIAN_POINT ( 'NONE',  ( 5.405949406249992428, -9.363379034771808662, -111.0937500020483810 ) ) ;
#39698=CARTESIAN_POINT ( 'NONE',  ( -9.999999999999998224, 1.224646799147353059E-15, -115.2499999999999858 ) ) ;
#39699=CARTESIAN_POINT ( 'NONE',  ( -4.999999999999996447, 8.660254037844387298, -127.5000000000000000 ) ) ;
#39700=CARTESIAN_POINT ( 'NONE',  ( -4.999999999999996447, 8.660254037844387298, -4.499999999999976019 ) ) ;
#39703=CARTESIAN_POINT ( 'NONE',  ( -5.000000000000003553, -8.660254037844383745, -178.3750000040967905 ) ) ;
#39705=CARTESIAN_POINT ( 'NONE',  ( 5.405949406249999534, 9.363379034771803333, -29.59375000204836326 ) ) ;
#39706=CARTESIAN_POINT ( 'NONE',  ( 5.405949406249999534, 9.363379034771803333, -142.0937500020483810 ) ) ;
#39708=CARTESIAN_POINT ( 'NONE',  ( -10.81189881249999729, 1.324075727343319199E-15, -38.28125000204838102 ) ) ;
#39711=AXIS2_PLACEMENT_3D ( 'NONE', #41650, #25281, #35624 ) ;
#39712=CARTESIAN_POINT ( 'NONE',  ( -4.999999999999996447, 8.660254037844387298, -59.99999999999997158 ) ) ;
#39713=CARTESIAN_POINT ( 'NONE',  ( 10.81189881249999907, 6.242252689847868297, -131.9062500020484094 ) ) ;
#39717=CARTESIAN_POINT ( 'NONE',  ( -9.999999999999998224, 1.224646799147353059E-15, -109.6250000040967763 ) ) ;
#39719=CARTESIAN_POINT ( 'NONE',  ( 10.81189881249999551, -6.242252689847874514, -62.96875000204838102 ) ) ;
#39720=ORIENTED_EDGE ( 'NONE', *, *, #29149, .T. ) ;
#39726=CARTESIAN_POINT ( 'NONE',  ( 5.000000000000000000, 8.660254037844385522, -33.62500000409676915 ) ) ;
#39727=CARTESIAN_POINT ( 'NONE',  ( -10.00000000000025580, 5.773502691896109873, -117.2500000040968047 ) ) ;
#39729=CARTESIAN_POINT ( 'NONE',  ( -10.00000000000025580, 5.773502691896109873, -121.7500000040967905 ) ) ;
#39742=CARTESIAN_POINT ( 'NONE',  ( -5.405949406249996869, 9.363379034771805109, -122.3437500020483952 ) ) ;
#39743=CARTESIAN_POINT ( 'NONE',  ( 10.81189881249999729, 0.000000000000000000, -135.0312500020484094 ) ) ;
#39745=CARTESIAN_POINT ( 'NONE',  ( -5.405949406250003975, -9.363379034771801557, -136.8437500020484094 ) ) ;
#39746=CARTESIAN_POINT ( 'NONE',  ( -9.999999999999998224, 1.224646799147353059E-15, -130.2499999999999716 ) ) ;
#39749=CARTESIAN_POINT ( 'NONE',  ( -9.999999999999998224, 1.224646799147353059E-15, -158.7500000000000000 ) ) ;
#39750=CARTESIAN_POINT ( 'NONE',  ( 10.81189881249999551, -6.242252689847874514, -0.1562500020483581498 ) ) ;
#39753=CARTESIAN_POINT ( 'NONE',  ( 7.644554776091147741E-16, 12.48450537969573659, -56.46875000204837391 ) ) ;
#39755=CARTESIAN_POINT ( 'NONE',  ( 5.405949406249999534, 9.363379034771803333, -166.0937500020484094 ) ) ;
#39758=DIRECTION ( 'NONE',  ( -0.000000000000000000, -0.000000000000000000, -1.000000000000000000 ) ) ;
#39760=CARTESIAN_POINT ( 'NONE',  ( -4.999999999999996447, 8.660254037844387298, -89.99999999999998579 ) ) ;
#39761=ORIENTED_EDGE ( 'NONE', *, *, #4849, .T. ) ;
#39762=( BOUNDED_CURVE ( )  B_SPLINE_CURVE ( 2, ( #5632, #15737, #18572, #42489, #41857, #42074, #12504 ),
 .UNSPECIFIED., .F., .F. ) 
 B_SPLINE_CURVE_WITH_KNOTS ( ( 3, 2, 2, 3 ),
 ( 0.1194029850746269744, 0.1206467661691543042, 0.1218905472636816062, 0.1231343283582089221 ),
 .UNSPECIFIED. ) 
 CURVE ( )  GEOMETRIC_REPRESENTATION_ITEM ( )  RATIONAL_B_SPLINE_CURVE ( ( 0.9999999999999880096, 0.8660254037844506980, 1.000000000000000000, 0.8660254037844387076, 1.000000000000000000, 0.8660254037844417052, 0.9999999999999970024 ) ) 
 REPRESENTATION_ITEM ( '' )  );
#39763=CARTESIAN_POINT ( 'NONE',  ( 7.644554776091147741E-16, 12.48450537969573659, -109.1562500020483810 ) ) ;
#39764=CARTESIAN_POINT ( 'NONE',  ( -4.999999999999996447, 8.660254037844387298, -130.8750000040967905 ) ) ;
#39769=CARTESIAN_POINT ( 'NONE',  ( 10.81189881249999729, 0.000000000000000000, -51.03125000204835970 ) ) ;
#39776=CARTESIAN_POINT ( 'NONE',  ( 9.999999999999998224, 0.000000000000000000, -171.5000000000000000 ) ) ;
#39781=ORIENTED_EDGE ( 'NONE', *, *, #11956, .F. ) ;
#39788=DIRECTION ( 'NONE',  ( -1.000000000000000000, 0.000000000000000000, 0.000000000000000000 ) ) ;
#39791=CARTESIAN_POINT ( 'NONE',  ( -10.81189881249999729, 6.242252689847871849, -146.2187500020483810 ) ) ;
#39792=CARTESIAN_POINT ( 'NONE',  ( 10.81189881249999551, -6.242252689847874514, -164.9687500020483810 ) ) ;
#39794=DIRECTION ( 'NONE',  ( -1.000000000000000000, 0.000000000000000000, 0.000000000000000000 ) ) ;
#39795=CARTESIAN_POINT ( 'NONE',  ( -5.000000000000003553, -8.660254037844383745, -184.0000000000000000 ) ) ;
#39798=CARTESIAN_POINT ( 'NONE',  ( -9.999999999999998224, 1.224646799147353059E-15, -151.2500000000000000 ) ) ;
#39801=CARTESIAN_POINT ( 'NONE',  ( 5.405949406249999534, 9.363379034771803333, -187.0937500020483810 ) ) ;
#39804=CARTESIAN_POINT ( 'NONE',  ( -10.81189881249999729, 6.242252689847871849, -56.40625000204838813 ) ) ;
#39806=CARTESIAN_POINT ( 'NONE',  ( 5.000000000000000000, 8.660254037844385522, -118.7500000000000000 ) ) ;
#39808=CARTESIAN_POINT ( 'NONE',  ( -2.293366432827344421E-15, -12.48450537969573659, -133.9062500020483810 ) ) ;
#39809=CARTESIAN_POINT ( 'NONE',  ( 5.405949406249999534, 9.363379034771803333, -145.2812500020483810 ) ) ;
#39812=CARTESIAN_POINT ( 'NONE',  ( -5.405949406250003975, -9.363379034771801557, -85.84375000204836681 ) ) ;
#39813=ORIENTED_EDGE ( 'NONE', *, *, #23289, .F. ) ;
#39815=CARTESIAN_POINT ( 'NONE',  ( -5.405949406250003975, -9.363379034771801557, -180.3437500020483810 ) ) ;
#39820=CARTESIAN_POINT ( 'NONE',  ( 5.405949406249992428, -9.363379034771808662, -76.78125000204838102 ) ) ;
#39822=CARTESIAN_POINT ( 'NONE',  ( -9.999999999999998224, 5.773502691896259087, -51.25000000409677625 ) ) ;
#39823=CARTESIAN_POINT ( 'NONE',  ( 5.405949406249992428, -9.363379034771808662, -7.593750002048343717 ) ) ;
#39826=CARTESIAN_POINT ( 'NONE',  ( 5.405949406249992428, -9.363379034771808662, -9.281250002048352599 ) ) ;
#39828=CYLINDRICAL_SURFACE ( 'NONE', #34458, 9.999999999999998224 ) ;
#39833=CYLINDRICAL_SURFACE ( 'NONE', #15144, 9.999999999999998224 ) ;
#39835=ORIENTED_EDGE ( 'NONE', *, *, #32845, .T. ) ;
#39840=ORIENTED_EDGE ( 'NONE', *, *, #4578, .T. ) ;
#39849=CARTESIAN_POINT ( 'NONE',  ( 7.644554776091147741E-16, 12.48450537969573659, -151.1562500020484094 ) ) ;
#39856=CARTESIAN_POINT ( 'NONE',  ( 5.405949406249999534, 9.363379034771803333, -68.59375000204836681 ) ) ;
#39857=CARTESIAN_POINT ( 'NONE',  ( -2.293366432827344421E-15, -12.48450537969573659, -73.90625000204836681 ) ) ;
#39859=DIRECTION ( 'NONE',  ( -0.000000000000000000, -0.000000000000000000, -1.000000000000000000 ) ) ;
#39860=CARTESIAN_POINT ( 'NONE',  ( -5.405949406249996869, 9.363379034771805109, -161.5312500020484094 ) ) ;
#39861=CARTESIAN_POINT ( 'NONE',  ( -2.293366432827344421E-15, -12.48450537969573659, -172.9062500020484379 ) ) ;
#39863=CARTESIAN_POINT ( 'NONE',  ( 10.81189881249999907, 6.242252689847868297, 0.2812499979516491777 ) ) ;
#39864=CARTESIAN_POINT ( 'NONE',  ( -10.00000000000051337, 5.773502691895962435, -108.2500000040967763 ) ) ;
#39865=CARTESIAN_POINT ( 'NONE',  ( -10.81189881249999907, -6.242252689847864744, -105.4687500020483668 ) ) ;
#39867=CARTESIAN_POINT ( 'NONE',  ( -5.405949406250003975, -9.363379034771801557, -6.531250002048377468 ) ) ;
#39870=CARTESIAN_POINT ( 'NONE',  ( 5.405949406249999534, 9.363379034771803333, -109.2812500020483810 ) ) ;
#39874=CARTESIAN_POINT ( 'NONE',  ( -9.999999999999998224, 1.224646799147353059E-15, -84.12500000409677625 ) ) ;
#39875=CARTESIAN_POINT ( 'NONE',  ( 9.999999999999998224, 0.000000000000000000, -134.3750000040967905 ) ) ;
#39876=CARTESIAN_POINT ( 'NONE',  ( 10.81189881249999551, -6.242252689847874514, -35.96875000204835260 ) ) ;
#39881=AXIS2_PLACEMENT_3D ( 'NONE', #8889, #8039, #1569 ) ;
#39882=CARTESIAN_POINT ( 'NONE',  ( 9.999999999999996447, -5.773502691896262640, -14.50000000409676382 ) ) ;
#39897=VERTEX_POINT ( 'NONE', #26054 ) ;
#39899=CARTESIAN_POINT ( 'NONE',  ( 7.070501591499376803E-16, 11.54700538379251284, -128.0000000040967905 ) ) ;
#39900=CARTESIAN_POINT ( 'NONE',  ( -10.81189881249999729, 1.324075727343319199E-15, -173.2812500020484094 ) ) ;
#39904=CARTESIAN_POINT ( 'NONE',  ( -10.81189881249999729, 1.324075727343319199E-15, -95.09375000204838102 ) ) ;
#39906=CARTESIAN_POINT ( 'NONE',  ( 10.81189881249999551, -6.242252689847874514, -103.6562500020483668 ) ) ;
#39908=CARTESIAN_POINT ( 'NONE',  ( -5.405949406249996869, 9.363379034771805109, -113.3437500020483810 ) ) ;
#39911=CARTESIAN_POINT ( 'NONE',  ( -5.405949406249996869, 9.363379034771805109, -179.5312500020483810 ) ) ;
#39912=CARTESIAN_POINT ( 'NONE',  ( -5.405949406249996869, 9.363379034771805109, -199.0312500020484094 ) ) ;
#39916=CARTESIAN_POINT ( 'NONE',  ( 9.999999999999998224, 0.000000000000000000, -182.3750000040967905 ) ) ;
#39918=CARTESIAN_POINT ( 'NONE',  ( -2.293366432827344421E-15, -12.48450537969573659, -27.21875000204837747 ) ) ;
#39920=CARTESIAN_POINT ( 'NONE',  ( 7.644554776091147741E-16, 12.48450537969573659, -129.9687500020483810 ) ) ;
#39922=CARTESIAN_POINT ( 'NONE',  ( 10.81189881249999729, 0.000000000000000000, -37.53125000204838102 ) ) ;
#39925=CARTESIAN_POINT ( 'NONE',  ( -10.00000000000000000, -5.773502691896251982, -56.62499999999997868 ) ) ;
#39926=CARTESIAN_POINT ( 'NONE',  ( 5.405949406249999534, 9.363379034771803333, -128.7812500020483810 ) ) ;
#39928=VERTEX_POINT ( 'NONE', #19350 ) ;
#39930=CARTESIAN_POINT ( 'NONE',  ( -9.999999999999998224, 1.224646799147353059E-15, -108.1250000040967763 ) ) ;
#39931=CARTESIAN_POINT ( 'NONE',  ( -9.999999999999998224, 1.224646799147353059E-15, -161.7500000000000000 ) ) ;
#39932=CARTESIAN_POINT ( 'NONE',  ( -10.81189881249999729, 1.324075727343319199E-15, -63.59375000204836681 ) ) ;
#39936=CARTESIAN_POINT ( 'NONE',  ( -4.999999999999996447, 8.660254037844387298, -36.37500000409676915 ) ) ;
#39938=DIRECTION ( 'NONE',  ( -1.000000000000000000, 0.000000000000000000, 0.000000000000000000 ) ) ;
#39941=AXIS2_PLACEMENT_3D ( 'NONE', #1862, #40887, #1643 ) ;
#39943=ORIENTED_EDGE ( 'NONE', *, *, #5390, .F. ) ;
#39944=CARTESIAN_POINT ( 'NONE',  ( -10.00000000000076916, 5.773502691895813221, -126.2500000040967763 ) ) ;
#39947=CARTESIAN_POINT ( 'NONE',  ( 0.000000000000000000, 0.000000000000000000, -99.99999999999998579 ) ) ;
#39949=CARTESIAN_POINT ( 'NONE',  ( -9.999999999999998224, 0.000000000000000000, -99.99999999999998579 ) ) ;
#39950=CARTESIAN_POINT ( 'NONE',  ( 9.999999999999479527, 5.773502691896553074, -150.3750000000000000 ) ) ;
#39953=( BOUNDED_CURVE ( )  B_SPLINE_CURVE ( 2, ( #33059, #12958, #36291, #36076, #20087, #39727, #22704 ),
 .UNSPECIFIED., .F., .F. ) 
 B_SPLINE_CURVE_WITH_KNOTS ( ( 3, 2, 2, 3 ),
 ( 0.4029850746268657802, 0.4042288557213931655, 0.4054726368159204397, 0.4067164179104478250 ),
 .UNSPECIFIED. ) 
 CURVE ( )  GEOMETRIC_REPRESENTATION_ITEM ( )  RATIONAL_B_SPLINE_CURVE ( ( 0.9999999999999880096, 0.8660254037844506980, 1.000000000000000000, 0.8660254037844387076, 1.000000000000000000, 0.8660254037844327124, 1.000000000000005995 ) ) 
 REPRESENTATION_ITEM ( '' )  );
#39955=CARTESIAN_POINT ( 'NONE',  ( -5.405949406250003975, -9.363379034771801557, -129.3437500020484094 ) ) ;
#39956=CARTESIAN_POINT ( 'NONE',  ( 9.999999999999996447, -5.773502691896262640, -196.0000000040968189 ) ) ;
#39957=CARTESIAN_POINT ( 'NONE',  ( 10.81189881249999551, -6.242252689847874514, -133.6562500020483810 ) ) ;
#39959=CARTESIAN_POINT ( 'NONE',  ( 10.81189881249999729, 6.242252689847867408, -139.2187500020483810 ) ) ;
#39961=CARTESIAN_POINT ( 'NONE',  ( -9.999999999999998224, 0.000000000000000000, -99.99999999999998579 ) ) ;
#39963=CARTESIAN_POINT ( 'NONE',  ( 7.070501591499377789E-16, 11.54700538379251284, -157.6250000000000000 ) ) ;
#39968=CARTESIAN_POINT ( 'NONE',  ( -5.405949406250003975, -9.363379034771801557, -51.34375000204835260 ) ) ;
#39970=CARTESIAN_POINT ( 'NONE',  ( -5.405949406250003975, -9.363379034771801557, -160.8437500020484094 ) ) ;
#39973=DIRECTION ( 'NONE',  ( -1.000000000000000000, 0.000000000000000000, 0.000000000000000000 ) ) ;
#39974=CARTESIAN_POINT ( 'NONE',  ( 10.00000000000000000, 5.773502691896255534, -84.37499999999998579 ) ) ;
#39977=CARTESIAN_POINT ( 'NONE',  ( -10.81189881249999729, 1.324075727343319199E-15, -111.7812500020483810 ) ) ;
#39978=CARTESIAN_POINT ( 'NONE',  ( 9.999999999999996447, -5.773502691896262640, -136.0000000040967905 ) ) ;
#39979=CARTESIAN_POINT ( 'NONE',  ( -5.000000000000003553, -8.660254037844383745, -178.0000000000000000 ) ) ;
#39982=CARTESIAN_POINT ( 'NONE',  ( 0.000000000000000000, 0.000000000000000000, -99.99999999999998579 ) ) ;
#39983=CARTESIAN_POINT ( 'NONE',  ( -10.81189881249999729, 1.324075727343319199E-15, -48.78125000204838813 ) ) ;
#39996=( BOUNDED_CURVE ( )  B_SPLINE_CURVE ( 2, ( #32846, #38462, #2644, #18823, #29181, #32216, #39301 ),
 .UNSPECIFIED., .F., .F. ) 
 B_SPLINE_CURVE_WITH_KNOTS ( ( 3, 2, 2, 3 ),
 ( 0.2052238805970149627, 0.2064676616915423202, 0.2077114427860697055, 0.2089552238805970630 ),
 .UNSPECIFIED. ) 
 CURVE ( )  GEOMETRIC_REPRESENTATION_ITEM ( )  RATIONAL_B_SPLINE_CURVE ( ( 0.9999999999999970024, 0.8660254037844417052, 1.000000000000000000, 0.8660254037844387076, 1.000000000000000000, 0.8660254037844327124, 1.000000000000005995 ) ) 
 REPRESENTATION_ITEM ( '' )  );
#39998=AXIS2_PLACEMENT_3D ( 'NONE', #24743, #11112, #37889 ) ;
#40006=CARTESIAN_POINT ( 'NONE',  ( -10.81189881249999907, -6.242252689847864744, -151.9687500020484094 ) ) ;
#40007=CARTESIAN_POINT ( 'NONE',  ( -10.81189881249999729, 6.242252689847871849, -159.7187500020483810 ) ) ;
#40011=CARTESIAN_POINT ( 'NONE',  ( 7.070501591499377789E-16, 11.54700538379251284, -183.1250000000000000 ) ) ;
#40016=CARTESIAN_POINT ( 'NONE',  ( 10.81189881249999729, 0.000000000000000000, -184.3437500020483810 ) ) ;
#40019=CARTESIAN_POINT ( 'NONE',  ( -5.405949406249996869, 9.363379034771805109, -56.53125000204836681 ) ) ;
#40021=CARTESIAN_POINT ( 'NONE',  ( -9.999999999999998224, 1.224646799147353059E-15, -110.7499999999999858 ) ) ;
#40024=CARTESIAN_POINT ( 'NONE',  ( -10.81189881249999729, 6.242252689847871849, -137.4062500020484094 ) ) ;
#40025=CARTESIAN_POINT ( 'NONE',  ( -10.81189881249999729, 1.324075727343319199E-15, -149.2812500020483810 ) ) ;
#40027=CARTESIAN_POINT ( 'NONE',  ( 10.81189881249999551, -6.242252689847874514, -83.96875000204838102 ) ) ;
#40028=VERTEX_POINT ( 'NONE', #7466 ) ;
#40030=CARTESIAN_POINT ( 'NONE',  ( 10.81189881249999551, -6.242252689847874514, -178.4687500020484094 ) ) ;
#40033=CARTESIAN_POINT ( 'NONE',  ( 4.999999999999992006, -8.660254037844389075, -175.1250000040968189 ) ) ;
#40034=CARTESIAN_POINT ( 'NONE',  ( 10.81189881249999907, 6.242252689847868297, -73.40625000204836681 ) ) ;
#40036=CARTESIAN_POINT ( 'NONE',  ( 9.999999999999996447, -5.773502691896262640, -55.00000000409677625 ) ) ;
#40037=CARTESIAN_POINT ( 'NONE',  ( -5.405949406249996869, 9.363379034771805109, -11.34375000204834727 ) ) ;
#40040=CARTESIAN_POINT ( 'NONE',  ( -5.405949406249996869, 9.363379034771805109, -7.031250002048378356 ) ) ;
#40043=CARTESIAN_POINT ( 'NONE',  ( -9.999999999999998224, 1.224646799147353059E-15, -177.1250000040968189 ) ) ;
#40047=CARTESIAN_POINT ( 'NONE',  ( 10.00000000000012257, -5.773502691896187144, -160.0000000040968189 ) ) ;
#40048=CARTESIAN_POINT ( 'NONE',  ( -10.81189881249999729, 6.242252689847871849, -102.7187500020483810 ) ) ;
#40056=CARTESIAN_POINT ( 'NONE',  ( -2.121150477449813534E-15, -11.54700538379251284, -115.2500000040967905 ) ) ;
#40057=CARTESIAN_POINT ( 'NONE',  ( 5.000000000000000000, 8.660254037844385522, -45.24999999999998579 ) ) ;
#40060=CARTESIAN_POINT ( 'NONE',  ( -2.121150477449813534E-15, -11.54700538379251284, -121.2500000040967905 ) ) ;
#40061=CARTESIAN_POINT ( 'NONE',  ( -9.999999999999998224, 1.224646799147353059E-15, -172.2500000000000000 ) ) ;
#40062=CARTESIAN_POINT ( 'NONE',  ( 10.81189881249999907, 6.242252689847868297, -151.4062500020484094 ) ) ;
#40071=CARTESIAN_POINT ( 'NONE',  ( 10.81189881249999551, -6.242252689847874514, -70.46875000204839523 ) ) ;
#40072=CARTESIAN_POINT ( 'NONE',  ( 5.405949406249999534, 9.363379034771803333, -74.78125000204838102 ) ) ;
#40074=CARTESIAN_POINT ( 'NONE',  ( -5.405949406250003975, -9.363379034771801557, -159.5312500020484094 ) ) ;
#40075=CARTESIAN_POINT ( 'NONE',  ( -5.405949406250003975, -9.363379034771801557, -170.0312500020484094 ) ) ;
#40077=CARTESIAN_POINT ( 'NONE',  ( 10.00000000000051159, -5.773502691895965988, -145.0000000040967620 ) ) ;
#40079=CARTESIAN_POINT ( 'NONE',  ( 7.644554776091147741E-16, 12.48450537969573659, -108.9687500020483952 ) ) ;
#40081=CARTESIAN_POINT ( 'NONE',  ( -10.81189881249999729, 6.242252689847871849, -3.906250002048361480 ) ) ;
#40085=CARTESIAN_POINT ( 'NONE',  ( -10.81189881249999729, 6.242252689847871849, -102.9062500020483810 ) ) ;
#40087=CARTESIAN_POINT ( 'NONE',  ( -9.999999999999998224, 1.224646799147353059E-15, -73.62500000409677625 ) ) ;
#40088=CARTESIAN_POINT ( 'NONE',  ( -9.999999999999998224, 1.224646799147353059E-15, -145.6250000040967905 ) ) ;
#40089=CARTESIAN_POINT ( 'NONE',  ( -10.81189881249999729, 1.324075727343319199E-15, -32.09375000204836681 ) ) ;
#40092=CARTESIAN_POINT ( 'NONE',  ( -10.81189881249999729, 1.324075727343319199E-15, -29.28125000204837036 ) ) ;
#40095=CARTESIAN_POINT ( 'NONE',  ( -4.999999999999996447, 8.660254037844387298, -1.875000004096766260 ) ) ;
#40098=CARTESIAN_POINT ( 'NONE',  ( -10.00000000000025580, 5.773502691896109873, -122.8750000000000000 ) ) ;
#40102=ORIENTED_EDGE ( 'NONE', *, *, #38051, .F. ) ;
#40108=VERTEX_POINT ( 'NONE', #16518 ) ;
#40110=CARTESIAN_POINT ( 'NONE',  ( -10.81189881249999907, -6.242252689847864744, -170.1562500020483810 ) ) ;
#40113=CARTESIAN_POINT ( 'NONE',  ( -10.81189881249999907, -6.242252689847864744, -94.96875000204838102 ) ) ;
#40114=CARTESIAN_POINT ( 'NONE',  ( 5.405949406249999534, 9.363379034771803333, -199.0937500020484094 ) ) ;
#40115=CARTESIAN_POINT ( 'NONE',  ( -10.81189881249999907, -6.242252689847864744, -101.1562500020483952 ) ) ;
#40117=CARTESIAN_POINT ( 'NONE',  ( 5.405949406249999534, 9.363379034771803333, -104.5937500020483810 ) ) ;
#40120=( BOUNDED_CURVE ( )  B_SPLINE_CURVE ( 2, ( #6076, #26134, #28, #19223, #3047, #39076, #19016 ),
 .UNSPECIFIED., .F., .F. ) 
 B_SPLINE_CURVE_WITH_KNOTS ( ( 3, 2, 2, 3 ),
 ( 0.4104477611940299253, 0.4116915422885572551, 0.4129353233830846959, 0.4141791044776120256 ),
 .UNSPECIFIED. ) 
 CURVE ( )  GEOMETRIC_REPRESENTATION_ITEM ( )  RATIONAL_B_SPLINE_CURVE ( ( 0.9999999999999940048, 0.8660254037844447028, 1.000000000000000000, 0.8660254037844387076, 1.000000000000000000, 0.8660254037844267172, 1.000000000000011990 ) ) 
 REPRESENTATION_ITEM ( '' )  );
#40121=CARTESIAN_POINT ( 'NONE',  ( -2.121150477449813534E-15, -11.54700538379251284, -104.7500000040967763 ) ) ;
#40122=CARTESIAN_POINT ( 'NONE',  ( -9.999999999999998224, 1.224646799147353059E-15, -132.1250000040967620 ) ) ;
#40123=CARTESIAN_POINT ( 'NONE',  ( 5.405949406249999534, 9.363379034771803333, -193.2812500020484094 ) ) ;
#40126=CARTESIAN_POINT ( 'NONE',  ( 9.999999999999998224, 0.000000000000000000, -168.8750000040967905 ) ) ;
#40128=CARTESIAN_POINT ( 'NONE',  ( 5.405949406249992428, -9.363379034771808662, -25.59375000204835970 ) ) ;
#40130=CARTESIAN_POINT ( 'NONE',  ( 5.405949406249992428, -9.363379034771808662, -132.0937500020483810 ) ) ;
#40133=CARTESIAN_POINT ( 'NONE',  ( -2.293366432827344421E-15, -12.48450537969573659, -25.90625000204838102 ) ) ;
#40136=CARTESIAN_POINT ( 'NONE',  ( -9.999999999999998224, 5.773502691896259087, -56.87499999999998579 ) ) ;
#40137=CARTESIAN_POINT ( 'NONE',  ( 10.81189881249999907, 6.242252689847868297, -127.4062500020483810 ) ) ;
#40141=CARTESIAN_POINT ( 'NONE',  ( 7.070501591499377789E-16, 11.54700538379251284, -101.0000000040967905 ) ) ;
#40142=CARTESIAN_POINT ( 'NONE',  ( -9.999999999999479527, -5.773502691896549521, -146.6249999999999716 ) ) ;
#40143=CARTESIAN_POINT ( 'NONE',  ( 10.81189881249999907, 6.242252689847868297, -56.71875000204838813 ) ) ;
#40146=VECTOR ( 'NONE', #40980, 1000.000000000000000 ) ;
#40148=CARTESIAN_POINT ( 'NONE',  ( -9.999999999999998224, 1.224646799147353059E-15, -36.12500000409676915 ) ) ;
#40152=ORIENTED_EDGE ( 'NONE', *, *, #12373, .T. ) ;
#40153=VERTEX_POINT ( 'NONE', #40250 ) ;
#40157=CARTESIAN_POINT ( 'NONE',  ( -10.81189881249999729, 1.324075727343319199E-15, -198.7812500020484094 ) ) ;
#40163=CARTESIAN_POINT ( 'NONE',  ( -2.293366432827344421E-15, -12.48450537969573659, -117.2187500020483952 ) ) ;
#40164=CARTESIAN_POINT ( 'NONE',  ( 7.070501591499377789E-16, 11.54700538379251284, -197.0000000040968189 ) ) ;
#40165=CARTESIAN_POINT ( 'NONE',  ( -5.405949406250003975, -9.363379034771801557, -125.0312500020483952 ) ) ;
#40167=CARTESIAN_POINT ( 'NONE',  ( 10.81189881249999729, 0.000000000000000000, -142.3437500020483810 ) ) ;
#40170=CARTESIAN_POINT ( 'NONE',  ( 5.000000000000000000, 8.660254037844385522, -159.2500000000000000 ) ) ;
#40171=CARTESIAN_POINT ( 'NONE',  ( -10.00000000000000000, -5.773502691896251982, -19.12499999999997513 ) ) ;
#40175=CARTESIAN_POINT ( 'NONE',  ( -5.405949406249996869, 9.363379034771805109, -45.84375000204838102 ) ) ;
#40177=CARTESIAN_POINT ( 'NONE',  ( 10.81189881249999907, 6.242252689847868297, -151.2187500020483810 ) ) ;
#40181=CARTESIAN_POINT ( 'NONE',  ( 1.917121039151881590, 10.12589884400897056, -180.0000000000000853 ) ) ;
#40182=CARTESIAN_POINT ( 'NONE',  ( -4.999999999999996447, 8.660254037844387298, -82.49999999999998579 ) ) ;
#40184=ADVANCED_FACE ( 'NONE', ( #10686 ), #39833, .F. ) ;
#40185=ORIENTED_EDGE ( 'NONE', *, *, #2738, .F. ) ;
#40186=CARTESIAN_POINT ( 'NONE',  ( -10.81189881249999729, 1.324075727343319199E-15, -108.7812500020483810 ) ) ;
#40187=CARTESIAN_POINT ( 'NONE',  ( -9.999999999999998224, 1.224646799147353059E-15, -132.1250000040967620 ) ) ;
#40188=CARTESIAN_POINT ( 'NONE',  ( 9.999999999999998224, 0.000000000000000000, -164.0000000000000000 ) ) ;
#40193=CARTESIAN_POINT ( 'NONE',  ( -10.81189881249999729, 1.324075727343319199E-15, -51.78125000204835970 ) ) ;
#40199=VERTEX_POINT ( 'NONE', #581 ) ;
#40212=CARTESIAN_POINT ( 'NONE',  ( 5.405949406249999534, 9.363379034771803333, -142.0937500020483810 ) ) ;
#40213=CARTESIAN_POINT ( 'NONE',  ( 10.81189881249999551, -6.242252689847874514, -158.9687500020484094 ) ) ;
#40216=CARTESIAN_POINT ( 'NONE',  ( -9.999999999999998224, 1.224646799147353059E-15, -182.7500000000000000 ) ) ;
#40218=CARTESIAN_POINT ( 'NONE',  ( -10.00000000000076916, 5.773502691895813221, -137.8750000000000000 ) ) ;
#40220=DIRECTION ( 'NONE',  ( -1.000000000000000000, 0.000000000000000000, 0.000000000000000000 ) ) ;
#40221=CARTESIAN_POINT ( 'NONE',  ( 10.81189881249999907, 6.242252689847868297, -175.2187500020484094 ) ) ;
#40224=CARTESIAN_POINT ( 'NONE',  ( 5.405949406249999534, 9.363379034771803333, -53.78125000204836681 ) ) ;
#40226=CARTESIAN_POINT ( 'NONE',  ( -10.00000000000000000, -5.773502691896251982, -106.1249999999999858 ) ) ;
#40228=CARTESIAN_POINT ( 'NONE',  ( 5.405949406249999534, 9.363379034771803333, -133.2812500020483810 ) ) ;
#40229=CARTESIAN_POINT ( 'NONE',  ( 5.405949406249999534, 9.363379034771803333, -148.2812500020483810 ) ) ;
#40231=CARTESIAN_POINT ( 'NONE',  ( 10.81189881249999907, 6.242252689847868297, -83.71875000204836681 ) ) ;
#40234=CARTESIAN_POINT ( 'NONE',  ( -5.405949406250003975, -9.363379034771801557, -177.3437500020483810 ) ) ;
#40237=CARTESIAN_POINT ( 'NONE',  ( -2.293366432827344421E-15, -12.48450537969573659, -76.90625000204839523 ) ) ;
#40239=CARTESIAN_POINT ( 'NONE',  ( -10.00000000000000000, -5.773502691896251982, -55.50000000409676915 ) ) ;
#40240=CARTESIAN_POINT ( 'NONE',  ( -2.293366432827344421E-15, -12.48450537969573659, -9.218750002048359704 ) ) ;
#40244=CARTESIAN_POINT ( 'NONE',  ( 7.644554776091147741E-16, 12.48450537969573659, -2.656250002048360592 ) ) ;
#40245=DIRECTION ( 'NONE',  ( 1.000000000000000000, 0.000000000000000000, 0.000000000000000000 ) ) ;
#40250=CARTESIAN_POINT ( 'NONE',  ( 9.999999999999998224, 0.000000000000000000, -165.5000000000000000 ) ) ;
#40252=ORIENTED_EDGE ( 'NONE', *, *, #35728, .F. ) ;
#40255=ORIENTED_EDGE ( 'NONE', *, *, #18282, .F. ) ;
#40258=( BOUNDED_CURVE ( )  B_SPLINE_CURVE ( 2, ( #26826, #14053, #4160, #36747, #17305, #26404, #6758 ),
 .UNSPECIFIED., .F., .F. ) 
 B_SPLINE_CURVE_WITH_KNOTS ( ( 3, 2, 2, 3 ),
 ( 0.4365671641791046276, 0.4378109452736320129, 0.4390547263681593981, 0.4402985074626867279 ),
 .UNSPECIFIED. ) 
 CURVE ( )  GEOMETRIC_REPRESENTATION_ITEM ( )  RATIONAL_B_SPLINE_CURVE ( ( 0.9999999999999820144, 0.8660254037844566932, 1.000000000000000000, 0.8660254037844387076, 1.000000000000000000, 0.8660254037844207220, 1.000000000000017986 ) ) 
 REPRESENTATION_ITEM ( '' )  );
#40261=CARTESIAN_POINT ( 'NONE',  ( 5.000000000000000000, 8.660254037844385522, -42.24999999999997868 ) ) ;
#40263=CARTESIAN_POINT ( 'NONE',  ( 10.81189881249999907, 6.242252689847868297, -164.7187500020483810 ) ) ;
#40266=CARTESIAN_POINT ( 'NONE',  ( 4.999999999999992006, -8.660254037844389075, -167.6250000040967905 ) ) ;
#40267=CARTESIAN_POINT ( 'NONE',  ( -4.999999999999996447, 8.660254037844387298, -144.0000000000000000 ) ) ;
#40273=CARTESIAN_POINT ( 'NONE',  ( -10.81189881249999729, 1.324075727343319199E-15, -71.09375000204836681 ) ) ;
#40274=CARTESIAN_POINT ( 'NONE',  ( 10.81189881249999729, 0.000000000000000000, -79.53125000204838102 ) ) ;
#40276=CARTESIAN_POINT ( 'NONE',  ( -2.293366432827344421E-15, -12.48450537969573659, -156.4062500020484379 ) ) ;
#40277=CARTESIAN_POINT ( 'NONE',  ( -5.405949406250003975, -9.363379034771801557, -173.0312500020484094 ) ) ;
#40278=CARTESIAN_POINT ( 'NONE',  ( -5.405949406250003975, -9.363379034771801557, -0.3437500020483652552 ) ) ;
#40279=CARTESIAN_POINT ( 'NONE',  ( 9.999999999999998224, 1.224646799147353059E-15, -99.99999999999998579 ) ) ;
#40280=CARTESIAN_POINT ( 'NONE',  ( -5.405949406249996869, 9.363379034771805109, -108.8437500020483810 ) ) ;
#40283=CARTESIAN_POINT ( 'NONE',  ( -10.81189881249999907, -6.242252689847864744, -6.656250002048364145 ) ) ;
#40286=CARTESIAN_POINT ( 'NONE',  ( -2.293366432827344421E-15, -12.48450537969573659, -99.40625000204839523 ) ) ;
#40288=CARTESIAN_POINT ( 'NONE',  ( -4.999999999999996447, 8.660254037844387298, -76.87500000409677625 ) ) ;
#40290=CARTESIAN_POINT ( 'NONE',  ( 5.405949406249992428, -9.363379034771808662, -36.09375000204836681 ) ) ;
#40293=CARTESIAN_POINT ( 'NONE',  ( 10.81189881249999907, 6.242252689847868297, -31.40625000204835615 ) ) ;
#40295=CARTESIAN_POINT ( 'NONE',  ( -10.00000000000000000, -5.773502691896251982, -6.000000004096756712 ) ) ;
#40313=CARTESIAN_POINT ( 'NONE',  ( -5.405949406250003975, -9.363379034771801557, -173.0312500020484094 ) ) ;
#40317=CARTESIAN_POINT ( 'NONE',  ( -10.81189881249999729, 6.242252689847871849, -95.21875000204838102 ) ) ;
#40319=CARTESIAN_POINT ( 'NONE',  ( 5.405949406249992428, -9.363379034771808662, -100.7812500020483952 ) ) ;
#40321=CARTESIAN_POINT ( 'NONE',  ( 5.405949406249992428, -9.363379034771808662, -108.0937500020483810 ) ) ;
#40323=AXIS2_PLACEMENT_3D ( 'NONE', #23158, #36321, #17723 ) ;
#40325=CARTESIAN_POINT ( 'NONE',  ( 9.999999999999998224, 0.000000000000000000, -132.8750000040967905 ) ) ;
#40326=CARTESIAN_POINT ( 'NONE',  ( -10.81189881249999729, 1.324075727343319199E-15, -195.7812500020484094 ) ) ;
#40329=CARTESIAN_POINT ( 'NONE',  ( 9.999999999999996447, -5.773502691896262640, -172.0000000040967905 ) ) ;
#40331=CARTESIAN_POINT ( 'NONE',  ( 10.81189881249999907, 6.242252689847868297, -23.71875000204837036 ) ) ;
#40332=CYLINDRICAL_SURFACE ( 'NONE', #2686, 9.999999999999998224 ) ;
#40333=CARTESIAN_POINT ( 'NONE',  ( -5.405949406250003975, -9.363379034771801557, -132.3437500020484094 ) ) ;
#40335=CARTESIAN_POINT ( 'NONE',  ( -10.81189881249999729, 6.242252689847871849, -32.40625000204835970 ) ) ;
#40336=CARTESIAN_POINT ( 'NONE',  ( 5.000000000000000000, 8.660254037844385522, -102.2500000000000000 ) ) ;
#40337=CARTESIAN_POINT ( 'NONE',  ( 4.999999999999992006, -8.660254037844389075, -56.24999999999996447 ) ) ;
#40338=CARTESIAN_POINT ( 'NONE',  ( 10.81189881249999907, 6.242252689847868297, -124.4062500020483810 ) ) ;
#40342=CARTESIAN_POINT ( 'NONE',  ( -5.000000000000003553, -8.660254037844383745, -103.3750000040967763 ) ) ;
#40344=CARTESIAN_POINT ( 'NONE',  ( 7.644554776091147741E-16, 12.48450537969573659, -60.96875000204838102 ) ) ;
#40349=CARTESIAN_POINT ( 'NONE',  ( 9.999999999999998224, 0.000000000000000000, -24.87500000409675849 ) ) ;
#40351=CARTESIAN_POINT ( 'NONE',  ( -2.121150477449813534E-15, -11.54700538379251284, -138.8750000000000000 ) ) ;
#40359=( BOUNDED_CURVE ( )  B_SPLINE_CURVE ( 2, ( #18912, #25820, #29266, #35332, #3152, #5759, #19535 ),
 .UNSPECIFIED., .F., .F. ) 
 B_SPLINE_CURVE_WITH_KNOTS ( ( 3, 2, 2, 3 ),
 ( 0.4701492537313434195, 0.4713930348258707492, 0.4726368159203981900, 0.4738805970149255198 ),
 .UNSPECIFIED. ) 
 CURVE ( )  GEOMETRIC_REPRESENTATION_ITEM ( )  RATIONAL_B_SPLINE_CURVE ( ( 0.9999999999999880096, 0.8660254037844506980, 1.000000000000000000, 0.8660254037844387076, 1.000000000000000000, 0.8660254037844207220, 1.000000000000017986 ) ) 
 REPRESENTATION_ITEM ( '' )  );
#40361=CARTESIAN_POINT ( 'NONE',  ( 10.81189881249999551, -6.242252689847874514, -195.1562500020484379 ) ) ;
#40367=CARTESIAN_POINT ( 'NONE',  ( 7.644554776091147741E-16, 12.48450537969573659, -117.9687500020483668 ) ) ;
#40368=CARTESIAN_POINT ( 'NONE',  ( -9.999999999999998224, 1.224646799147353059E-15, -193.6250000040967905 ) ) ;
#40369=CARTESIAN_POINT ( 'NONE',  ( 5.405949406249992428, -9.363379034771808662, -124.7812500020483952 ) ) ;
#40371=CARTESIAN_POINT ( 'NONE',  ( -10.81189881249999729, 1.324075727343319199E-15, -126.5937500020483668 ) ) ;
#40373=CARTESIAN_POINT ( 'NONE',  ( -2.121150477449813534E-15, -11.54700538379251284, -155.3750000000000000 ) ) ;
#40374=CARTESIAN_POINT ( 'NONE',  ( -2.121150477449813534E-15, -11.54700538379251284, -21.87499999999997868 ) ) ;
#40377=CARTESIAN_POINT ( 'NONE',  ( 0.000000000000000000, 0.000000000000000000, -99.99999999999998579 ) ) ;
#40379=CARTESIAN_POINT ( 'NONE',  ( 10.81189881249999729, 0.000000000000000000, -43.34375000204837391 ) ) ;
#40381=CARTESIAN_POINT ( 'NONE',  ( 5.405949406249992428, -9.363379034771808662, -153.0937500020483810 ) ) ;
#40384=CARTESIAN_POINT ( 'NONE',  ( -4.999999999999996447, 8.660254037844387298, -80.99999999999998579 ) ) ;
#40386=ORIENTED_EDGE ( 'NONE', *, *, #40453, .T. ) ;
#40387=CARTESIAN_POINT ( 'NONE',  ( -10.81189881249999729, 6.242252689847871849, -107.4062500020483668 ) ) ;
#40388=CARTESIAN_POINT ( 'NONE',  ( 5.000000000000000000, 8.660254037844385522, -125.1250000040967620 ) ) ;
#40391=CARTESIAN_POINT ( 'NONE',  ( -10.81189881249999729, 6.242252689847871849, -54.90625000204837391 ) ) ;
#40397=CARTESIAN_POINT ( 'NONE',  ( 7.070501591499376803E-16, 11.54700538379251284, -164.0000000040967905 ) ) ;
#40406=CARTESIAN_POINT ( 'NONE',  ( -10.00000000000051337, 5.773502691895962435, -103.3749999999999858 ) ) ;
#40410=DIRECTION ( 'NONE',  ( -0.000000000000000000, -0.000000000000000000, -1.000000000000000000 ) ) ;
#40415=CARTESIAN_POINT ( 'NONE',  ( -10.81189881249999729, 6.242252689847871849, -140.2187500020483810 ) ) ;
#40416=CARTESIAN_POINT ( 'NONE',  ( -5.405949406249996869, 9.363379034771805109, -158.3437500020483810 ) ) ;
#40419=CARTESIAN_POINT ( 'NONE',  ( 5.000000000000000000, 8.660254037844385522, -175.7500000000000284 ) ) ;
#40424=CARTESIAN_POINT ( 'NONE',  ( 5.405949406249999534, 9.363379034771803333, -181.0937500020483810 ) ) ;
#40428=CARTESIAN_POINT ( 'NONE',  ( -10.81189881249999907, -6.242252689847864744, -51.65625000204837391 ) ) ;
#40430=CARTESIAN_POINT ( 'NONE',  ( 5.000000000000000000, 8.660254037844385522, -111.2499999999999858 ) ) ;
#40432=CARTESIAN_POINT ( 'NONE',  ( -5.405949406249996869, 9.363379034771805109, -133.0312500020484094 ) ) ;
#40433=CARTESIAN_POINT ( 'NONE',  ( -9.999999999999998224, 1.224646799147353059E-15, -148.6250000040967905 ) ) ;
#40434=CARTESIAN_POINT ( 'NONE',  ( -10.81189881249999907, -6.242252689847864744, -152.1562500020484094 ) ) ;
#40439=CARTESIAN_POINT ( 'NONE',  ( -10.81189881249999729, 1.324075727343319199E-15, -180.5937500020484094 ) ) ;
#40442=CARTESIAN_POINT ( 'NONE',  ( -2.121150477449813534E-15, -11.54700538379251284, -110.3749999999999858 ) ) ;
#40443=DIRECTION ( 'NONE',  ( -0.000000000000000000, -0.000000000000000000, -1.000000000000000000 ) ) ;
#40444=CARTESIAN_POINT ( 'NONE',  ( 10.81189881249999729, 0.000000000000000000, -78.03125000204838102 ) ) ;
#40446=CARTESIAN_POINT ( 'NONE',  ( 4.999999999999992006, -8.660254037844389075, -52.12500000409675494 ) ) ;
#40447=CARTESIAN_POINT ( 'NONE',  ( -5.405949406250003975, -9.363379034771801557, -12.34375000204834905 ) ) ;
#40448=DIRECTION ( 'NONE',  ( -0.000000000000000000, -0.000000000000000000, -1.000000000000000000 ) ) ;
#40450=CARTESIAN_POINT ( 'NONE',  ( 10.81189881249999729, 0.000000000000000000, -3.031250002048374803 ) ) ;
#40452=CARTESIAN_POINT ( 'NONE',  ( 9.999999999999998224, 0.000000000000000000, -106.9999999999999858 ) ) ;
#40453=EDGE_CURVE ( 'NONE', #27421, #13539, #37671, .T. ) ;
#40455=DIRECTION ( 'NONE',  ( -1.000000000000000000, 0.000000000000000000, 0.000000000000000000 ) ) ;
#40459=ORIENTED_EDGE ( 'NONE', *, *, #14833, .T. ) ;
#40466=CARTESIAN_POINT ( 'NONE',  ( -2.121150477449813534E-15, -11.54700538379251284, -44.37499999999997158 ) ) ;
#40468=CARTESIAN_POINT ( 'NONE',  ( 5.405949406249999534, 9.363379034771803333, -167.5937500020484094 ) ) ;
#40472=CARTESIAN_POINT ( 'NONE',  ( -9.999999999999998224, 1.224646799147353059E-15, -125.7499999999999716 ) ) ;
#40479=CARTESIAN_POINT ( 'NONE',  ( 10.81189881249999551, -6.242252689847874514, -67.46875000204838102 ) ) ;
#40480=CARTESIAN_POINT ( 'NONE',  ( -10.81189881249999729, 6.242252689847871849, -77.40625000204838102 ) ) ;
#40482=CARTESIAN_POINT ( 'NONE',  ( -5.000000000000003553, -8.660254037844383745, -134.5000000000000000 ) ) ;
#40484=CARTESIAN_POINT ( 'NONE',  ( -2.293366432827344421E-15, -12.48450537969573659, -160.9062500020483810 ) ) ;
#40485=CARTESIAN_POINT ( 'NONE',  ( -5.405949406250003975, -9.363379034771801557, -171.5312500020484094 ) ) ;
#40486=DIRECTION ( 'NONE',  ( 0.000000000000000000, 0.000000000000000000, 1.000000000000000000 ) ) ;
#40488=CARTESIAN_POINT ( 'NONE',  ( 5.405949406249999534, 9.363379034771803333, -106.0937500020483810 ) ) ;
#40491=CARTESIAN_POINT ( 'NONE',  ( -2.293366432827344421E-15, -12.48450537969573659, -3.406250002048361036 ) ) ;
#40494=CARTESIAN_POINT ( 'NONE',  ( 10.81189881249999551, -6.242252689847874514, -97.65625000204839523 ) ) ;
#40497=CARTESIAN_POINT ( 'NONE',  ( 4.999999999999992006, -8.660254037844389075, -79.12500000409677625 ) ) ;
#40499=CARTESIAN_POINT ( 'NONE',  ( -10.81189881249999729, 1.324075727343319199E-15, -38.09375000204837391 ) ) ;
#40502=CARTESIAN_POINT ( 'NONE',  ( 5.405949406249992428, -9.363379034771808662, -31.78125000204837391 ) ) ;
#40504=CARTESIAN_POINT ( 'NONE',  ( -4.999999999999996447, 8.660254037844387298, -160.5000000000000000 ) ) ;
#40505=CARTESIAN_POINT ( 'NONE',  ( 4.999999999999992006, -8.660254037844389075, -7.125000004096743389 ) ) ;
#40511=VERTEX_POINT ( 'NONE', #18015 ) ;
#40514=ORIENTED_EDGE ( 'NONE', *, *, #12373, .F. ) ;
#40522=CARTESIAN_POINT ( 'NONE',  ( 10.81189881249999729, 0.000000000000000000, -169.5312500020484094 ) ) ;
#40526=CARTESIAN_POINT ( 'NONE',  ( 5.405949406249999534, 9.363379034771803333, -94.09375000204838102 ) ) ;
#40528=CARTESIAN_POINT ( 'NONE',  ( -10.00000000000051337, 5.773502691895962435, -106.3749999999999716 ) ) ;
#40529=CARTESIAN_POINT ( 'NONE',  ( 7.644554776091147741E-16, 12.48450537969573659, -100.1562500020483952 ) ) ;
#40531=CARTESIAN_POINT ( 'NONE',  ( -10.81189881249999729, -6.242252689847864744, -109.9687500020483810 ) ) ;
#40535=CARTESIAN_POINT ( 'NONE',  ( -10.81189881249999729, 6.242252689847871849, -197.4062500020484379 ) ) ;
#40538=CARTESIAN_POINT ( 'NONE',  ( -9.999999999999998224, 1.224646799147353059E-15, -175.6250000040968189 ) ) ;
#40540=CARTESIAN_POINT ( 'NONE',  ( -10.81189881249999729, 1.324075727343319199E-15, -20.09375000204835615 ) ) ;
#40542=CARTESIAN_POINT ( 'NONE',  ( 5.405949406249992428, -9.363379034771808662, -133.5937500020483810 ) ) ;
#40544=CARTESIAN_POINT ( 'NONE',  ( -2.293366432827344421E-15, -12.48450537969573659, -27.40625000204838102 ) ) ;
#40547=CARTESIAN_POINT ( 'NONE',  ( 4.999999999999992006, -8.660254037844389075, -60.74999999999997158 ) ) ;
#40548=CARTESIAN_POINT ( 'NONE',  ( -2.293366432827344421E-15, -12.48450537969573659, -127.9062500020483952 ) ) ;
#40552=CARTESIAN_POINT ( 'NONE',  ( 4.999999999999992006, -8.660254037844389075, -117.7500000000000000 ) ) ;
#40553=CARTESIAN_POINT ( 'NONE',  ( -4.999999999999996447, 8.660254037844387298, -102.3750000040967905 ) ) ;
#40556=CARTESIAN_POINT ( 'NONE',  ( -5.405949406249996869, 9.363379034771805109, -59.34375000204835970 ) ) ;
#40561=CARTESIAN_POINT ( 'NONE',  ( 0.000000000000000000, 0.000000000000000000, -99.99999999999998579 ) ) ;
#40562=CARTESIAN_POINT ( 'NONE',  ( 7.070501591499377789E-16, 11.54700538379251284, -32.00000000409674783 ) ) ;
#40571=CYLINDRICAL_SURFACE ( 'NONE', #25229, 9.999999999999998224 ) ;
#40575=CARTESIAN_POINT ( 'NONE',  ( 10.81189881249999907, 6.242252689847868297, -193.4062500020484094 ) ) ;
#40582=CARTESIAN_POINT ( 'NONE',  ( -10.81189881249999907, -6.242252689847864744, -120.4687500020483810 ) ) ;
#40583=CARTESIAN_POINT ( 'NONE',  ( 9.999999999999998224, 0.000000000000000000, -198.8750000040967905 ) ) ;
#40584=CARTESIAN_POINT ( 'NONE',  ( -5.405949406250003975, -9.363379034771801557, -128.0312500020484094 ) ) ;
#40586=CARTESIAN_POINT ( 'NONE',  ( -10.81189881249999729, -6.242252689847864744, -132.4687500020483810 ) ) ;
#40589=CARTESIAN_POINT ( 'NONE',  ( -4.999999999999996447, 8.660254037844387298, -156.0000000000000000 ) ) ;
#40590=CARTESIAN_POINT ( 'NONE',  ( -2.121150477449813534E-15, -11.54700538379251284, -17.37499999999997513 ) ) ;
#40595=CARTESIAN_POINT ( 'NONE',  ( 7.644554776091147741E-16, 12.48450537969573659, -47.46875000204836681 ) ) ;
#40596=CARTESIAN_POINT ( 'NONE',  ( -10.81189881249999907, -6.242252689847864744, -151.9687500020484094 ) ) ;
#40600=CARTESIAN_POINT ( 'NONE',  ( -10.00000000000000000, -5.773502691896251982, -82.12499999999998579 ) ) ;
#40603=CARTESIAN_POINT ( 'NONE',  ( -10.81189881249999729, 1.324075727343319199E-15, -102.7812500020483952 ) ) ;
#40604=CARTESIAN_POINT ( 'NONE',  ( 7.070501591499377789E-16, 11.54700538379251284, -120.5000000040967905 ) ) ;
#40608=CARTESIAN_POINT ( 'NONE',  ( -2.293366432827344421E-15, -12.48450537969573659, -52.90625000204837391 ) ) ;
#40612=CARTESIAN_POINT ( 'NONE',  ( 5.000000000000000000, 8.660254037844385522, -109.7499999999999858 ) ) ;
#40615=VERTEX_POINT ( 'NONE', #21904 ) ;
#40628=CARTESIAN_POINT ( 'NONE',  ( -2.293366432827344421E-15, -12.48450537969573659, -144.2187500020483810 ) ) ;
#40629=CARTESIAN_POINT ( 'NONE',  ( 7.644554776091147741E-16, 12.48450537969573659, -153.9687500020484094 ) ) ;
#40631=CYLINDRICAL_SURFACE ( 'NONE', #5469, 9.999999999999998224 ) ;
#40632=CARTESIAN_POINT ( 'NONE',  ( 4.999999999999992006, -8.660254037844389075, -180.7500000000000284 ) ) ;
#40635=DIRECTION ( 'NONE',  ( -1.000000000000000000, 0.000000000000000000, 0.000000000000000000 ) ) ;
#40638=CARTESIAN_POINT ( 'NONE',  ( 5.405949406249992428, -9.363379034771808662, -180.0937500020484094 ) ) ;
#40641=CYLINDRICAL_SURFACE ( 'NONE', #16492, 9.999999999999998224 ) ;
#40642=CARTESIAN_POINT ( 'NONE',  ( -10.81189881249999907, -6.242252689847864744, -47.15625000204837391 ) ) ;
#40644=CARTESIAN_POINT ( 'NONE',  ( -2.121150477449813534E-15, -11.54700538379251284, -108.8749999999999858 ) ) ;
#40646=CARTESIAN_POINT ( 'NONE',  ( 7.644554776091147741E-16, 12.48450537969573659, -122.6562500020483952 ) ) ;
#40647=CARTESIAN_POINT ( 'NONE',  ( 5.000000000000000000, 8.660254037844385522, -147.6250000040967905 ) ) ;
#40651=CARTESIAN_POINT ( 'NONE',  ( -5.405949406249996869, 9.363379034771805109, -180.8437500020483810 ) ) ;
#40656=EDGE_CURVE ( 'NONE', #18647, #36180, #39270, .T. ) ;
#40657=CARTESIAN_POINT ( 'NONE',  ( -5.405949406250003975, -9.363379034771801557, -75.53125000204838102 ) ) ;
#40659=CARTESIAN_POINT ( 'NONE',  ( -9.999999999999998224, 5.773502691896259087, -55.75000000409677625 ) ) ;
#40660=CARTESIAN_POINT ( 'NONE',  ( -10.81189881249999729, 1.324075727343319199E-15, -11.09375000204834727 ) ) ;
#40661=DIRECTION ( 'NONE',  ( -1.000000000000000000, 0.000000000000000000, 0.000000000000000000 ) ) ;
#40663=CARTESIAN_POINT ( 'NONE',  ( -10.81189881249999907, -6.242252689847864744, -2.156250002048359704 ) ) ;
#40665=CARTESIAN_POINT ( 'NONE',  ( 5.000000000000000000, 8.660254037844385522, -148.7500000000000000 ) ) ;
#40669=AXIS2_PLACEMENT_3D ( 'NONE', #1052, #4928, #14826 ) ;
#40672=( NAMED_UNIT ( * ) SI_UNIT ( $, .STERADIAN. ) SOLID_ANGLE_UNIT ( ) );
#40675=EDGE_LOOP ( 'NONE', ( #24257, #944, #15928, #24039 ) ) ;
#40676=ORIENTED_EDGE ( 'NONE', *, *, #5559, .F. ) ;
#40681=CARTESIAN_POINT ( 'NONE',  ( -2.121150477449813534E-15, -11.54700538379251284, -122.3749999999999858 ) ) ;
#40682=CARTESIAN_POINT ( 'NONE',  ( 9.999999999999996447, -5.773502691896262640, -41.12499999999997158 ) ) ;
#40685=CARTESIAN_POINT ( 'NONE',  ( -2.293366432827344421E-15, -12.48450537969573659, -162.2187500020483810 ) ) ;
#40686=CARTESIAN_POINT ( 'NONE',  ( 10.81189881249999729, 0.000000000000000000, -178.3437500020483810 ) ) ;
#40688=LINE ( 'NONE', #24331, #19851 ) ;
#40689=CARTESIAN_POINT ( 'NONE',  ( 9.999999999999998224, 0.000000000000000000, -126.5000000000000000 ) ) ;
#40695=CARTESIAN_POINT ( 'NONE',  ( 5.405949406249999534, 9.363379034771803333, -73.09375000204838102 ) ) ;
#40696=CARTESIAN_POINT ( 'NONE',  ( -5.405949406249996869, 9.363379034771805109, -76.03125000204838102 ) ) ;
#40698=CARTESIAN_POINT ( 'NONE',  ( 9.999999999999996447, -5.773502691896262640, -128.1249999999999716 ) ) ;
#40699=CARTESIAN_POINT ( 'NONE',  ( 5.405949406249992428, -9.363379034771808662, -157.7812500020484094 ) ) ;
#40700=CARTESIAN_POINT ( 'NONE',  ( 5.405949406249992428, -9.363379034771808662, -171.2812500020484094 ) ) ;
#40704=CARTESIAN_POINT ( 'NONE',  ( 10.81189881249999907, 6.242252689847868297, -104.7187500020483810 ) ) ;
#40705=DIRECTION ( 'NONE',  ( -0.000000000000000000, -0.000000000000000000, -1.000000000000000000 ) ) ;
#40707=CARTESIAN_POINT ( 'NONE',  ( -10.81189881249999907, -6.242252689847864744, -8.156250002048365033 ) ) ;
#40711=CARTESIAN_POINT ( 'NONE',  ( 10.81189881249999907, 6.242252689847868297, -101.9062500020484094 ) ) ;
#40713=EDGE_CURVE ( 'NONE', #26528, #36280, #25162, .T. ) ;
#40714=CARTESIAN_POINT ( 'NONE',  ( -5.000000000000003553, -8.660254037844383745, -79.37500000409677625 ) ) ;
#40715=CARTESIAN_POINT ( 'NONE',  ( -10.00000000000025580, 5.773502691896109873, -118.3750000000000142 ) ) ;
#40716=CARTESIAN_POINT ( 'NONE',  ( 10.81189881249999551, -6.242252689847874514, -37.46875000204835970 ) ) ;
#40720=CARTESIAN_POINT ( 'NONE',  ( 10.81189881249999551, -6.242252689847874514, -25.65625000204838102 ) ) ;
#40723=CARTESIAN_POINT ( 'NONE',  ( 9.999999999999996447, -5.773502691896262640, -1.000000004096751605 ) ) ;
#40738=DIRECTION ( 'NONE',  ( -0.000000000000000000, -0.000000000000000000, -1.000000000000000000 ) ) ;
#40742=CARTESIAN_POINT ( 'NONE',  ( -2.293366432827344421E-15, -12.48450537969573659, -162.4062500020483810 ) ) ;
#40745=CARTESIAN_POINT ( 'NONE',  ( -5.405949406249996869, 9.363379034771805109, -90.84375000204838102 ) ) ;
#40747=CARTESIAN_POINT ( 'NONE',  ( -10.81189881249999729, 6.242252689847871849, -198.7187500020484379 ) ) ;
#40748=CARTESIAN_POINT ( 'NONE',  ( -10.81189881249999729, 1.324075727343319199E-15, -98.28125000204839523 ) ) ;
#40750=CARTESIAN_POINT ( 'NONE',  ( -10.81189881249999729, 1.324075727343319199E-15, -104.0937500020483810 ) ) ;
#40753=CARTESIAN_POINT ( 'NONE',  ( 9.975233911794434860, 6.725301395491736223, -179.8869040731969449 ) ) ;
#40754=CARTESIAN_POINT ( 'NONE',  ( -5.405949406249996869, 9.363379034771805109, -194.5312500020484094 ) ) ;
#40756=CARTESIAN_POINT ( 'NONE',  ( 7.070501591499377789E-16, 11.54700538379251284, -174.5000000040967905 ) ) ;
#40758=CARTESIAN_POINT ( 'NONE',  ( 10.81189881249999907, 6.242252689847868297, -22.21875000204836681 ) ) ;
#40760=CARTESIAN_POINT ( 'NONE',  ( 10.81189881249999907, 6.242252689847868297, -130.2187500020483810 ) ) ;
#40762=CARTESIAN_POINT ( 'NONE',  ( 5.405949406249999534, 9.363379034771803333, -26.78125000204836681 ) ) ;
#40764=CARTESIAN_POINT ( 'NONE',  ( 9.999999999999479527, 5.773502691896553074, -102.3749999999999858 ) ) ;
#40765=CARTESIAN_POINT ( 'NONE',  ( 9.999999999999996447, -5.773502691896262640, -53.12499999999997868 ) ) ;
#40766=CARTESIAN_POINT ( 'NONE',  ( 5.405949406249999534, 9.363379034771803333, -127.2812500020483810 ) ) ;
#40769=CARTESIAN_POINT ( 'NONE',  ( -10.00000000000000000, -5.773502691896251982, -99.00000000409679046 ) ) ;
#40770=CARTESIAN_POINT ( 'NONE',  ( 4.999999999999992006, -8.660254037844389075, -151.1250000040967905 ) ) ;
#40772=CARTESIAN_POINT ( 'NONE',  ( 5.405949406249992428, -9.363379034771808662, -55.59375000204835970 ) ) ;
#40775=CARTESIAN_POINT ( 'NONE',  ( 5.000000000000000000, 8.660254037844385522, -11.12500000409674605 ) ) ;
#40778=FACE_OUTER_BOUND ( 'NONE', #10788, .T. ) ;
#40779=CARTESIAN_POINT ( 'NONE',  ( -2.121150477449813534E-15, -11.54700538379251284, -31.25000000409675494 ) ) ;
#40781=EDGE_CURVE ( 'NONE', #7470, #40028, #21476, .T. ) ;
#40784=ORIENTED_EDGE ( 'NONE', *, *, #19372, .F. ) ;
#40786=VERTEX_POINT ( 'NONE', #17419 ) ;
#40791=CARTESIAN_POINT ( 'NONE',  ( 5.405949406249999534, 9.363379034771803333, -193.2812500020484094 ) ) ;
#40797=CARTESIAN_POINT ( 'NONE',  ( 5.405949406249999534, 9.363379034771803333, -119.5937500020483810 ) ) ;
#40798=CARTESIAN_POINT ( 'NONE',  ( -5.000000000000003553, -8.660254037844383745, -197.8750000040967905 ) ) ;
#40799=CARTESIAN_POINT ( 'NONE',  ( -10.81189881249999907, -6.242252689847864744, -128.1562500020483810 ) ) ;
#40801=CARTESIAN_POINT ( 'NONE',  ( -5.405949406250003975, -9.363379034771801557, -132.3437500020484094 ) ) ;
#40804=CARTESIAN_POINT ( 'NONE',  ( -10.00000000000000000, -5.773502691896251982, -145.1250000000000284 ) ) ;
#40805=CARTESIAN_POINT ( 'NONE',  ( -9.999999999999998224, 5.773502691896259087, -22.37499999999997868 ) ) ;
#40809=CARTESIAN_POINT ( 'NONE',  ( -9.999999999999742428, -5.773502691896402084, -159.0000000040967905 ) ) ;
#40811=CARTESIAN_POINT ( 'NONE',  ( -2.293366432827344421E-15, -12.48450537969573659, -48.21875000204836681 ) ) ;
#40812=CARTESIAN_POINT ( 'NONE',  ( -2.121150477449813534E-15, -11.54700538379251284, -163.2500000040968189 ) ) ;
#40813=CARTESIAN_POINT ( 'NONE',  ( -10.81189881249999729, 1.324075727343319199E-15, -155.0937500020483810 ) ) ;
#40817=CARTESIAN_POINT ( 'NONE',  ( -2.121150477449813534E-15, -11.54700538379251284, -83.37499999999997158 ) ) ;
#40820=CARTESIAN_POINT ( 'NONE',  ( 10.81189881249999729, 6.242252689847867408, -106.4062500020483952 ) ) ;
#40821=CARTESIAN_POINT ( 'NONE',  ( 4.999999999999992006, -8.660254037844389075, -124.1250000040967905 ) ) ;
#40824=CARTESIAN_POINT ( 'NONE',  ( -5.405949406250003975, -9.363379034771801557, -47.03125000204838813 ) ) ;
#40829=EDGE_LOOP ( 'NONE', ( #12837, #22974, #21934, #35086 ) ) ;
#40830=( BOUNDED_CURVE ( )  B_SPLINE_CURVE ( 2, ( #3282, #16409, #30037, #13387, #26579, #39729, #13598 ),
 .UNSPECIFIED., .F., .F. ) 
 B_SPLINE_CURVE_WITH_KNOTS ( ( 3, 2, 2, 3 ),
 ( 0.3805970149253732338, 0.3818407960199006190, 0.3830845771144278933, 0.3843283582089552786 ),
 .UNSPECIFIED. ) 
 CURVE ( )  GEOMETRIC_REPRESENTATION_ITEM ( )  RATIONAL_B_SPLINE_CURVE ( ( 0.9999999999999880096, 0.8660254037844506980, 1.000000000000000000, 0.8660254037844387076, 1.000000000000000000, 0.8660254037844327124, 1.000000000000005995 ) ) 
 REPRESENTATION_ITEM ( '' )  );
#40836=ORIENTED_EDGE ( 'NONE', *, *, #1914, .T. ) ;
#40845=CARTESIAN_POINT ( 'NONE',  ( -9.999999999999998224, 1.224646799147353059E-15, -149.7500000000000000 ) ) ;
#40846=CARTESIAN_POINT ( 'NONE',  ( 10.81189881249999551, -6.242252689847874514, -142.4687500020483810 ) ) ;
#40847=CARTESIAN_POINT ( 'NONE',  ( 5.405949406249992428, -9.363379034771808662, -150.2812500020483810 ) ) ;
#40848=CARTESIAN_POINT ( 'NONE',  ( -10.81189881249999729, 1.324075727343319199E-15, -153.5937500020483810 ) ) ;
#40850=CARTESIAN_POINT ( 'NONE',  ( -9.999999999999998224, 1.224646799147353059E-15, -102.1250000040967905 ) ) ;
#40851=CARTESIAN_POINT ( 'NONE',  ( -9.999999999999998224, 5.773502691896259087, -181.3750000000000000 ) ) ;
#40853=CARTESIAN_POINT ( 'NONE',  ( -9.999999999999998224, 0.000000000000000000, -99.99999999999998579 ) ) ;
#40855=CARTESIAN_POINT ( 'NONE',  ( 10.81189881249999907, 6.242252689847868297, -179.7187500020484094 ) ) ;
#40859=CARTESIAN_POINT ( 'NONE',  ( 10.81189881249999551, -6.242252689847874514, -46.65625000204836681 ) ) ;
#40861=CARTESIAN_POINT ( 'NONE',  ( 4.999999999999992006, -8.660254037844389075, -105.7499999999999858 ) ) ;
#40863=CARTESIAN_POINT ( 'NONE',  ( 5.405949406249992428, -9.363379034771808662, -126.2812500020483668 ) ) ;
#40864=CARTESIAN_POINT ( 'NONE',  ( -4.999999999999996447, 8.660254037844387298, -144.3750000040967905 ) ) ;
#40869=CARTESIAN_POINT ( 'NONE',  ( -5.405949406250003975, -9.363379034771801557, -172.8437500020484094 ) ) ;
#40873=CARTESIAN_POINT ( 'NONE',  ( -10.81189881249999729, 1.324075727343319199E-15, -66.78125000204838102 ) ) ;
#40875=( BOUNDED_CURVE ( )  B_SPLINE_CURVE ( 2, ( #23357, #274, #3078, #32443, #36088, #39315, #6946 ),
 .UNSPECIFIED., .F., .F. ) 
 B_SPLINE_CURVE_WITH_KNOTS ( ( 3, 2, 2, 3 ),
 ( 0.4328358208955225273, 0.4340796019900499125, 0.4353233830845772978, 0.4365671641791046276 ),
 .UNSPECIFIED. ) 
 CURVE ( )  GEOMETRIC_REPRESENTATION_ITEM ( )  RATIONAL_B_SPLINE_CURVE ( ( 0.9999999999999820144, 0.8660254037844566932, 1.000000000000000000, 0.8660254037844387076, 1.000000000000000000, 0.8660254037844207220, 1.000000000000017986 ) ) 
 REPRESENTATION_ITEM ( '' )  );
#40876=CARTESIAN_POINT ( 'NONE',  ( 9.999999999999998224, 0.000000000000000000, -47.37500000409677625 ) ) ;
#40877=CARTESIAN_POINT ( 'NONE',  ( -10.81189881249999729, 6.242252689847871849, -2.218750002048353043 ) ) ;
#40880=CARTESIAN_POINT ( 'NONE',  ( -4.999999999999996447, 8.660254037844387298, -138.3750000040967905 ) ) ;
#40887=DIRECTION ( 'NONE',  ( -0.000000000000000000, -0.000000000000000000, -1.000000000000000000 ) ) ;
#40897=CARTESIAN_POINT ( 'NONE',  ( -9.999999999999998224, 5.773502691896259087, -32.87499999999995737 ) ) ;
#40900=CARTESIAN_POINT ( 'NONE',  ( 10.81189881249999907, 6.242252689847868297, -169.2187500020483810 ) ) ;
#40901=CARTESIAN_POINT ( 'NONE',  ( -10.81189881249999729, -6.242252689847864744, -178.9687500020484094 ) ) ;
#40904=CARTESIAN_POINT ( 'NONE',  ( 9.999999999999479527, 5.773502691896553074, -104.2500000040967478 ) ) ;
#40910=CARTESIAN_POINT ( 'NONE',  ( 7.644554776091147741E-16, 12.48450537969573659, -59.46875000204837391 ) ) ;
#40911=CARTESIAN_POINT ( 'NONE',  ( -10.81189881249999729, 6.242252689847871849, -65.40625000204838102 ) ) ;
#40913=CARTESIAN_POINT ( 'NONE',  ( -9.999999999999998224, 5.773502691896259087, -131.8749999999999716 ) ) ;
#40914=CARTESIAN_POINT ( 'NONE',  ( 10.81189881249999729, 6.242252689847867408, -152.9062500020483810 ) ) ;
#40915=CARTESIAN_POINT ( 'NONE',  ( -10.81189881249999729, 1.324075727343319199E-15, -167.2812500020484094 ) ) ;
#40917=CARTESIAN_POINT ( 'NONE',  ( 9.999999999999998224, 0.000000000000000000, -150.8750000040967905 ) ) ;
#40918=CARTESIAN_POINT ( 'NONE',  ( 5.405949406249992428, -9.363379034771808662, -102.0937500020483810 ) ) ;
#40920=CARTESIAN_POINT ( 'NONE',  ( -5.405949406249996869, 9.363379034771805109, -192.8437500020484094 ) ) ;
#40923=CARTESIAN_POINT ( 'NONE',  ( 10.81189881249999729, 0.000000000000000000, -94.53125000204838102 ) ) ;
#40925=CARTESIAN_POINT ( 'NONE',  ( -5.000000000000003553, -8.660254037844383745, -74.87500000409677625 ) ) ;
#40926=CARTESIAN_POINT ( 'NONE',  ( 10.81189881249999907, 6.242252689847868297, -22.21875000204836681 ) ) ;
#40930=CARTESIAN_POINT ( 'NONE',  ( 10.81189881249999729, 0.000000000000000000, -31.53125000204837391 ) ) ;
#40933=CARTESIAN_POINT ( 'NONE',  ( -5.000000000000003553, -8.660254037844383745, -4.375000004096768258 ) ) ;
#40940=ORIENTED_EDGE ( 'NONE', *, *, #18399, .F. ) ;
#40948=CARTESIAN_POINT ( 'NONE',  ( 6.372319074206731493, 8.485273278836908517, -99.99999999999994316 ) ) ;
#40951=CARTESIAN_POINT ( 'NONE',  ( 5.405949406249992428, -9.363379034771808662, -160.7812500020484094 ) ) ;
#40955=CARTESIAN_POINT ( 'NONE',  ( 10.81189881249999551, -6.242252689847874514, -88.46875000204836681 ) ) ;
#40957=CARTESIAN_POINT ( 'NONE',  ( -5.405949406250003975, -9.363379034771801557, -196.8437500020484094 ) ) ;
#40958=CARTESIAN_POINT ( 'NONE',  ( 5.405949406249999534, 9.363379034771803333, -95.78125000204838102 ) ) ;
#40962=CARTESIAN_POINT ( 'NONE',  ( 5.405949406249999534, 9.363379034771803333, -170.7812500020484094 ) ) ;
#40963=CARTESIAN_POINT ( 'NONE',  ( -2.293366432827344421E-15, -12.48450537969573659, -189.4062500020484094 ) ) ;
#40965=CARTESIAN_POINT ( 'NONE',  ( -10.00000000000000000, -5.773502691896251982, -172.5000000040967905 ) ) ;
#40967=CARTESIAN_POINT ( 'NONE',  ( 10.81189881249999551, -6.242252689847874514, -25.46875000204837391 ) ) ;
#40968=CARTESIAN_POINT ( 'NONE',  ( -9.999999999999998224, 1.224646799147353059E-15, -125.7499999999999716 ) ) ;
#40969=CARTESIAN_POINT ( 'NONE',  ( -10.81189881249999729, 1.324075727343319199E-15, -119.0937500020483810 ) ) ;
#40971=CARTESIAN_POINT ( 'NONE',  ( -10.81189881249999907, -6.242252689847864744, -30.65625000204835970 ) ) ;
#40974=CARTESIAN_POINT ( 'NONE',  ( 4.999999999999992006, -8.660254037844389075, -53.24999999999996447 ) ) ;
#40975=CARTESIAN_POINT ( 'NONE',  ( -10.81189881249999729, 1.324075727343319199E-15, -128.2812500020483810 ) ) ;
#40977=ORIENTED_EDGE ( 'NONE', *, *, #303, .T. ) ;
#40978=AXIS2_PLACEMENT_3D ( 'NONE', #39033, #22637, #10095 ) ;
#40979=CARTESIAN_POINT ( 'NONE',  ( 10.00000000000000000, 5.773502691896255534, -96.75000000409679046 ) ) ;
#40980=DIRECTION ( 'NONE',  ( -0.000000000000000000, -0.000000000000000000, -1.000000000000000000 ) ) ;
#40982=CARTESIAN_POINT ( 'NONE',  ( -10.81189881249999729, 6.242252689847871849, -59.21875000204837391 ) ) ;
#40989=CARTESIAN_POINT ( 'NONE',  ( 9.999999999999998224, 0.000000000000000000, -30.87500000409676559 ) ) ;
#40993=VERTEX_POINT ( 'NONE', #18068 ) ;
#40998=CARTESIAN_POINT ( 'NONE',  ( 9.999999999999998224, 0.000000000000000000, -177.5000000000000000 ) ) ;
#41001=CARTESIAN_POINT ( 'NONE',  ( 10.81189881249999551, -6.242252689847874514, -190.6562500020484094 ) ) ;
#41003=CARTESIAN_POINT ( 'NONE',  ( 9.999999999999742428, 5.773502691896404748, -129.3750000000000000 ) ) ;
#41007=CARTESIAN_POINT ( 'NONE',  ( 10.81189881249999729, 0.000000000000000000, -112.3437500020483810 ) ) ;
#41008=CARTESIAN_POINT ( 'NONE',  ( -10.81189881249999907, -6.242252689847864744, -123.6562500020484094 ) ) ;
#41010=CARTESIAN_POINT ( 'NONE',  ( -5.405949406249996869, 9.363379034771805109, -132.8437500020484094 ) ) ;
#41011=CARTESIAN_POINT ( 'NONE',  ( -9.999999999999998224, 1.224646799147353059E-15, -164.7500000000000000 ) ) ;
#41012=CYLINDRICAL_SURFACE ( 'NONE', #4076, 9.999999999999998224 ) ;
#41013=CARTESIAN_POINT ( 'NONE',  ( 4.999999999999992006, -8.660254037844389075, -147.7500000000000000 ) ) ;
#41014=CARTESIAN_POINT ( 'NONE',  ( 10.00000000000000000, 5.773502691896255534, -24.37499999999997868 ) ) ;
#41018=CARTESIAN_POINT ( 'NONE',  ( -9.999999999999998224, 1.224646799147353059E-15, -145.2500000000000000 ) ) ;
#41020=CARTESIAN_POINT ( 'NONE',  ( 10.81189881249999907, 6.242252689847868297, -47.71875000204835970 ) ) ;
#41022=CARTESIAN_POINT ( 'NONE',  ( 5.405949406249999534, 9.363379034771803333, -155.5937500020483810 ) ) ;
#41025=VECTOR ( 'NONE', #5908, 1000.000000000000000 ) ;
#41026=CARTESIAN_POINT ( 'NONE',  ( -9.999999999999998224, 5.773502691896259087, -73.37499999999997158 ) ) ;
#41029=CARTESIAN_POINT ( 'NONE',  ( -2.293366432827344421E-15, -12.48450537969573659, -103.9062500020483810 ) ) ;
#41030=CARTESIAN_POINT ( 'NONE',  ( 4.999999999999992006, -8.660254037844389075, -122.6250000040967905 ) ) ;
#41032=CARTESIAN_POINT ( 'NONE',  ( -5.405949406249996869, 9.363379034771805109, -81.84375000204838102 ) ) ;
#41034=CARTESIAN_POINT ( 'NONE',  ( -10.00000000000076916, 5.773502691895813221, -130.3750000000000000 ) ) ;
#41035=CARTESIAN_POINT ( 'NONE',  ( -10.81189881249999907, -6.242252689847864744, -44.15625000204837391 ) ) ;
#41036=CARTESIAN_POINT ( 'NONE',  ( -9.999999999999998224, 1.224646799147353059E-15, -137.7499999999999716 ) ) ;
#41044=VERTEX_POINT ( 'NONE', #18281 ) ;
#41045=CARTESIAN_POINT ( 'NONE',  ( -9.999999999999998224, 1.224646799147353059E-15, -104.7499999999999858 ) ) ;
#41049=CARTESIAN_POINT ( 'NONE',  ( -9.999999999999998224, 1.224646799147353059E-15, -177.1250000040968189 ) ) ;
#41054=CARTESIAN_POINT ( 'NONE',  ( 5.405949406249992428, -9.363379034771808662, -142.5937500020483810 ) ) ;
#41055=CARTESIAN_POINT ( 'NONE',  ( -10.81189881249999907, -6.242252689847864744, -149.1562500020483810 ) ) ;
#41056=CARTESIAN_POINT ( 'NONE',  ( 5.405949406249992428, -9.363379034771808662, -156.0937500020483810 ) ) ;
#41058=DIRECTION ( 'NONE',  ( -1.000000000000000000, 0.000000000000000000, 0.000000000000000000 ) ) ;
#41059=CARTESIAN_POINT ( 'NONE',  ( -4.999999999999996447, 8.660254037844387298, -172.5000000000000284 ) ) ;
#41062=CARTESIAN_POINT ( 'NONE',  ( -5.000000000000003553, -8.660254037844383745, -99.99999999999998579 ) ) ;
#41063=CARTESIAN_POINT ( 'NONE',  ( 5.405949406249992428, -9.363379034771808662, -178.5937500020484094 ) ) ;
#41067=CARTESIAN_POINT ( 'NONE',  ( -2.293366432827344421E-15, -12.48450537969573659, -40.90625000204836681 ) ) ;
#41069=CARTESIAN_POINT ( 'NONE',  ( 5.000000000000000000, 8.660254037844385522, -102.2500000000000000 ) ) ;
#41071=CARTESIAN_POINT ( 'NONE',  ( 7.644554776091147741E-16, 12.48450537969573659, -127.1562500020483810 ) ) ;
#41072=CARTESIAN_POINT ( 'NONE',  ( -4.999999999999996447, 8.660254037844387298, -151.8750000040967905 ) ) ;
#41076=CARTESIAN_POINT ( 'NONE',  ( -2.293366432827344421E-15, -12.48450537969573659, -175.7187500020483810 ) ) ;
#41081=CARTESIAN_POINT ( 'NONE',  ( 10.81189881249999729, 0.000000000000000000, -70.53125000204838102 ) ) ;
#41084=CARTESIAN_POINT ( 'NONE',  ( -10.00000000000000000, -5.773502691896251982, -45.00000000409676204 ) ) ;
#41085=CARTESIAN_POINT ( 'NONE',  ( -5.405949406250003975, -9.363379034771801557, -4.843750002048369474 ) ) ;
#41095=EDGE_LOOP ( 'NONE', ( #40252, #21105, #23458, #20547 ) ) ;
#41106=CARTESIAN_POINT ( 'NONE',  ( 10.00000000000000000, 5.773502691896255534, -39.37499999999996447 ) ) ;
#41108=CARTESIAN_POINT ( 'NONE',  ( 5.405949406249992428, -9.363379034771808662, -169.5937500020484094 ) ) ;
#41109=CARTESIAN_POINT ( 'NONE',  ( 7.644554776091147741E-16, 12.48450537969573659, -179.4687500020484094 ) ) ;
#41112=CARTESIAN_POINT ( 'NONE',  ( 9.999999999999998224, 0.000000000000000000, -140.0000000000000000 ) ) ;
#41114=CARTESIAN_POINT ( 'NONE',  ( 4.999999999999992006, -8.660254037844389075, -197.2500000000000000 ) ) ;
#41120=CARTESIAN_POINT ( 'NONE',  ( -5.405949406250003975, -9.363379034771801557, -61.84375000204836681 ) ) ;
#41121=CARTESIAN_POINT ( 'NONE',  ( -5.405949406249996869, 9.363379034771805109, -67.03125000204838102 ) ) ;
#41123=CARTESIAN_POINT ( 'NONE',  ( 7.070501591499377789E-16, 11.54700538379251284, -127.6249999999999858 ) ) ;
#41124=( BOUNDED_CURVE ( )  B_SPLINE_CURVE ( 2, ( #34233, #578, #4226, #23877, #4649, #27104, #787 ),
 .UNSPECIFIED., .F., .F. ) 
 B_SPLINE_CURVE_WITH_KNOTS ( ( 3, 2, 2, 3 ),
 ( 0.4738805970149255198, 0.4751243781094529051, 0.4763681592039803459, 0.4776119402985076756 ),
 .UNSPECIFIED. ) 
 CURVE ( )  GEOMETRIC_REPRESENTATION_ITEM ( )  RATIONAL_B_SPLINE_CURVE ( ( 0.9999999999999820144, 0.8660254037844566932, 1.000000000000000000, 0.8660254037844387076, 1.000000000000000000, 0.8660254037844148378, 1.000000000000023981 ) ) 
 REPRESENTATION_ITEM ( '' )  );
#41125=CARTESIAN_POINT ( 'NONE',  ( 7.644554776091147741E-16, 12.48450537969573659, -148.1562500020484094 ) ) ;
#41126=CARTESIAN_POINT ( 'NONE',  ( -2.293366432827344421E-15, -12.48450537969573659, -165.4062500020483810 ) ) ;
#41127=DIRECTION ( 'NONE',  ( -0.000000000000000000, -0.000000000000000000, -1.000000000000000000 ) ) ;
#41129=CARTESIAN_POINT ( 'NONE',  ( -10.81189881249999907, -6.242252689847864744, -96.46875000204838102 ) ) ;
#41132=CARTESIAN_POINT ( 'NONE',  ( 5.405949406249999534, 9.363379034771803333, -196.0937500020484094 ) ) ;
#41134=CARTESIAN_POINT ( 'NONE',  ( 10.81189881249999551, -6.242252689847874514, -94.65625000204838102 ) ) ;
#41136=( BOUNDED_CURVE ( )  B_SPLINE_CURVE ( 2, ( #7138, #36698, #22913, #20502, #29597, #10154, #32839 ),
 .UNSPECIFIED., .F., .F. ) 
 B_SPLINE_CURVE_WITH_KNOTS ( ( 3, 2, 2, 3 ),
 ( 0.4850746268656717652, 0.4863184079601990950, 0.4875621890547264248, 0.4888059701492538101 ),
 .UNSPECIFIED. ) 
 CURVE ( )  GEOMETRIC_REPRESENTATION_ITEM ( )  RATIONAL_B_SPLINE_CURVE ( ( 0.9999999999999880096, 0.8660254037844506980, 1.000000000000000000, 0.8660254037844387076, 1.000000000000000000, 0.8660254037844327124, 1.000000000000005995 ) ) 
 REPRESENTATION_ITEM ( '' )  );
#41137=CARTESIAN_POINT ( 'NONE',  ( 5.000000000000000000, 8.660254037844385522, -69.62500000409677625 ) ) ;
#41139=CARTESIAN_POINT ( 'NONE',  ( 7.644554776091147741E-16, 12.48450537969573659, -27.96875000204837747 ) ) ;
#41142=CARTESIAN_POINT ( 'NONE',  ( 10.81189881249999907, 6.242252689847868297, -17.90625000204837391 ) ) ;
#41148=CARTESIAN_POINT ( 'NONE',  ( -10.00000000000025580, 5.773502691896109873, -151.7500000040967336 ) ) ;
#41160=CARTESIAN_POINT ( 'NONE',  ( 0.000000000000000000, 0.000000000000000000, -99.99999999999998579 ) ) ;
#41161=AXIS2_PLACEMENT_3D ( 'NONE', #25856, #2981, #28891 ) ;
#41162=CARTESIAN_POINT ( 'NONE',  ( 9.999999999999998224, 0.000000000000000000, -114.4999999999999858 ) ) ;
#41164=CARTESIAN_POINT ( 'NONE',  ( 5.405949406249999534, 9.363379034771803333, -166.2812500020484094 ) ) ;
#41167=CARTESIAN_POINT ( 'NONE',  ( -10.81189881249999907, -6.242252689847864744, -82.96875000204836681 ) ) ;
#41169=CARTESIAN_POINT ( 'NONE',  ( 7.644554776091147741E-16, 12.48450537969573659, -191.4687500020484094 ) ) ;
#41170=CARTESIAN_POINT ( 'NONE',  ( -2.293366432827344421E-15, -12.48450537969573659, -90.40625000204838102 ) ) ;
#41174=CARTESIAN_POINT ( 'NONE',  ( 10.81189881249999729, 0.000000000000000000, -177.0312500020483810 ) ) ;
#41175=CARTESIAN_POINT ( 'NONE',  ( -10.81189881249999729, 1.324075727343319199E-15, -191.2812500020484094 ) ) ;
#41177=CARTESIAN_POINT ( 'NONE',  ( 9.999999999999998224, 0.000000000000000000, -161.3750000040967905 ) ) ;
#41179=CARTESIAN_POINT ( 'NONE',  ( -10.81189881249999729, 1.324075727343319199E-15, -12.59375000204834905 ) ) ;
#41181=CARTESIAN_POINT ( 'NONE',  ( 10.81189881249999729, 0.000000000000000000, -125.8437500020483952 ) ) ;
#41183=CARTESIAN_POINT ( 'NONE',  ( -2.293366432827344421E-15, -12.48450537969573659, -21.40625000204837747 ) ) ;
#41186=CARTESIAN_POINT ( 'NONE',  ( 5.000000000000000000, 8.660254037844385522, -49.74999999999998579 ) ) ;
#41187=CARTESIAN_POINT ( 'NONE',  ( 10.81189881249999551, -6.242252689847874514, -120.1562500020483810 ) ) ;
#41189=EDGE_LOOP ( 'NONE', ( #40836, #19774, #7742, #32741 ) ) ;
#41190=CARTESIAN_POINT ( 'NONE',  ( -2.121150477449813534E-15, -11.54700538379251284, -95.75000000409677625 ) ) ;
#41193=CARTESIAN_POINT ( 'NONE',  ( 10.81189881249999551, -6.242252689847874514, -52.46875000204837391 ) ) ;
#41196=EDGE_CURVE ( 'NONE', #12994, #40615, #25645, .T. ) ;
#41197=EDGE_CURVE ( 'NONE', #26528, #16951, #18449, .T. ) ;
#41200=AXIS2_PLACEMENT_3D ( 'NONE', #13025, #29242, #3764 ) ;
#41202=CARTESIAN_POINT ( 'NONE',  ( 5.000000000000000000, 8.660254037844385522, -27.62500000409676204 ) ) ;
#41207=( BOUNDED_CURVE ( )  B_SPLINE_CURVE ( 2, ( #25093, #38239, #463, #38873, #6290, #42515, #29168 ),
 .UNSPECIFIED., .F., .F. ) 
 B_SPLINE_CURVE_WITH_KNOTS ( ( 3, 2, 2, 3 ),
 ( 0.2574626865671643117, 0.2587064676616916414, 0.2599502487562190267, 0.2611940298507463565 ),
 .UNSPECIFIED. ) 
 CURVE ( )  GEOMETRIC_REPRESENTATION_ITEM ( )  RATIONAL_B_SPLINE_CURVE ( ( 0.9999999999999880096, 0.8660254037844506980, 1.000000000000000000, 0.8660254037844387076, 1.000000000000000000, 0.8660254037844267172, 1.000000000000011990 ) ) 
 REPRESENTATION_ITEM ( '' )  );
#41216=CARTESIAN_POINT ( 'NONE',  ( 0.000000000000000000, 0.000000000000000000, -99.99999999999998579 ) ) ;
#41218=CARTESIAN_POINT ( 'NONE',  ( -10.81189881249999729, 1.324075727343319199E-15, -186.7812500020484094 ) ) ;
#41225=CARTESIAN_POINT ( 'NONE',  ( 5.405949406249992428, -9.363379034771808662, -111.0937500020483810 ) ) ;
#41227=CARTESIAN_POINT ( 'NONE',  ( -10.81189881249999729, 6.242252689847871849, -113.4062500020483810 ) ) ;
#41229=CARTESIAN_POINT ( 'NONE',  ( -5.405949406250003975, -9.363379034771801557, -129.3437500020484094 ) ) ;
#41231=CARTESIAN_POINT ( 'NONE',  ( -9.999999999999998224, 1.224646799147353059E-15, -178.6250000040968189 ) ) ;
#41232=CARTESIAN_POINT ( 'NONE',  ( 9.999999999999998224, 0.000000000000000000, -150.5000000000000000 ) ) ;
#41233=CARTESIAN_POINT ( 'NONE',  ( -5.000000000000003553, -8.660254037844383745, -9.999999999999953815 ) ) ;
#41236=CARTESIAN_POINT ( 'NONE',  ( 9.999999999999996447, -5.773502691896262640, -187.0000000040968189 ) ) ;
#41238=CARTESIAN_POINT ( 'NONE',  ( 10.81189881249999729, 0.000000000000000000, -34.34375000204836681 ) ) ;
#41239=CARTESIAN_POINT ( 'NONE',  ( -9.999999999999998224, 1.224646799147353059E-15, -142.6250000040967905 ) ) ;
#41240=CARTESIAN_POINT ( 'NONE',  ( -10.81189881249999907, -6.242252689847864744, -147.4687500020484094 ) ) ;
#41242=CARTESIAN_POINT ( 'NONE',  ( -9.999999999999998224, 0.000000000000000000, -99.99999999999998579 ) ) ;
#41243=CARTESIAN_POINT ( 'NONE',  ( 7.070501591499377789E-16, 11.54700538379251284, -72.12499999999997158 ) ) ;
#41244=CARTESIAN_POINT ( 'NONE',  ( 7.644554776091147741E-16, 12.48450537969573659, -142.1562500020483810 ) ) ;
#41247=CARTESIAN_POINT ( 'NONE',  ( 10.81189881249999729, 6.242252689847867408, -101.9062500020483952 ) ) ;
#41248=CARTESIAN_POINT ( 'NONE',  ( -5.000000000000003553, -8.660254037844383745, -122.8750000040967905 ) ) ;
#41250=CARTESIAN_POINT ( 'NONE',  ( -10.81189881249999907, -6.242252689847864744, -76.96875000204836681 ) ) ;
#41253=CARTESIAN_POINT ( 'NONE',  ( 5.405949406249992428, -9.363379034771808662, -46.78125000204838813 ) ) ;
#41254=( BOUNDED_CURVE ( )  B_SPLINE_CURVE ( 2, ( #18828, #18396, #32222, #25108, #22492, #2236, #25742 ),
 .UNSPECIFIED., .F., .F. ) 
 B_SPLINE_CURVE_WITH_KNOTS ( ( 3, 2, 2, 3 ),
 ( 0.2313432835820896372, 0.2325870646766169947, 0.2338308457711443245, 0.2350746268656717097 ),
 .UNSPECIFIED. ) 
 CURVE ( )  GEOMETRIC_REPRESENTATION_ITEM ( )  RATIONAL_B_SPLINE_CURVE ( ( 0.9999999999999910072, 0.8660254037844477004, 1.000000000000000000, 0.8660254037844387076, 1.000000000000000000, 0.8660254037844327124, 1.000000000000005995 ) ) 
 REPRESENTATION_ITEM ( '' )  );
#41255=EDGE_CURVE ( 'NONE', #24567, #17213, #25895, .T. ) ;
#41261=VECTOR ( 'NONE', #33086, 1000.000000000000000 ) ;
#41263=CARTESIAN_POINT ( 'NONE',  ( 4.999999999999992006, -8.660254037844389075, -120.7500000000000000 ) ) ;
#41277=CARTESIAN_POINT ( 'NONE',  ( 5.405949406249992428, -9.363379034771808662, -132.0937500020483810 ) ) ;
#41278=CARTESIAN_POINT ( 'NONE',  ( -5.405949406249996869, 9.363379034771805109, -139.0312500020484094 ) ) ;
#41279=CARTESIAN_POINT ( 'NONE',  ( 5.405949406249992428, -9.363379034771808662, -157.5937500020483810 ) ) ;
#41282=CARTESIAN_POINT ( 'NONE',  ( -10.00000000000000000, -5.773502691896251982, -173.6249999999999716 ) ) ;
#41286=CARTESIAN_POINT ( 'NONE',  ( 5.000000000000000000, 8.660254037844385522, -133.7499999999999716 ) ) ;
#41287=CARTESIAN_POINT ( 'NONE',  ( -5.405949406249996869, 9.363379034771805109, -167.3437500020484094 ) ) ;
#41291=CARTESIAN_POINT ( 'NONE',  ( -5.405949406250003975, -9.363379034771801557, -48.53125000204838813 ) ) ;
#41293=CARTESIAN_POINT ( 'NONE',  ( 7.070501591499377789E-16, 11.54700538379251284, -97.62499999999997158 ) ) ;
#41295=CARTESIAN_POINT ( 'NONE',  ( 10.81189881249999551, -6.242252689847874514, -124.6562500020483952 ) ) ;
#41296=CARTESIAN_POINT ( 'NONE',  ( 9.999999999999996447, -5.773502691896262640, -151.0000000040967905 ) ) ;
#41297=CARTESIAN_POINT ( 'NONE',  ( -9.999999999999872102, -5.773502691896326589, -167.6250000000000000 ) ) ;
#41301=CARTESIAN_POINT ( 'NONE',  ( -10.81189881249999729, 6.242252689847871849, -176.2187500020483810 ) ) ;
#41303=CARTESIAN_POINT ( 'NONE',  ( 4.999999999999992006, -8.660254037844389075, -165.7500000000000000 ) ) ;
#41305=CARTESIAN_POINT ( 'NONE',  ( 5.405949406249992428, -9.363379034771808662, -67.78125000204838102 ) ) ;
#41306=CARTESIAN_POINT ( 'NONE',  ( 4.999999999999992006, -8.660254037844389075, -44.62500000409677625 ) ) ;
#41307=CARTESIAN_POINT ( 'NONE',  ( -10.81189881249999729, 6.242252689847871849, -3.718750002048354819 ) ) ;
#41310=CARTESIAN_POINT ( 'NONE',  ( 9.999999999999998224, 0.000000000000000000, -105.8750000040967763 ) ) ;
#41312=VERTEX_POINT ( 'NONE', #35136 ) ;
#41321=EDGE_LOOP ( 'NONE', ( #6255, #16840, #22367, #8751 ) ) ;
#41328=CARTESIAN_POINT ( 'NONE',  ( -10.00000000000076916, 5.773502691895813221, -112.3749999999999858 ) ) ;
#41329=CARTESIAN_POINT ( 'NONE',  ( -2.121150477449813534E-15, -11.54700538379251284, -38.37499999999996447 ) ) ;
#41332=CARTESIAN_POINT ( 'NONE',  ( -10.81189881249999729, 6.242252689847871849, -159.7187500020483526 ) ) ;
#41337=CARTESIAN_POINT ( 'NONE',  ( -10.00000000000000000, -5.773502691896251982, -196.1250000000000568 ) ) ;
#41339=CARTESIAN_POINT ( 'NONE',  ( -9.999999999999998224, 0.000000000000000000, -99.99999999999998579 ) ) ;
#41342=( BOUNDED_CURVE ( )  B_SPLINE_CURVE ( 2, ( #21313, #8594, #15037, #20510, #10368, #41148, #37939 ),
 .UNSPECIFIED., .F., .F. ) 
 B_SPLINE_CURVE_WITH_KNOTS ( ( 3, 2, 2, 3 ),
 ( 0.2313432835820896372, 0.2325870646766169947, 0.2338308457711443245, 0.2350746268656717097 ),
 .UNSPECIFIED. ) 
 CURVE ( )  GEOMETRIC_REPRESENTATION_ITEM ( )  RATIONAL_B_SPLINE_CURVE ( ( 0.9999999999999910072, 0.8660254037844477004, 1.000000000000000000, 0.8660254037844387076, 1.000000000000000000, 0.8660254037844327124, 1.000000000000005995 ) ) 
 REPRESENTATION_ITEM ( '' )  );
#41343=CARTESIAN_POINT ( 'NONE',  ( 5.405949406249992428, -9.363379034771808662, -67.78125000204838102 ) ) ;
#41345=CARTESIAN_POINT ( 'NONE',  ( 4.999999999999992006, -8.660254037844389075, -125.2500000000000000 ) ) ;
#41346=CARTESIAN_POINT ( 'NONE',  ( -10.81189881249999729, -6.242252689847864744, -150.6562500020484094 ) ) ;
#41347=CARTESIAN_POINT ( 'NONE',  ( -2.293366432827344421E-15, -12.48450537969573659, -163.9062500020483810 ) ) ;
#41348=CYLINDRICAL_SURFACE ( 'NONE', #28921, 9.999999999999998224 ) ;
#41350=CARTESIAN_POINT ( 'NONE',  ( 5.405949406249992428, -9.363379034771808662, -99.09375000204838102 ) ) ;
#41353=CARTESIAN_POINT ( 'NONE',  ( 10.81189881249999729, 0.000000000000000000, -197.8437500020484094 ) ) ;
#41355=CARTESIAN_POINT ( 'NONE',  ( 9.999999999999994671, -5.773502691896262640, -133.0000000040967905 ) ) ;
#41357=CARTESIAN_POINT ( 'NONE',  ( -2.293366432827344421E-15, -12.48450537969573659, -88.90625000204838102 ) ) ;
#41359=CARTESIAN_POINT ( 'NONE',  ( -10.00000000000000000, -5.773502691896251982, -64.50000000409677625 ) ) ;
#41361=CARTESIAN_POINT ( 'NONE',  ( -10.81189881249999729, 1.324075727343319199E-15, -26.09375000204835970 ) ) ;
#41362=CARTESIAN_POINT ( 'NONE',  ( 7.070501591499376803E-16, 11.54700538379251284, -100.6250000000000000 ) ) ;
#41365=CARTESIAN_POINT ( 'NONE',  ( -5.405949406250003975, -9.363379034771801557, -23.03125000204836326 ) ) ;
#41374=ORIENTED_EDGE ( 'NONE', *, *, #24570, .T. ) ;
#41381=DIRECTION ( 'NONE',  ( -0.000000000000000000, -0.000000000000000000, -1.000000000000000000 ) ) ;
#41386=CARTESIAN_POINT ( 'NONE',  ( -10.81189881249999729, 1.324075727343319199E-15, -162.7812500020484094 ) ) ;
#41391=CARTESIAN_POINT ( 'NONE',  ( 10.81189881249999729, 0.000000000000000000, -86.84375000204836681 ) ) ;
#41393=CARTESIAN_POINT ( 'NONE',  ( -5.405949406249996869, 9.363379034771805109, -192.8437500020484094 ) ) ;
#41394=CARTESIAN_POINT ( 'NONE',  ( -10.81189881249999907, -6.242252689847864744, -90.65625000204836681 ) ) ;
#41399=CARTESIAN_POINT ( 'NONE',  ( -2.293366432827344421E-15, -12.48450537969573659, -174.4062500020484379 ) ) ;
#41400=CARTESIAN_POINT ( 'NONE',  ( 5.405949406249999534, 9.363379034771803333, -190.2812500020484094 ) ) ;
#41402=CARTESIAN_POINT ( 'NONE',  ( 9.999999999999996447, -5.773502691896262640, -161.5000000040968189 ) ) ;
#41404=CARTESIAN_POINT ( 'NONE',  ( -5.405949406250003975, -9.363379034771801557, -15.34375000204835082 ) ) ;
#41406=CARTESIAN_POINT ( 'NONE',  ( 10.81189881249999551, -6.242252689847874514, -125.9687500020483810 ) ) ;
#41408=CARTESIAN_POINT ( 'NONE',  ( 10.81189881249999551, -6.242252689847874514, -24.15625000204837747 ) ) ;
#41411=CARTESIAN_POINT ( 'NONE',  ( 9.999999999999996447, -5.773502691896262640, -54.62499999999997868 ) ) ;
#41412=CARTESIAN_POINT ( 'NONE',  ( -10.81189881249999729, 1.324075727343319199E-15, -117.7812500020483952 ) ) ;
#41414=ORIENTED_EDGE ( 'NONE', *, *, #30941, .T. ) ;
#41415=CARTESIAN_POINT ( 'NONE',  ( -5.000000000000003553, -8.660254037844383745, -91.37500000409677625 ) ) ;
#41416=CARTESIAN_POINT ( 'NONE',  ( 4.999999999999992006, -8.660254037844389075, -101.2499999999999858 ) ) ;
#41418=CARTESIAN_POINT ( 'NONE',  ( 7.644554776091147741E-16, 12.48450537969573659, -50.46875000204836681 ) ) ;
#41419=VERTEX_POINT ( 'NONE', #15671 ) ;
#41423=CARTESIAN_POINT ( 'NONE',  ( -10.00000000000000000, -5.773502691896251982, -18.00000000409676559 ) ) ;
#41424=VECTOR ( 'NONE', #20508, 1000.000000000000000 ) ;
#41430=EDGE_LOOP ( 'NONE', ( #24357, #12084, #36070, #583 ) ) ;
#41434=EDGE_LOOP ( 'NONE', ( #31757, #791, #34074, #29641 ) ) ;
#41438=CARTESIAN_POINT ( 'NONE',  ( 5.405949406249999534, 9.363379034771803333, -185.7812500020484094 ) ) ;
#41444=CARTESIAN_POINT ( 'NONE',  ( -5.405949406249996869, 9.363379034771805109, -111.8437500020483810 ) ) ;
#41446=CARTESIAN_POINT ( 'NONE',  ( -2.293366432827344421E-15, -12.48450537969573659, -118.9062500020483952 ) ) ;
#41448=CARTESIAN_POINT ( 'NONE',  ( -10.81189881249999729, 6.242252689847871849, -125.2187500020483810 ) ) ;
#41452=CARTESIAN_POINT ( 'NONE',  ( 5.000000000000000000, 8.660254037844385522, -148.7500000000000000 ) ) ;
#41453=CARTESIAN_POINT ( 'NONE',  ( 4.999999999999992006, -8.660254037844389075, -12.74999999999995559 ) ) ;
#41457=CARTESIAN_POINT ( 'NONE',  ( -9.999999999999998224, 5.773502691896259087, -186.2500000040967905 ) ) ;
#41459=CARTESIAN_POINT ( 'NONE',  ( 10.81189881249999551, -6.242252689847874514, -37.46875000204835970 ) ) ;
#41461=CARTESIAN_POINT ( 'NONE',  ( -5.405949406249996869, 9.363379034771805109, -143.3437500020483810 ) ) ;
#41464=CARTESIAN_POINT ( 'NONE',  ( 9.999999999999998224, 0.000000000000000000, -72.49999999999998579 ) ) ;
#41465=CARTESIAN_POINT ( 'NONE',  ( 7.644554776091147741E-16, 12.48450537969573659, -137.6562500020483810 ) ) ;
#41467=ORIENTED_EDGE ( 'NONE', *, *, #24143, .T. ) ;
#41468=CARTESIAN_POINT ( 'NONE',  ( -5.405949406249996869, 9.363379034771805109, -106.0312500020483810 ) ) ;
#41469=CARTESIAN_POINT ( 'NONE',  ( -9.999999999999998224, 1.224646799147353059E-15, -114.1250000040967763 ) ) ;
#41470=CARTESIAN_POINT ( 'NONE',  ( -2.121150477449813534E-15, -11.54700538379251284, -140.3750000000000000 ) ) ;
#41471=CARTESIAN_POINT ( 'NONE',  ( 10.81189881249999551, -6.242252689847874514, -70.46875000204839523 ) ) ;
#41472=AXIS2_PLACEMENT_3D ( 'NONE', #23087, #36248, #23518 ) ;
#41477=CARTESIAN_POINT ( 'NONE',  ( -10.81189881249999907, -6.242252689847864744, -47.15625000204837391 ) ) ;
#41496=CARTESIAN_POINT ( 'NONE',  ( 7.644554776091147741E-16, 12.48450537969573659, -134.4687500020483810 ) ) ;
#41497=CARTESIAN_POINT ( 'NONE',  ( 5.405949406249999534, 9.363379034771803333, -142.2812500020483810 ) ) ;
#41498=CARTESIAN_POINT ( 'NONE',  ( -2.293366432827344421E-15, -12.48450537969573659, -148.7187500020484094 ) ) ;
#41501=LINE ( 'NONE', #28996, #6148 ) ;
#41502=CARTESIAN_POINT ( 'NONE',  ( -4.999999999999996447, 8.660254037844387298, -168.0000000000000000 ) ) ;
#41505=CARTESIAN_POINT ( 'NONE',  ( -5.482716661060788255, 9.345839531454744886, -99.99999999999997158 ) ) ;
#41507=CARTESIAN_POINT ( 'NONE',  ( 7.070501591499376803E-16, 11.54700538379251284, -133.6250000000000000 ) ) ;
#41508=CARTESIAN_POINT ( 'NONE',  ( 10.81189881249999907, 6.242252689847868297, -170.7187500020483810 ) ) ;
#41513=CARTESIAN_POINT ( 'NONE',  ( 10.81189881249999551, -6.242252689847874514, -43.65625000204836681 ) ) ;
#41515=CARTESIAN_POINT ( 'NONE',  ( 4.999999999999992006, -8.660254037844389075, -102.7500000000000000 ) ) ;
#41516=AXIS2_PLACEMENT_3D ( 'NONE', #4213, #30766, #7666 ) ;
#41519=CARTESIAN_POINT ( 'NONE',  ( -10.81189881249999729, 1.324075727343319199E-15, -126.7812500020483668 ) ) ;
#41520=CARTESIAN_POINT ( 'NONE',  ( 9.999999999999998224, 0.000000000000000000, -141.8750000040967905 ) ) ;
#41524=CARTESIAN_POINT ( 'NONE',  ( 10.81189881249999551, -6.242252689847874514, -173.9687500020484094 ) ) ;
#41528=CARTESIAN_POINT ( 'NONE',  ( -5.405949406249996869, 9.363379034771805109, -68.53125000204838102 ) ) ;
#41529=CARTESIAN_POINT ( 'NONE',  ( -10.00000000000000000, -5.773502691896251982, -46.50000000409676204 ) ) ;
#41536=EDGE_LOOP ( 'NONE', ( #15261, #15046, #2915, #9104 ) ) ;
#41541=ORIENTED_EDGE ( 'NONE', *, *, #5126, .F. ) ;
#41549=ORIENTED_EDGE ( 'NONE', *, *, #21998, .T. ) ;
#41550=CARTESIAN_POINT ( 'NONE',  ( -9.999999999999998224, 1.224646799147353059E-15, -123.1250000040967905 ) ) ;
#41551=CARTESIAN_POINT ( 'NONE',  ( -10.00000000000000000, -5.773502691896251982, -34.12499999999996447 ) ) ;
#41554=CARTESIAN_POINT ( 'NONE',  ( -10.81189881249999907, -6.242252689847864744, -159.4687500020484094 ) ) ;
#41557=CARTESIAN_POINT ( 'NONE',  ( 7.070501591499377789E-16, 11.54700538379251284, -198.1250000000000000 ) ) ;
#41562=CARTESIAN_POINT ( 'NONE',  ( -10.81189881249999729, 6.242252689847871849, -71.40625000204839523 ) ) ;
#41564=CARTESIAN_POINT ( 'NONE',  ( -9.999999999999998224, 5.773502691896259087, -121.3750000000000000 ) ) ;
#41565=ORIENTED_EDGE ( 'NONE', *, *, #34023, .T. ) ;
#41566=CARTESIAN_POINT ( 'NONE',  ( -10.81189881249999729, 1.324075727343319199E-15, -153.7812500020484094 ) ) ;
#41567=CARTESIAN_POINT ( 'NONE',  ( -10.81189881249999729, 6.242252689847871849, -165.9062500020483810 ) ) ;
#41571=CARTESIAN_POINT ( 'NONE',  ( 5.405949406249999534, 9.363379034771803333, -98.59375000204838102 ) ) ;
#41572=ORIENTED_EDGE ( 'NONE', *, *, #21729, .T. ) ;
#41574=CARTESIAN_POINT ( 'NONE',  ( -5.405949406250003975, -9.363379034771801557, -196.8437500020484094 ) ) ;
#41576=CARTESIAN_POINT ( 'NONE',  ( 8.048493842490250572, -7.181085626304623659, -179.9999999999999716 ) ) ;
#41577=CARTESIAN_POINT ( 'NONE',  ( -9.999999999999479527, -5.773502691896549521, -124.1249999999999858 ) ) ;
#41578=CARTESIAN_POINT ( 'NONE',  ( -2.293366432827344421E-15, -12.48450537969573659, -94.90625000204838102 ) ) ;
#41580=CARTESIAN_POINT ( 'NONE',  ( 4.999999999999992006, -8.660254037844389075, -68.62500000409677625 ) ) ;
#41582=CARTESIAN_POINT ( 'NONE',  ( -5.405949406250003975, -9.363379034771801557, -25.84375000204835970 ) ) ;
#41583=ORIENTED_EDGE ( 'NONE', *, *, #27828, .F. ) ;
#41585=CARTESIAN_POINT ( 'NONE',  ( -5.405949406249996869, 9.363379034771805109, -19.03125000204835970 ) ) ;
#41587=CARTESIAN_POINT ( 'NONE',  ( 5.000000000000000000, 8.660254037844385522, -137.1250000040967620 ) ) ;
#41589=CARTESIAN_POINT ( 'NONE',  ( 4.999999999999992006, -8.660254037844389075, 0.3749999959032357388 ) ) ;
#41597=VERTEX_POINT ( 'NONE', #22868 ) ;
#41600=CARTESIAN_POINT ( 'NONE',  ( -10.00000000000000000, -5.773502691896252870, -173.6249999999999716 ) ) ;
#41604=CARTESIAN_POINT ( 'NONE',  ( 10.81189881249999729, 0.000000000000000000, -168.0312500020484094 ) ) ;
#41608=CARTESIAN_POINT ( 'NONE',  ( -10.81189881249999729, 1.324075727343319199E-15, -84.59375000204836681 ) ) ;
#41609=CARTESIAN_POINT ( 'NONE',  ( 10.81189881249999907, 6.242252689847868297, -194.7187500020484094 ) ) ;
#41610=CARTESIAN_POINT ( 'NONE',  ( -2.293366432827344421E-15, -12.48450537969573659, -91.90625000204838102 ) ) ;
#41614=CARTESIAN_POINT ( 'NONE',  ( -5.405949406250003975, -9.363379034771801557, -174.5312500020484094 ) ) ;
#41615=CARTESIAN_POINT ( 'NONE',  ( 10.81189881249999729, 0.000000000000000000, -187.5312500020484094 ) ) ;
#41617=CARTESIAN_POINT ( 'NONE',  ( -2.121150477449813534E-15, -11.54700538379251284, -160.2500000040967620 ) ) ;
#41619=CARTESIAN_POINT ( 'NONE',  ( -5.405949406250003975, -9.363379034771801557, -13.84375000204834905 ) ) ;
#41621=CARTESIAN_POINT ( 'NONE',  ( 5.405949406249999534, 9.363379034771803333, -125.5937500020483668 ) ) ;
#41623=CARTESIAN_POINT ( 'NONE',  ( -2.293366432827344421E-15, -12.48450537969573659, -24.40625000204838102 ) ) ;
#41626=CARTESIAN_POINT ( 'NONE',  ( -2.293366432827344421E-15, -12.48450537969573659, -114.4062500020483952 ) ) ;
#41629=CARTESIAN_POINT ( 'NONE',  ( 10.00000000000000000, 5.773502691896255534, -92.25000000409679046 ) ) ;
#41632=CARTESIAN_POINT ( 'NONE',  ( -10.81189881249999729, 1.324075727343319199E-15, -53.09375000204835970 ) ) ;
#41637=CARTESIAN_POINT ( 'NONE',  ( -4.999999999999996447, 8.660254037844387298, -18.37500000409675494 ) ) ;
#41642=CARTESIAN_POINT ( 'NONE',  ( 9.999999999999998224, 0.000000000000000000, -143.3750000040967905 ) ) ;
#41643=ORIENTED_EDGE ( 'NONE', *, *, #26060, .T. ) ;
#41650=CARTESIAN_POINT ( 'NONE',  ( 0.000000000000000000, 0.000000000000000000, -99.99999999999998579 ) ) ;
#41651=CARTESIAN_POINT ( 'NONE',  ( -9.999999999999998224, 1.224646799147353059E-15, -170.7500000000000000 ) ) ;
#41654=CARTESIAN_POINT ( 'NONE',  ( 5.405949406249992428, -9.363379034771808662, -192.2812500020484094 ) ) ;
#41658=CARTESIAN_POINT ( 'NONE',  ( -5.405949406250003975, -9.363379034771801557, -109.8437500020483810 ) ) ;
#41660=CARTESIAN_POINT ( 'NONE',  ( 10.81189881249999729, 0.000000000000000000, -115.5312500020483952 ) ) ;
#41662=CARTESIAN_POINT ( 'NONE',  ( -2.293366432827344421E-15, -12.48450537969573659, -124.7187500020483952 ) ) ;
#41664=DIRECTION ( 'NONE',  ( -1.000000000000000000, 0.000000000000000000, 0.000000000000000000 ) ) ;
#41665=CARTESIAN_POINT ( 'NONE',  ( 7.070501591499377789E-16, 11.54700538379251284, -144.1250000000000000 ) ) ;
#41666=CARTESIAN_POINT ( 'NONE',  ( 4.999999999999992006, -8.660254037844389075, -9.749999999999953815 ) ) ;
#41669=CARTESIAN_POINT ( 'NONE',  ( -2.121150477449813534E-15, -11.54700538379251284, -184.2500000040967905 ) ) ;
#41671=CARTESIAN_POINT ( 'NONE',  ( 10.81189881249999907, 6.242252689847868297, -37.21875000204835260 ) ) ;
#41673=CARTESIAN_POINT ( 'NONE',  ( 10.81189881249999729, 0.000000000000000000, -142.3437500020483810 ) ) ;
#41675=CYLINDRICAL_SURFACE ( 'NONE', #38286, 9.999999999999998224 ) ;
#41676=CARTESIAN_POINT ( 'NONE',  ( 7.070501591499377789E-16, 11.54700538379251284, -78.12500000000000000 ) ) ;
#41677=CARTESIAN_POINT ( 'NONE',  ( 10.81189881249999551, -6.242252689847874514, -144.1562500020484094 ) ) ;
#41681=CARTESIAN_POINT ( 'NONE',  ( 9.999999999999998224, 0.000000000000000000, -116.3750000040967905 ) ) ;
#41683=CARTESIAN_POINT ( 'NONE',  ( -5.405949406250003975, -9.363379034771801557, -75.34375000204838102 ) ) ;
#41687=CARTESIAN_POINT ( 'NONE',  ( -5.405949406250003975, -9.363379034771801557, -38.03125000204838102 ) ) ;
#41693=CARTESIAN_POINT ( 'NONE',  ( -5.000000000000003553, -8.660254037844383745, -173.8750000040968189 ) ) ;
#41694=ORIENTED_EDGE ( 'NONE', *, *, #29565, .F. ) ;
#41703=CARTESIAN_POINT ( 'NONE',  ( -10.81189881249999729, 1.324075727343319199E-15, -137.0937500020483810 ) ) ;
#41705=CARTESIAN_POINT ( 'NONE',  ( -10.81189881249999729, 1.324075727343319199E-15, -137.2812500020483810 ) ) ;
#41706=CARTESIAN_POINT ( 'NONE',  ( 5.405949406249999534, 9.363379034771803333, -148.0937500020483810 ) ) ;
#41709=CARTESIAN_POINT ( 'NONE',  ( -4.999999999999996447, 8.660254037844387298, -169.5000000000000000 ) ) ;
#41713=CARTESIAN_POINT ( 'NONE',  ( -10.81189881249999729, 1.324075727343319199E-15, -173.0937500020484094 ) ) ;
#41719=CARTESIAN_POINT ( 'NONE',  ( -5.405949406249996869, 9.363379034771805109, -38.53125000204838102 ) ) ;
#41721=CARTESIAN_POINT ( 'NONE',  ( -9.999999999999998224, 1.224646799147353059E-15, -101.7500000000000000 ) ) ;
#41723=CARTESIAN_POINT ( 'NONE',  ( 10.81189881249999729, 6.242252689847867408, -116.9062500020483952 ) ) ;
#41724=CARTESIAN_POINT ( 'NONE',  ( 4.999999999999992006, -8.660254037844389075, -140.6250000040967905 ) ) ;
#41730=CARTESIAN_POINT ( 'NONE',  ( -5.405949406250003975, -9.363379034771801557, -69.53125000204838102 ) ) ;
#41735=EDGE_CURVE ( 'NONE', #11758, #17267, #34730, .T. ) ;
#41736=VERTEX_POINT ( 'NONE', #2390 ) ;
#41739=VECTOR ( 'NONE', #22721, 1000.000000000000000 ) ;
#41741=VECTOR ( 'NONE', #20298, 1000.000000000000000 ) ;
#41753=VERTEX_POINT ( 'NONE', #42066 ) ;
#41754=CARTESIAN_POINT ( 'NONE',  ( -2.121150477449813534E-15, -11.54700538379251284, -36.87499999999996447 ) ) ;
#41758=CARTESIAN_POINT ( 'NONE',  ( 5.405949406249992428, -9.363379034771808662, -159.0937500020484094 ) ) ;
#41759=( BOUNDED_CURVE ( )  B_SPLINE_CURVE ( 2, ( #36996, #24488, #10867, #7431, #24058, #20582, #33772 ),
 .UNSPECIFIED., .F., .F. ) 
 B_SPLINE_CURVE_WITH_KNOTS ( ( 3, 2, 2, 3 ),
 ( 0.3694029850746269883, 0.3706467661691543181, 0.3718905472636816478, 0.3731343283582090331 ),
 .UNSPECIFIED. ) 
 CURVE ( )  GEOMETRIC_REPRESENTATION_ITEM ( )  RATIONAL_B_SPLINE_CURVE ( ( 0.9999999999999880096, 0.8660254037844506980, 1.000000000000000000, 0.8660254037844387076, 1.000000000000000000, 0.8660254037844327124, 1.000000000000005995 ) ) 
 REPRESENTATION_ITEM ( '' )  );
#41760=CARTESIAN_POINT ( 'NONE',  ( -10.81189881249999729, 6.242252689847871849, -171.7187500020483810 ) ) ;
#41764=CARTESIAN_POINT ( 'NONE',  ( 9.999999999999996447, -5.773502691896262640, -198.6250000000000284 ) ) ;
#41770=CARTESIAN_POINT ( 'NONE',  ( -10.81189881249999729, 1.324075727343319199E-15, -69.78125000204838102 ) ) ;
#41772=CARTESIAN_POINT ( 'NONE',  ( 9.999999999999996447, -5.773502691896262640, -123.6250000000000000 ) ) ;
#41773=CARTESIAN_POINT ( 'NONE',  ( 5.405949406249992428, -9.363379034771808662, -151.7812500020484094 ) ) ;
#41774=CARTESIAN_POINT ( 'NONE',  ( -5.405949406250003975, -9.363379034771801557, -164.0312500020484094 ) ) ;
#41776=CARTESIAN_POINT ( 'NONE',  ( -2.293366432827344421E-15, -12.48450537969573659, -99.21875000204839523 ) ) ;
#41779=CARTESIAN_POINT ( 'NONE',  ( -10.81189881249999729, 1.324075727343319199E-15, -194.0937500020484094 ) ) ;
#41782=CARTESIAN_POINT ( 'NONE',  ( -8.460957583164166351, -5.382509563854436685, -180.0000000000000853 ) ) ;
#41784=CARTESIAN_POINT ( 'NONE',  ( 5.405949406249992428, -9.363379034771808662, -91.78125000204838102 ) ) ;
#41786=CARTESIAN_POINT ( 'NONE',  ( 4.999999999999992006, -8.660254037844389075, -67.12500000409676204 ) ) ;
#41788=CARTESIAN_POINT ( 'NONE',  ( -5.405949406249996869, 9.363379034771805109, -24.84375000204835970 ) ) ;
#41789=ORIENTED_EDGE ( 'NONE', *, *, #27249, .T. ) ;
#41791=CARTESIAN_POINT ( 'NONE',  ( 5.405949406249992428, -9.363379034771808662, -24.28125000204836681 ) ) ;
#41800=CARTESIAN_POINT ( 'NONE',  ( 9.999999999999998224, 0.000000000000000000, -116.3750000040967905 ) ) ;
#41808=CARTESIAN_POINT ( 'NONE',  ( 7.320067886350967612, 7.614036460224446579, -99.99999999999998579 ) ) ;
#41811=CARTESIAN_POINT ( 'NONE',  ( 5.405949406249992428, -9.363379034771808662, -153.2812500020484094 ) ) ;
#41816=CARTESIAN_POINT ( 'NONE',  ( -5.405949406250003975, -9.363379034771801557, -84.34375000204836681 ) ) ;
#41817=CARTESIAN_POINT ( 'NONE',  ( 10.81189881249999729, 0.000000000000000000, -90.03125000204838102 ) ) ;
#41821=CARTESIAN_POINT ( 'NONE',  ( 5.405949406249999534, 9.363379034771803333, -175.2812500020484094 ) ) ;
#41822=CARTESIAN_POINT ( 'NONE',  ( 5.405949406249999534, 9.363379034771803333, -185.7812500020484094 ) ) ;
#41824=CARTESIAN_POINT ( 'NONE',  ( 9.999999999999998224, 0.000000000000000000, -162.8750000040967905 ) ) ;
#41826=CARTESIAN_POINT ( 'NONE',  ( 5.405949406249999534, 9.363379034771803333, -17.59375000204835260 ) ) ;
#41827=CARTESIAN_POINT ( 'NONE',  ( -5.000000000000003553, -8.660254037844383745, -157.0000000000000000 ) ) ;
#41828=CARTESIAN_POINT ( 'NONE',  ( -5.405949406250003975, -9.363379034771801557, -121.8437500020483952 ) ) ;
#41830=CARTESIAN_POINT ( 'NONE',  ( -5.405949406249996869, 9.363379034771805109, -17.53125000204835970 ) ) ;
#41833=CARTESIAN_POINT ( 'NONE',  ( -10.81189881249999729, 1.324075727343319199E-15, -113.2812500020483952 ) ) ;
#41835=ORIENTED_EDGE ( 'NONE', *, *, #19278, .T. ) ;
#41836=CARTESIAN_POINT ( 'NONE',  ( -5.000000000000003553, -8.660254037844383745, -92.87500000409677625 ) ) ;
#41837=LINE ( 'NONE', #36644, #21546 ) ;
#41839=CARTESIAN_POINT ( 'NONE',  ( -10.81189881249999729, 6.242252689847871849, -50.21875000204837391 ) ) ;
#41844=CARTESIAN_POINT ( 'NONE',  ( -4.999999999999996447, 8.660254037844387298, -22.87500000409675849 ) ) ;
#41845=DIRECTION ( 'NONE',  ( -0.000000000000000000, -0.000000000000000000, -1.000000000000000000 ) ) ;
#41850=ORIENTED_EDGE ( 'NONE', *, *, #40713, .T. ) ;
#41856=ORIENTED_EDGE ( 'NONE', *, *, #1558, .F. ) ;
#41857=CARTESIAN_POINT ( 'NONE',  ( -4.999999999999996447, 8.660254037844387298, -175.5000000000000284 ) ) ;
#41858=CARTESIAN_POINT ( 'NONE',  ( 10.00000000000000000, 5.773502691896255534, -171.3750000000000000 ) ) ;
#41860=CARTESIAN_POINT ( 'NONE',  ( -10.81189881249999729, 1.324075727343319199E-15, -191.2812500020484094 ) ) ;
#41863=CARTESIAN_POINT ( 'NONE',  ( 5.405949406249992428, -9.363379034771808662, -106.5937500020483810 ) ) ;
#41865=CARTESIAN_POINT ( 'NONE',  ( 7.644554776091147741E-16, 12.48450537969573659, -119.6562500020484094 ) ) ;
#41867=CARTESIAN_POINT ( 'NONE',  ( 10.81189881249999729, 6.242252689847867408, -125.7187500020483810 ) ) ;
#41871=CARTESIAN_POINT ( 'NONE',  ( 10.00000000000000000, 5.773502691896255534, -138.3750000000000000 ) ) ;
#41872=CARTESIAN_POINT ( 'NONE',  ( 9.999999999999996447, -5.773502691896262640, -12.62499999999996980 ) ) ;
#41875=CARTESIAN_POINT ( 'NONE',  ( -5.000000000000003553, -8.660254037844383745, -187.3750000040967905 ) ) ;
#41877=AXIS2_PLACEMENT_3D ( 'NONE', #33082, #29848, #6958 ) ;
#41878=CARTESIAN_POINT ( 'NONE',  ( -10.81189881249999907, -6.242252689847864744, -39.46875000204835970 ) ) ;
#41879=CARTESIAN_POINT ( 'NONE',  ( -2.121150477449813534E-15, -11.54700538379251284, -107.7500000040967763 ) ) ;
#41880=CARTESIAN_POINT ( 'NONE',  ( 10.81189881249999729, 0.000000000000000000, -146.8437500020483810 ) ) ;
#41883=CARTESIAN_POINT ( 'NONE',  ( -9.999999999999479527, -5.773502691896549521, -102.0000000040967620 ) ) ;
#41884=CARTESIAN_POINT ( 'NONE',  ( -4.999999999999996447, 8.660254037844387298, -77.99999999999998579 ) ) ;
#41885=CARTESIAN_POINT ( 'NONE',  ( -5.405949406249996869, 9.363379034771805109, -140.5312500020484094 ) ) ;
#41890=CARTESIAN_POINT ( 'NONE',  ( -5.000000000000003553, -8.660254037844383745, -112.3750000040967763 ) ) ;
#41892=CARTESIAN_POINT ( 'NONE',  ( 10.81189881249999729, 0.000000000000000000, -74.84375000204838102 ) ) ;
#41896=CARTESIAN_POINT ( 'NONE',  ( -9.999999999999227285, -5.773502691896698735, -132.0000000040967620 ) ) ;
#41897=CARTESIAN_POINT ( 'NONE',  ( -10.81189881249999729, 6.242252689847871849, -33.90625000204835970 ) ) ;
#41898=( BOUNDED_CURVE ( )  B_SPLINE_CURVE ( 2, ( #27613, #40753, #24173, #24393, #39911, #23530, #20910, #26964, #33885, #17024, #13781, #30223, #662, #12258, #31293, #18098, #21339, #28261, #21987, #31506, #28694, #9038, #25034, #34743, #41174, #34955, #8411, #2150, #34527, #22203, #38176, #5164, #11613, #38598, #1936, #4951, #18316, #28482, #41821, #15062, #1724, #15285, #8620, #14851, #41614, #41399, #21776, #24821, #11833, #31935, #28048, #37966, #25453, #15489, #37748, #5379, #21562, #35164, #18530, #31720, #8192, #35378, #2362, #12048, #25244, #38389, #8830, #5590, #18743, #5803, #18956, #1507, #14641, #27830, #40962, #11405, #24599, #15702, #9669, #12672, #16328, #16117, #2781, #36422, #19794, #22842, #32766, #19377, #9878, #6440, #6857, #35800, #25868, #32143, #6017, #39443, #15909, #2992, #29527, #42669, #29314, #32357, #10086, #39647, #29111, #9459, #23263, #42458, #13093, #2573, #28901, #42247, #42036, #13311, #22626, #6231, #39023, #12465, #32981, #25659, #32565, #38814, #23051, #9241, #3202, #26294, #12886, #19167, #26080, #22411, #6644, #35589, #19583, #36208, #36004, #39231, #3410, #16546, #29744, #190, #26500, #33201, #20224, #1243, #16760, #30805, #7075, #36628, #39860, #3632, #33832, #10716, #34046, #40484, #20862, #4257, #10930, #7713, #37484, #7493, #33414, #14368, #17399, #26708, #40074, #20009, #611, #4468, #7283, #29960, #23910, #26916, #20646, #10294, #27565, #818, #10505, #16975, #40699, #20436, #23480, #37055, #30597, #13522, #3841, #27348, #400, #30173, #1027, #40276, #24124, #13727, #27133, #14149, #23692, #4043, #36839, #33621, #37264, #17187, #17610, #30385, #11143, #13940, #24342, #14589, #8570, #4900, #17829, #27779, #41566, #38127, #12000, #25195, #18047, #1671, #38336, #40914, #15443, #2102, #31243, #31886, #34265, #28213, #14799, #34903, #41773, #18690, #8778, #28430, #11356, #24551, #24772, #37916, #21935, #41346, #5325, #27995, #8143, #18480, #37701, #34478, #21512, #31668, #15232, #34693, #12206, #31025, #8360, #21291, #21720, #11565, #5539, #2316, #5113, #41125, #35115, #28642, #18262, #25399, #31451, #1885, #7927, #21077, #4681, #15014, #11783, #1455, #24984, #19120, #41986, #19746, #13257, #5968, #9821, #12623, #12415, #2941, #6179, #16493, #26029, #22788, #36157, #9408, #38766, #6590, #9615, #32512, #9193, #39181, #38972, #16070, #35539, #22571, #26239, #22363, #15650, #23003, #32927, #32091, #35751, #29691, #19318, #5756, #135, #35949, #38545, #39388, #6391, #42196, #29263, #28850, #25608, #42407, #3360, #32305, #12838, #8986, #2727, #32716, #19532, #15859, #3149, #25817, #16277, #22154, #29475, #29058, #35329, #18909, #42617, #13045, #2525, #4203, #766, #1190, #30120, #7023, #26444, #344, #33780, #40024, #23855, #10662, #10454, #17557, #36369, #557, #33146, #27085, #13678, #24068, #37210, #26869, #13465, #17346, #13892, #10240, #30550, #3575, #7439, #4417, #27297, #30757, #33364, #29905, #6805, #26658, #20175, #39808, #7657, #39596, #36576, #10030, #40228, #17135, #40432, #977, #10876, #37004, #14095, #3785, #30337, #16919, #33996, #20810, #20592, #16708, #23645, #23211, #36791, #19960, #7228, #23428, #20379, #33568, #3992, #34215, #21887, #17777, #38287, #1403, #14533, #37435, #31617, #27512, #31402, #14963, #34638, #21025, #18428, #37650, #5064, #4846, #35066, #8733, #11734, #4631, #34426, #31837, #8090, #30973, #27727, #41071, #34853, #1620, #41519, #5493, #28377, #31190, #40863, #21454, #24718, #18643, #1837, #18212, #28161, #7878, #11304, #21670, #11088, #8309, #24498, #41295, #14749, #24933, #21241, #27944, #2050, #17990, #11516, #11949, #25140, #37864, #38077, #8517, #5275, #15181, #14312, #40646, #24291, #3103, #29219, #5921, #9359, #22107, #18866, #22528, #29431, #5714, #35701, #32674, #32046, #39135, #42150, #26191, #28592, #6130, #25567, #42358, #36113, #15604, #6546, #16231, #19273, #2893, #32253, #22741, #32469, #19700, #19072, #38719, #2274, #2475, #9567, #28806, #15814, #12791, #25983, #29010, #15395, #22958, #9778, #41938, #22320, #41723, #12581, #35907, #12161, #25353, #12369, #38500, #39339, #35495, #2680, #9153, #8943, #42572, #35281, #25774, #38927, #6344, #16023, #19487, #12995, #16659, #9983, #17303, #4158, #26402, #30076, #29860, #10616, #23162, #26824, #39552, #33528, #298, #86, #36325, #23804, #6756, #19910, #10408, #30507, #33097, #39977, #20548, #3523, #27042, #517, #14051, #16444, #23600, #13419, #17089, #24024, #934, #36958, #7400, #26614, #3951, #20128, #33737, #7182, #7611, #36532, #39763, #32883, #10197, #40186, #23383, #3741, #30288, #727, #16871, #37164, #13208, #6973, #33316, #13846, #40387, #13632, #27246, #3314, #29642, #36745, #20336, #10830, #40820, #11260, #20982, #41468, #21631, #11903, #27682, #24240, #1142, #37391, #1357, #7834, #21194, #34168, #4588, #14266, #38034, #33954, #37819, #21407, #41029, #27468, #24885, #14487, #11472, #24457, #28330, #2006, #18165, #40603, #37604, #38244, #17727, #30922, #11046, #4797, #41247, #8047, #5232, #15133, #34809, #34381, #17946, #27896, #31144, #25098, #8262, #24673, #34593, #1577, #14706, #28119, #20765, #1790 ),
 .UNSPECIFIED., .F., .F. ) 
 B_SPLINE_CURVE_WITH_KNOTS ( ( 3, 2, 2, 2, 2, 2, 2, 2, 2, 2, 2, 2, 2, 2, 2, 2, 2, 2, 2, 2, 2, 2, 2, 2, 2, 2, 2, 2, 2, 2, 2, 2, 2, 2, 2, 2, 2, 2, 2, 2, 2, 2, 2, 2, 2, 2, 2, 2, 2, 2, 2, 2, 2, 2, 2, 2, 2, 2, 2, 2, 2, 2, 2, 2, 2, 2, 2, 2, 2, 2, 2, 2, 2, 2, 2, 2, 2, 2, 2, 2, 2, 2, 2, 2, 2, 2, 2, 2, 2, 2, 2, 2, 2, 2, 2, 2, 2, 2, 2, 2, 2, 2, 2, 2, 2, 2, 2, 2, 2, 2, 2, 2, 2, 2, 2, 2, 2, 2, 2, 2, 2, 2, 2, 2, 2, 2, 2, 2, 2, 2, 2, 2, 2, 2, 2, 2, 2, 2, 2, 2, 2, 2, 2, 2, 2, 2, 2, 2, 2, 2, 2, 2, 2, 2, 2, 2, 2, 2, 2, 2, 2, 2, 2, 2, 2, 2, 2, 2, 2, 2, 2, 2, 2, 2, 2, 2, 2, 2, 2, 2, 2, 2, 2, 2, 2, 2, 2, 2, 2, 2, 2, 2, 2, 2, 2, 2, 2, 2, 2, 2, 2, 2, 2, 2, 2, 2, 2, 2, 2, 2, 2, 2, 2, 2, 2, 2, 2, 2, 2, 2, 2, 2, 2, 2, 2, 2, 2, 2, 2, 2, 2, 2, 2, 2, 2, 2, 2, 2, 2, 2, 2, 2, 2, 2, 2, 2, 2, 2, 2, 2, 2, 2, 2, 2, 2, 2, 2, 2, 2, 2, 2, 2, 2, 2, 2, 2, 2, 2, 2, 2, 2, 2, 2, 2, 2, 2, 2, 2, 2, 2, 2, 2, 2, 2, 2, 2, 2, 2, 2, 2, 2, 2, 2, 2, 2, 2, 2, 2, 2, 2, 2, 2, 2, 2, 2, 2, 2, 2, 2, 2, 2, 2, 2, 2, 2, 2, 2, 2, 2, 2, 2, 3 ),
 ( 0.09718516234321271374, 0.09825870646766168837, 0.09950248756218905977, 0.1007462686567164173, 0.1019900497512437748, 0.1032338308457711462, 0.1044776119402985037, 0.1057213930348258751, 0.1069651741293532327, 0.1082089552238805902, 0.1094527363184079616, 0.1106965174129353191, 0.1119402985074626905, 0.1131840796019900480, 0.1144278606965174194, 0.1156716417910447769, 0.1169154228855721345, 0.1181592039800995059, 0.1194029850746268634, 0.1206467661691542348, 0.1218905472636815923, 0.1231343283582089498, 0.1243781094527363212, 0.1256218905472636926, 0.1268656716417910502, 0.1281094527363184077, 0.1293532338308457652, 0.1305970149253731227, 0.1318407960199005080, 0.1330845771144278655, 0.1343283582089552231, 0.1355721393034825806, 0.1368159203980099381, 0.1380597014925373234, 0.1393034825870646809, 0.1405472636815920384, 0.1417910447761193959, 0.1430348258706467535, 0.1442786069651741387, 0.1455223880597014963, 0.1467661691542288538, 0.1480099502487562113, 0.1492537313432835688, 0.1504975124378109541, 0.1517412935323383116, 0.1529850746268656692, 0.1542288557213930267, 0.1554726368159203842, 0.1567164179104477695, 0.1579601990049751270, 0.1592039800995024845, 0.1604477611940298420, 0.1616915422885572273, 0.1629353233830845848, 0.1641791044776119424, 0.1654228855721392999, 0.1666666666666666574, 0.1679104477611940427, 0.1691542288557214002, 0.1703980099502487577, 0.1716417910447761153, 0.1728855721393034728, 0.1741293532338308581, 0.1753731343283582156, 0.1766169154228855731, 0.1778606965174129306, 0.1791044776119402882, 0.1803482587064676734, 0.1815920398009950310, 0.1828358208955223885, 0.1840796019900497460, 0.1853233830845771035, 0.1865671641791044888, 0.1878109452736318463, 0.1890547263681591761, 0.1902985074626865614, 0.1915422885572139189, 0.1927860696517413042, 0.1940298507462686617, 0.1952736318407959915, 0.1965174129353233767, 0.1977611940298507343, 0.1990049751243781195, 0.2002487562189054771, 0.2014925373134328623, 0.2027363184079601921, 0.2039800995024875496, 0.2052238805970149349, 0.2064676616915422924, 0.2077114427860696777, 0.2089552238805970075, 0.2101990049751243650, 0.2114427860696517503, 0.2126865671641791078, 0.2139303482587064931, 0.2151741293532338228, 0.2164179104477611804, 0.2176616915422885656, 0.2189054726368159232, 0.2201492537313432807, 0.2213930348258706382, 0.2226368159203980235, 0.2238805970149254088, 0.2251243781094527385, 0.2263681592039801238, 0.2276119402985074536, 0.2288557213930348389, 0.2300995024875622241, 0.2313432835820895539, 0.2325870646766169392, 0.2338308457711442689, 0.2350746268656716542, 0.2363184079601990395, 0.2375621890547263693, 0.2388059701492537545, 0.2400497512437810843, 0.2412935323383084696, 0.2425373134328358549, 0.2437810945273631846, 0.2450248756218905699, 0.2462686567164178997, 0.2475124378109452850, 0.2487562189054726702, 0.2500000000000000000, 0.2512437810945273853, 0.2524875621890547150, 0.2537313432835821003, 0.2549751243781094301, 0.2562189054726368154, 0.2574626865671642006, 0.2587064676616914749, 0.2599502487562189157, 0.2611940298507462455, 0.2624378109452736307, 0.2636815920398010160, 0.2649253731343282903, 0.2661691542288557311, 0.2674129353233830608, 0.2686567164179104461, 0.2699004975124378314, 0.2711442786069651611, 0.2723880597014925464, 0.2736318407960198762, 0.2748756218905472615, 0.2761194029850746468, 0.2773631840796019765, 0.2786069651741293618, 0.2798507462686566361, 0.2810945273631840768, 0.2823383084577114621, 0.2835820895522387919, 0.2848258706467661772, 0.2860696517412934514, 0.2873134328358208922, 0.2885572139303482775, 0.2898009950248756073, 0.2910447761194029925, 0.2922885572139302668, 0.2935323383084577076, 0.2947761194029850929, 0.2960199004975124226, 0.2972636815920398079, 0.2985074626865670822, 0.2997512437810945229, 0.3009950248756219082, 0.3022388059701492380, 0.3034825870646766233, 0.3047263681592038975, 0.3059701492537313383, 0.3072139303482587236, 0.3084577114427860534, 0.3097014925373134386, 0.3109452736318407684, 0.3121890547263681537, 0.3134328358208955390, 0.3146766169154228687, 0.3159203980099502540, 0.3171641791044776393, 0.3184079601990049690, 0.3196517412935323543, 0.3208955223880596841, 0.3221393034825870694, 0.3233830845771144546, 0.3246268656716417844, 0.3258706467661691697, 0.3271144278606964995, 0.3283582089552238847, 0.3296019900497512700, 0.3308457711442785998, 0.3320895522388059851, 0.3333333333333333148, 0.3345771144278607001, 0.3358208955223880854, 0.3370646766169154152, 0.3383084577114428004, 0.3395522388059701302, 0.3407960199004975155, 0.3420398009950249008, 0.3432835820895522305, 0.3445273631840796158, 0.3457711442786069456, 0.3470149253731343308, 0.3482587064676617161, 0.3495024875621890459, 0.3507462686567164312, 0.3519900497512437609, 0.3532338308457711462, 0.3544776119402985315, 0.3557213930348258613, 0.3569651741293532465, 0.3582089552238805763, 0.3594527363184079616, 0.3606965174129353469, 0.3619402985074626766, 0.3631840796019900619, 0.3644278606965173917, 0.3656716417910447769, 0.3669154228855721622, 0.3681592039800994920, 0.3694029850746268773, 0.3706467661691542070, 0.3718905472636815923, 0.3731343283582089776, 0.3743781094527363074, 0.3756218905472636926, 0.3768656716417910224, 0.3781094527363184077, 0.3793532338308457930, 0.3805970149253731227, 0.3818407960199005080, 0.3830845771144278378, 0.3843283582089552231, 0.3855721393034826083, 0.3868159203980099381, 0.3880597014925373234, 0.3893034825870646531, 0.3905472636815920384, 0.3917910447761194237, 0.3930348258706467535, 0.3942786069651741387, 0.3955223880597014685, 0.3967661691542288538, 0.3980099502487562391, 0.3992537313432835688, 0.4004975124378109541, 0.4017412935323382839, 0.4029850746268656692, 0.4042288557213930544, 0.4054726368159203842, 0.4067164179104477695, 0.4079601990049750992, 0.4092039800995024845, 0.4104477611940298698, 0.4116915422885571996, 0.4129353233830845848, 0.4141791044776118591, 0.4154228855721392999, 0.4166666666666666852, 0.4179104477611940704, 0.4191542288557214002, 0.4203980099502487300, 0.4216417910447761708, 0.4228855721393035005, 0.4241293532338308303, 0.4253731343283582156, 0.4266169154228854898, 0.4278606965174129306, 0.4291044776119403159, 0.4303482587064677012, 0.4315920398009950310, 0.4328358208955223607, 0.4340796019900497460, 0.4353233830845771313, 0.4365671641791044610, 0.4378109452736318463, 0.4390547263681592316, 0.4402985074626865614, 0.4415422885572139466, 0.4427860696517413319, 0.4440298507462686617, 0.4452736318407960470, 0.4465174129353233767, 0.4477611940298507620, 0.4490049751243780918, 0.4502487562189054771, 0.4514925373134328623, 0.4527363184079601921, 0.4539800995024875774, 0.4552238805970149627, 0.4564676616915422924, 0.4577114427860696777, 0.4589552238805970075, 0.4601990049751243927, 0.4614427860696517225, 0.4626865671641791078, 0.4639303482587064931, 0.4651741293532338228, 0.4664179104477612081, 0.4676616915422885379, 0.4689054726368159232, 0.4701492537313433084, 0.4713930348258706382, 0.4726368159203980235, 0.4738805970149253532, 0.4751243781094527385, 0.4763681592039801238, 0.4776119402985074536, 0.4788557213930348389, 0.4800995024875621686, 0.4813432835820895539, 0.4825870646766169392, 0.4838308457711442689, 0.4850746268656716542, 0.4863184079601989840, 0.4875621890547263693, 0.4888059701492537545, 0.4900497512437810843, 0.4912935323383084696, 0.4925373134328357994, 0.4937810945273631846, 0.4950248756218905699, 0.4951951125919689112 ),
 .UNSPECIFIED. ) 
 CURVE ( )  GEOMETRIC_REPRESENTATION_ITEM ( )  RATIONAL_B_SPLINE_CURVE ( ( 0.9683452906431517793, 0.8843625769635171663, 1.000000000000000000, 0.8660254037844387076, 1.000000000000000000, 0.8660254037844387076, 1.000000000000000000, 0.8660254037844387076, 1.000000000000000000, 0.8660254037844387076, 1.000000000000000000, 0.8660254037844387076, 1.000000000000000000, 0.8660254037844387076, 1.000000000000000000, 0.8660254037844387076, 1.000000000000000000, 0.8660254037844387076, 1.000000000000000000, 0.8660254037844387076, 1.000000000000000000, 0.8660254037844387076, 1.000000000000000000, 0.8660254037844387076, 1.000000000000000000, 0.8660254037844387076, 1.000000000000000000, 0.8660254037844387076, 1.000000000000000000, 0.8660254037844387076, 1.000000000000000000, 0.8660254037844387076, 1.000000000000000000, 0.8660254037844387076, 1.000000000000000000, 0.8660254037844387076, 1.000000000000000000, 0.8660254037844387076, 1.000000000000000000, 0.8660254037844387076, 1.000000000000000000, 0.8660254037844387076, 1.000000000000000000, 0.8660254037844387076, 1.000000000000000000, 0.8660254037844387076, 1.000000000000000000, 0.8660254037844387076, 1.000000000000000000, 0.8660254037844387076, 1.000000000000000000, 0.8660254037844387076, 1.000000000000000000, 0.8660254037844387076, 1.000000000000000000, 0.8660254037844387076, 1.000000000000000000, 0.8660254037844387076, 1.000000000000000000, 0.8660254037844387076, 1.000000000000000000, 0.8660254037844387076, 1.000000000000000000, 0.8660254037844387076, 1.000000000000000000, 0.8660254037844387076, 1.000000000000000000, 0.8660254037844387076, 1.000000000000000000, 0.8660254037844387076, 1.000000000000000000, 0.8660254037844387076, 1.000000000000000000, 0.8660254037844387076, 1.000000000000000000, 0.8660254037844387076, 1.000000000000000000, 0.8660254037844387076, 1.000000000000000000, 0.8660254037844387076, 1.000000000000000000, 0.8660254037844387076, 1.000000000000000000, 0.8660254037844387076, 1.000000000000000000, 0.8660254037844387076, 1.000000000000000000, 0.8660254037844387076, 1.000000000000000000, 0.8660254037844387076, 1.000000000000000000, 0.8660254037844387076, 1.000000000000000000, 0.8660254037844387076, 1.000000000000000000, 0.8660254037844387076, 1.000000000000000000, 0.8660254037844387076, 1.000000000000000000, 0.8660254037844387076, 1.000000000000000000, 0.8660254037844387076, 1.000000000000000000, 0.8660254037844387076, 1.000000000000000000, 0.8660254037844387076, 1.000000000000000000, 0.8660254037844387076, 1.000000000000000000, 0.8660254037844387076, 1.000000000000000000, 0.8660254037844387076, 1.000000000000000000, 0.8660254037844387076, 1.000000000000000000, 0.8660254037844387076, 1.000000000000000000, 0.8660254037844387076, 1.000000000000000000, 0.8660254037844387076, 1.000000000000000000, 0.8660254037844387076, 1.000000000000000000, 0.8660254037844387076, 1.000000000000000000, 0.8660254037844387076, 1.000000000000000000, 0.8660254037844387076, 1.000000000000000000, 0.8660254037844387076, 1.000000000000000000, 0.8660254037844387076, 1.000000000000000000, 0.8660254037844387076, 1.000000000000000000, 0.8660254037844387076, 1.000000000000000000, 0.8660254037844387076, 1.000000000000000000, 0.8660254037844387076, 1.000000000000000000, 0.8660254037844387076, 1.000000000000000000, 0.8660254037844387076, 1.000000000000000000, 0.8660254037844387076, 1.000000000000000000, 0.8660254037844387076, 1.000000000000000000, 0.8660254037844387076, 1.000000000000000000, 0.8660254037844387076, 1.000000000000000000, 0.8660254037844387076, 1.000000000000000000, 0.8660254037844387076, 1.000000000000000000, 0.8660254037844387076, 1.000000000000000000, 0.8660254037844387076, 1.000000000000000000, 0.8660254037844387076, 1.000000000000000000, 0.8660254037844387076, 1.000000000000000000, 0.8660254037844387076, 1.000000000000000000, 0.8660254037844387076, 1.000000000000000000, 0.8660254037844387076, 1.000000000000000000, 0.8660254037844387076, 1.000000000000000000, 0.8660254037844387076, 1.000000000000000000, 0.8660254037844387076, 1.000000000000000000, 0.8660254037844387076, 1.000000000000000000, 0.8660254037844387076, 1.000000000000000000, 0.8660254037844387076, 1.000000000000000000, 0.8660254037844387076, 1.000000000000000000, 0.8660254037844387076, 1.000000000000000000, 0.8660254037844387076, 1.000000000000000000, 0.8660254037844387076, 1.000000000000000000, 0.8660254037844387076, 1.000000000000000000, 0.8660254037844387076, 1.000000000000000000, 0.8660254037844387076, 1.000000000000000000, 0.8660254037844387076, 1.000000000000000000, 0.8660254037844387076, 1.000000000000000000, 0.8660254037844387076, 1.000000000000000000, 0.8660254037844387076, 1.000000000000000000, 0.8660254037844387076, 1.000000000000000000, 0.8660254037844387076, 1.000000000000000000, 0.8660254037844387076, 1.000000000000000000, 0.8660254037844387076, 1.000000000000000000, 0.8660254037844387076, 1.000000000000000000, 0.8660254037844387076, 1.000000000000000000, 0.8660254037844387076, 1.000000000000000000, 0.8660254037844387076, 1.000000000000000000, 0.8660254037844387076, 1.000000000000000000, 0.8660254037844387076, 1.000000000000000000, 0.8660254037844387076, 1.000000000000000000, 0.8660254037844387076, 1.000000000000000000, 0.8660254037844387076, 1.000000000000000000, 0.8660254037844387076, 1.000000000000000000, 0.8660254037844387076, 1.000000000000000000, 0.8660254037844387076, 1.000000000000000000, 0.8660254037844387076, 1.000000000000000000, 0.8660254037844387076, 1.000000000000000000, 0.8660254037844387076, 1.000000000000000000, 0.8660254037844387076, 1.000000000000000000, 0.8660254037844387076, 1.000000000000000000, 0.8660254037844387076, 1.000000000000000000, 0.8660254037844387076, 1.000000000000000000, 0.8660254037844387076, 1.000000000000000000, 0.8660254037844387076, 1.000000000000000000, 0.8660254037844387076, 1.000000000000000000, 0.8660254037844387076, 1.000000000000000000, 0.8660254037844387076, 1.000000000000000000, 0.8660254037844387076, 1.000000000000000000, 0.8660254037844387076, 1.000000000000000000, 0.8660254037844387076, 1.000000000000000000, 0.8660254037844387076, 1.000000000000000000, 0.8660254037844387076, 1.000000000000000000, 0.8660254037844387076, 1.000000000000000000, 0.8660254037844387076, 1.000000000000000000, 0.8660254037844387076, 1.000000000000000000, 0.8660254037844387076, 1.000000000000000000, 0.8660254037844387076, 1.000000000000000000, 0.8660254037844387076, 1.000000000000000000, 0.8660254037844387076, 1.000000000000000000, 0.8660254037844387076, 1.000000000000000000, 0.8660254037844387076, 1.000000000000000000, 0.8660254037844387076, 1.000000000000000000, 0.8660254037844387076, 1.000000000000000000, 0.8660254037844387076, 1.000000000000000000, 0.8660254037844387076, 1.000000000000000000, 0.8660254037844387076, 1.000000000000000000, 0.8660254037844387076, 1.000000000000000000, 0.8660254037844387076, 1.000000000000000000, 0.8660254037844387076, 1.000000000000000000, 0.8660254037844387076, 1.000000000000000000, 0.8660254037844387076, 1.000000000000000000, 0.8660254037844387076, 1.000000000000000000, 0.8660254037844387076, 1.000000000000000000, 0.8660254037844387076, 1.000000000000000000, 0.8660254037844387076, 1.000000000000000000, 0.8660254037844387076, 1.000000000000000000, 0.8660254037844387076, 1.000000000000000000, 0.8660254037844387076, 1.000000000000000000, 0.8660254037844387076, 1.000000000000000000, 0.8660254037844387076, 1.000000000000000000, 0.8660254037844387076, 1.000000000000000000, 0.8660254037844387076, 1.000000000000000000, 0.8660254037844387076, 1.000000000000000000, 0.8660254037844387076, 1.000000000000000000, 0.8660254037844387076, 1.000000000000000000, 0.8660254037844387076, 1.000000000000000000, 0.8660254037844387076, 1.000000000000000000, 0.8660254037844387076, 1.000000000000000000, 0.8660254037844387076, 1.000000000000000000, 0.8660254037844387076, 1.000000000000000000, 0.8660254037844387076, 1.000000000000000000, 0.8660254037844387076, 1.000000000000000000, 0.8660254037844387076, 1.000000000000000000, 0.8660254037844387076, 1.000000000000000000, 0.8660254037844387076, 1.000000000000000000, 0.8660254037844387076, 1.000000000000000000, 0.8660254037844387076, 1.000000000000000000, 0.8660254037844387076, 1.000000000000000000, 0.8660254037844387076, 1.000000000000000000, 0.8660254037844387076, 1.000000000000000000, 0.8660254037844387076, 1.000000000000000000, 0.8660254037844387076, 1.000000000000000000, 0.8660254037844387076, 1.000000000000000000, 0.8660254037844387076, 1.000000000000000000, 0.8660254037844387076, 1.000000000000000000, 0.8660254037844387076, 1.000000000000000000, 0.8660254037844387076, 1.000000000000000000, 0.8660254037844387076, 1.000000000000000000, 0.8660254037844387076, 1.000000000000000000, 0.8660254037844387076, 1.000000000000000000, 0.8660254037844387076, 1.000000000000000000, 0.8660254037844387076, 1.000000000000000000, 0.8660254037844387076, 1.000000000000000000, 0.8660254037844387076, 1.000000000000000000, 0.8660254037844387076, 1.000000000000000000, 0.8660254037844387076, 1.000000000000000000, 0.8660254037844387076, 1.000000000000000000, 0.8660254037844387076, 1.000000000000000000, 0.8660254037844387076, 1.000000000000000000, 0.8660254037844387076, 1.000000000000000000, 0.8660254037844387076, 1.000000000000000000, 0.8660254037844387076, 1.000000000000000000, 0.8660254037844387076, 1.000000000000000000, 0.8660254037844387076, 1.000000000000000000, 0.8660254037844387076, 1.000000000000000000, 0.8660254037844387076, 1.000000000000000000, 0.8660254037844387076, 1.000000000000000000, 0.8660254037844387076, 1.000000000000000000, 0.8660254037844387076, 1.000000000000000000, 0.8660254037844387076, 1.000000000000000000, 0.8660254037844387076, 1.000000000000000000, 0.8660254037844387076, 1.000000000000000000, 0.8660254037844387076, 1.000000000000000000, 0.8660254037844387076, 1.000000000000000000, 0.8660254037844387076, 1.000000000000000000, 0.8660254037844387076, 1.000000000000000000, 0.8660254037844387076, 1.000000000000000000, 0.8660254037844387076, 1.000000000000000000, 0.8660254037844387076, 1.000000000000000000, 0.8660254037844387076, 1.000000000000000000, 0.8660254037844387076, 1.000000000000000000, 0.8660254037844387076, 1.000000000000000000, 0.8660254037844387076, 1.000000000000000000, 0.8660254037844387076, 1.000000000000000000, 0.8660254037844387076, 1.000000000000000000, 0.8660254037844387076, 1.000000000000000000, 0.8660254037844387076, 1.000000000000000000, 0.8660254037844387076, 1.000000000000000000, 0.8660254037844387076, 1.000000000000000000, 0.8660254037844387076, 1.000000000000000000, 0.8660254037844387076, 1.000000000000000000, 0.8660254037844387076, 1.000000000000000000, 0.8660254037844387076, 1.000000000000000000, 0.8660254037844387076, 1.000000000000000000, 0.8660254037844387076, 1.000000000000000000, 0.8660254037844387076, 1.000000000000000000, 0.8660254037844387076, 1.000000000000000000, 0.8660254037844387076, 1.000000000000000000, 0.8660254037844387076, 1.000000000000000000, 0.8660254037844387076, 1.000000000000000000, 0.8660254037844387076, 1.000000000000000000, 0.8660254037844387076, 1.000000000000000000, 0.8660254037844387076, 1.000000000000000000, 0.8660254037844387076, 1.000000000000000000, 0.8660254037844387076, 1.000000000000000000, 0.8660254037844387076, 1.000000000000000000, 0.8660254037844387076, 1.000000000000000000, 0.8660254037844387076, 1.000000000000000000, 0.8660254037844387076, 1.000000000000000000, 0.8660254037844387076, 1.000000000000000000, 0.8660254037844387076, 1.000000000000000000, 0.8660254037844387076, 1.000000000000000000, 0.8660254037844387076, 1.000000000000000000, 0.8660254037844387076, 1.000000000000000000, 0.8660254037844387076, 1.000000000000000000, 0.8660254037844387076, 1.000000000000000000, 0.8660254037844387076, 1.000000000000000000, 0.8660254037844387076, 1.000000000000000000, 0.8660254037844387076, 1.000000000000000000, 0.8660254037844387076, 1.000000000000000000, 0.8660254037844387076, 1.000000000000000000, 0.8660254037844387076, 1.000000000000000000, 0.8660254037844387076, 1.000000000000000000, 0.8660254037844387076, 1.000000000000000000, 0.8660254037844387076, 1.000000000000000000, 0.8660254037844387076, 1.000000000000000000, 0.8660254037844387076, 1.000000000000000000, 0.8660254037844387076, 1.000000000000000000, 0.8660254037844387076, 1.000000000000000000, 0.8660254037844387076, 1.000000000000000000, 0.8660254037844387076, 1.000000000000000000, 0.8660254037844387076, 1.000000000000000000, 0.8660254037844387076, 1.000000000000000000, 0.8660254037844387076, 1.000000000000000000, 0.8660254037844387076, 1.000000000000000000, 0.8660254037844387076, 1.000000000000000000, 0.8660254037844387076, 1.000000000000000000, 0.8660254037844387076, 1.000000000000000000, 0.8660254037844387076, 1.000000000000000000, 0.8660254037844387076, 1.000000000000000000, 0.8660254037844387076, 1.000000000000000000, 0.8660254037844387076, 1.000000000000000000, 0.8660254037844387076, 1.000000000000000000, 0.8660254037844387076, 1.000000000000000000, 0.8660254037844387076, 1.000000000000000000, 0.8660254037844387076, 1.000000000000000000, 0.8660254037844387076, 1.000000000000000000, 0.8660254037844387076, 1.000000000000000000, 0.8660254037844387076, 1.000000000000000000, 0.8660254037844387076, 1.000000000000000000, 0.8660254037844387076, 1.000000000000000000, 0.8660254037844387076, 1.000000000000000000, 0.8660254037844387076, 1.000000000000000000, 0.8660254037844387076, 1.000000000000000000, 0.8660254037844387076, 1.000000000000000000, 0.8660254037844387076, 1.000000000000000000, 0.8660254037844387076, 1.000000000000000000, 0.8660254037844387076, 1.000000000000000000, 0.8660254037844387076, 1.000000000000000000, 0.8660254037844387076, 1.000000000000000000, 0.8660254037844387076, 1.000000000000000000, 0.8660254037844387076, 1.000000000000000000, 0.8660254037844387076, 1.000000000000000000, 0.8660254037844387076, 1.000000000000000000, 0.8660254037844387076, 1.000000000000000000, 0.8660254037844387076, 1.000000000000000000, 0.8660254037844387076, 1.000000000000000000, 0.8660254037844387076, 1.000000000000000000, 0.8660254037844387076, 1.000000000000000000, 0.8660254037844387076, 1.000000000000000000, 0.8660254037844387076, 1.000000000000000000, 0.8660254037844387076, 1.000000000000000000, 0.8660254037844387076, 1.000000000000000000, 0.8660254037844387076, 1.000000000000000000, 0.8660254037844387076, 1.000000000000000000, 0.8660254037844387076, 1.000000000000000000, 0.8660254037844387076, 1.000000000000000000, 0.9816628268209255381, 0.9683452906431576634 ) ) 
 REPRESENTATION_ITEM ( '' )  );
#41907=VERTEX_POINT ( 'NONE', #23936 ) ;
#41908=ORIENTED_EDGE ( 'NONE', *, *, #6438, .F. ) ;
#41913=CARTESIAN_POINT ( 'NONE',  ( 9.999999999999998224, 0.000000000000000000, -167.0000000000000000 ) ) ;
#41916=DIRECTION ( 'NONE',  ( -1.000000000000000000, 0.000000000000000000, 0.000000000000000000 ) ) ;
#41917=CARTESIAN_POINT ( 'NONE',  ( -10.81189881249999907, -6.242252689847864744, -136.9687500020483810 ) ) ;
#41918=CARTESIAN_POINT ( 'NONE',  ( -5.405949406249996869, 9.363379034771805109, -137.5312500020484094 ) ) ;
#41920=CARTESIAN_POINT ( 'NONE',  ( 10.81189881249999729, 0.000000000000000000, -143.8437500020483810 ) ) ;
#41921=LINE ( 'NONE', #18412, #35745 ) ;
#41923=CARTESIAN_POINT ( 'NONE',  ( -2.121150477449813534E-15, -11.54700538379251284, -173.3750000000000000 ) ) ;
#41925=CARTESIAN_POINT ( 'NONE',  ( -9.999999999999227285, -5.773502691896698735, -115.1249999999999574 ) ) ;
#41927=CARTESIAN_POINT ( 'NONE',  ( -5.405949406249996869, 9.363379034771805109, -60.84375000204836681 ) ) ;
#41928=CARTESIAN_POINT ( 'NONE',  ( -9.727846154639308907, -3.402673899969083759, -99.99999999999998579 ) ) ;
#41930=CARTESIAN_POINT ( 'NONE',  ( 7.644554776091147741E-16, 12.48450537969573659, -167.4687500020483810 ) ) ;
#41934=CARTESIAN_POINT ( 'NONE',  ( 10.81189881249999729, 0.000000000000000000, -39.03125000204838102 ) ) ;
#41936=CARTESIAN_POINT ( 'NONE',  ( -9.999999999999998224, 1.224646799147353059E-15, -100.2499999999999858 ) ) ;
#41938=CARTESIAN_POINT ( 'NONE',  ( 10.81189881249999551, -6.242252689847874514, -117.1562500020483952 ) ) ;
#41939=CARTESIAN_POINT ( 'NONE',  ( 10.00000000000000000, 5.773502691896255534, -137.2500000040967905 ) ) ;
#41944=CARTESIAN_POINT ( 'NONE',  ( -9.999999999999998224, 1.224646799147353059E-15, -154.6250000040967905 ) ) ;
#41945=CARTESIAN_POINT ( 'NONE',  ( -5.405949406249996869, 9.363379034771805109, -64.03125000204836681 ) ) ;
#41948=CARTESIAN_POINT ( 'NONE',  ( 10.00000000000076916, -5.773502691895816774, -106.0000000040967763 ) ) ;
#41954=VERTEX_POINT ( 'NONE', #39676 ) ;
#41957=ORIENTED_EDGE ( 'NONE', *, *, #8053, .T. ) ;
#41963=EDGE_LOOP ( 'NONE', ( #6035, #23715, #30308, #23174 ) ) ;
#41965=CARTESIAN_POINT ( 'NONE',  ( 9.999999999999996447, -5.773502691896262640, -29.12499999999998579 ) ) ;
#41969=CARTESIAN_POINT ( 'NONE',  ( 10.81189881249999551, -6.242252689847874514, -158.9687500020484094 ) ) ;
#41970=CARTESIAN_POINT ( 'NONE',  ( 7.644554776091147741E-16, 12.48450537969573659, -167.4687500020483526 ) ) ;
#41973=CARTESIAN_POINT ( 'NONE',  ( -9.999999999999998224, 1.224646799147353059E-15, -196.2500000000000000 ) ) ;
#41980=EDGE_CURVE ( 'NONE', #32014, #23494, #3229, .T. ) ;
#41981=CARTESIAN_POINT ( 'NONE',  ( 10.81189881249999729, 0.000000000000000000, -57.03125000204836681 ) ) ;
#41983=CARTESIAN_POINT ( 'NONE',  ( 7.070501591499377789E-16, 11.54700538379251284, -123.1249999999999858 ) ) ;
#41986=CARTESIAN_POINT ( 'NONE',  ( -10.81189881249999729, 1.324075727343319199E-15, -146.2812500020483810 ) ) ;
#41987=CARTESIAN_POINT ( 'NONE',  ( -10.81189881249999729, 6.242252689847871849, -153.9062500020483810 ) ) ;
#41990=CARTESIAN_POINT ( 'NONE',  ( -10.81189881249999729, 1.324075727343319199E-15, -90.59375000204838102 ) ) ;
#41993=CARTESIAN_POINT ( 'NONE',  ( -2.293366432827344421E-15, -12.48450537969573659, -184.7187500020484094 ) ) ;
#41995=CARTESIAN_POINT ( 'NONE',  ( 9.999999999999998224, 0.000000000000000000, -116.3750000040967905 ) ) ;
#41997=CARTESIAN_POINT ( 'NONE',  ( 5.405949406249992428, -9.363379034771808662, -81.28125000204839523 ) ) ;
#41999=CARTESIAN_POINT ( 'NONE',  ( -5.000000000000003553, -8.660254037844383745, -67.37500000409676204 ) ) ;
#42001=CARTESIAN_POINT ( 'NONE',  ( -5.405949406249996869, 9.363379034771805109, -21.84375000204835615 ) ) ;
#42004=CARTESIAN_POINT ( 'NONE',  ( 5.405949406249999534, 9.363379034771803333, -23.78125000204836681 ) ) ;
#42025=CARTESIAN_POINT ( 'NONE',  ( 10.81189881249999907, 6.242252689847868297, -155.9062500020484094 ) ) ;
#42027=DIRECTION ( 'NONE',  ( -0.000000000000000000, -0.000000000000000000, -1.000000000000000000 ) ) ;
#42031=CARTESIAN_POINT ( 'NONE',  ( 10.81189881249999551, -6.242252689847874514, -79.46875000204838102 ) ) ;
#42032=CARTESIAN_POINT ( 'NONE',  ( -2.293366432827344421E-15, -12.48450537969573659, -87.40625000204838102 ) ) ;
#42036=CARTESIAN_POINT ( 'NONE',  ( -5.405949406249996869, 9.363379034771805109, -166.0312500020484094 ) ) ;
#42037=CARTESIAN_POINT ( 'NONE',  ( 5.405949406249999534, 9.363379034771803333, -182.7812500020484094 ) ) ;
#42041=CARTESIAN_POINT ( 'NONE',  ( 7.070501591499377789E-16, 11.54700538379251284, -164.0000000040967905 ) ) ;
#42043=CARTESIAN_POINT ( 'NONE',  ( 5.405949406249999534, 9.363379034771803333, -16.09375000204835260 ) ) ;
#42045=CARTESIAN_POINT ( 'NONE',  ( 5.405949406249992428, -9.363379034771808662, -112.5937500020483810 ) ) ;
#42047=CARTESIAN_POINT ( 'NONE',  ( 10.81189881249999907, 6.242252689847868297, -17.90625000204837391 ) ) ;
#42050=CARTESIAN_POINT ( 'NONE',  ( 10.81189881249999551, -6.242252689847874514, -117.1562500020483810 ) ) ;
#42053=CARTESIAN_POINT ( 'NONE',  ( -4.999999999999996447, 8.660254037844387298, -91.87500000409677625 ) ) ;
#42054=CARTESIAN_POINT ( 'NONE',  ( -9.999999999999742428, -5.773502691896402084, -101.6249999999999716 ) ) ;
#42055=CARTESIAN_POINT ( 'NONE',  ( 5.405949406249999534, 9.363379034771803333, -47.59375000204838102 ) ) ;
#42060=ADVANCED_FACE ( 'NONE', ( #31272 ), #13095, .T. ) ;
#42061=CARTESIAN_POINT ( 'NONE',  ( -10.00000000000000000, -5.773502691896251982, -21.00000000409677270 ) ) ;
#42066=CARTESIAN_POINT ( 'NONE',  ( -9.999999999999998224, 1.224646799147353059E-15, -158.7500000000000000 ) ) ;
#42067=ORIENTED_EDGE ( 'NONE', *, *, #9956, .T. ) ;
#42074=CARTESIAN_POINT ( 'NONE',  ( -9.999999999999868550, 5.773502691896333694, -175.3750000000000000 ) ) ;
#42077=CARTESIAN_POINT ( 'NONE',  ( 10.81189881249999729, 0.000000000000000000, -183.0312500020484094 ) ) ;
#42079=CARTESIAN_POINT ( 'NONE',  ( 0.000000000000000000, 0.000000000000000000, -176.9999999999999432 ) ) ;
#42081=CARTESIAN_POINT ( 'NONE',  ( -10.81189881249999729, 1.324075727343319199E-15, -101.0937500020483810 ) ) ;
#42083=CARTESIAN_POINT ( 'NONE',  ( -2.293366432827344421E-15, -12.48450537969573659, -111.4062500020483952 ) ) ;
#42085=CARTESIAN_POINT ( 'NONE',  ( 10.81189881249999729, 6.242252689847867408, -119.7187500020483810 ) ) ;
#42088=CARTESIAN_POINT ( 'NONE',  ( -5.000000000000003553, -8.660254037844383745, -139.0000000000000000 ) ) ;
#42089=CARTESIAN_POINT ( 'NONE',  ( -10.00000000000000000, -5.773502691896251982, -10.12499999999996803 ) ) ;
#42092=CARTESIAN_POINT ( 'NONE',  ( -10.00000000000000000, -5.773502691896251982, -190.5000000040967905 ) ) ;
#42094=CARTESIAN_POINT ( 'NONE',  ( -10.81189881249999729, 6.242252689847871849, -35.21875000204835260 ) ) ;
#42095=CARTESIAN_POINT ( 'NONE',  ( -2.293366432827344421E-15, -12.48450537969573659, -145.7187500020484094 ) ) ;
#42098=CARTESIAN_POINT ( 'NONE',  ( 4.999999999999992006, -8.660254037844389075, -65.24999999999997158 ) ) ;
#42099=CARTESIAN_POINT ( 'NONE',  ( 5.405949406249992428, -9.363379034771808662, -138.2812500020483810 ) ) ;
#42103=CARTESIAN_POINT ( 'NONE',  ( -2.121150477449813534E-15, -11.54700538379251284, -115.2500000040967763 ) ) ;
#42105=CARTESIAN_POINT ( 'NONE',  ( 5.405949406249992428, -9.363379034771808662, -72.09375000204836681 ) ) ;
#42112=CARTESIAN_POINT ( 'NONE',  ( -2.293366432827344421E-15, -12.48450537969573659, -39.40625000204836681 ) ) ;
#42113=CARTESIAN_POINT ( 'NONE',  ( -9.999999999999996447, 5.773502691896259975, -166.3750000000000000 ) ) ;
#42116=CARTESIAN_POINT ( 'NONE',  ( -5.000000000000003553, -8.660254037844383745, -164.8750000040967905 ) ) ;
#42129=CARTESIAN_POINT ( 'NONE',  ( -5.000000000000003553, -8.660254037844383745, -176.5000000000000000 ) ) ;
#42130=CARTESIAN_POINT ( 'NONE',  ( 10.81189881249999907, 6.242252689847868297, -130.2187500020483810 ) ) ;
#42131=CARTESIAN_POINT ( 'NONE',  ( -10.81189881249999729, 6.242252689847871849, -140.4062500020484094 ) ) ;
#42134=CARTESIAN_POINT ( 'NONE',  ( -5.405949406249996869, 9.363379034771805109, -143.3437500020483810 ) ) ;
#42135=CYLINDRICAL_SURFACE ( 'NONE', #4706, 9.999999999999998224 ) ;
#42137=CARTESIAN_POINT ( 'NONE',  ( 9.999999999999996447, -5.773502691896262640, -161.1250000000000284 ) ) ;
#42138=AXIS2_PLACEMENT_3D ( 'NONE', #10681, #14333, #40245 ) ;
#42141=CARTESIAN_POINT ( 'NONE',  ( 10.81189881249999729, 0.000000000000000000, -64.34375000204836681 ) ) ;
#42143=CARTESIAN_POINT ( 'NONE',  ( -5.405949406250003975, -9.363379034771801557, -168.3437500020484094 ) ) ;
#42148=CARTESIAN_POINT ( 'NONE',  ( -10.00000000000000000, -5.773502691896251982, -94.12499999999998579 ) ) ;
#42150=CARTESIAN_POINT ( 'NONE',  ( -10.81189881249999729, 1.324075727343319199E-15, -120.7812500020483952 ) ) ;
#42151=CARTESIAN_POINT ( 'NONE',  ( -9.999999999999998224, 1.224646799147353059E-15, -142.6250000040967905 ) ) ;
#42156=CARTESIAN_POINT ( 'NONE',  ( 10.81189881249999907, 6.242252689847868297, -59.90625000204838102 ) ) ;
#42178=CARTESIAN_POINT ( 'NONE',  ( -5.000000000000003553, -8.660254037844383745, -26.49999999999996803 ) ) ;
#42181=CARTESIAN_POINT ( 'NONE',  ( -5.405949406250003975, -9.363379034771801557, -157.8437500020483810 ) ) ;
#42183=CARTESIAN_POINT ( 'NONE',  ( -10.81189881249999729, -6.242252689847864744, -171.4687500020483526 ) ) ;
#42184=DIRECTION ( 'NONE',  ( -0.000000000000000000, -0.000000000000000000, -1.000000000000000000 ) ) ;
#42186=CARTESIAN_POINT ( 'NONE',  ( -10.00000000000000000, -5.773502691896251982, -190.1250000000000284 ) ) ;
#42192=CARTESIAN_POINT ( 'NONE',  ( -10.81189881249999729, 1.324075727343319199E-15, -60.78125000204836681 ) ) ;
#42194=CARTESIAN_POINT ( 'NONE',  ( 7.070501591499377789E-16, 11.54700538379251284, -121.6249999999999858 ) ) ;
#42196=CARTESIAN_POINT ( 'NONE',  ( -2.293366432827344421E-15, -12.48450537969573659, -141.4062500020484094 ) ) ;
#42197=CARTESIAN_POINT ( 'NONE',  ( -10.81189881249999907, -6.242252689847864744, -158.1562500020484094 ) ) ;
#42200=CARTESIAN_POINT ( 'NONE',  ( -2.121150477449813534E-15, -11.54700538379251284, -179.3750000000000000 ) ) ;
#42201=CARTESIAN_POINT ( 'NONE',  ( 5.405949406249999534, 9.363379034771803333, -91.09375000204838102 ) ) ;
#42202=ORIENTED_EDGE ( 'NONE', *, *, #18426, .T. ) ;
#42204=CARTESIAN_POINT ( 'NONE',  ( -5.405949406250003975, -9.363379034771801557, -190.8437500020484094 ) ) ;
#42208=CARTESIAN_POINT ( 'NONE',  ( -2.293366432827344421E-15, -12.48450537969573659, -85.90625000204839523 ) ) ;
#42210=CARTESIAN_POINT ( 'NONE',  ( 5.000000000000000000, 8.660254037844385522, -63.62500000409676204 ) ) ;
#42211=CARTESIAN_POINT ( 'NONE',  ( 5.405949406249999534, 9.363379034771803333, -17.59375000204835260 ) ) ;
#42212=ORIENTED_EDGE ( 'NONE', *, *, #12691, .T. ) ;
#42214=CARTESIAN_POINT ( 'NONE',  ( 7.644554776091147741E-16, 12.48450537969573659, -13.15625000204836859 ) ) ;
#42217=CARTESIAN_POINT ( 'NONE',  ( 9.999999999999998224, 0.000000000000000000, -114.8750000040967905 ) ) ;
#42222=EDGE_LOOP ( 'NONE', ( #19718, #14991, #35356, #20673 ) ) ;
#42223=CARTESIAN_POINT ( 'NONE',  ( -10.00000000000051337, 5.773502691895962435, -115.7500000040967905 ) ) ;
#42226=( BOUNDED_CURVE ( )  B_SPLINE_CURVE ( 2, ( #41642, #25273, #22022, #5622, #18774, #11436, #24634 ),
 .UNSPECIFIED., .F., .F. ) 
 B_SPLINE_CURVE_WITH_KNOTS ( ( 3, 2, 2, 3 ),
 ( 0.2761194029850747578, 0.2773631840796020875, 0.2786069651741294728, 0.2798507462686568026 ),
 .UNSPECIFIED. ) 
 CURVE ( )  GEOMETRIC_REPRESENTATION_ITEM ( )  RATIONAL_B_SPLINE_CURVE ( ( 0.9999999999999880096, 0.8660254037844506980, 1.000000000000000000, 0.8660254037844387076, 1.000000000000000000, 0.8660254037844267172, 1.000000000000011990 ) ) 
 REPRESENTATION_ITEM ( '' )  );
#42228=ORIENTED_EDGE ( 'NONE', *, *, #41255, .T. ) ;
#42234=CARTESIAN_POINT ( 'NONE',  ( 7.608343550068628502, 7.301534541193676731, -99.99999999999997158 ) ) ;
#42237=CARTESIAN_POINT ( 'NONE',  ( 7.644554776091147741E-16, 12.48450537969573659, -160.1562500020484094 ) ) ;
#42243=CARTESIAN_POINT ( 'NONE',  ( -5.405949406250003975, -9.363379034771801557, -79.84375000204838102 ) ) ;
#42244=CARTESIAN_POINT ( 'NONE',  ( -5.405949406249996869, 9.363379034771805109, -83.53125000204838102 ) ) ;
#42247=CARTESIAN_POINT ( 'NONE',  ( 7.644554776091147741E-16, 12.48450537969573659, -166.1562500020483810 ) ) ;
#42248=CARTESIAN_POINT ( 'NONE',  ( -5.405949406249996869, 9.363379034771805109, -184.0312500020484094 ) ) ;
#42249=CARTESIAN_POINT ( 'NONE',  ( -2.121150477449813534E-15, -11.54700538379251284, -158.7500000040968189 ) ) ;
#42251=CARTESIAN_POINT ( 'NONE',  ( -2.293366432827344421E-15, -12.48450537969573659, -3.218750002048353931 ) ) ;
#42253=CARTESIAN_POINT ( 'NONE',  ( 10.81189881249999551, -6.242252689847874514, -112.4687500020483810 ) ) ;
#42255=CARTESIAN_POINT ( 'NONE',  ( -2.293366432827344421E-15, -12.48450537969573659, -9.406250002048365033 ) ) ;
#42258=CARTESIAN_POINT ( 'NONE',  ( -10.81189881249999907, -6.242252689847864744, -107.1562500020483952 ) ) ;
#42261=CARTESIAN_POINT ( 'NONE',  ( -10.00000000000000000, -5.773502691896251982, -87.00000000409677625 ) ) ;
#42263=CARTESIAN_POINT ( 'NONE',  ( -10.81189881249999907, -6.242252689847864744, -42.46875000204835970 ) ) ;
#42267=CARTESIAN_POINT ( 'NONE',  ( -9.999999999999998224, 1.224646799147353059E-15, -24.12500000409675849 ) ) ;
#42272=CARTESIAN_POINT ( 'NONE',  ( 4.999999999999992006, -8.660254037844389075, -152.2500000000000000 ) ) ;
#42274=EDGE_CURVE ( 'NONE', #31861, #13677, #1913, .T. ) ;
#42276=ADVANCED_FACE ( 'NONE', ( #4285 ), #31052, .F. ) ;
#42280=EDGE_LOOP ( 'NONE', ( #25899, #18354, #32779, #3699 ) ) ;
#42285=CARTESIAN_POINT ( 'NONE',  ( 5.405949406249999534, 9.363379034771803333, -184.2812500020484094 ) ) ;
#42287=CARTESIAN_POINT ( 'NONE',  ( 9.999999999999994671, -5.773502691896262640, -132.6250000000000000 ) ) ;
#42290=CARTESIAN_POINT ( 'NONE',  ( -10.81189881249999729, 6.242252689847871849, -99.71875000204839523 ) ) ;
#42292=CARTESIAN_POINT ( 'NONE',  ( -10.81189881249999907, -6.242252689847864744, -110.1562500020483952 ) ) ;
#42294=CARTESIAN_POINT ( 'NONE',  ( 10.81189881249999551, -6.242252689847874514, -121.4687500020484237 ) ) ;
#42297=CARTESIAN_POINT ( 'NONE',  ( 9.999999999999998224, 0.000000000000000000, -138.5000000000000000 ) ) ;
#42298=CARTESIAN_POINT ( 'NONE',  ( -10.00000000000000000, -5.773502691896251982, -5.624999999999963585 ) ) ;
#42299=EDGE_CURVE ( 'NONE', #21209, #28518, #22612, .T. ) ;
#42302=CARTESIAN_POINT ( 'NONE',  ( 4.999999999999992006, -8.660254037844389075, -181.1250000040967905 ) ) ;
#42304=CARTESIAN_POINT ( 'NONE',  ( -10.81189881249999907, -6.242252689847864744, -31.96875000204834905 ) ) ;
#42305=CARTESIAN_POINT ( 'NONE',  ( -5.000000000000003553, -8.660254037844383745, -107.8750000040967763 ) ) ;
#42306=CARTESIAN_POINT ( 'NONE',  ( 5.405949406249992428, -9.363379034771808662, -139.5937500020483810 ) ) ;
#42309=CARTESIAN_POINT ( 'NONE',  ( -9.999999999999998224, 1.224646799147353059E-15, -67.24999999999997158 ) ) ;
#42310=CARTESIAN_POINT ( 'NONE',  ( -10.81189881249999729, 6.242252689847871849, -132.9062500020483810 ) ) ;
#42314=CARTESIAN_POINT ( 'NONE',  ( -4.999999999999996447, 8.660254037844387298, -114.3750000040967763 ) ) ;
#42316=CARTESIAN_POINT ( 'NONE',  ( -10.81189881249999729, 6.242252689847871849, -62.21875000204838102 ) ) ;
#42320=EDGE_CURVE ( 'NONE', #41736, #31697, #2220, .T. ) ;
#42322=CARTESIAN_POINT ( 'NONE',  ( -4.999999999999996447, 8.660254037844387298, -46.87500000409677625 ) ) ;
#42323=CARTESIAN_POINT ( 'NONE',  ( 7.644554776091147741E-16, 12.48450537969573659, -32.65625000204835970 ) ) ;
#42328=ORIENTED_EDGE ( 'NONE', *, *, #30246, .T. ) ;
#42329=ORIENTED_EDGE ( 'NONE', *, *, #2100, .T. ) ;
#42338=CARTESIAN_POINT ( 'NONE',  ( -9.999999999999998224, 1.224646799147353059E-15, -100.2499999999999858 ) ) ;
#42339=CARTESIAN_POINT ( 'NONE',  ( 5.405949406249992428, -9.363379034771808662, -127.5937500020483668 ) ) ;
#42340=CARTESIAN_POINT ( 'NONE',  ( 10.81189881249999907, 6.242252689847868297, -133.4062500020483810 ) ) ;
#42342=CARTESIAN_POINT ( 'NONE',  ( -10.81189881249999729, -6.242252689847864744, -145.9687500020484094 ) ) ;
#42343=CARTESIAN_POINT ( 'NONE',  ( 10.01657826025561704, -4.085534667769917583, -180.0000000000000284 ) ) ;
#42345=CARTESIAN_POINT ( 'NONE',  ( 5.000000000000000000, 8.660254037844385522, -165.2500000000000000 ) ) ;
#42349=CARTESIAN_POINT ( 'NONE',  ( 10.81189881249999907, 6.242252689847868297, -55.21875000204836681 ) ) ;
#42351=CARTESIAN_POINT ( 'NONE',  ( 10.81189881249999907, 6.242252689847868297, -158.7187500020483810 ) ) ;
#42356=CARTESIAN_POINT ( 'NONE',  ( -2.121150477449813534E-15, -11.54700538379251284, -89.37499999999997158 ) ) ;
#42358=CARTESIAN_POINT ( 'NONE',  ( 10.81189881249999551, -6.242252689847874514, -120.1562500020483952 ) ) ;
#42359=CARTESIAN_POINT ( 'NONE',  ( 4.999999999999992006, -8.660254037844389075, -139.1250000040967905 ) ) ;
#42364=CARTESIAN_POINT ( 'NONE',  ( 7.644554776091147741E-16, 12.48450537969573659, -58.15625000204838102 ) ) ;
#42371=ORIENTED_EDGE ( 'NONE', *, *, #38942, .F. ) ;
#42377=VERTEX_POINT ( 'NONE', #31698 ) ;
#42387=CARTESIAN_POINT ( 'NONE',  ( -10.00000000000000000, -5.773502691896251982, -31.12499999999995737 ) ) ;
#42390=CARTESIAN_POINT ( 'NONE',  ( -10.81189881249999729, 6.242252689847871849, -147.7187500020484094 ) ) ;
#42391=CARTESIAN_POINT ( 'NONE',  ( -5.405949406250003975, -9.363379034771801557, -172.8437500020484094 ) ) ;
#42392=CARTESIAN_POINT ( 'NONE',  ( -10.00000000000051337, 5.773502691895962435, -123.2500000040967763 ) ) ;
#42394=CYLINDRICAL_SURFACE ( 'NONE', #39147, 9.999999999999998224 ) ;
#42395=CARTESIAN_POINT ( 'NONE',  ( -4.999999999999996447, 8.660254037844387298, -190.5000000000000000 ) ) ;
#42400=CARTESIAN_POINT ( 'NONE',  ( 10.81189881249999907, 6.242252689847868297, -197.7187500020484094 ) ) ;
#42402=CARTESIAN_POINT ( 'NONE',  ( 5.405949406249999534, 9.363379034771803333, -56.78125000204836681 ) ) ;
#42404=CARTESIAN_POINT ( 'NONE',  ( 9.999999999999998224, 0.000000000000000000, -117.5000000000000000 ) ) ;
#42407=CARTESIAN_POINT ( 'NONE',  ( 10.81189881249999729, 6.242252689847867408, -140.9062500020484094 ) ) ;
#42408=CARTESIAN_POINT ( 'NONE',  ( 10.81189881249999551, -6.242252689847874514, -153.1562500020484379 ) ) ;
#42411=CARTESIAN_POINT ( 'NONE',  ( -10.81189881249999729, 1.324075727343319199E-15, -89.09375000204838102 ) ) ;
#42414=CARTESIAN_POINT ( 'NONE',  ( 5.405949406249992428, -9.363379034771808662, -189.0937500020483810 ) ) ;
#42416=CARTESIAN_POINT ( 'NONE',  ( 9.999999999999998224, 1.224646799147353059E-15, -99.99999999999998579 ) ) ;
#42418=CARTESIAN_POINT ( 'NONE',  ( -10.81189881249999729, 1.324075727343319199E-15, -86.28125000204838102 ) ) ;
#42420=VECTOR ( 'NONE', #30996, 1000.000000000000000 ) ;
#42421=CARTESIAN_POINT ( 'NONE',  ( 7.070501591499377789E-16, 11.54700538379251284, -63.50000000409677625 ) ) ;
#42422=CARTESIAN_POINT ( 'NONE',  ( -10.81189881249999729, 1.324075727343319199E-15, -21.59375000204835615 ) ) ;
#42425=CARTESIAN_POINT ( 'NONE',  ( 7.644554776091147741E-16, 12.48450537969573659, -10.15625000204836681 ) ) ;
#42434=EDGE_CURVE ( 'NONE', #40786, #17582, #3589, .T. ) ;
#42435=CARTESIAN_POINT ( 'NONE',  ( 9.999999999999742428, 5.773502691896404748, -116.2500000040967620 ) ) ;
#42437=VERTEX_POINT ( 'NONE', #12236 ) ;
#42445=VECTOR ( 'NONE', #12087, 1000.000000000000000 ) ;
#42448=CARTESIAN_POINT ( 'NONE',  ( 10.81189881249999907, 6.242252689847868297, -160.4062500020484094 ) ) ;
#42454=CARTESIAN_POINT ( 'NONE',  ( -2.293366432827344421E-15, -12.48450537969573659, -81.21875000204838102 ) ) ;
#42455=CARTESIAN_POINT ( 'NONE',  ( 5.405949406249992428, -9.363379034771808662, -85.78125000204838102 ) ) ;
#42458=CARTESIAN_POINT ( 'NONE',  ( 10.81189881249999551, -6.242252689847874514, -166.6562500020484094 ) ) ;
#42459=CARTESIAN_POINT ( 'NONE',  ( 5.405949406249992428, -9.363379034771808662, -183.2812500020484094 ) ) ;
#42460=CARTESIAN_POINT ( 'NONE',  ( -10.00000000000000000, -5.773502691896251982, -154.5000000040967905 ) ) ;
#42461=DIRECTION ( 'NONE',  ( -0.000000000000000000, -0.000000000000000000, -1.000000000000000000 ) ) ;
#42462=CARTESIAN_POINT ( 'NONE',  ( 5.405949406249992428, -9.363379034771808662, -6.093750002048370362 ) ) ;
#42463=CARTESIAN_POINT ( 'NONE',  ( -5.405949406249996869, 9.363379034771805109, -116.3437500020483810 ) ) ;
#42466=CARTESIAN_POINT ( 'NONE',  ( 10.81189881249999729, 0.000000000000000000, -16.53125000204835970 ) ) ;
#42469=CARTESIAN_POINT ( 'NONE',  ( -10.81189881249999907, -6.242252689847864744, -110.1562500020483952 ) ) ;
#42472=CARTESIAN_POINT ( 'NONE',  ( 9.999999999999996447, -5.773502691896262640, -88.00000000409677625 ) ) ;
#42473=CARTESIAN_POINT ( 'NONE',  ( 5.405949406249999534, 9.363379034771803333, -38.59375000204837391 ) ) ;
#42477=( BOUNDED_CURVE ( )  B_SPLINE_CURVE ( 2, ( #19246, #22709, #36080, #35876, #32644, #3071, #16197 ),
 .UNSPECIFIED., .F., .F. ) 
 B_SPLINE_CURVE_WITH_KNOTS ( ( 3, 2, 2, 3 ),
 ( 0.2388059701492538378, 0.2400497512437811953, 0.2412935323383085806, 0.2425373134328359381 ),
 .UNSPECIFIED. ) 
 CURVE ( )  GEOMETRIC_REPRESENTATION_ITEM ( )  RATIONAL_B_SPLINE_CURVE ( ( 0.9999999999999880096, 0.8660254037844506980, 1.000000000000000000, 0.8660254037844387076, 1.000000000000000000, 0.8660254037844267172, 1.000000000000011990 ) ) 
 REPRESENTATION_ITEM ( '' )  );
#42478=CARTESIAN_POINT ( 'NONE',  ( 7.070501591499377789E-16, 11.54700538379251284, -9.500000004096758488 ) ) ;
#42480=CARTESIAN_POINT ( 'NONE',  ( -9.999999999999742428, -5.773502691896402084, -120.0000000040967905 ) ) ;
#42489=CARTESIAN_POINT ( 'NONE',  ( 7.070501591499376803E-16, 11.54700538379251284, -175.6250000000000000 ) ) ;
#42491=CARTESIAN_POINT ( 'NONE',  ( 5.405949406249999534, 9.363379034771803333, -176.7812500020484094 ) ) ;
#42495=CARTESIAN_POINT ( 'NONE',  ( -10.81189881249999907, -6.242252689847864744, -103.9687500020483668 ) ) ;
#42496=CARTESIAN_POINT ( 'NONE',  ( 10.00000000000051159, -5.773502691895965988, -143.1250000000000000 ) ) ;
#42497=CARTESIAN_POINT ( 'NONE',  ( 10.81189881249999907, 6.242252689847868297, -110.9062500020483952 ) ) ;
#42499=CARTESIAN_POINT ( 'NONE',  ( -5.405949406250003975, -9.363379034771801557, -117.3437500020483810 ) ) ;
#42502=CARTESIAN_POINT ( 'NONE',  ( 7.070501591499377789E-16, 11.54700538379251284, -139.6250000000000000 ) ) ;
#42503=CARTESIAN_POINT ( 'NONE',  ( 4.999999999999992006, -8.660254037844389075, -3.749999999999975575 ) ) ;
#42508=CARTESIAN_POINT ( 'NONE',  ( -9.999999999999998224, 1.224646799147353059E-15, -183.1250000040967905 ) ) ;
#42510=CARTESIAN_POINT ( 'NONE',  ( 10.81189881249999729, 0.000000000000000000, -26.84375000204835970 ) ) ;
#42511=CARTESIAN_POINT ( 'NONE',  ( -5.000000000000003553, -8.660254037844383745, -105.9999999999999858 ) ) ;
#42512=CARTESIAN_POINT ( 'NONE',  ( 7.644554776091147741E-16, 12.48450537969573659, -141.9687500020483810 ) ) ;
#42515=CARTESIAN_POINT ( 'NONE',  ( 10.00000000000051159, -5.773502691895965988, -147.6249999999999716 ) ) ;
#42516=EDGE_CURVE ( 'NONE', #15509, #31308, #15411, .T. ) ;
#42517=CARTESIAN_POINT ( 'NONE',  ( -9.999999999999998224, 5.773502691896259087, -64.37499999999998579 ) ) ;
#42518=CARTESIAN_POINT ( 'NONE',  ( 10.81189881249999551, -6.242252689847874514, -132.1562500020484094 ) ) ;
#42523=CARTESIAN_POINT ( 'NONE',  ( -2.121150477449813534E-15, -11.54700538379251284, -106.2500000040967763 ) ) ;
#42525=CARTESIAN_POINT ( 'NONE',  ( 10.81189881249999729, 0.000000000000000000, -68.84375000204836681 ) ) ;
#42531=CARTESIAN_POINT ( 'NONE',  ( 5.000000000000000000, 8.660254037844385522, -35.12500000409676915 ) ) ;
#42532=CARTESIAN_POINT ( 'NONE',  ( 5.405949406249999534, 9.363379034771803333, -38.78125000204838102 ) ) ;
#42533=( BOUNDED_CURVE ( )  B_SPLINE_CURVE ( 2, ( #35681, #21867, #42129, #2451, #29198, #38908, #12348 ),
 .UNSPECIFIED., .F., .F. ) 
 B_SPLINE_CURVE_WITH_KNOTS ( ( 3, 2, 2, 3 ),
 ( 0.1156716417910447492, 0.1169154228855721483, 0.1181592039800995753, 0.1194029850746269744 ),
 .UNSPECIFIED. ) 
 CURVE ( )  GEOMETRIC_REPRESENTATION_ITEM ( )  RATIONAL_B_SPLINE_CURVE ( ( 1.000000000000003109, 0.8660254037844358210, 1.000000000000000000, 0.8660254037844387076, 1.000000000000000000, 0.8660254037844267172, 1.000000000000011990 ) ) 
 REPRESENTATION_ITEM ( '' )  );
#42547=CARTESIAN_POINT ( 'NONE',  ( -9.999999999999998224, 1.224646799147353059E-15, -103.2500000000000000 ) ) ;
#42550=CARTESIAN_POINT ( 'NONE',  ( 9.999999999999998224, 0.000000000000000000, -119.0000000000000000 ) ) ;
#42551=CARTESIAN_POINT ( 'NONE',  ( 10.81189881249999551, -6.242252689847874514, -125.9687500020483810 ) ) ;
#42552=CARTESIAN_POINT ( 'NONE',  ( -5.405949406250003975, -9.363379034771801557, -129.5312500020484094 ) ) ;
#42554=CARTESIAN_POINT ( 'NONE',  ( 5.405949406249992428, -9.363379034771808662, -135.0937500020483810 ) ) ;
#42557=CARTESIAN_POINT ( 'NONE',  ( 9.999999999999996447, -5.773502691896262640, -159.6250000000000284 ) ) ;
#42558=CARTESIAN_POINT ( 'NONE',  ( 10.81189881249999729, 0.000000000000000000, -1.531250002048373249 ) ) ;
#42561=CARTESIAN_POINT ( 'NONE',  ( 10.81189881249999729, 0.000000000000000000, -50.84375000204835260 ) ) ;
#42563=CARTESIAN_POINT ( 'NONE',  ( 5.405949406249999534, 9.363379034771803333, -164.5937500020484094 ) ) ;
#42569=CARTESIAN_POINT ( 'NONE',  ( 4.999999999999992006, -8.660254037844389075, -92.24999999999998579 ) ) ;
#42572=CARTESIAN_POINT ( 'NONE',  ( 10.81189881249999729, 6.242252689847867408, -115.4062500020484094 ) ) ;
#42573=CARTESIAN_POINT ( 'NONE',  ( 10.00000000000000000, 5.773502691896255534, -131.2500000040967905 ) ) ;
#42579=CARTESIAN_POINT ( 'NONE',  ( 5.405949406249992428, -9.363379034771808662, -60.28125000204836681 ) ) ;
#42583=VECTOR ( 'NONE', #13299, 1000.000000000000000 ) ;
#42587=CARTESIAN_POINT ( 'NONE',  ( 5.000000000000000000, 8.660254037844385522, -131.1250000040967620 ) ) ;
#42593=ORIENTED_EDGE ( 'NONE', *, *, #40781, .F. ) ;
#42594=( BOUNDED_CURVE ( )  B_SPLINE_CURVE ( 2, ( #38664, #5224, #18380, #18809, #12318, #31995, #28543 ),
 .UNSPECIFIED., .F., .F. ) 
 B_SPLINE_CURVE_WITH_KNOTS ( ( 3, 2, 2, 3 ),
 ( 0.2686567164179105571, 0.2699004975124379424, 0.2711442786069652722, 0.2723880597014926574 ),
 .UNSPECIFIED. ) 
 CURVE ( )  GEOMETRIC_REPRESENTATION_ITEM ( )  RATIONAL_B_SPLINE_CURVE ( ( 0.9999999999999880096, 0.8660254037844506980, 1.000000000000000000, 0.8660254037844387076, 1.000000000000000000, 0.8660254037844267172, 1.000000000000011990 ) ) 
 REPRESENTATION_ITEM ( '' )  );
#42600=CARTESIAN_POINT ( 'NONE',  ( -9.999999999999998224, 5.773502691896259087, -28.37499999999998224 ) ) ;
#42603=CARTESIAN_POINT ( 'NONE',  ( -10.81189881249999907, -6.242252689847864744, -150.4687500020484094 ) ) ;
#42604=CARTESIAN_POINT ( 'NONE',  ( -2.293366432827344421E-15, -12.48450537969573659, -172.7187500020483810 ) ) ;
#42606=CARTESIAN_POINT ( 'NONE',  ( 4.999999999999992006, -8.660254037844389075, -185.2500000000000000 ) ) ;
#42611=CARTESIAN_POINT ( 'NONE',  ( -5.405949406249996869, 9.363379034771805109, -182.3437500020483810 ) ) ;
#42613=CARTESIAN_POINT ( 'NONE',  ( -5.405949406249996869, 9.363379034771805109, -62.53125000204837391 ) ) ;
#42615=CARTESIAN_POINT ( 'NONE',  ( -10.00000000000000000, -5.773502691896251982, -115.1249999999999858 ) ) ;
#42617=CARTESIAN_POINT ( 'NONE',  ( -10.81189881249999729, 1.324075727343319199E-15, -138.7812500020483810 ) ) ;
#42618=CARTESIAN_POINT ( 'NONE',  ( -5.405949406250003975, -9.363379034771801557, -158.0312500020484094 ) ) ;
#42620=CARTESIAN_POINT ( 'NONE',  ( 5.405949406249992428, -9.363379034771808662, -87.09375000204836681 ) ) ;
#42623=CARTESIAN_POINT ( 'NONE',  ( 7.644554776091147741E-16, 12.48450537969573659, -188.4687500020484094 ) ) ;
#42626=CARTESIAN_POINT ( 'NONE',  ( -5.000000000000003553, -8.660254037844383745, -124.0000000000000000 ) ) ;
#42627=CARTESIAN_POINT ( 'NONE',  ( -5.405949406249996869, 9.363379034771805109, -82.03125000204839523 ) ) ;
#42629=CARTESIAN_POINT ( 'NONE',  ( -9.999999999999998224, 5.773502691896259087, -57.25000000409677625 ) ) ;
#42630=CARTESIAN_POINT ( 'NONE',  ( -10.81189881249999729, 1.324075727343319199E-15, -20.09375000204835615 ) ) ;
#42634=CARTESIAN_POINT ( 'NONE',  ( 5.405949406249999534, 9.363379034771803333, -14.78125000204835793 ) ) ;
#42639=( BOUNDED_CURVE ( )  B_SPLINE_CURVE ( 2, ( #5731, #21907, #28825, #35087, #5512, #18663, #28613 ),
 .UNSPECIFIED., .F., .F. ) 
 B_SPLINE_CURVE_WITH_KNOTS ( ( 3, 2, 2, 3 ),
 ( 0.1007462686567163757, 0.1019900497512437887, 0.1032338308457712017, 0.1044776119402986148 ),
 .UNSPECIFIED. ) 
 CURVE ( )  GEOMETRIC_REPRESENTATION_ITEM ( )  RATIONAL_B_SPLINE_CURVE ( ( 1.000000000000004441, 0.8660254037844342667, 1.000000000000000000, 0.8660254037844387076, 1.000000000000000000, 0.8660254037844267172, 1.000000000000011990 ) ) 
 REPRESENTATION_ITEM ( '' )  );
#42659=CARTESIAN_POINT ( 'NONE',  ( 5.405949406249999534, 9.363379034771803333, -160.2812500020484094 ) ) ;
#42665=CARTESIAN_POINT ( 'NONE',  ( 10.81189881249999551, -6.242252689847874514, -74.96875000204838102 ) ) ;
#42666=CARTESIAN_POINT ( 'NONE',  ( 10.81189881249999551, -6.242252689847874514, -81.15625000204839523 ) ) ;
#42669=CARTESIAN_POINT ( 'NONE',  ( 7.644554776091147741E-16, 12.48450537969573659, -167.6562500020484094 ) ) ;
#42670=CARTESIAN_POINT ( 'NONE',  ( -10.81189881249999729, 1.324075727343319199E-15, -183.7812500020484094 ) ) ;
#42671=CARTESIAN_POINT ( 'NONE',  ( -9.999999999999998224, 5.773502691896259087, -153.2500000040967620 ) ) ;
#42673=CARTESIAN_POINT ( 'NONE',  ( 10.81189881249999729, 0.000000000000000000, -8.843750002048345493 ) ) ;
#42675=CARTESIAN_POINT ( 'NONE',  ( 10.81189881249999551, -6.242252689847874514, -115.4687500020483810 ) ) ;
#42677=CARTESIAN_POINT ( 'NONE',  ( -2.293366432827344421E-15, -12.48450537969573659, -10.90625000204836681 ) ) ;
#42680=CARTESIAN_POINT ( 'NONE',  ( 10.81189881249999907, 6.242252689847868297, -110.9062500020483952 ) ) ;
#42684=CARTESIAN_POINT ( 'NONE',  ( -2.121150477449813534E-15, -11.54700538379251284, -80.75000000409677625 ) ) ;
#42685=CARTESIAN_POINT ( 'NONE',  ( 4.999999999999992006, -8.660254037844389075, -140.6250000040967905 ) ) ;
#42686=CARTESIAN_POINT ( 'NONE',  ( -10.81189881249999907, -6.242252689847864744, -39.46875000204835970 ) ) ;
#42711=COLOUR_RGB('Sky Blue', 0.31764706, 0.68627451, 0.89019608);
#42712=FILL_AREA_STYLE_COLOUR('',#42711);
#42713=FILL_AREA_STYLE('',(#42712));
#42714=SURFACE_STYLE_FILL_AREA(#42713);
#42715=SURFACE_SIDE_STYLE('',(#42714));
#42716=SURFACE_STYLE_USAGE(.BOTH.,#42715);
#42717=PRESENTATION_STYLE_ASSIGNMENT((#42716));
#42745=STYLED_ITEM('',(#42717),#28380);
#42746=MECHANICAL_DESIGN_GEOMETRIC_PRESENTATION_REPRESENTATION('',(#42745),#29026);
ENDSEC;
END-ISO-10303-21;
